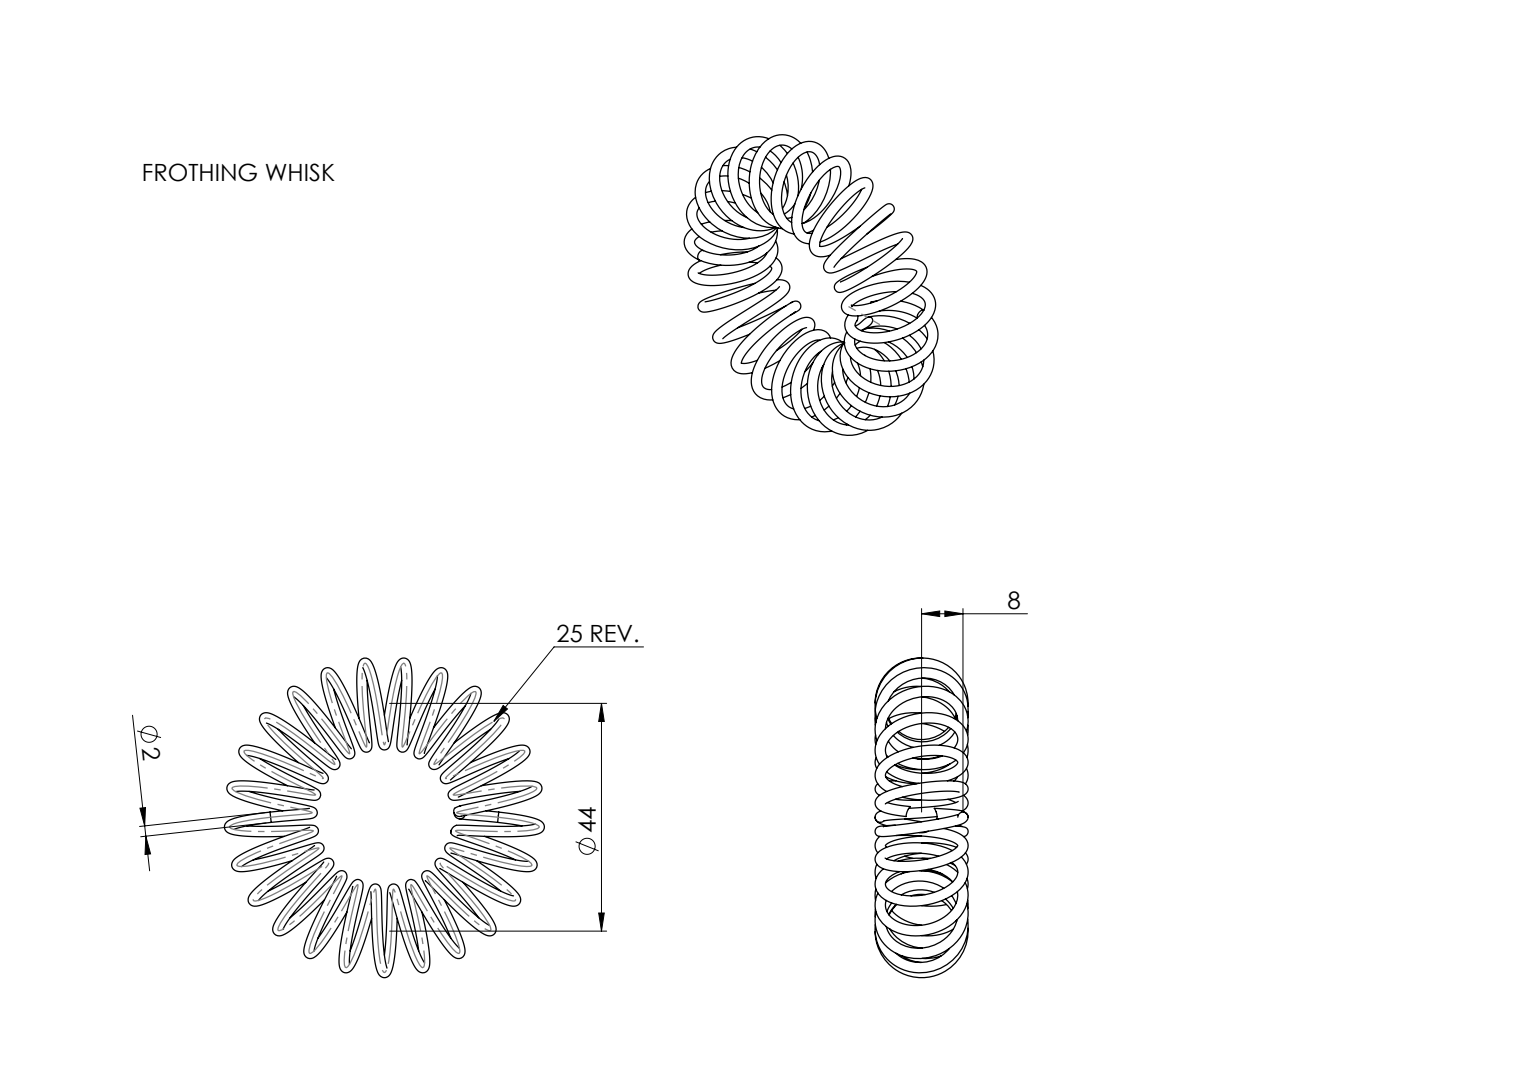
ISO-10303-21;
HEADER;
FILE_DESCRIPTION (('STEP AP214'),
    '1' );
FILE_NAME ('Frothing Whisk.step',
    '2026-10-08T15:02:10',
    ( '' ),
    ( '' ),
    'SwSTEP 2.0',
    'SolidWorks 2026',
    '' );
FILE_SCHEMA (( 'AUTOMOTIVE_DESIGN' ));
ENDSEC;

DATA;
#1=CARTESIAN_POINT ( 'NONE',  ( -16.20471097821853235, -2.781505378741172319, -220.1484675126197317 ) ) ;
#2=CARTESIAN_POINT ( 'NONE',  ( -19.86079186537285324, -0.7838168488858909821, -215.1601656726509475 ) ) ;
#3=CARTESIAN_POINT ( 'NONE',  ( -18.57671526409105667, -15.84599122335686161, -218.9973662248357300 ) ) ;
#5=CARTESIAN_POINT ( 'NONE',  ( 13.07616324839670341, -23.69356132834180784, -230.7206382488779184 ) ) ;
#6=CARTESIAN_POINT ( 'NONE',  ( -16.32047052250102581, 2.570795953410685009, -230.9329235942756213 ) ) ;
#7=CARTESIAN_POINT ( 'NONE',  ( 10.40160332990717151, 27.59713857063802323, -221.5374724512453213 ) ) ;
#8=CARTESIAN_POINT ( 'NONE',  ( -4.824452364631481416, 22.01523768541901305, -216.8350837474290245 ) ) ;
#10=CARTESIAN_POINT ( 'NONE',  ( 20.64894435305043174, -4.471500992710556233, -235.2405168901568686 ) ) ;
#12=CARTESIAN_POINT ( 'NONE',  ( 12.99034161053428349, 11.71468708507361889, -230.9043293568357740 ) ) ;
#13=CARTESIAN_POINT ( 'NONE',  ( -7.812160407601123069, 10.19183344000749081, -223.8148904943605828 ) ) ;
#14=CARTESIAN_POINT ( 'NONE',  ( -12.30606003331388543, 10.59782772616791036, -231.0021630509705801 ) ) ;
#15=CARTESIAN_POINT ( 'NONE',  ( -11.57846532275044460, -10.37575015818511304, -229.3776965522603462 ) ) ;
#17=CARTESIAN_POINT ( 'NONE',  ( 16.21758812354607215, 4.665393561625732488, -232.5634757513959983 ) ) ;
#18=CARTESIAN_POINT ( 'NONE',  ( -25.36936018126600345, 11.57160208538938306, -224.9662154788713622 ) ) ;
#19=CARTESIAN_POINT ( 'NONE',  ( 16.71363093372661979, 20.70203100498337179, -215.6856694095356488 ) ) ;
#20=CARTESIAN_POINT ( 'NONE',  ( 25.85597688020959239, 3.954559836939000039, -230.6766427064781624 ) ) ;
#22=CARTESIAN_POINT ( 'NONE',  ( -4.451292041429703694, -15.86428280493796628, -231.0943874731633798 ) ) ;
#24=CARTESIAN_POINT ( 'NONE',  ( -8.978805095734141872, -14.89723076936793156, -219.0730636071341451 ) ) ;
#25=CARTESIAN_POINT ( 'NONE',  ( -4.813101935419741295, 13.68373293383429434, -229.7840611589179503 ) ) ;
#26=CARTESIAN_POINT ( 'NONE',  ( 1.541778504653760429, -23.48174737203985529, -233.9922866444541967 ) ) ;
#27=CARTESIAN_POINT ( 'NONE',  ( -7.395406416482832590, 12.93623984139929739, -219.2606224730616873 ) ) ;
#28=CARTESIAN_POINT ( 'NONE',  ( 22.70267758588118312, -6.899298642777032420, -215.6456595153534863 ) ) ;
#30=CARTESIAN_POINT ( 'NONE',  ( -13.52935284690462758, -5.503084506376929141, -222.3607690796775671 ) ) ;
#31=CARTESIAN_POINT ( 'NONE',  ( -14.58575946311604277, 2.190332613129932327, -228.6717927865686590 ) ) ;
#33=CARTESIAN_POINT ( 'NONE',  ( -3.139695637132168038, 25.12735071829084177, -230.1469660918596389 ) ) ;
#34=CARTESIAN_POINT ( 'NONE',  ( 18.30177952310522471, 1.918278963380847468, -233.8574151782075887 ) ) ;
#35=CARTESIAN_POINT ( 'NONE',  ( 7.639528166734322667, 11.92751229241157596, -224.6077814063189635 ) ) ;
#36=CARTESIAN_POINT ( 'NONE',  ( 12.15450584778660570, 2.288537795953278220, -225.7049340319972828 ) ) ;
#37=CARTESIAN_POINT ( 'NONE',  ( -3.630465294598614889, -13.73165509241056093, -221.1424077787270619 ) ) ;
#38=CARTESIAN_POINT ( 'NONE',  ( 8.546572992885776543, 19.06776382077057974, -214.7173484156796519 ) ) ;
#40=CARTESIAN_POINT ( 'NONE',  ( 8.654719819004025538, -19.13368099829532909, -232.5229659899653711 ) ) ;
#41=CARTESIAN_POINT ( 'NONE',  ( -9.661739055621840322, 20.41227307912577871, -232.0920144483423257 ) ) ;
#42=CARTESIAN_POINT ( 'NONE',  ( 3.192353461299334061, 22.13718518159985393, -217.1103300728619843 ) ) ;
#43=CARTESIAN_POINT ( 'NONE',  ( -21.08965452150356867, -10.66825825602615296, -217.1903588586143314 ) ) ;
#44=CARTESIAN_POINT ( 'NONE',  ( 28.65393683769942967, 4.398063292302325067, -219.1542358361629965 ) ) ;
#45=CARTESIAN_POINT ( 'NONE',  ( 12.56362091610784049, 9.747446748398973071, -231.6428467497164547 ) ) ;
#47=CARTESIAN_POINT ( 'NONE',  ( 9.333020543840051531, 16.91085096921651143, -217.7308990335875762 ) ) ;
#48=CARTESIAN_POINT ( 'NONE',  ( 25.31834813234691595, -9.473547856983202564, -230.2364162768838298 ) ) ;
#49=CARTESIAN_POINT ( 'NONE',  ( 12.90474009670415967, -3.145873754258878385, -224.5449843457338375 ) ) ;
#51=CARTESIAN_POINT ( 'NONE',  ( 13.61707622192329481, 14.84143455326118932, -217.6958999636067063 ) ) ;
#52=CARTESIAN_POINT ( 'NONE',  ( -13.46535974834342220, -4.471564630954283359, -230.9063312536467834 ) ) ;
#53=CARTESIAN_POINT ( 'NONE',  ( -6.870552667427666904, -18.85419487977974029, -216.2130481585807047 ) ) ;
#54=CARTESIAN_POINT ( 'NONE',  ( 5.609436632608550966, -13.11664087352601094, -229.3324225951633650 ) ) ;
#55=CARTESIAN_POINT ( 'NONE',  ( -1.364406401035816785, 24.33111505239456918, -219.5658712396381418 ) ) ;
#56=CARTESIAN_POINT ( 'NONE',  ( 20.41968681625622040, 10.18377600976054076, -218.1989382652844256 ) ) ;
#57=CARTESIAN_POINT ( 'NONE',  ( -26.58771759052039485, 5.114955214121561511, -218.2823714869195442 ) ) ;
#58=CARTESIAN_POINT ( 'NONE',  ( -9.106229537879125147, 25.89784491087598184, -228.9807674929363372 ) ) ;
#59=CARTESIAN_POINT ( 'NONE',  ( -21.75565187119130428, -2.221346625543990427, -217.0768970814220609 ) ) ;
#62=CARTESIAN_POINT ( 'NONE',  ( -11.85645341316062051, 18.51497629668490674, -217.8828067666886454 ) ) ;
#63=CARTESIAN_POINT ( 'NONE',  ( 15.88043104796248528, 11.88135572392608807, -216.2525917828042168 ) ) ;
#64=CARTESIAN_POINT ( 'NONE',  ( 24.00840102751045890, 17.37402299239434100, -218.3110108534040137 ) ) ;
#66=CARTESIAN_POINT ( 'NONE',  ( 27.81506808824343580, -10.52944849582878106, -221.0913368219556503 ) ) ;
#69=CARTESIAN_POINT ( 'NONE',  ( -8.172572110426221670, 16.86653848210977813, -233.4220330256369493 ) ) ;
#70=EDGE_CURVE ( 'NONE', #4018, #8552, #5732, .T. ) ;
#71=CARTESIAN_POINT ( 'NONE',  ( -12.00435701841128022, -1.798699874815819166, -227.7674894005143074 ) ) ;
#74=CARTESIAN_POINT ( 'NONE',  ( 14.73698509926073186, 4.443590625350892331, -227.4062002049096236 ) ) ;
#75=CARTESIAN_POINT ( 'NONE',  ( -13.69675006931110417, 3.702342960760605539, -228.0723273272095355 ) ) ;
#76=CARTESIAN_POINT ( 'NONE',  ( 9.104026917753444081, -10.66572815660443041, -221.9193219976906448 ) ) ;
#78=CARTESIAN_POINT ( 'NONE',  ( -27.82842955277035202, 11.70195273568964112, -227.9294339757464911 ) ) ;
#80=CARTESIAN_POINT ( 'NONE',  ( -15.15434969228324924, 4.423874646950748613, -230.6144467931089821 ) ) ;
#81=CARTESIAN_POINT ( 'NONE',  ( 1.102456202203287550, -23.13885590315818064, -232.0370787247644557 ) ) ;
#85=CARTESIAN_POINT ( 'NONE',  ( -28.13472254077564116, 12.33996625515159629, -224.9141344439281909 ) ) ;
#86=CARTESIAN_POINT ( 'NONE',  ( 17.16551562789753049, -17.52877442517796780, -218.8649675774640286 ) ) ;
#87=CARTESIAN_POINT ( 'NONE',  ( 12.82607305708569889, -2.701876713238477556, -226.3171933651010761 ) ) ;
#90=CARTESIAN_POINT ( 'NONE',  ( 10.01015180241662605, 20.19019600914695900, -219.1042218506083543 ) ) ;
#92=CARTESIAN_POINT ( 'NONE',  ( 14.78510113471881304, 14.77128235908076803, -230.8056908117964383 ) ) ;
#93=CARTESIAN_POINT ( 'NONE',  ( -2.652888268066178945, -28.18865072326549637, -221.4226523288203623 ) ) ;
#94=CARTESIAN_POINT ( 'NONE',  ( 15.54083024098960486, -10.44392130763852222, -217.6620978190037476 ) ) ;
#96=CARTESIAN_POINT ( 'NONE',  ( -12.43544732248594720, 12.69828336922617318, -219.3367909706387877 ) ) ;
#97=CARTESIAN_POINT ( 'NONE',  ( -24.92290506463145405, 6.124412323591598373, -220.3779252408000104 ) ) ;
#98=CARTESIAN_POINT ( 'NONE',  ( -12.45629340980802269, 5.675423426979704367, -220.8874502847910719 ) ) ;
#100=CARTESIAN_POINT ( 'NONE',  ( -11.04629350503636864, -16.47921676447750983, -219.6257371594006145 ) ) ;
#103=CARTESIAN_POINT ( 'NONE',  ( 22.37138132874926910, 6.723028048925958622, -217.7073806909121743 ) ) ;
#104=CARTESIAN_POINT ( 'NONE',  ( 19.38320831645075870, -15.01455373846949293, -219.3474289024948689 ) ) ;
#105=CARTESIAN_POINT ( 'NONE',  ( 4.603870848087811218, 30.13529352683433515, -225.9623629403671430 ) ) ;
#106=CARTESIAN_POINT ( 'NONE',  ( -16.65698539163286540, 11.03290537638306112, -233.6474915129378758 ) ) ;
#109=CARTESIAN_POINT ( 'NONE',  ( 12.66989206167516357, 2.082990619159506007, -225.6419847029432901 ) ) ;
#111=CARTESIAN_POINT ( 'NONE',  ( 7.168644370073567806, 19.32044210858112265, -233.1278450877711634 ) ) ;
#112=CARTESIAN_POINT ( 'NONE',  ( 22.03647168420945590, 0.3315607655625663064, -232.0572713672586644 ) ) ;
#113=CARTESIAN_POINT ( 'NONE',  ( 6.589392574981438599, -17.08498810221841069, -232.9613445306918322 ) ) ;
#114=CARTESIAN_POINT ( 'NONE',  ( 14.31589812732703670, -5.349901619299376243, -221.2752230612865105 ) ) ;
#117=CARTESIAN_POINT ( 'NONE',  ( 15.01439307471096463, 1.118969480519667048, -226.7488225241675366 ) ) ;
#118=CARTESIAN_POINT ( 'NONE',  ( -15.02551512915570697, -20.93241195546420741, -218.9083119944682778 ) ) ;
#119=VECTOR ( 'NONE', #1597, 1000.000000000000000 ) ;
#121=CARTESIAN_POINT ( 'NONE',  ( -22.13857085231108712, 6.545953331035805789, -217.2801712530867633 ) ) ;
#122=CARTESIAN_POINT ( 'NONE',  ( -0.3197916200495275474, 16.38897215927557482, -229.9606066735827028 ) ) ;
#123=CARTESIAN_POINT ( 'NONE',  ( 2.085064686336211892, 14.99578618537741548, -226.0985834012817861 ) ) ;
#124=CARTESIAN_POINT ( 'NONE',  ( -27.59531865868800082, -2.367229732415436771, -222.8128998708299093 ) ) ;
#125=CARTESIAN_POINT ( 'NONE',  ( 7.995304978256253747, 13.28024228361502779, -220.6535174700288451 ) ) ;
#126=CARTESIAN_POINT ( 'NONE',  ( -10.95054816480499760, 8.339404316518379545, -224.1596700080921778 ) ) ;
#127=CARTESIAN_POINT ( 'NONE',  ( -16.40443871513620522, 4.023423476741658789, -228.9829044427089002 ) ) ;
#128=CARTESIAN_POINT ( 'NONE',  ( -11.18311023676720062, -15.30649302686804347, -231.8766562234714002 ) ) ;
#130=CARTESIAN_POINT ( 'NONE',  ( 20.76808360334631232, 5.412616674732960931, -234.1222385626545304 ) ) ;
#132=CARTESIAN_POINT ( 'NONE',  ( -14.22959263369750182, 18.28478771081826793, -217.8090497856120464 ) ) ;
#134=CARTESIAN_POINT ( 'NONE',  ( 5.964915545484365644, 11.50358694729900577, -229.9646467236423462 ) ) ;
#135=CARTESIAN_POINT ( 'NONE',  ( -21.08008464085897060, -0.9048411197481797119, -217.0000000010748522 ) ) ;
#136=CARTESIAN_POINT ( 'NONE',  ( -20.47121909278842722, -2.147015668718357695, -235.2226201655121258 ) ) ;
#138=CARTESIAN_POINT ( 'NONE',  ( -28.43596199216294806, -10.51226423640377838, -227.0041752157952430 ) ) ;
#139=CARTESIAN_POINT ( 'NONE',  ( -15.64710113362562183, 25.90300453978063189, -220.8637308366217269 ) ) ;
#140=CARTESIAN_POINT ( 'NONE',  ( -5.525229149912007642, -13.32411127922494742, -220.4018445532201440 ) ) ;
#141=CARTESIAN_POINT ( 'NONE',  ( -4.620781219515533778, 16.99182040716223696, -217.1278208835672672 ) ) ;
#142=CARTESIAN_POINT ( 'NONE',  ( 29.03861746756086859, -6.579333063807603743, -229.8282242506458317 ) ) ;
#143=CARTESIAN_POINT ( 'NONE',  ( -29.22168435891936156, -1.352755938724206519, -225.9547066689444250 ) ) ;
#144=CARTESIAN_POINT ( 'NONE',  ( 29.81944548462877975, 8.043843257819576209, -228.1755181449411793 ) ) ;
#146=CARTESIAN_POINT ( 'NONE',  ( -0.7879796667336372851, 21.22375955577181372, -219.1554080315090118 ) ) ;
#147=CARTESIAN_POINT ( 'NONE',  ( -29.16153046926437753, 6.356672163541281506, -226.4393515956758165 ) ) ;
#148=CARTESIAN_POINT ( 'NONE',  ( 18.76922974182421555, 13.12635134380198210, -217.8010375391909008 ) ) ;
#149=CARTESIAN_POINT ( 'NONE',  ( 19.55931020704464274, 3.833820734573247346, -215.4549349108404783 ) ) ;
#150=CARTESIAN_POINT ( 'NONE',  ( 3.585135836405817233, -11.76492230538331896, -228.1718440842192024 ) ) ;
#151=CARTESIAN_POINT ( 'NONE',  ( 1.660345614755502686, 12.19060476922103931, -223.1112690039082906 ) ) ;
#154=CARTESIAN_POINT ( 'NONE',  ( 0.5037192024386412115, -21.28831724695581684, -215.7417742237681466 ) ) ;
#155=CARTESIAN_POINT ( 'NONE',  ( -8.317278876689359279, 23.15034512777772235, -218.2935523245793092 ) ) ;
#156=CARTESIAN_POINT ( 'NONE',  ( 14.20064147608437821, 14.63411858269657806, -233.6150408276221242 ) ) ;
#157=CARTESIAN_POINT ( 'NONE',  ( -26.43144772945995413, -6.745116643720071359, -219.5134289301136050 ) ) ;
#158=CARTESIAN_POINT ( 'NONE',  ( -22.38528940623734798, 16.50235888036280230, -227.1443357386333162 ) ) ;
#159=CARTESIAN_POINT ( 'NONE',  ( -17.89085717681497201, 10.08962028281416856, -232.3705156551908431 ) ) ;
#160=CARTESIAN_POINT ( 'NONE',  ( 27.79670308438203108, 10.67628923451848877, -225.2981230784098727 ) ) ;
#161=VERTEX_POINT ( 'NONE', #16052 ) ;
#162=CARTESIAN_POINT ( 'NONE',  ( 12.23063869552301242, 12.84118223717021934, -218.8273164334868284 ) ) ;
#163=CARTESIAN_POINT ( 'NONE',  ( 10.59565547865383728, -13.75865772189005476, -221.5384683668846435 ) ) ;
#165=CARTESIAN_POINT ( 'NONE',  ( 27.76845665997775114, -9.103683020204879739, -229.9743915588940979 ) ) ;
#166=CARTESIAN_POINT ( 'NONE',  ( -0.6272116608575281083, 20.18031380156121202, -219.3960054794027030 ) ) ;
#170=CARTESIAN_POINT ( 'NONE',  ( 23.04897566969193079, 17.95862962700741861, -223.6438515760422661 ) ) ;
#171=CARTESIAN_POINT ( 'NONE',  ( -11.65988442122670676, -3.998659314375652141, -223.4258670541443621 ) ) ;
#172=CARTESIAN_POINT ( 'NONE',  ( -5.902479482706956659, -14.78727544128710214, -218.5565286504736946 ) ) ;
#173=CARTESIAN_POINT ( 'NONE',  ( 13.04434844185555420, -10.19049307777131297, -230.8679447648462713 ) ) ;
#174=CARTESIAN_POINT ( 'NONE',  ( -7.366083718505351818, 19.86648438590005838, -231.8662444779758971 ) ) ;
#176=CARTESIAN_POINT ( 'NONE',  ( 17.02590609996173754, 6.796709046606974169, -230.8496778635019098 ) ) ;
#177=CARTESIAN_POINT ( 'NONE',  ( -13.55591840520136770, 8.363404288414606924, -231.2690188357804857 ) ) ;
#178=CARTESIAN_POINT ( 'NONE',  ( -5.589224416770360193, 14.13652937339764115, -225.1481999119820330 ) ) ;
#180=CARTESIAN_POINT ( 'NONE',  ( 5.359747511823000465, 20.14556701535824601, -232.9094821222151381 ) ) ;
#181=CARTESIAN_POINT ( 'NONE',  ( -18.90911063232017142, 5.352531560950812839, -219.6301177803536575 ) ) ;
#182=CARTESIAN_POINT ( 'NONE',  ( 13.85207896949186335, 7.847214149978243292, -217.3457543576531066 ) ) ;
#183=CARTESIAN_POINT ( 'NONE',  ( 5.133806223762193532, -16.42362916962670383, -230.4968203642818310 ) ) ;
#187=CARTESIAN_POINT ( 'NONE',  ( -6.101488798441174310, 11.33371047077072369, -225.3616985956418546 ) ) ;
#188=CARTESIAN_POINT ( 'NONE',  ( -25.17982544627478703, 0.9072515815786372784, -215.5253307415545692 ) ) ;
#189=CARTESIAN_POINT ( 'NONE',  ( 26.48152825632016061, -2.044474411990439666, -219.3412966555575565 ) ) ;
#190=CARTESIAN_POINT ( 'NONE',  ( 25.69300549816939494, 5.947472783069708946, -230.6131061331718115 ) ) ;
#191=FACE_OUTER_BOUND ( 'NONE', #11098, .T. ) ;
#193=CARTESIAN_POINT ( 'NONE',  ( 20.25084204406298127, -10.11176871144018818, -232.7817218064674591 ) ) ;
#194=CARTESIAN_POINT ( 'NONE',  ( -8.823862513872974489, 14.92351368520778898, -217.1499513473673346 ) ) ;
#195=CARTESIAN_POINT ( 'NONE',  ( -28.17543631911187063, 3.557555778861649642, -230.1980773687482156 ) ) ;
#196=CARTESIAN_POINT ( 'NONE',  ( -1.432270239486107766, -17.91381153981195951, -219.1344183636291802 ) ) ;
#200=CARTESIAN_POINT ( 'NONE',  ( -20.18153419852512442, 14.25141268122526483, -233.5059133483111964 ) ) ;
#201=CARTESIAN_POINT ( 'NONE',  ( 23.31955656579280145, -13.39010844438576520, -228.3495985225334266 ) ) ;
#202=CARTESIAN_POINT ( 'NONE',  ( -27.85133024402786006, -1.794102530182491773, -229.4204807338591081 ) ) ;
#204=CARTESIAN_POINT ( 'NONE',  ( 24.14003655968566520, 13.76285650325712773, -228.1266575292093819 ) ) ;
#205=CARTESIAN_POINT ( 'NONE',  ( -4.813101935419741295, 13.68373293383429434, -229.7840611589179503 ) ) ;
#206=CARTESIAN_POINT ( 'NONE',  ( 17.42772712443221650, 11.35756022693713341, -231.2166398222404382 ) ) ;
#207=CARTESIAN_POINT ( 'NONE',  ( -7.194605141218047173, -25.04260655977047278, -230.2952862975163271 ) ) ;
#209=CARTESIAN_POINT ( 'NONE',  ( 23.45680152528306550, 2.072154465955917235, -232.7243927205664704 ) ) ;
#212=CARTESIAN_POINT ( 'NONE',  ( 2.579827969572558111, 15.91317371615649101, -219.7652087782269916 ) ) ;
#213=CARTESIAN_POINT ( 'NONE',  ( -22.90687623753526125, 9.466200233939549236, -230.1557007022273638 ) ) ;
#214=CARTESIAN_POINT ( 'NONE',  ( -30.35034897870229287, 7.696526532841741819, -221.5749790623549416 ) ) ;
#216=CARTESIAN_POINT ( 'NONE',  ( -12.46707500365009480, -15.03319212650626824, -230.3369784839848933 ) ) ;
#219=CARTESIAN_POINT ( 'NONE',  ( 24.78222556642275620, 17.97262539535998371, -226.6641400693514470 ) ) ;
#220=CARTESIAN_POINT ( 'NONE',  ( 18.79065350309113214, -20.33706828427738600, -226.6662063318914591 ) ) ;
#221=CARTESIAN_POINT ( 'NONE',  ( 23.49048926389013658, 9.645778135078892035, -218.7307869890797463 ) ) ;
#222=CARTESIAN_POINT ( 'NONE',  ( -16.39453490553961856, 20.24836633112041184, -233.1722131570092245 ) ) ;
#224=CARTESIAN_POINT ( 'NONE',  ( 14.54999166170408209, 3.068772298969228096, -219.4784171371563275 ) ) ;
#226=CARTESIAN_POINT ( 'NONE',  ( 13.43170911749896490, 19.07691563292472026, -232.7497845103644636 ) ) ;
#228=CARTESIAN_POINT ( 'NONE',  ( 6.427665535191954937, -16.40046818492683656, -232.5919299485929912 ) ) ;
#229=CARTESIAN_POINT ( 'NONE',  ( 11.43609017326686050, -13.06727081285745307, -217.8903327850316316 ) ) ;
#232=CARTESIAN_POINT ( 'NONE',  ( -23.95129667199961077, 20.99391807043993552, -227.1541646794576081 ) ) ;
#233=CARTESIAN_POINT ( 'NONE',  ( -22.78589867900506150, -1.373495078166624861, -218.8339345403132370 ) ) ;
#234=CARTESIAN_POINT ( 'NONE',  ( 30.47710800431509170, 7.409378661937554789, -223.2007768404241688 ) ) ;
#235=CARTESIAN_POINT ( 'NONE',  ( -1.301562195391901877, 16.19210386685474390, -220.0867867038183192 ) ) ;
#236=CARTESIAN_POINT ( 'NONE',  ( 1.847452069095833593, 15.11597492720254543, -223.6261404253179421 ) ) ;
#238=CARTESIAN_POINT ( 'NONE',  ( 14.54962894845190036, -2.357901078066860112, -232.0046840244626765 ) ) ;
#240=CARTESIAN_POINT ( 'NONE',  ( 22.66390650824515873, 11.48342577402021725, -231.3155567808436217 ) ) ;
#241=CARTESIAN_POINT ( 'NONE',  ( -11.10182655035041144, 8.778638955377752850, -227.1050196202568827 ) ) ;
#242=CARTESIAN_POINT ( 'NONE',  ( -12.26337789213896201, 9.274758280606999250, -219.9806108963443876 ) ) ;
#243=CARTESIAN_POINT ( 'NONE',  ( -24.60063047153272819, -17.11178239752603858, -226.7032704813509554 ) ) ;
#244=CARTESIAN_POINT ( 'NONE',  ( -16.63766460830045091, 5.158675778507696208, -232.1659425527909093 ) ) ;
#248=CARTESIAN_POINT ( 'NONE',  ( -12.04619960554013502, 10.22290173510000777, -223.1766370265664534 ) ) ;
#249=CARTESIAN_POINT ( 'NONE',  ( 25.41781277602550304, 19.49958712797920057, -223.1230538376805441 ) ) ;
#251=CARTESIAN_POINT ( 'NONE',  ( 27.84414217501293010, 2.965433895642837214, -221.8999927093654492 ) ) ;
#252=CARTESIAN_POINT ( 'NONE',  ( -13.00317340065129557, -2.278067296278880161, -219.8118061108488916 ) ) ;
#254=CARTESIAN_POINT ( 'NONE',  ( -23.08212926897555306, -14.71479305961103101, -218.7697472404056214 ) ) ;
#255=CARTESIAN_POINT ( 'NONE',  ( -7.312583518931054627, 16.22063427959223958, -217.3454962955413521 ) ) ;
#256=CARTESIAN_POINT ( 'NONE',  ( -14.34280792637948743, -22.10828917559366147, -217.4172704053049756 ) ) ;
#257=CARTESIAN_POINT ( 'NONE',  ( 7.743212835174657194, 11.90778931056080481, -226.0491028376908105 ) ) ;
#258=CARTESIAN_POINT ( 'NONE',  ( 6.415926650623908323, -16.27382107952271895, -215.7995092914603674 ) ) ;
#259=CARTESIAN_POINT ( 'NONE',  ( 14.03461600111380037, -0.1787097712218918000, -227.9951367205099473 ) ) ;
#260=CARTESIAN_POINT ( 'NONE',  ( -28.61025869263052712, 6.891613135096296361, -222.2489362813765013 ) ) ;
#261=CARTESIAN_POINT ( 'NONE',  ( -5.764806379010653181, 14.19340719117484007, -223.8851086052821415 ) ) ;
#262=CARTESIAN_POINT ( 'NONE',  ( 26.06405806384012536, 5.488112530166501024, -216.5020692413490622 ) ) ;
#263=CARTESIAN_POINT ( 'NONE',  ( -13.56011990957801139, -0.3895158544032599202, -219.3211261236655218 ) ) ;
#264=CARTESIAN_POINT ( 'NONE',  ( 12.79953165872901266, 10.20044330008568778, -230.3912386799665626 ) ) ;
#265=CARTESIAN_POINT ( 'NONE',  ( -0.4062606655315902371, -23.43967590431752512, -234.4451928229410100 ) ) ;
#266=CARTESIAN_POINT ( 'NONE',  ( 5.264801124131998300, 10.54092478143144795, -226.4890466082630098 ) ) ;
#267=CARTESIAN_POINT ( 'NONE',  ( 21.31262902390056624, 0.4111834581965390645, -232.0572713672585792 ) ) ;
#268=CARTESIAN_POINT ( 'NONE',  ( 0.2152704783746036410, -12.84635275796930642, -226.1081088095504015 ) ) ;
#269=CARTESIAN_POINT ( 'NONE',  ( -11.85645341316062051, 18.51497629668490674, -217.8828067666886454 ) ) ;
#270=CARTESIAN_POINT ( 'NONE',  ( 12.74913679152205148, 9.185760885856177893, -218.6542381594888980 ) ) ;
#271=CARTESIAN_POINT ( 'NONE',  ( -27.88251101234890328, -7.575382714962081820, -221.6715981084135478 ) ) ;
#272=CARTESIAN_POINT ( 'NONE',  ( -18.90911063232017142, 5.352531560950812839, -219.6301177803536575 ) ) ;
#274=CARTESIAN_POINT ( 'NONE',  ( -4.678665819194652187, 12.50541869316310262, -220.1509054161798247 ) ) ;
#275=CARTESIAN_POINT ( 'NONE',  ( 13.89183999136464820, 6.553741795688899252, -220.8646181278399752 ) ) ;
#277=CARTESIAN_POINT ( 'NONE',  ( 10.85678324124089755, -13.97331853324622131, -221.1336851750754420 ) ) ;
#279=CARTESIAN_POINT ( 'NONE',  ( 5.511302051500400090, -18.01881380728196902, -231.5522404100356084 ) ) ;
#280=CARTESIAN_POINT ( 'NONE',  ( -7.928079932584687128, 26.12067226064367986, -221.2051195461628197 ) ) ;
#283=CARTESIAN_POINT ( 'NONE',  ( 21.25094435758043332, 17.68230636442804027, -229.7964888993842010 ) ) ;
#284=CARTESIAN_POINT ( 'NONE',  ( 26.54225689383817866, -6.924125931238839016, -230.1506921200174247 ) ) ;
#285=CARTESIAN_POINT ( 'NONE',  ( -1.632242579688942596, -13.62074943359385415, -221.1585305289511041 ) ) ;
#286=CARTESIAN_POINT ( 'NONE',  ( -3.300598509645395584, -18.18730530649546395, -233.4303386612170925 ) ) ;
#287=CARTESIAN_POINT ( 'NONE',  ( -2.015708574708954259, 26.78900769828807782, -221.5371848586876808 ) ) ;
#289=CARTESIAN_POINT ( 'NONE',  ( 17.24423567610276109, 8.542587572837451404, -218.6562240232607621 ) ) ;
#290=CARTESIAN_POINT ( 'NONE',  ( -11.26857159993117996, 28.96895336474501192, -225.6039696848669678 ) ) ;
#291=CARTESIAN_POINT ( 'NONE',  ( -8.463283775975803280, 12.69606588598396613, -228.6351674091961286 ) ) ;
#293=CARTESIAN_POINT ( 'NONE',  ( -1.433739110790628102, 17.19322394474796667, -219.1420620387681879 ) ) ;
#294=CARTESIAN_POINT ( 'NONE',  ( -16.37512411505367282, 2.406627362596846620, -227.7341547288202719 ) ) ;
#295=CARTESIAN_POINT ( 'NONE',  ( 7.651502705057454889, 16.60422307457919544, -215.4679461133464144 ) ) ;
#296=CARTESIAN_POINT ( 'NONE',  ( 5.452943511046377090, -14.64908918772281865, -221.6090591728701611 ) ) ;
#299=CARTESIAN_POINT ( 'NONE',  ( -11.69688825528096388, 18.63404371591177622, -215.8612738028812714 ) ) ;
#300=CARTESIAN_POINT ( 'NONE',  ( 21.83031488338151149, -1.542591969257156803, -231.3901500139511427 ) ) ;
#301=CARTESIAN_POINT ( 'NONE',  ( 27.02029988085337919, -0.4174685747284823112, -230.1188858631967378 ) ) ;
#302=CARTESIAN_POINT ( 'NONE',  ( 13.03557269046774714, 7.519834803053426775, -226.9490612297269081 ) ) ;
#303=CARTESIAN_POINT ( 'NONE',  ( -13.65925618638770800, 3.289586759644148817, -222.1579143493116533 ) ) ;
#304=CARTESIAN_POINT ( 'NONE',  ( 5.451525948382545117, -12.45300865616632713, -227.8545162512558306 ) ) ;
#306=CARTESIAN_POINT ( 'NONE',  ( -10.30050448363967419, 10.07750059423401190, -220.1837019037183723 ) ) ;
#307=CARTESIAN_POINT ( 'NONE',  ( -12.80532875684362715, 24.61139456694233374, -232.5885756414849084 ) ) ;
#308=CARTESIAN_POINT ( 'NONE',  ( -16.71711190488355570, 0.6105529133557690002, -230.9511258789794681 ) ) ;
#309=CARTESIAN_POINT ( 'NONE',  ( -13.02663300398358892, -17.15584419188240162, -232.5492131852532793 ) ) ;
#312=CARTESIAN_POINT ( 'NONE',  ( -13.65925618638770800, 3.289586759644148817, -222.1579143493116533 ) ) ;
#313=CARTESIAN_POINT ( 'NONE',  ( 8.958604797576050771, -20.52636309154128114, -232.6441826665315205 ) ) ;
#315=EDGE_CURVE ( 'NONE', #15629, #11616, #21983, .T. ) ;
#317=CARTESIAN_POINT ( 'NONE',  ( 20.64430047260004031, 12.67811357335941480, -231.0449411089858813 ) ) ;
#318=CARTESIAN_POINT ( 'NONE',  ( -12.38801939673351704, 9.361418580567464787, -232.8075769614211765 ) ) ;
#321=CARTESIAN_POINT ( 'NONE',  ( 11.40028598017942230, 13.60807601628675023, -220.9105305289655519 ) ) ;
#322=CARTESIAN_POINT ( 'NONE',  ( 2.859576749041432553, -13.55982619688326984, -227.5954719880151345 ) ) ;
#323=CARTESIAN_POINT ( 'NONE',  ( 22.47485217157460724, -0.5904823501021798648, -216.4383471256914220 ) ) ;
#325=CARTESIAN_POINT ( 'NONE',  ( -4.784012432433236484, 23.31984772163034947, -232.0554186943449508 ) ) ;
#326=CARTESIAN_POINT ( 'NONE',  ( -27.32939371162572684, 5.861081283609568260, -224.9659309793921409 ) ) ;
#327=CARTESIAN_POINT ( 'NONE',  ( -20.76981451797363576, 10.27702766794165257, -234.3988437453480742 ) ) ;
#329=CARTESIAN_POINT ( 'NONE',  ( -13.78780214743967214, -7.867619234746639378, -226.3818292120506044 ) ) ;
#332=CARTESIAN_POINT ( 'NONE',  ( 15.21408433160105034, 3.021350230896802103, -222.3056493717910769 ) ) ;
#333=CARTESIAN_POINT ( 'NONE',  ( -2.392195434554431177, -23.29395655963766387, -232.4094703796048691 ) ) ;
#334=CARTESIAN_POINT ( 'NONE',  ( 13.49011766416699842, 7.659170998773840111, -228.1905628957712793 ) ) ;
#335=CARTESIAN_POINT ( 'NONE',  ( -19.00318367631585659, 13.14621133775862916, -233.8403879275295765 ) ) ;
#337=CARTESIAN_POINT ( 'NONE',  ( 22.49659352743751128, 7.060662713609715979, -215.7089950799439180 ) ) ;
#338=CARTESIAN_POINT ( 'NONE',  ( 11.33210854356620523, 22.81476816607802149, -217.8536224460118262 ) ) ;
#340=CARTESIAN_POINT ( 'NONE',  ( 2.378655016347637652, -14.31292064579845302, -219.9942319014987220 ) ) ;
#341=CARTESIAN_POINT ( 'NONE',  ( 14.02668320743028119, -5.282748560960272677, -221.9001732195871739 ) ) ;
#344=CARTESIAN_POINT ( 'NONE',  ( -22.56222084847001597, 18.89892770556097901, -231.8972396388394088 ) ) ;
#345=CARTESIAN_POINT ( 'NONE',  ( -21.86011749369748713, -1.271659148212478385, -218.8339345395071689 ) ) ;
#346=CARTESIAN_POINT ( 'NONE',  ( 18.30177952310522471, 1.918278963380847468, -233.8574151782075887 ) ) ;
#347=CARTESIAN_POINT ( 'NONE',  ( -1.433739110790628102, 17.19322394474796667, -219.1420620387681879 ) ) ;
#348=CARTESIAN_POINT ( 'NONE',  ( 5.563568780623874943, 21.86458082533069103, -218.6474243140849012 ) ) ;
#350=CARTESIAN_POINT ( 'NONE',  ( 16.60513614482655598, -17.51558294309126396, -234.8138649271977556 ) ) ;
#352=B_SPLINE_CURVE_WITH_KNOTS ( 'NONE', 3,
 ( #8357, #15550, #7861, #19875, #11124, #19133, #17576, #21456, #15667, #18213, #874, #4462, #19250, #14508, #21343, #11230, #7115, #13028, #2035, #4244, #2667, #20932 ),
 .UNSPECIFIED., .F., .F.,
 ( 4, 2, 2, 2, 2, 2, 2, 2, 2, 2, 4 ),
 ( 4.821909171845164511E-17, 0.0003011134387877908666, 0.0006022268775755335946, 0.001204453755151019051, 0.001806680632726504615, 0.002408907510301990396, 0.003011134387877475744, 0.003613361265452961091, 0.004215588143028446873, 0.004516701581816189547, 0.004817815020603932220 ),
 .UNSPECIFIED. ) ;
#353=CARTESIAN_POINT ( 'NONE',  ( 15.42212722119060864, 5.401662248084913465, -220.8333402320903645 ) ) ;
#354=CARTESIAN_POINT ( 'NONE',  ( -14.30096418567650041, 6.974026439069829664, -228.7941652905285537 ) ) ;
#355=CARTESIAN_POINT ( 'NONE',  ( -11.19223248830523332, 8.463078350427430507, -222.6400917074981578 ) ) ;
#356=CARTESIAN_POINT ( 'NONE',  ( -29.74115761720981510, -1.844952462305729401, -220.6656484738778943 ) ) ;
#358=CARTESIAN_POINT ( 'NONE',  ( -12.90983082593748676, 14.84936372681532823, -233.8009687022269532 ) ) ;
#360=CARTESIAN_POINT ( 'NONE',  ( 29.55842656951424985, 4.785221541509360854, -220.5134865854112718 ) ) ;
#361=CARTESIAN_POINT ( 'NONE',  ( -13.06839468023815165, 25.32320678245788059, -229.0099538679170053 ) ) ;
#362=CARTESIAN_POINT ( 'NONE',  ( 17.65694480011521250, 15.62497337860048674, -235.2008064134603273 ) ) ;
#363=CARTESIAN_POINT ( 'NONE',  ( -13.93333636822611155, 3.327141996558931947, -221.4468162587888287 ) ) ;
#364=CARTESIAN_POINT ( 'NONE',  ( -21.94322237485859972, -13.31528874885349900, -215.4027562252440759 ) ) ;
#365=B_SPLINE_CURVE_WITH_KNOTS ( 'NONE', 3,
 ( #19193, #15943, #12227, #16055, #301, #15724, #3991, #3770, #10538, #17522, #13928, #189, #519, #20763, #5345, #3654, #17407, #7171, #15832, #5457, #14265, #12340 ),
 .UNSPECIFIED., .F., .F.,
 ( 4, 2, 2, 2, 2, 2, 2, 2, 2, 2, 4 ),
 ( 0.4999446919652688059, 0.5028747035357847839, 0.5058047151063008728, 0.5087347266768169618, 0.5116647382473329397, 0.5145947498178489177, 0.5175247613883648956, 0.5204547729588808735, 0.5233847845293969625, 0.5268031313616656774, 0.5278645943380111394 ),
 .UNSPECIFIED. ) ;
#366=CARTESIAN_POINT ( 'NONE',  ( -29.90835019730369737, -3.078401082523886334, -228.7630230812432046 ) ) ;
#367=CARTESIAN_POINT ( 'NONE',  ( -19.40752943788874774, 15.61499612050012864, -234.7624367253776541 ) ) ;
#368=CARTESIAN_POINT ( 'NONE',  ( -5.519971913460887336, -12.21762732219001713, -227.2962593638428359 ) ) ;
#369=CARTESIAN_POINT ( 'NONE',  ( 8.496844655769807630, 14.66037471857024599, -219.1631158796573118 ) ) ;
#370=CARTESIAN_POINT ( 'NONE',  ( 12.77158894069672357, -20.43488010613652150, -235.1868042311012914 ) ) ;
#372=CARTESIAN_POINT ( 'NONE',  ( -16.32047052250102581, 2.570795953410685009, -230.9329235942756213 ) ) ;
#373=CARTESIAN_POINT ( 'NONE',  ( 1.296323513242173542, 20.09034598902932345, -230.5712631353794961 ) ) ;
#374=CARTESIAN_POINT ( 'NONE',  ( -16.27882490622757672, 1.520697279646460398, -219.2607721384596289 ) ) ;
#375=CARTESIAN_POINT ( 'NONE',  ( 24.57222455393806015, 12.08236629421828212, -229.7319216558644541 ) ) ;
#376=CARTESIAN_POINT ( 'NONE',  ( -22.10934047915427314, 0.9940043559354312386, -216.9999999999999716 ) ) ;
#377=CARTESIAN_POINT ( 'NONE',  ( -16.08690871037762449, -24.16943144049835368, -222.8355329163958345 ) ) ;
#378=CARTESIAN_POINT ( 'NONE',  ( 2.276720224425493821, 13.44951395023989171, -229.9230017221896105 ) ) ;
#380=CARTESIAN_POINT ( 'NONE',  ( -1.821616882984092411, -20.20372127477041246, -234.2708619787750308 ) ) ;
#381=CARTESIAN_POINT ( 'NONE',  ( -8.407534899841293097, 16.91942258446019665, -231.3029992963236339 ) ) ;
#382=CARTESIAN_POINT ( 'NONE',  ( 6.566035546683759883, 15.06745272174450712, -218.8330720708048034 ) ) ;
#383=CARTESIAN_POINT ( 'NONE',  ( -23.77327857871830830, 11.53128597905896768, -221.0855018166512025 ) ) ;
#384=CARTESIAN_POINT ( 'NONE',  ( -13.41298582792616934, 27.85383138489214616, -228.6457525465575884 ) ) ;
#385=CARTESIAN_POINT ( 'NONE',  ( 28.62253243811995418, 3.652502539191337494, -225.4068779441649326 ) ) ;
#387=CARTESIAN_POINT ( 'NONE',  ( 6.831421020708281944, -16.86748893536391591, -229.5305077739217552 ) ) ;
#388=CARTESIAN_POINT ( 'NONE',  ( 11.75796858304313375, -24.75965012883946414, -219.8219186532837455 ) ) ;
#389=CARTESIAN_POINT ( 'NONE',  ( -9.175187729848801155, 26.50888816229029743, -227.9285554593684253 ) ) ;
#391=CARTESIAN_POINT ( 'NONE',  ( 10.85888002857596923, 15.81835858589122878, -232.3913150909872627 ) ) ;
#392=CARTESIAN_POINT ( 'NONE',  ( 19.63495056682994289, -4.096126682090319271, -232.1271738766904207 ) ) ;
#393=CARTESIAN_POINT ( 'NONE',  ( -12.44777057840899559, -8.577008958641105352, -229.4809580173677830 ) ) ;
#394=CARTESIAN_POINT ( 'NONE',  ( 1.729916699924999746, -18.64927252049523432, -233.5000329212076906 ) ) ;
#395=CARTESIAN_POINT ( 'NONE',  ( -3.139695637132168038, 25.12735071829084177, -230.1469660918596389 ) ) ;
#396=CARTESIAN_POINT ( 'NONE',  ( 19.31922195716811430, 9.600631919686000160, -218.1359845693048101 ) ) ;
#397=CARTESIAN_POINT ( 'NONE',  ( -2.772442535524381579, 13.75675912271027457, -228.9770533867650215 ) ) ;
#398=CARTESIAN_POINT ( 'NONE',  ( -4.285397168228398890, 18.56782363833054106, -219.4990091916804715 ) ) ;
#400=CARTESIAN_POINT ( 'NONE',  ( 8.860681144154234801, 27.11956268701432293, -229.8503778060109823 ) ) ;
#401=CARTESIAN_POINT ( 'NONE',  ( 21.96352831578506937, -0.3315607655626218175, -233.9427286327412787 ) ) ;
#402=CARTESIAN_POINT ( 'NONE',  ( 26.50744623559791435, 1.694095366541529923, -217.6968951254705473 ) ) ;
#403=CARTESIAN_POINT ( 'NONE',  ( 5.920964624126254350, -19.79845160325395526, -232.2234910544682123 ) ) ;
#404=CARTESIAN_POINT ( 'NONE',  ( 15.51129552754472307, 0.2180314803830030457, -231.3815478022924879 ) ) ;
#406=CARTESIAN_POINT ( 'NONE',  ( 4.301648988406530094, 13.23079486486395240, -223.2766268961034655 ) ) ;
#407=CARTESIAN_POINT ( 'NONE',  ( 19.48258831087540344, -3.612136468958778934, -219.4255404790470436 ) ) ;
#409=CARTESIAN_POINT ( 'NONE',  ( 15.52719855059926424, 1.633696074270991172, -221.7349885876216433 ) ) ;
#410=CARTESIAN_POINT ( 'NONE',  ( 5.569356713096689226, -12.06902110579006226, -223.1407905962607003 ) ) ;
#412=CARTESIAN_POINT ( 'NONE',  ( -13.58874046263339608, 12.73011668665171392, -216.5659449791897941 ) ) ;
#413=CARTESIAN_POINT ( 'NONE',  ( -8.329232059016652201, 11.81357365351366617, -230.1839637212758021 ) ) ;
#415=CARTESIAN_POINT ( 'NONE',  ( -17.88126539071149779, 5.766250685202066961, -232.9050303536861293 ) ) ;
#416=CARTESIAN_POINT ( 'NONE',  ( -10.46545893407769157, -9.768586176915025732, -226.8636372813723199 ) ) ;
#419=CARTESIAN_POINT ( 'NONE',  ( -29.95012366401462955, 4.746560250930182967, -224.6954343660969471 ) ) ;
#420=CARTESIAN_POINT ( 'NONE',  ( 5.240643865192946116, -17.54789557311951143, -217.3772572127879812 ) ) ;
#423=CARTESIAN_POINT ( 'NONE',  ( 12.56556766396551872, 9.776144415819011613, -223.4791766911294815 ) ) ;
#424=CARTESIAN_POINT ( 'NONE',  ( -14.00980274651940682, 20.05588230486321066, -234.2453272803952586 ) ) ;
#426=CARTESIAN_POINT ( 'NONE',  ( 14.72046356508972309, 21.23077830076469041, -229.4562045376679578 ) ) ;
#427=CARTESIAN_POINT ( 'NONE',  ( 4.354371064427007276, -19.91633591276652382, -233.4790676556106348 ) ) ;
#429=CARTESIAN_POINT ( 'NONE',  ( -4.170472558179216804, 16.67407401355319152, -230.2690496885289804 ) ) ;
#430=CARTESIAN_POINT ( 'NONE',  ( -12.04619960554013502, 10.22290173510000777, -223.1766370265664534 ) ) ;
#431=CARTESIAN_POINT ( 'NONE',  ( -25.00745438246740804, 14.90779342625281778, -219.2410538611701156 ) ) ;
#433=CARTESIAN_POINT ( 'NONE',  ( -20.58582428111024853, -15.24952116403520463, -229.8418230779359135 ) ) ;
#436=CARTESIAN_POINT ( 'NONE',  ( 14.70646826691583975, 6.155951851203820269, -230.2899142379868920 ) ) ;
#437=CARTESIAN_POINT ( 'NONE',  ( 6.831421020708281944, -16.86748893536391591, -229.5305077739217552 ) ) ;
#438=CARTESIAN_POINT ( 'NONE',  ( 26.29894631880581812, 12.29609390142961090, -226.3100047295820332 ) ) ;
#439=CARTESIAN_POINT ( 'NONE',  ( -24.24202834850560606, 19.05981756344202438, -226.6980666352953335 ) ) ;
#441=CARTESIAN_POINT ( 'NONE',  ( 16.77642802340811556, -0.6192566135115280535, -218.8326447441449432 ) ) ;
#443=CARTESIAN_POINT ( 'NONE',  ( 4.603870848087811218, 30.13529352683433515, -225.9623629403671430 ) ) ;
#445=CARTESIAN_POINT ( 'NONE',  ( -11.07688804854283049, -12.81333559660784971, -232.1241261852632363 ) ) ;
#446=CARTESIAN_POINT ( 'NONE',  ( 20.25084204406298127, -10.11176871144018818, -232.7817218064674591 ) ) ;
#449=CARTESIAN_POINT ( 'NONE',  ( -18.67456582549428390, 11.07053394491094345, -214.7114755712704550 ) ) ;
#450=CARTESIAN_POINT ( 'NONE',  ( -16.09675311661892039, -3.241155435977624677, -226.6155721728984531 ) ) ;
#451=CARTESIAN_POINT ( 'NONE',  ( -17.39737143130126285, 7.531548707695031375, -232.0788227848755696 ) ) ;
#452=CARTESIAN_POINT ( 'NONE',  ( 3.219568897812384645, 28.82511222849302257, -221.5626884747494216 ) ) ;
#453=CARTESIAN_POINT ( 'NONE',  ( -2.125813515909480866, 15.68152656492264363, -220.3943115937447317 ) ) ;
#455=CARTESIAN_POINT ( 'NONE',  ( 20.57969228301723419, -8.207465571703625784, -214.6085555290863454 ) ) ;
#457=CARTESIAN_POINT ( 'NONE',  ( 28.02123297569005089, 5.903198806000402143, -227.5759114383273811 ) ) ;
#459=CARTESIAN_POINT ( 'NONE',  ( -12.39195900010699702, 23.13258866008456138, -233.4668451572263166 ) ) ;
#460=CARTESIAN_POINT ( 'NONE',  ( -15.10760069511485604, 3.026516874529453283, -224.5685390982118861 ) ) ;
#461=CARTESIAN_POINT ( 'NONE',  ( -15.34124043857492303, -4.213426711746545372, -218.8308339851419078 ) ) ;
#462=CARTESIAN_POINT ( 'NONE',  ( -19.25929423112888017, 9.818144317380269825, -216.1837936240308409 ) ) ;
#465=CARTESIAN_POINT ( 'NONE',  ( 23.21336156720804667, 12.57464006230432574, -232.9346648124233070 ) ) ;
#466=CARTESIAN_POINT ( 'NONE',  ( -13.01542355754912172, 26.77630951171455820, -225.1545229496516356 ) ) ;
#467=CARTESIAN_POINT ( 'NONE',  ( 11.17228388010293649, 5.622653638471959425, -222.3672781564363845 ) ) ;
#468=CARTESIAN_POINT ( 'NONE',  ( -21.89065952084848021, -0.9940043559354364566, -216.9999999999999716 ) ) ;
#470=CARTESIAN_POINT ( 'NONE',  ( -19.24125987773642166, -8.201885216777814236, -235.2928755229699789 ) ) ;
#472=CARTESIAN_POINT ( 'NONE',  ( -19.29805292978571885, -8.785194383212417080, -233.3520286081516133 ) ) ;
#474=CARTESIAN_POINT ( 'NONE',  ( -1.973648319964989462, 15.33498294326524203, -220.9958390492969329 ) ) ;
#475=CARTESIAN_POINT ( 'NONE',  ( -7.460068573003235670, -29.58770008691625364, -228.1902472473001637 ) ) ;
#476=CARTESIAN_POINT ( 'NONE',  ( 4.484811161826725900, 15.38298568785217313, -219.4617573400562662 ) ) ;
#477=CARTESIAN_POINT ( 'NONE',  ( 3.668385877085885927, -11.51845067838601366, -222.7629028536941291 ) ) ;
#479=CARTESIAN_POINT ( 'NONE',  ( 29.47107563651793427, 6.731311671946880182, -220.0565342412898815 ) ) ;
#480=CARTESIAN_POINT ( 'NONE',  ( 30.39189047201120175, -1.943849802383817993, -228.0804048816970919 ) ) ;
#481=CARTESIAN_POINT ( 'NONE',  ( -4.285397168228398890, 18.56782363833054106, -219.4990091916804715 ) ) ;
#482=CARTESIAN_POINT ( 'NONE',  ( 17.34461553379066601, 6.893916422670210764, -233.3442385185644525 ) ) ;
#483=CARTESIAN_POINT ( 'NONE',  ( 24.42567939027770407, 10.22651298688739097, -219.4562066833365748 ) ) ;
#484=CARTESIAN_POINT ( 'NONE',  ( -13.44952714103469305, -17.53057434768947331, -217.9956016333683237 ) ) ;
#486=CARTESIAN_POINT ( 'NONE',  ( 1.220475224794998370, 29.83033731899746144, -230.4224274340063801 ) ) ;
#490=CARTESIAN_POINT ( 'NONE',  ( -3.608027314846280031, -12.96557536209330763, -219.9492366723279702 ) ) ;
#491=CARTESIAN_POINT ( 'NONE',  ( -7.240690404266621805, 13.01623002570985044, -225.3000933658701967 ) ) ;
#492=CARTESIAN_POINT ( 'NONE',  ( 23.22505041959077232, 19.39625294115234055, -221.5972645870541555 ) ) ;
#493=CARTESIAN_POINT ( 'NONE',  ( -11.82020046940938407, 10.16362659047642758, -224.3364193436540575 ) ) ;
#494=CARTESIAN_POINT ( 'NONE',  ( -3.309130212696198559, 28.80211350556483296, -217.4284252357080334 ) ) ;
#495=CARTESIAN_POINT ( 'NONE',  ( 14.70646826691583975, 6.155951851203820269, -230.2899142379868920 ) ) ;
#496=CARTESIAN_POINT ( 'NONE',  ( 11.33829581046623858, -17.80819325066959635, -230.7883484307220385 ) ) ;
#498=CARTESIAN_POINT ( 'NONE',  ( 11.72194121175188997, -15.95900783718691507, -217.6519982781775013 ) ) ;
#499=CARTESIAN_POINT ( 'NONE',  ( -6.901278853520646628, 15.41233971300566807, -220.5972764307651346 ) ) ;
#501=CARTESIAN_POINT ( 'NONE',  ( 17.60676319847677007, 21.31475060840986302, -219.8266339603936785 ) ) ;
#502=CARTESIAN_POINT ( 'NONE',  ( 24.56541673123750158, -5.996287403333383281, -231.6940117905984664 ) ) ;
#503=CARTESIAN_POINT ( 'NONE',  ( -15.22366728182010043, -5.552021002219007961, -230.2511309519622671 ) ) ;
#504=CARTESIAN_POINT ( 'NONE',  ( -7.800954605602409053, -29.95157606033723496, -226.5906573908930000 ) ) ;
#505=CARTESIAN_POINT ( 'NONE',  ( -5.125319492185865577, 20.53749879880200524, -218.7557759432853288 ) ) ;
#507=CARTESIAN_POINT ( 'NONE',  ( 20.22510869507564024, 17.05975164568011238, -220.7829296213589316 ) ) ;
#508=CARTESIAN_POINT ( 'NONE',  ( -17.75316132689678383, 25.03468689048078843, -222.1645193425721061 ) ) ;
#509=CARTESIAN_POINT ( 'NONE',  ( -9.115411286166651195, 13.66191091052436235, -230.3338332872444312 ) ) ;
#511=CARTESIAN_POINT ( 'NONE',  ( 6.040050017043670394, 13.67534390435379699, -220.4759402345340504 ) ) ;
#512=CARTESIAN_POINT ( 'NONE',  ( -23.67953786836281083, 9.946055673977088674, -229.5560005648173671 ) ) ;
#513=CARTESIAN_POINT ( 'NONE',  ( 20.64287812348744566, 0.2024751443801864337, -216.7518974727033481 ) ) ;
#514=CARTESIAN_POINT ( 'NONE',  ( 15.69671663880151868, -19.77919342852767315, -217.9503656454650411 ) ) ;
#517=CARTESIAN_POINT ( 'NONE',  ( 5.331555957413248059, 27.50712867803999728, -219.0801070358024276 ) ) ;
#518=CARTESIAN_POINT ( 'NONE',  ( 24.34559900986324621, -8.951716371391148286, -220.6604487471163623 ) ) ;
#519=CARTESIAN_POINT ( 'NONE',  ( 25.54997870115619207, -2.097555195297153841, -218.7002440566220400 ) ) ;
#520=CARTESIAN_POINT ( 'NONE',  ( 4.201723131641114328, -20.76291977712905279, -215.9522215885928347 ) ) ;
#521=CARTESIAN_POINT ( 'NONE',  ( -22.17339560624464312, 16.26550580028390769, -232.0582861498566274 ) ) ;
#523=CARTESIAN_POINT ( 'NONE',  ( -11.40916210110096962, 20.01996232974788725, -234.3205435716851923 ) ) ;
#524=CARTESIAN_POINT ( 'NONE',  ( -9.443239614166923701, 9.388015667058336788, -222.3195230688234290 ) ) ;
#525=CARTESIAN_POINT ( 'NONE',  ( -24.95227886253013239, -16.82584358170602101, -223.8363818545792299 ) ) ;
#528=CARTESIAN_POINT ( 'NONE',  ( -15.48255455842386219, 10.01793346089237069, -233.1197357361336913 ) ) ;
#529=CARTESIAN_POINT ( 'NONE',  ( -0.3008257096753846893, -14.77709807386645480, -230.6673697011181048 ) ) ;
#531=CARTESIAN_POINT ( 'NONE',  ( 17.24423567610276109, 8.542587572837451404, -218.6562240232607621 ) ) ;
#532=CARTESIAN_POINT ( 'NONE',  ( -8.894613172508529786, 25.42460746921206294, -232.3150764041658363 ) ) ;
#533=CARTESIAN_POINT ( 'NONE',  ( 13.70753084697862612, 0.1061737631881888994, -227.9987150399367408 ) ) ;
#534=CARTESIAN_POINT ( 'NONE',  ( 10.64724148863252395, 12.28344647332184181, -223.6549461381946173 ) ) ;
#535=CARTESIAN_POINT ( 'NONE',  ( 2.980115756258533644, -14.12936798750240008, -229.0659090661425807 ) ) ;
#537=CARTESIAN_POINT ( 'NONE',  ( -8.857704405076667342, 24.20848540845601704, -218.8859504303524091 ) ) ;
#538=CARTESIAN_POINT ( 'NONE',  ( -13.06839468023815165, 25.32320678245788059, -229.0099538679170053 ) ) ;
#539=CARTESIAN_POINT ( 'NONE',  ( -27.12694304224540076, 7.756125161462346540, -217.3817363082233101 ) ) ;
#541=CARTESIAN_POINT ( 'NONE',  ( -14.65844530258765310, -17.20867344037294444, -230.8340913472024170 ) ) ;
#545=CARTESIAN_POINT ( 'NONE',  ( -25.29098058636142810, 5.014641116111857144, -217.4658967307323110 ) ) ;
#546=CARTESIAN_POINT ( 'NONE',  ( 8.290903921942224031, -23.90349455650518351, -230.1727405421096364 ) ) ;
#547=CARTESIAN_POINT ( 'NONE',  ( 10.78187269046063435, 10.73871010366167944, -221.9206544238666368 ) ) ;
#548=CARTESIAN_POINT ( 'NONE',  ( -8.501641725227710111, 25.47064987787527102, -217.3358698761548737 ) ) ;
#549=CARTESIAN_POINT ( 'NONE',  ( -15.60078324628501356, 3.527872497691606934, -227.4630248446626695 ) ) ;
#551=CARTESIAN_POINT ( 'NONE',  ( 4.484811161826725900, 15.38298568785217313, -219.4617573400562662 ) ) ;
#554=CARTESIAN_POINT ( 'NONE',  ( -15.62091161899253855, -26.00636881980398840, -222.1463585103649905 ) ) ;
#556=CARTESIAN_POINT ( 'NONE',  ( 17.28140336138120858, -11.48510652344925020, -216.9852223368602893 ) ) ;
#559=CARTESIAN_POINT ( 'NONE',  ( -14.08083899843152231, 10.81596681319144970, -234.3239311387574446 ) ) ;
#560=CARTESIAN_POINT ( 'NONE',  ( -27.33303184979533285, -3.055344081261842870, -227.4850045670461043 ) ) ;
#561=CARTESIAN_POINT ( 'NONE',  ( -13.31590776630363315, 5.340120742929252096, -225.6956515496373186 ) ) ;
#562=CARTESIAN_POINT ( 'NONE',  ( 8.379126514044342500, 15.76264856365358646, -232.1787896114811360 ) ) ;
#563=CARTESIAN_POINT ( 'NONE',  ( -1.238249567024760189, 29.30580384236933966, -223.2399636023643836 ) ) ;
#565=CARTESIAN_POINT ( 'NONE',  ( 19.43707201973751708, -21.22621598813149646, -232.3303264720597667 ) ) ;
#567=CARTESIAN_POINT ( 'NONE',  ( 18.46552355142154411, 5.019711608606525211, -231.5099115070375433 ) ) ;
#568=CARTESIAN_POINT ( 'NONE',  ( -4.531689447889125866, 14.11317536318881416, -231.6806015375303502 ) ) ;
#569=CARTESIAN_POINT ( 'NONE',  ( -6.111257124579617894, 15.89946952501658295, -216.3497764690875727 ) ) ;
#570=CARTESIAN_POINT ( 'NONE',  ( -14.31049420963804586, -8.435107166214018903, -218.7432863707801403 ) ) ;
#571=CARTESIAN_POINT ( 'NONE',  ( -9.171998067665157350, 9.395241133357435714, -226.3428046914542051 ) ) ;
#575=CARTESIAN_POINT ( 'NONE',  ( -12.96364545172611571, 10.77137376900670063, -221.1208843751685720 ) ) ;
#576=CARTESIAN_POINT ( 'NONE',  ( -19.50431861204945605, -0.7624880359591150736, -219.4666829195064395 ) ) ;
#577=CARTESIAN_POINT ( 'NONE',  ( -14.87984907657228639, 0.2138881189739126887, -228.7773920408832282 ) ) ;
#578=CARTESIAN_POINT ( 'NONE',  ( 7.995304978256253747, 13.28024228361502779, -220.6535174700288451 ) ) ;
#579=CARTESIAN_POINT ( 'NONE',  ( -24.09642229725868745, -17.04339013636034750, -228.1169379854252384 ) ) ;
#581=CARTESIAN_POINT ( 'NONE',  ( -6.072587425033909803, 24.65158735603439055, -217.4249768037189767 ) ) ;
#582=CARTESIAN_POINT ( 'NONE',  ( -5.636842872076440081, -13.76003991320737541, -219.7405193562604495 ) ) ;
#583=CARTESIAN_POINT ( 'NONE',  ( 16.54345861550681107, 19.37554510112122230, -218.2240151908141002 ) ) ;
#584=CARTESIAN_POINT ( 'NONE',  ( 6.919598145955467849, -31.16410449029495311, -226.5345828574877487 ) ) ;
#587=CARTESIAN_POINT ( 'NONE',  ( -9.954421844142357756, 11.21484508112568079, -226.0177122452137439 ) ) ;
#589=CARTESIAN_POINT ( 'NONE',  ( 21.96352831578812115, -0.3315607655626495731, -233.9427286327413356 ) ) ;
#590=CARTESIAN_POINT ( 'NONE',  ( 13.50603691942335693, 22.79443449215731832, -229.7689193854997995 ) ) ;
#591=CARTESIAN_POINT ( 'NONE',  ( -12.33203608746942237, 8.428128317385924717, -222.9277009507565026 ) ) ;
#592=CARTESIAN_POINT ( 'NONE',  ( 21.31262902390056624, 0.4111834581965390645, -232.0572713672585792 ) ) ;
#593=CARTESIAN_POINT ( 'NONE',  ( -9.981957700435337699, -28.23530775694580441, -222.3321348641582347 ) ) ;
#594=CARTESIAN_POINT ( 'NONE',  ( 13.70863938672594529, 6.616599615120571265, -232.1343637516268643 ) ) ;
#596=CARTESIAN_POINT ( 'NONE',  ( 0.4504461526642338232, -19.62726417856956473, -215.9916429883993487 ) ) ;
#597=CARTESIAN_POINT ( 'NONE',  ( 2.893760225568064115, 14.39521026618305477, -227.6654023557511550 ) ) ;
#599=CARTESIAN_POINT ( 'NONE',  ( 14.69853173970351179, 23.44775873627089524, -231.2711109634281001 ) ) ;
#600=CARTESIAN_POINT ( 'NONE',  ( -8.892156391762910062, 11.89593067802204551, -225.4519868197583889 ) ) ;
#601=CARTESIAN_POINT ( 'NONE',  ( -4.154119475380428916, 11.54776298361823095, -227.0876712548254943 ) ) ;
#602=CARTESIAN_POINT ( 'NONE',  ( 15.28706223449149348, 2.473424253736659306, -227.9634568993954531 ) ) ;
#603=CARTESIAN_POINT ( 'NONE',  ( 9.097575839043912538, -18.13002900832716335, -219.2719510042808224 ) ) ;
#605=CARTESIAN_POINT ( 'NONE',  ( 13.17817051516727922, -26.22376201054615308, -223.3126545406654486 ) ) ;
#606=CARTESIAN_POINT ( 'NONE',  ( -6.769588938507062004, 18.22485903270490937, -231.3660928915624879 ) ) ;
#608=CARTESIAN_POINT ( 'NONE',  ( 27.04607490430786854, 4.607450003618843049, -220.3758934308003461 ) ) ;
#609=CARTESIAN_POINT ( 'NONE',  ( 28.52058947142581502, -1.755848367977142610, -221.9695116608532715 ) ) ;
#610=CARTESIAN_POINT ( 'NONE',  ( -20.11874861854083463, -21.11755179634840474, -229.7504124090357323 ) ) ;
#611=CARTESIAN_POINT ( 'NONE',  ( 1.623338700557370951, -21.82196275546919040, -234.1129525514646730 ) ) ;
#612=CARTESIAN_POINT ( 'NONE',  ( 8.829458998963966465, 22.90677303676718779, -219.2026791561175685 ) ) ;
#614=CARTESIAN_POINT ( 'NONE',  ( -28.99982533490676317, 5.894721259135065949, -231.5937499788843468 ) ) ;
#615=CARTESIAN_POINT ( 'NONE',  ( -3.643097910890548796, 22.16888955197135047, -233.9701981029593298 ) ) ;
#616=CARTESIAN_POINT ( 'NONE',  ( 4.044213993247089967, 16.45246633354041421, -227.9255899743332918 ) ) ;
#617=CARTESIAN_POINT ( 'NONE',  ( -2.692720963948733282, 24.67937284847025481, -218.0912907784291406 ) ) ;
#618=CARTESIAN_POINT ( 'NONE',  ( -12.04619960554013502, 10.22290173510000777, -223.1766370265664534 ) ) ;
#619=CARTESIAN_POINT ( 'NONE',  ( 14.17826651990317188, -1.167225063855702683, -222.4240311848849387 ) ) ;
#620=CARTESIAN_POINT ( 'NONE',  ( 7.045253012492558753, -17.38872841331140862, -218.3726031779064556 ) ) ;
#624=CARTESIAN_POINT ( 'NONE',  ( 4.543450689403089271, 15.91052110650461771, -218.9437823786444426 ) ) ;
#625=CARTESIAN_POINT ( 'NONE',  ( -25.88730550323791491, -2.172607277783750845, -234.4881349215252726 ) ) ;
#628=CARTESIAN_POINT ( 'NONE',  ( 8.021672912688133650, -23.92397517040199872, -233.3380040120402441 ) ) ;
#630=CARTESIAN_POINT ( 'NONE',  ( -21.02719846458807851, 18.12262440796364871, -218.0220709499931502 ) ) ;
#631=CARTESIAN_POINT ( 'NONE',  ( -11.59874896804548250, 27.28969409813203484, -218.8626241359735332 ) ) ;
#633=CARTESIAN_POINT ( 'NONE',  ( -14.00380962569832199, 8.747390586476997854, -231.7950903513155936 ) ) ;
#634=CARTESIAN_POINT ( 'NONE',  ( -15.95714424191699266, -19.90201571590360885, -231.7641511196865451 ) ) ;
#637=CARTESIAN_POINT ( 'NONE',  ( -18.09776816382430908, 23.50806826204562583, -229.9568677523880638 ) ) ;
#638=CARTESIAN_POINT ( 'NONE',  ( 9.923594862512629788, -27.47695806889172943, -228.4416101659923015 ) ) ;
#639=CARTESIAN_POINT ( 'NONE',  ( -11.49049084071896409, 11.06834963248926940, -218.3354249205727058 ) ) ;
#640=CARTESIAN_POINT ( 'NONE',  ( 18.30590144060498403, 15.06309558287673767, -219.0459394567220102 ) ) ;
#641=CARTESIAN_POINT ( 'NONE',  ( 5.711092584709906106, 26.13380667269736790, -220.5232813324456629 ) ) ;
#643=CARTESIAN_POINT ( 'NONE',  ( 24.38255093784924199, 7.851200578213498815, -231.2687759850219607 ) ) ;
#644=CARTESIAN_POINT ( 'NONE',  ( -11.82770121052164924, -14.33821066513346487, -229.8071374592849452 ) ) ;
#646=CARTESIAN_POINT ( 'NONE',  ( -3.996294969088721505, 28.80481464818193515, -222.8623509149411746 ) ) ;
#647=CARTESIAN_POINT ( 'NONE',  ( -20.29166677327761903, 16.18344358422343632, -220.0060062064338524 ) ) ;
#648=CARTESIAN_POINT ( 'NONE',  ( -8.548213857283494477, 12.07277636836182211, -222.5354997492170241 ) ) ;
#649=CARTESIAN_POINT ( 'NONE',  ( -17.67448836398429890, -11.08962652971676199, -218.7915233441472367 ) ) ;
#652=CARTESIAN_POINT ( 'NONE',  ( -28.17543631911187063, 3.557555778861649642, -230.1980773687482156 ) ) ;
#653=CARTESIAN_POINT ( 'NONE',  ( 0.1655890855189643129, -14.86936674525315993, -225.9040401458518943 ) ) ;
#654=CARTESIAN_POINT ( 'NONE',  ( 18.76922974182421555, 13.12635134380198210, -217.8010375391909008 ) ) ;
#655=CARTESIAN_POINT ( 'NONE',  ( -2.817219543927646175, 14.13981714106644993, -229.6779615865167443 ) ) ;
#657=CARTESIAN_POINT ( 'NONE',  ( -26.91858181626453472, 10.72837452931393187, -223.4556356000267670 ) ) ;
#658=CARTESIAN_POINT ( 'NONE',  ( 12.65306858828212810, 29.42930486385247590, -226.3758484992818012 ) ) ;
#659=CARTESIAN_POINT ( 'NONE',  ( 16.84848658399567611, 11.39632653812981644, -217.9589513831453473 ) ) ;
#661=CARTESIAN_POINT ( 'NONE',  ( 14.83698775855651952, 1.948536915275967507, -222.7182371053496865 ) ) ;
#662=CARTESIAN_POINT ( 'NONE',  ( -18.64257584594551531, -16.66392856591270899, -217.1407738418131999 ) ) ;
#663=CARTESIAN_POINT ( 'NONE',  ( 2.967317674205219191, -16.40215926535219282, -217.6245344443522924 ) ) ;
#666=CARTESIAN_POINT ( 'NONE',  ( -7.352050649209116884, 10.05454564170545417, -223.7370967983176229 ) ) ;
#667=CARTESIAN_POINT ( 'NONE',  ( -26.02538399328502905, -8.003917019953526335, -222.3553134616452098 ) ) ;
#668=CARTESIAN_POINT ( 'NONE',  ( -14.35594238341465889, 9.236863657925704629, -219.6542735655305307 ) ) ;
#669=CARTESIAN_POINT ( 'NONE',  ( 23.18902850759750933, 20.27908137164207147, -226.2847847834817117 ) ) ;
#670=CARTESIAN_POINT ( 'NONE',  ( 10.73846460100926592, 12.62787417135106161, -222.6344468496098159 ) ) ;
#672=CARTESIAN_POINT ( 'NONE',  ( 18.85502272441424765, -23.46047257272994102, -219.5236553823413317 ) ) ;
#673=CARTESIAN_POINT ( 'NONE',  ( 16.38151749656409351, 8.902090001712490874, -231.2955017965201989 ) ) ;
#674=CARTESIAN_POINT ( 'NONE',  ( -13.41298582792616934, 27.85383138489214616, -228.6457525465575884 ) ) ;
#676=CARTESIAN_POINT ( 'NONE',  ( -4.155456637169709921, 11.30291311430030987, -225.2606024264729001 ) ) ;
#677=CARTESIAN_POINT ( 'NONE',  ( -22.73457989858237127, -6.881456255901889030, -216.4806380023168799 ) ) ;
#678=CARTESIAN_POINT ( 'NONE',  ( -10.30050448363967419, 10.07750059423401190, -220.1837019037183723 ) ) ;
#681=CARTESIAN_POINT ( 'NONE',  ( 24.21331552874348958, 0.07051084380047288602, -231.7986140076958463 ) ) ;
#682=CARTESIAN_POINT ( 'NONE',  ( -6.804439720554941395, 15.25609613835249156, -218.7834354895107651 ) ) ;
#683=CARTESIAN_POINT ( 'NONE',  ( 17.96045420455031305, -0.3746358454349600908, -217.9627609769914613 ) ) ;
#684=CARTESIAN_POINT ( 'NONE',  ( -23.98802705797876200, 19.46654170242919690, -223.5293093576406989 ) ) ;
#685=CARTESIAN_POINT ( 'NONE',  ( 6.093530912645064745, 16.79941505724243811, -232.1766444656230419 ) ) ;
#687=CARTESIAN_POINT ( 'NONE',  ( 0.3355639943343493026, 23.87279439325363128, -218.0067922387550823 ) ) ;
#688=CARTESIAN_POINT ( 'NONE',  ( -25.61235545225478560, -15.41032726095661509, -226.9890212492312855 ) ) ;
#689=CARTESIAN_POINT ( 'NONE',  ( 11.67669251569587985, 24.04736029062789981, -218.5856804285192254 ) ) ;
#690=CARTESIAN_POINT ( 'NONE',  ( 8.343550503364536297, -10.95302570107183726, -218.8523668966870446 ) ) ;
#692=CARTESIAN_POINT ( 'NONE',  ( -20.97727766418175932, 9.381545086430262970, -232.5968905491617420 ) ) ;
#694=CARTESIAN_POINT ( 'NONE',  ( -17.19162585816985001, -4.675655174483583032, -230.6997921109560821 ) ) ;
#695=CARTESIAN_POINT ( 'NONE',  ( 14.02816775221371337, 20.58276248714641810, -218.7180790146936999 ) ) ;
#696=CARTESIAN_POINT ( 'NONE',  ( -22.38347148959098121, 12.58966534755613687, -218.4978713241202399 ) ) ;
#697=CARTESIAN_POINT ( 'NONE',  ( 15.01439307471096463, 1.118969480519667048, -226.7488225241675366 ) ) ;
#698=CARTESIAN_POINT ( 'NONE',  ( -7.534279315020126155, -14.09704863723370494, -220.2840498463326355 ) ) ;
#699=CARTESIAN_POINT ( 'NONE',  ( 25.17176037151762813, 18.95054595444721102, -221.3490360113488862 ) ) ;
#701=CARTESIAN_POINT ( 'NONE',  ( -27.72233273893307981, -16.15685914833838410, -223.8945077613443289 ) ) ;
#702=CARTESIAN_POINT ( 'NONE',  ( 3.160467108836292116, 14.95099014189016629, -228.9242958482614370 ) ) ;
#703=CARTESIAN_POINT ( 'NONE',  ( 29.89309326230132058, 6.052383583152112223, -228.3539431708548477 ) ) ;
#705=CARTESIAN_POINT ( 'NONE',  ( -12.01777041390050726, 10.97692933293401474, -227.6853890888168053 ) ) ;
#706=CARTESIAN_POINT ( 'NONE',  ( -9.747505956077446854, 15.39125695327449783, -233.2799778227147840 ) ) ;
#707=CARTESIAN_POINT ( 'NONE',  ( 21.19180206786061405, -1.472355559550188264, -231.3901500139509722 ) ) ;
#708=CARTESIAN_POINT ( 'NONE',  ( -5.472810246302690196, -26.30400724048815420, -218.4657170016378416 ) ) ;
#710=CARTESIAN_POINT ( 'NONE',  ( 5.625090746907006611, -14.93184515622287201, -221.0486942310484721 ) ) ;
#712=CARTESIAN_POINT ( 'NONE',  ( 22.18132842682159733, 5.591149267797686839, -232.0584733989884114 ) ) ;
#713=CARTESIAN_POINT ( 'NONE',  ( 26.16486877413895584, -0.2437668799822691745, -230.8325409000573814 ) ) ;
#714=CARTESIAN_POINT ( 'NONE',  ( -19.88402822078561627, -6.951120502836210413, -232.7962440186676361 ) ) ;
#715=CARTESIAN_POINT ( 'NONE',  ( 5.668262076144046979, -25.28042871382391965, -216.8182873783340483 ) ) ;
#716=CARTESIAN_POINT ( 'NONE',  ( 6.173705828530630768, 14.85108299334794957, -222.6284669816953112 ) ) ;
#718=CARTESIAN_POINT ( 'NONE',  ( -12.45629340980802269, 5.675423426979704367, -220.8874502847910719 ) ) ;
#719=CARTESIAN_POINT ( 'NONE',  ( -10.84997096467605182, 25.01800101807719301, -232.4518260228253155 ) ) ;
#720=CARTESIAN_POINT ( 'NONE',  ( -2.532949683519015949, 17.18298404079579100, -229.0924323441805086 ) ) ;
#721=CARTESIAN_POINT ( 'NONE',  ( 11.97659261343968851, -3.740017786417877854, -223.6042415182018033 ) ) ;
#723=CARTESIAN_POINT ( 'NONE',  ( 14.63115627273841923, 9.024791562541032874, -232.5054678133655841 ) ) ;
#724=CARTESIAN_POINT ( 'NONE',  ( -17.07311071032027172, 18.59516984069744794, -230.9440421721702137 ) ) ;
#725=CARTESIAN_POINT ( 'NONE',  ( 18.50073117969547098, -1.889592114545683987, -232.6396648696776026 ) ) ;
#726=CARTESIAN_POINT ( 'NONE',  ( -5.056986327342952947, -15.36481113542577503, -220.7955371552936583 ) ) ;
#729=CARTESIAN_POINT ( 'NONE',  ( 17.68508104102419409, 23.41266195669770767, -227.5327139115408954 ) ) ;
#730=CARTESIAN_POINT ( 'NONE',  ( 14.87638776485545122, -7.040696290218329878, -226.6726542491997805 ) ) ;
#732=CARTESIAN_POINT ( 'NONE',  ( -1.643553855084622928, -13.05119293000219294, -222.7191902239112551 ) ) ;
#734=CARTESIAN_POINT ( 'NONE',  ( 5.169766346882679997, 29.28517558595074988, -221.5178724947562614 ) ) ;
#735=CARTESIAN_POINT ( 'NONE',  ( -10.95054816480499760, 8.339404316518379545, -224.1596700080921778 ) ) ;
#737=CARTESIAN_POINT ( 'NONE',  ( -12.31207293045244988, 6.732038552366256923, -221.0952066824360713 ) ) ;
#738=CARTESIAN_POINT ( 'NONE',  ( -17.01799258133205228, -17.74971190556693657, -217.5843211863294755 ) ) ;
#741=CARTESIAN_POINT ( 'NONE',  ( -3.060450601941519189, 13.29454208326677289, -222.0135664617158682 ) ) ;
#742=CARTESIAN_POINT ( 'NONE',  ( 0.8130732720878883768, -26.02312037787507393, -216.7203152272084878 ) ) ;
#743=CARTESIAN_POINT ( 'NONE',  ( 14.67391514392257612, -1.621881806925726588, -222.4758702327235653 ) ) ;
#744=CARTESIAN_POINT ( 'NONE',  ( -9.443239614166923701, 9.388015667058336788, -222.3195230688234290 ) ) ;
#745=CARTESIAN_POINT ( 'NONE',  ( -13.33011381921379090, 5.829915729572584304, -219.4453182727427816 ) ) ;
#747=CARTESIAN_POINT ( 'NONE',  ( -2.125813515909480866, 15.68152656492264363, -220.3943115937447317 ) ) ;
#749=CARTESIAN_POINT ( 'NONE',  ( 13.80707869872719762, 6.429545566348308760, -225.7152177910682553 ) ) ;
#750=CARTESIAN_POINT ( 'NONE',  ( -9.995627826723184839, -14.18420632236771439, -221.4333122433492633 ) ) ;
#752=CARTESIAN_POINT ( 'NONE',  ( 11.01659168199870287, 19.17922986229587323, -233.3715978632214387 ) ) ;
#753=CARTESIAN_POINT ( 'NONE',  ( -11.82020046940938407, 10.16362659047642758, -224.3364193436540575 ) ) ;
#754=CARTESIAN_POINT ( 'NONE',  ( -11.11821474075380678, 16.53100589793018926, -232.3736596382188395 ) ) ;
#755=CARTESIAN_POINT ( 'NONE',  ( -27.94976817795961210, -4.610981384744690104, -229.1808304932418139 ) ) ;
#759=CARTESIAN_POINT ( 'NONE',  ( -20.54164754914381064, 7.122791156791981493, -233.5720402887671980 ) ) ;
#760=CARTESIAN_POINT ( 'NONE',  ( 4.144298419883110540, -16.00443160190133085, -221.4341300285535965 ) ) ;
#762=CARTESIAN_POINT ( 'NONE',  ( 1.382955251742491898, 16.46353944795171032, -231.7743150979565030 ) ) ;
#764=CARTESIAN_POINT ( 'NONE',  ( 20.92846067405557520, -2.114533307883533109, -233.2756072794335580 ) ) ;
#765=CARTESIAN_POINT ( 'NONE',  ( 15.33651282626308010, 7.807290788239344970, -218.6940806506825652 ) ) ;
#766=CARTESIAN_POINT ( 'NONE',  ( 22.84140515590350518, 18.29101041979067332, -226.2334522600520472 ) ) ;
#768=CARTESIAN_POINT ( 'NONE',  ( -9.606889355748592152, -11.26588727105406385, -229.9123324032181586 ) ) ;
#769=CARTESIAN_POINT ( 'NONE',  ( 1.780803752597676537, -13.83832444325970101, -229.2250779460899537 ) ) ;
#771=CARTESIAN_POINT ( 'NONE',  ( -3.130305314451475418, 18.08417128930788209, -217.9058652980469333 ) ) ;
#772=CARTESIAN_POINT ( 'NONE',  ( 30.30544834784952002, -1.486206387887903047, -219.3838232483325896 ) ) ;
#773=CARTESIAN_POINT ( 'NONE',  ( 22.14341918773124362, -7.622004812940091689, -217.4502831791021720 ) ) ;
#774=CARTESIAN_POINT ( 'NONE',  ( -14.94640692938030746, 5.382918922058764544, -220.5478552936960455 ) ) ;
#775=CARTESIAN_POINT ( 'NONE',  ( 11.63337745479824292, 8.229076005436313679, -220.5472098800687206 ) ) ;
#776=CARTESIAN_POINT ( 'NONE',  ( 18.90025403853754327, 17.70150481658638952, -229.5234643039372315 ) ) ;
#778=CARTESIAN_POINT ( 'NONE',  ( 15.43677305580571435, -6.701975615562529853, -215.9934368197604897 ) ) ;
#781=CARTESIAN_POINT ( 'NONE',  ( 4.952019330116582907, 28.88045068338265509, -217.6369327391592208 ) ) ;
#782=CARTESIAN_POINT ( 'NONE',  ( -5.467362224022371819, 23.92882567691090046, -234.7811165710531611 ) ) ;
#783=CARTESIAN_POINT ( 'NONE',  ( -17.83852468596024110, -8.357198216422425219, -233.0481596892792879 ) ) ;
#784=CARTESIAN_POINT ( 'NONE',  ( -9.749377714296398878, 10.28442384816749922, -229.3722863967025205 ) ) ;
#789=CARTESIAN_POINT ( 'NONE',  ( -8.900302563431933933, 20.17395648083808268, -216.9116515890487733 ) ) ;
#790=CARTESIAN_POINT ( 'NONE',  ( 25.09997929702755926, 1.294103573351435221, -217.0485712200477906 ) ) ;
#791=CARTESIAN_POINT ( 'NONE',  ( -26.74045434827795020, 12.41518252455047744, -220.4617428697642652 ) ) ;
#792=CARTESIAN_POINT ( 'NONE',  ( 15.87442104186276381, 8.674488492264579520, -230.9702037640878416 ) ) ;
#793=CARTESIAN_POINT ( 'NONE',  ( 15.37450427861381286, -5.898921106289613847E-14, -228.0000000000000853 ) ) ;
#795=CARTESIAN_POINT ( 'NONE',  ( 3.522445101072706475, 23.08420003150784439, -231.7850044194335055 ) ) ;
#796=CARTESIAN_POINT ( 'NONE',  ( -21.52428768452188734, -21.65989873160339840, -225.4304055049964006 ) ) ;
#797=CARTESIAN_POINT ( 'NONE',  ( 13.49011766416699842, 7.659170998773840111, -228.1905628957712793 ) ) ;
#798=CARTESIAN_POINT ( 'NONE',  ( -7.215839073791710412, -12.32959168003491968, -224.1142876912989834 ) ) ;
#801=CARTESIAN_POINT ( 'NONE',  ( -12.62195384480319582, 9.244619650382723819, -228.6283004876635516 ) ) ;
#803=CARTESIAN_POINT ( 'NONE',  ( -29.01652113304903935, -3.607535226192160049, -222.1063433863846228 ) ) ;
#804=CARTESIAN_POINT ( 'NONE',  ( 3.241594727517011609, 27.64703009302456138, -225.5540025036233374 ) ) ;
#805=CARTESIAN_POINT ( 'NONE',  ( -10.29720673141181209, 11.14783905173092649, -222.8560683878917530 ) ) ;
#806=CARTESIAN_POINT ( 'NONE',  ( -26.98548179121306845, 3.096138561569834913, -233.8324893795610251 ) ) ;
#807=CARTESIAN_POINT ( 'NONE',  ( -9.206457440458645891, -21.52042488620018545, -217.0715276568171248 ) ) ;
#808=CARTESIAN_POINT ( 'NONE',  ( 16.67941620816951698, 4.093285459228785506, -217.1675623234529269 ) ) ;
#810=CARTESIAN_POINT ( 'NONE',  ( -10.76360437932642533, -14.08317586560949408, -234.4387784497120890 ) ) ;
#811=CARTESIAN_POINT ( 'NONE',  ( -0.7041916573665241152, 14.60214745152014437, -226.3818583194645555 ) ) ;
#813=CARTESIAN_POINT ( 'NONE',  ( 17.91327661571172314, 1.545939370248587075, -216.9938266089438912 ) ) ;
#815=CARTESIAN_POINT ( 'NONE',  ( -6.094651895680649467, 13.59752566126439177, -221.0608041154719103 ) ) ;
#816=CARTESIAN_POINT ( 'NONE',  ( 9.253342549662157523, 15.33540844142859605, -216.2601104504267937 ) ) ;
#817=ORIENTED_EDGE ( 'NONE', *, *, #5810, .F. ) ;
#818=CARTESIAN_POINT ( 'NONE',  ( 2.435323595375026073, -28.08909517487921192, -228.1503986837488469 ) ) ;
#819=CARTESIAN_POINT ( 'NONE',  ( -4.253447013113726527, -22.64852647464574531, -232.0531923962242615 ) ) ;
#820=CARTESIAN_POINT ( 'NONE',  ( 28.51464931495100785, 5.422321182929326966, -223.8116416110474347 ) ) ;
#821=CARTESIAN_POINT ( 'NONE',  ( 17.02763684969102798, -14.67205317233652195, -233.2001291093645818 ) ) ;
#822=CARTESIAN_POINT ( 'NONE',  ( 29.52516483900593158, -0.1522717672070824924, -221.3034020690409704 ) ) ;
#823=CARTESIAN_POINT ( 'NONE',  ( -14.13781561609191328, -15.90667165809925621, -233.6615929499251649 ) ) ;
#824=CARTESIAN_POINT ( 'NONE',  ( 9.253909228257674258, 17.69332415812615977, -230.9900471521432621 ) ) ;
#826=CARTESIAN_POINT ( 'NONE',  ( -20.76981451797363576, 10.27702766794165257, -234.3988437453480742 ) ) ;
#827=CARTESIAN_POINT ( 'NONE',  ( 0.2389779871941385414, 16.64595486589868045, -218.1658233406367629 ) ) ;
#828=CARTESIAN_POINT ( 'NONE',  ( -3.071946796551161984, 23.17078151772539485, -231.0066194318698933 ) ) ;
#829=CARTESIAN_POINT ( 'NONE',  ( 26.86542643433637423, 1.561297562127881511, -231.3515426572852505 ) ) ;
#832=CARTESIAN_POINT ( 'NONE',  ( 6.491278574642851851, 13.23281603069746382, -229.0355254242266767 ) ) ;
#833=CARTESIAN_POINT ( 'NONE',  ( -16.48883219358909713, 20.84100960965193394, -219.4392138569792507 ) ) ;
#834=CARTESIAN_POINT ( 'NONE',  ( 15.06072304412464291, 3.291435955319735651, -218.8606307204261725 ) ) ;
#835=CARTESIAN_POINT ( 'NONE',  ( -6.507186921339367380, -21.94905981650347826, -217.8194053188079238 ) ) ;
#838=CARTESIAN_POINT ( 'NONE',  ( 5.343558017910363667, 26.29639771561252459, -218.1010331760174665 ) ) ;
#839=CARTESIAN_POINT ( 'NONE',  ( 16.20395612672116314, -10.90071921976151081, -219.5016540749954856 ) ) ;
#841=CARTESIAN_POINT ( 'NONE',  ( -3.300598509645395584, -18.18730530649546395, -233.4303386612170925 ) ) ;
#843=CARTESIAN_POINT ( 'NONE',  ( -2.698926868850080041, 12.89339462271858316, -226.7595176699009585 ) ) ;
#845=CARTESIAN_POINT ( 'NONE',  ( -4.154119475380428916, 11.54776298361823095, -227.0876712548254943 ) ) ;
#847=CARTESIAN_POINT ( 'NONE',  ( -12.90983082593748676, 14.84936372681532823, -233.8009687022269532 ) ) ;
#848=CARTESIAN_POINT ( 'NONE',  ( -23.63383474287343589, -9.908731599815467916, -232.6396219513094081 ) ) ;
#851=CARTESIAN_POINT ( 'NONE',  ( 14.96415947227435339, -1.927366939720012606, -222.7010313878448358 ) ) ;
#852=CARTESIAN_POINT ( 'NONE',  ( -18.70100282803782576, 16.58357028540773115, -216.4425743468854080 ) ) ;
#853=CARTESIAN_POINT ( 'NONE',  ( -3.877698871368953082, -12.59008950621349676, -229.3284496285515388 ) ) ;
#854=CARTESIAN_POINT ( 'NONE',  ( 28.22932473237819551, -8.039268142081398949, -226.6539694142420558 ) ) ;
#855=CARTESIAN_POINT ( 'NONE',  ( -18.39892766464214446, 25.11039525536027739, -225.3444503920457294 ) ) ;
#856=CARTESIAN_POINT ( 'NONE',  ( -28.99982533490676317, 5.894721259135065949, -231.5937499788843468 ) ) ;
#857=CARTESIAN_POINT ( 'NONE',  ( -0.7292515499105728383, 28.18841485102515776, -220.8637599502617093 ) ) ;
#859=CARTESIAN_POINT ( 'NONE',  ( 26.92457506054779515, 6.538608665672222209, -219.8654465082432807 ) ) ;
#860=CARTESIAN_POINT ( 'NONE',  ( -8.182256202386261279, -21.48229377488409497, -218.8195705044138606 ) ) ;
#863=CARTESIAN_POINT ( 'NONE',  ( 3.312424284731937618, 15.29837714273186045, -229.5209971419123747 ) ) ;
#864=CARTESIAN_POINT ( 'NONE',  ( -15.95412330064426065, 13.09400588185824077, -218.6613039563597169 ) ) ;
#865=CARTESIAN_POINT ( 'NONE',  ( -15.63515374589483109, 24.59141623553136569, -226.9057426066772507 ) ) ;
#866=CARTESIAN_POINT ( 'NONE',  ( 21.96352831578812115, -0.3315607655626495731, -233.9427286327413356 ) ) ;
#869=CARTESIAN_POINT ( 'NONE',  ( 19.29259174080182504, 0.5828707127177102931, -219.2781652733668807 ) ) ;
#870=CARTESIAN_POINT ( 'NONE',  ( -5.974374721719333259, -11.49502099717533454, -225.7652523315031488 ) ) ;
#871=CARTESIAN_POINT ( 'NONE',  ( 15.44226594370987726, 1.149341673865845959, -227.7740803137426724 ) ) ;
#873=CARTESIAN_POINT ( 'NONE',  ( -0.9414827276148034496, 23.96885519606619752, -216.4491898092606164 ) ) ;
#874=CARTESIAN_POINT ( 'NONE',  ( 14.69910494674137702, -2.970304755374192585, -224.5345499258161794 ) ) ;
#875=UNCERTAINTY_MEASURE_WITH_UNIT (LENGTH_MEASURE( 1.000000000000000082E-05 ), #1097, 'distance_accuracy_value', 'NONE');
#877=CARTESIAN_POINT ( 'NONE',  ( 13.85822045549773129, -1.469587484828172919, -226.8778453516271156 ) ) ;
#878=CARTESIAN_POINT ( 'NONE',  ( 9.818699534354031755, 13.69084898312510390, -233.4870046949650089 ) ) ;
#879=CARTESIAN_POINT ( 'NONE',  ( 17.60676319847677007, 21.31475060840986302, -219.8266339603936785 ) ) ;
#881=CARTESIAN_POINT ( 'NONE',  ( -13.44328839870790837, -7.440897691988615392, -217.2299511873609106 ) ) ;
#882=CARTESIAN_POINT ( 'NONE',  ( -15.22366728182010043, -5.552021002219007961, -230.2511309519622671 ) ) ;
#886=CARTESIAN_POINT ( 'NONE',  ( -9.350291727197115321, 27.53754332352430367, -230.1504993026967441 ) ) ;
#887=CARTESIAN_POINT ( 'NONE',  ( 26.46513128492211564, -16.79977778982552650, -229.3906297761492681 ) ) ;
#888=CARTESIAN_POINT ( 'NONE',  ( 20.15756451863428111, -2.090604891399794774, -217.8900786001194945 ) ) ;
#890=CARTESIAN_POINT ( 'NONE',  ( -16.32047052250102581, 2.570795953410685009, -230.9329235942756213 ) ) ;
#891=CARTESIAN_POINT ( 'NONE',  ( 18.81274554574540403, 10.85963742466947224, -234.0446454529665345 ) ) ;
#892=CARTESIAN_POINT ( 'NONE',  ( 8.250760074138732136, 14.96691001493985951, -221.7548416114337613 ) ) ;
#894=CARTESIAN_POINT ( 'NONE',  ( 1.792482182455914064, -21.59191373485632681, -217.1959973011389593 ) ) ;
#896=CARTESIAN_POINT ( 'NONE',  ( -5.191169535941942748, 31.49570301054888688, -227.4714364261087098 ) ) ;
#897=CARTESIAN_POINT ( 'NONE',  ( -4.877547524699579640, 12.94924496403020697, -219.3991240521417581 ) ) ;
#898=CARTESIAN_POINT ( 'NONE',  ( 25.79934686323926840, -4.908228874239597417, -218.4849570602390543 ) ) ;
#899=CARTESIAN_POINT ( 'NONE',  ( -11.26857159993117996, 28.96895336474501192, -225.6039696848669678 ) ) ;
#902=CARTESIAN_POINT ( 'NONE',  ( 2.770531592831002143, 22.28948935999365943, -215.1307751200139649 ) ) ;
#903=CARTESIAN_POINT ( 'NONE',  ( 14.29548763234129538, 2.320071712424730315, -230.2610858871018422 ) ) ;
#904=CARTESIAN_POINT ( 'NONE',  ( -27.29953305526601426, 11.21644211419729054, -229.3676346105362995 ) ) ;
#905=CARTESIAN_POINT ( 'NONE',  ( 14.22574309452842733, 4.476723532073429546, -225.5862451792618231 ) ) ;
#906=CARTESIAN_POINT ( 'NONE',  ( 15.61471550013173548, 0.4039561045782734117, -227.9741642728169211 ) ) ;
#908=CARTESIAN_POINT ( 'NONE',  ( -1.386728072030569692, 16.52832439466973824, -230.7516952943509807 ) ) ;
#909=CARTESIAN_POINT ( 'NONE',  ( -22.23616899077527975, -11.51447210886970751, -217.5950109096934568 ) ) ;
#910=CARTESIAN_POINT ( 'NONE',  ( 15.76910524310159900, 5.601482066865847820, -220.3440822020379528 ) ) ;
#911=CARTESIAN_POINT ( 'NONE',  ( -3.600307272616782406, -16.89541809348436630, -217.5924753110707570 ) ) ;
#913=CARTESIAN_POINT ( 'NONE',  ( -25.19248792833826300, 13.40115236862232528, -221.2817950683888455 ) ) ;
#915=CARTESIAN_POINT ( 'NONE',  ( 8.211296573249146746, -12.45047565346596130, -222.1279395315445413 ) ) ;
#916=CARTESIAN_POINT ( 'NONE',  ( 13.41709597927210496, 19.57823531746157997, -218.2666972400567147 ) ) ;
#917=CARTESIAN_POINT ( 'NONE',  ( -22.04240660558204823, 19.10355008918698871, -223.9524535985323723 ) ) ;
#918=CARTESIAN_POINT ( 'NONE',  ( -10.98447002683091256, 8.146786682930290624, -230.8316952156193338 ) ) ;
#919=CARTESIAN_POINT ( 'NONE',  ( -15.58915292315067802, -7.289217648355976742, -221.6802381019405175 ) ) ;
#921=CARTESIAN_POINT ( 'NONE',  ( 29.33969601628096768, 11.98971187598327504, -225.2039690377576733 ) ) ;
#923=CARTESIAN_POINT ( 'NONE',  ( -13.46535974834342220, -4.471564630954283359, -230.9063312536467834 ) ) ;
#924=CARTESIAN_POINT ( 'NONE',  ( -3.996294969088721505, 28.80481464818193515, -222.8623509149411746 ) ) ;
#926=CARTESIAN_POINT ( 'NONE',  ( 12.23284375931666013, 4.108221165122169616, -224.0993108960438462 ) ) ;
#927=CARTESIAN_POINT ( 'NONE',  ( -6.496078068315311427, 23.46891392553531119, -233.1042179568201220 ) ) ;
#928=CARTESIAN_POINT ( 'NONE',  ( 10.35958063030883025, 8.003303894222913328, -225.9303204057916048 ) ) ;
#931=CARTESIAN_POINT ( 'NONE',  ( -0.6467335922136470128, -17.26771294536504442, -230.4732896975262122 ) ) ;
#932=MECHANICAL_DESIGN_GEOMETRIC_PRESENTATION_REPRESENTATION('',(#4162),#19607);
#933=CARTESIAN_POINT ( 'NONE',  ( 7.092430827040528740, -27.48041265710635628, -228.4891580147104548 ) ) ;
#934=CARTESIAN_POINT ( 'NONE',  ( 20.58703255433590940, 0.4816031003617209372, -231.9427175861361263 ) ) ;
#935=CARTESIAN_POINT ( 'NONE',  ( 17.15627899979664051, -18.64955541608202694, -217.1729447097152388 ) ) ;
#936=CARTESIAN_POINT ( 'NONE',  ( -26.98579662683621194, -8.531126968542736222, -229.5232528995939845 ) ) ;
#937=CARTESIAN_POINT ( 'NONE',  ( -5.420780812268581883, -12.08122409751860360, -226.5143039284326392 ) ) ;
#938=CARTESIAN_POINT ( 'NONE',  ( 3.060417506408009469, 27.46204888741655026, -226.6022202862033623 ) ) ;
#941=CARTESIAN_POINT ( 'NONE',  ( -22.10934047915441170, 0.9940043559354162506, -215.0000000000000000 ) ) ;
#942=CARTESIAN_POINT ( 'NONE',  ( 4.343013938751969505, 13.02036404005131587, -224.7825435359082178 ) ) ;
#943=CARTESIAN_POINT ( 'NONE',  ( 0.6289891638115701067, 16.47510600144228832, -227.0521699048171342 ) ) ;
#944=CARTESIAN_POINT ( 'NONE',  ( 13.17462184258262070, -16.01403271225657932, -214.6792330615317610 ) ) ;
#946=CARTESIAN_POINT ( 'NONE',  ( 11.96568375430165254, 8.504117401580989721, -219.8633768076029753 ) ) ;
#947=CARTESIAN_POINT ( 'NONE',  ( -11.86888352782322897, 15.29489941890347282, -218.1379771575364259 ) ) ;
#948=CARTESIAN_POINT ( 'NONE',  ( -16.23590288079963173, 0.2625226423351309513, -226.8300841971807813 ) ) ;
#949=CARTESIAN_POINT ( 'NONE',  ( -1.544051355262263225, -15.46116467022245011, -222.0171457641791903 ) ) ;
#953=CARTESIAN_POINT ( 'NONE',  ( 11.87982377808925527, 10.85265283465803421, -229.5027252913499183 ) ) ;
#954=CARTESIAN_POINT ( 'NONE',  ( 11.49416291172809856, -12.02598964588280595, -221.0946228713814889 ) ) ;
#956=CARTESIAN_POINT ( 'NONE',  ( -18.14952719657095415, 1.368063294522122275, -218.0005379682515922 ) ) ;
#957=CARTESIAN_POINT ( 'NONE',  ( -1.608171596096409806, -16.77465153034988887, -217.4618546331240054 ) ) ;
#958=CARTESIAN_POINT ( 'NONE',  ( 4.730976410881341465, 17.65764351829336931, -217.6025626048331674 ) ) ;
#960=CARTESIAN_POINT ( 'NONE',  ( 3.714886539878811789, 12.88803176524806560, -219.5889136906770034 ) ) ;
#962=CARTESIAN_POINT ( 'NONE',  ( -17.39699619235753048, 15.64332637722790054, -216.0406373264262641 ) ) ;
#963=CARTESIAN_POINT ( 'NONE',  ( -14.28784611495131784, -7.281039336628973402, -230.6208668958216208 ) ) ;
#966=CARTESIAN_POINT ( 'NONE',  ( -7.395406416482832590, 12.93623984139929739, -219.2606224730616873 ) ) ;
#967=CARTESIAN_POINT ( 'NONE',  ( -3.564252528062037406, -12.01378896085460291, -227.6748268428467270 ) ) ;
#968=CARTESIAN_POINT ( 'NONE',  ( 14.83290459615719215, -2.296615622475745688, -226.9301701175285757 ) ) ;
#969=CARTESIAN_POINT ( 'NONE',  ( -15.66530208164916260, 23.23467148471576849, -218.1250122661128046 ) ) ;
#970=CARTESIAN_POINT ( 'NONE',  ( -12.13127060986278316, 5.971392262169284315, -229.0615017441034524 ) ) ;
#972=CARTESIAN_POINT ( 'NONE',  ( 5.248013545904832711, 18.51731616863089158, -219.3673127389703552 ) ) ;
#974=CARTESIAN_POINT ( 'NONE',  ( -12.12559971566433958, 1.856299769312002912, -227.8748781050665286 ) ) ;
#975=CARTESIAN_POINT ( 'NONE',  ( -14.93084585968405875, -14.53813297593447373, -219.1962364975631772 ) ) ;
#977=CARTESIAN_POINT ( 'NONE',  ( 15.37089934297015503, 20.64239674606488961, -217.2018742121147170 ) ) ;
#978=CARTESIAN_POINT ( 'NONE',  ( 2.276720224425493821, 13.44951395023989171, -229.9230017221896105 ) ) ;
#979=CARTESIAN_POINT ( 'NONE',  ( 30.81364357021286793, -2.580535071768633060, -224.0234450364292513 ) ) ;
#982=CARTESIAN_POINT ( 'NONE',  ( 18.69835413980967687, -1.262199651413310031, -230.6153330080101966 ) ) ;
#984=CARTESIAN_POINT ( 'NONE',  ( -3.496415903701482808, -16.44974864882642152, -218.6042005240371111 ) ) ;
#985=CARTESIAN_POINT ( 'NONE',  ( 24.03642272140365677, 3.646960756862087205, -218.2320643939070806 ) ) ;
#986=CARTESIAN_POINT ( 'NONE',  ( -10.24288955603410933, 28.30762631303078791, -220.8855665231519083 ) ) ;
#988=CARTESIAN_POINT ( 'NONE',  ( 13.70635042947887428, -1.390919209824193592, -225.3477037409554953 ) ) ;
#990=CARTESIAN_POINT ( 'NONE',  ( 11.20580770355584299, 27.81589616365139150, -231.3138133330081132 ) ) ;
#993=CARTESIAN_POINT ( 'NONE',  ( 25.80927844399814930, 11.21489550116160316, -221.3538377621514996 ) ) ;
#995=CARTESIAN_POINT ( 'NONE',  ( 14.68060984531904012, -6.704174034294832829, -225.1581031080203559 ) ) ;
#996=CARTESIAN_POINT ( 'NONE',  ( -25.61235545225478560, -15.41032726095661509, -226.9890212492312855 ) ) ;
#999=CARTESIAN_POINT ( 'NONE',  ( -6.072587425033909803, 24.65158735603439055, -217.4249768037189767 ) ) ;
#1000=CARTESIAN_POINT ( 'NONE',  ( 25.69865375807269459, -17.81673768310515626, -220.5381737609034474 ) ) ;
#1001=CARTESIAN_POINT ( 'NONE',  ( 22.44368505003003378, -11.72633196808685163, -232.1179326287041533 ) ) ;
#1002=CARTESIAN_POINT ( 'NONE',  ( -26.19327040236159831, 13.44417515682194875, -223.7810975255189874 ) ) ;
#1003=CARTESIAN_POINT ( 'NONE',  ( 24.81079154715000357, 3.171651085595392772, -216.4177249688571578 ) ) ;
#1004=CARTESIAN_POINT ( 'NONE',  ( 20.22510869507564024, 17.05975164568011238, -220.7829296213589316 ) ) ;
#1006=CARTESIAN_POINT ( 'NONE',  ( 8.821624174887295666, -16.56651460208862758, -234.0193988870521196 ) ) ;
#1008=CARTESIAN_POINT ( 'NONE',  ( -1.302381543002304687, 18.65968181418110206, -215.1730913991678449 ) ) ;
#1009=CARTESIAN_POINT ( 'NONE',  ( 4.719925043692215993, 22.16918918211828782, -214.6883144083888908 ) ) ;
#1010=CARTESIAN_POINT ( 'NONE',  ( 21.29805123434030634, -10.14609140759417905, -218.4136040999194108 ) ) ;
#1011=CARTESIAN_POINT ( 'NONE',  ( -8.823862513872974489, 14.92351368520778898, -217.1499513473673346 ) ) ;
#1013=CARTESIAN_POINT ( 'NONE',  ( -5.727886109716582297, 15.25217619989539486, -230.5419623196804650 ) ) ;
#1014=CARTESIAN_POINT ( 'NONE',  ( 29.96674103997387206, 4.060923908484647349, -228.5323681967686298 ) ) ;
#1015=CARTESIAN_POINT ( 'NONE',  ( -22.11084984981285118, 10.96048252433489623, -216.6117774006995376 ) ) ;
#1016=CARTESIAN_POINT ( 'NONE',  ( 16.00819137755116373, 4.595691552992191120, -229.5669508871464757 ) ) ;
#1017=CARTESIAN_POINT ( 'NONE',  ( 9.489894741926459432, 25.96007012349547338, -222.3210984495278524 ) ) ;
#1018=CARTESIAN_POINT ( 'NONE',  ( 15.50065424546137827, 0.1434261877680026442, -227.9977536057407690 ) ) ;
#1020=CARTESIAN_POINT ( 'NONE',  ( 6.685304925496912354, 17.61973327427626046, -230.4152170797364931 ) ) ;
#1021=CARTESIAN_POINT ( 'NONE',  ( -11.39823187951283501, -7.998194509987097689, -226.8062974464413912 ) ) ;
#1022=CARTESIAN_POINT ( 'NONE',  ( 15.89706143421296147, 10.57416387607782227, -218.3862415393350318 ) ) ;
#1023=CARTESIAN_POINT ( 'NONE',  ( -7.879270980303660465, -15.58863178937888350, -218.8267223810934752 ) ) ;
#1025=CARTESIAN_POINT ( 'NONE',  ( -26.11114532382342901, 12.73400870066318902, -227.7653936945517046 ) ) ;
#1026=CARTESIAN_POINT ( 'NONE',  ( 19.33791609681259160, -22.44220124466257360, -223.0821732511882090 ) ) ;
#1028=CARTESIAN_POINT ( 'NONE',  ( 10.97349919442152810, 9.416813005082010690, -227.3764328406868742 ) ) ;
#1029=CARTESIAN_POINT ( 'NONE',  ( -12.43544732248594720, 12.69828336922617318, -219.3367909706387877 ) ) ;
#1030=CARTESIAN_POINT ( 'NONE',  ( -12.61443312487471324, 8.399394471292156439, -217.5740162615319093 ) ) ;
#1032=CARTESIAN_POINT ( 'NONE',  ( -24.13290183362846264, -6.995619630784887022, -220.0347092962472288 ) ) ;
#1034=CARTESIAN_POINT ( 'NONE',  ( 11.17228388010293649, 5.622653638471959425, -222.3672781564363845 ) ) ;
#1036=CARTESIAN_POINT ( 'NONE',  ( -15.94006964721192432, -5.209069452486915885, -233.2212940081757040 ) ) ;
#1037=CARTESIAN_POINT ( 'NONE',  ( 8.175342817246784577, 19.41817470142738244, -216.6818271833384699 ) ) ;
#1038=CARTESIAN_POINT ( 'NONE',  ( -21.48978835671764287, 1.062155088816892468, -219.0000000007146355 ) ) ;
#1039=CARTESIAN_POINT ( 'NONE',  ( -10.45265333418718612, 16.71118685480038479, -231.7490466715443631 ) ) ;
#1040=CARTESIAN_POINT ( 'NONE',  ( 4.024086222410633518, 12.48004227094270746, -230.0177668608922374 ) ) ;
#1042=CARTESIAN_POINT ( 'NONE',  ( 0.6118723529980315545, -20.11903950562274446, -217.9558718073025716 ) ) ;
#1044=CARTESIAN_POINT ( 'NONE',  ( -6.723652888800149441, -28.28510889945508211, -226.1741921951756638 ) ) ;
#1045=CARTESIAN_POINT ( 'NONE',  ( 16.38151749656409351, 8.902090001712490874, -231.2955017965201989 ) ) ;
#1046=CARTESIAN_POINT ( 'NONE',  ( 13.82188917133564132, -5.740199443570373816, -227.9076376976435654 ) ) ;
#1047=CARTESIAN_POINT ( 'NONE',  ( 30.21546680466445167, 0.1681144524405517038, -223.7059097242262737 ) ) ;
#1048=CARTESIAN_POINT ( 'NONE',  ( -8.878187501988019648, -11.23476449186280846, -221.0271673637577123 ) ) ;
#1049=CARTESIAN_POINT ( 'NONE',  ( 3.755404788550845474, 24.96758616565139022, -220.0839658302907935 ) ) ;
#1051=CARTESIAN_POINT ( 'NONE',  ( -16.40095417437164471, 2.582410108382750646, -233.5151473761628154 ) ) ;
#1052=CARTESIAN_POINT ( 'NONE',  ( -0.9414827276148034496, 23.96885519606619752, -216.4491898092606164 ) ) ;
#1053=CARTESIAN_POINT ( 'NONE',  ( 2.445562843591592372, 25.89340784564244657, -229.2671352353737859 ) ) ;
#1054=CARTESIAN_POINT ( 'NONE',  ( 15.44393261315032184, -28.37553556939610999, -226.2064134899511600 ) ) ;
#1055=CARTESIAN_POINT ( 'NONE',  ( 28.03290210476798094, 13.48017620089690638, -224.9212082181537937 ) ) ;
#1056=CARTESIAN_POINT ( 'NONE',  ( -11.83954511762131112, 10.58068896997146346, -226.6171226499791089 ) ) ;
#1057=CARTESIAN_POINT ( 'NONE',  ( -20.67624351032310059, -0.8683020119106035217, -219.0957770725675005 ) ) ;
#1058=CARTESIAN_POINT ( 'NONE',  ( -6.749503758482277682, -23.22604375411988187, -218.1095993038993299 ) ) ;
#1061=CARTESIAN_POINT ( 'NONE',  ( 15.85665641241444668, 18.24713744004561988, -217.7195292979064902 ) ) ;
#1062=CARTESIAN_POINT ( 'NONE',  ( 13.74877878529187747, -9.499568690286848138, -221.9332727739125346 ) ) ;
#1063=CARTESIAN_POINT ( 'NONE',  ( -24.15814485343234352, 4.373587128574028426, -232.6698675874553430 ) ) ;
#1064=CARTESIAN_POINT ( 'NONE',  ( -9.078153229956912540, -10.71731945587431056, -228.5228069477245469 ) ) ;
#1066=CARTESIAN_POINT ( 'NONE',  ( 4.907833106823921376, 13.98151846258800290, -229.0190609869640923 ) ) ;
#1067=CARTESIAN_POINT ( 'NONE',  ( 3.490829917597003895, 11.40812925993816229, -222.8973702487053004 ) ) ;
#1069=CARTESIAN_POINT ( 'NONE',  ( -3.205260335674071648, 17.52234722004434531, -232.9754319808710363 ) ) ;
#1070=CARTESIAN_POINT ( 'NONE',  ( -30.29980174031923923, -2.072322947205907706, -221.9291348703773679 ) ) ;
#1073=CARTESIAN_POINT ( 'NONE',  ( -14.83974801774860630, 13.71714848582103485, -216.0935642439352762 ) ) ;
#1074=CARTESIAN_POINT ( 'NONE',  ( -2.809719670556939608, -23.45209095268191390, -234.3886352793013543 ) ) ;
#1076=CARTESIAN_POINT ( 'NONE',  ( -15.58461825850822180, 18.91734573546571951, -233.7691177939990723 ) ) ;
#1077=CARTESIAN_POINT ( 'NONE',  ( -12.79639481117843935, 1.974037863663017589, -229.6094308443170746 ) ) ;
#1078=CARTESIAN_POINT ( 'NONE',  ( -0.4548635697939061306, 27.30478022265488036, -219.8474162243132071 ) ) ;
#1080=CARTESIAN_POINT ( 'NONE',  ( 22.37742875470728876, 11.29804624588327577, -218.9256858961603882 ) ) ;
#1081=CARTESIAN_POINT ( 'NONE',  ( -6.877419757825867563, -14.31154863906730412, -224.3431884172090918 ) ) ;
#1083=CARTESIAN_POINT ( 'NONE',  ( -15.11329978779464689, 11.41628732213579411, -231.7124318929555500 ) ) ;
#1084=CARTESIAN_POINT ( 'NONE',  ( 10.95881707662767290, 12.06788758096456782, -231.4359029166177208 ) ) ;
#1085=CARTESIAN_POINT ( 'NONE',  ( -4.021035526861677312, 25.02763064454595110, -216.6167103172201678 ) ) ;
#1086=CARTESIAN_POINT ( 'NONE',  ( 14.79879825009101069, -3.130997509566451953, -219.4569190381675696 ) ) ;
#1089=CARTESIAN_POINT ( 'NONE',  ( -13.58874046263339608, 12.73011668665171392, -216.5659449791897941 ) ) ;
#1090=CARTESIAN_POINT ( 'NONE',  ( -15.77287877451090203, -21.23371664991514152, -233.2776952697515185 ) ) ;
#1092=CARTESIAN_POINT ( 'NONE',  ( 10.02513374692848913, 18.81568788741115128, -217.1505009242214612 ) ) ;
#1095=CARTESIAN_POINT ( 'NONE',  ( -15.10945752141584464, 6.470132813599071220, -220.1568141593501764 ) ) ;
#1096=CARTESIAN_POINT ( 'NONE',  ( 13.09827881591457022, 28.40264942367575784, -221.1045935444571455 ) ) ;
#1097=( LENGTH_UNIT ( ) NAMED_UNIT ( * ) SI_UNIT ( .MILLI., .METRE. ) );
#1099=CARTESIAN_POINT ( 'NONE',  ( 16.54345861550681107, 19.37554510112122230, -218.2240151908141002 ) ) ;
#1101=CARTESIAN_POINT ( 'NONE',  ( 17.78543650172321833, -3.538499054913423869, -220.4382406111031401 ) ) ;
#1103=CARTESIAN_POINT ( 'NONE',  ( -12.13177435108894642, -8.392035797555511323, -228.8392847287196332 ) ) ;
#1106=CARTESIAN_POINT ( 'NONE',  ( -1.238249567024760189, 29.30580384236933966, -223.2399636023643836 ) ) ;
#1107=CARTESIAN_POINT ( 'NONE',  ( 15.19497947618244460, -8.176986896541109218, -234.2449823452919304 ) ) ;
#1108=CARTESIAN_POINT ( 'NONE',  ( 22.14671607713456325, -14.13547298543019437, -218.1897693226341914 ) ) ;
#1109=CARTESIAN_POINT ( 'NONE',  ( -13.97943781666340790, 5.798109546139844639, -228.2992319913466019 ) ) ;
#1110=CARTESIAN_POINT ( 'NONE',  ( 14.33191776452776622, 5.147404080619256916, -219.0172570056664938 ) ) ;
#1111=CARTESIAN_POINT ( 'NONE',  ( 12.94599882983645145, 15.82237817288049442, -219.3332542656393116 ) ) ;
#1113=CARTESIAN_POINT ( 'NONE',  ( -0.09985864093865706725, -15.05342968659714309, -222.4585048042796132 ) ) ;
#1115=CARTESIAN_POINT ( 'NONE',  ( -15.35982698007958724, 5.508237851081846159, -233.6994028941782631 ) ) ;
#1116=CARTESIAN_POINT ( 'NONE',  ( 7.393167209263542539, 10.77319710117329699, -221.1179833906701049 ) ) ;
#1117=CARTESIAN_POINT ( 'NONE',  ( -2.577721557973523314, 25.83760098923793791, -215.4660676095525389 ) ) ;
#1118=CARTESIAN_POINT ( 'NONE',  ( 29.05460218321669785, -4.534277981440765437, -222.0637325791020373 ) ) ;
#1119=CARTESIAN_POINT ( 'NONE',  ( -8.172572110426221670, 16.86653848210977813, -233.4220330256369493 ) ) ;
#1120=CARTESIAN_POINT ( 'NONE',  ( -20.94800339253696109, 4.477632454355491731, -216.5423208360950298 ) ) ;
#1121=CARTESIAN_POINT ( 'NONE',  ( 2.165130313308041288, 31.55305250914585002, -225.6791154433767304 ) ) ;
#1122=CARTESIAN_POINT ( 'NONE',  ( -18.04102731735134313, 0.8647102676311391178, -229.4625228093430849 ) ) ;
#1123=CARTESIAN_POINT ( 'NONE',  ( -15.15434969228324924, 4.423874646950748613, -230.6144467931089821 ) ) ;
#1124=CARTESIAN_POINT ( 'NONE',  ( 18.76922974182421555, 13.12635134380198210, -217.8010375391909008 ) ) ;
#1125=CARTESIAN_POINT ( 'NONE',  ( 2.445562843591592372, 25.89340784564244657, -229.2671352353737859 ) ) ;
#1128=CARTESIAN_POINT ( 'NONE',  ( 8.539351012053531420, 16.03230746435535181, -220.6282946404833751 ) ) ;
#1129=CARTESIAN_POINT ( 'NONE',  ( -14.76273180397945772, -6.370707202906876532, -220.0066229284273334 ) ) ;
#1130=CARTESIAN_POINT ( 'NONE',  ( 17.00168025137501004, 6.212099629982537508, -219.0548246536471595 ) ) ;
#1131=CARTESIAN_POINT ( 'NONE',  ( -5.234434610370643171, -17.78654814248861626, -233.1081320952062867 ) ) ;
#1134=CARTESIAN_POINT ( 'NONE',  ( -16.12870690754239078, 23.19263481078822053, -221.6099859194323471 ) ) ;
#1136=CARTESIAN_POINT ( 'NONE',  ( 13.93061470302797389, -11.80544459979379646, -217.9389246709861538 ) ) ;
#1137=CARTESIAN_POINT ( 'NONE',  ( 26.72610819325501907, 14.97064052581051108, -224.6384473985499426 ) ) ;
#1138=CARTESIAN_POINT ( 'NONE',  ( -11.03778527004271659, 26.96286968643956428, -225.4057095641571209 ) ) ;
#1139=CARTESIAN_POINT ( 'NONE',  ( -12.14471622011552832, 3.716031503296523653, -220.6237729066402835 ) ) ;
#1140=CARTESIAN_POINT ( 'NONE',  ( -23.54933555373352050, -14.29320362656835997, -227.5895276738501423 ) ) ;
#1142=CARTESIAN_POINT ( 'NONE',  ( 15.87399429023076003, -1.683916961781461552, -230.8621029165058758 ) ) ;
#1145=CARTESIAN_POINT ( 'NONE',  ( -18.48589171870721870, -21.38265182533571362, -233.2911668074952729 ) ) ;
#1146=CARTESIAN_POINT ( 'NONE',  ( 20.26651059498356844, 18.95255124124090074, -231.7206897233655525 ) ) ;
#1147=CARTESIAN_POINT ( 'NONE',  ( 25.50289296650958448, 5.998088869914441901, -233.1161630295026157 ) ) ;
#1149=CARTESIAN_POINT ( 'NONE',  ( -4.021035526861677312, 25.02763064454595110, -216.6167103172201678 ) ) ;
#1151=CARTESIAN_POINT ( 'NONE',  ( 12.46318849118074112, 25.01309605388695445, -216.9820503660967859 ) ) ;
#1153=CARTESIAN_POINT ( 'NONE',  ( 0.5598654370342924791, -17.79304497667748564, -219.0037976856824571 ) ) ;
#1154=CARTESIAN_POINT ( 'NONE',  ( -6.507186921339367380, -21.94905981650347826, -217.8194053188079238 ) ) ;
#1156=CARTESIAN_POINT ( 'NONE',  ( -13.91932826323387395, 8.983986115891950064, -216.4624824187541776 ) ) ;
#1157=CARTESIAN_POINT ( 'NONE',  ( 17.28140336138120858, -11.48510652344925020, -216.9852223368602893 ) ) ;
#1158=CARTESIAN_POINT ( 'NONE',  ( -18.34948365288241590, -1.907751280579004893, -231.5848060246952116 ) ) ;
#1159=CARTESIAN_POINT ( 'NONE',  ( -21.28605893225895684, -20.43870967537180050, -221.0356759888913700 ) ) ;
#1160=CARTESIAN_POINT ( 'NONE',  ( 16.73391517716289911, 11.95167056011791828, -233.0268722588312755 ) ) ;
#1162=CARTESIAN_POINT ( 'NONE',  ( -9.982417347796181062, 8.907629238417765549, -225.5124013436514474 ) ) ;
#1163=CARTESIAN_POINT ( 'NONE',  ( 13.25330606581809789, 10.40242132629824034, -230.9170765704288044 ) ) ;
#1164=CARTESIAN_POINT ( 'NONE',  ( 11.67669251569587985, 24.04736029062789981, -218.5856804285192254 ) ) ;
#1165=CARTESIAN_POINT ( 'NONE',  ( 20.85755584069816493, 20.53615333921957742, -227.2010381488614996 ) ) ;
#1166=CARTESIAN_POINT ( 'NONE',  ( 12.01003603113874441, -9.270215614621081457, -232.3219482526175170 ) ) ;
#1167=CARTESIAN_POINT ( 'NONE',  ( 20.26651059498356844, 18.95255124124090074, -231.7206897233655525 ) ) ;
#1168=CARTESIAN_POINT ( 'NONE',  ( -12.14452111807825041, 26.21581784948545035, -221.1455569020914140 ) ) ;
#1169=CARTESIAN_POINT ( 'NONE',  ( -2.609511328024065602, -16.97143768612226822, -230.2205646068415490 ) ) ;
#1170=CARTESIAN_POINT ( 'NONE',  ( -14.87984907657228639, 0.2138881189739126887, -228.7773920408832282 ) ) ;
#1174=CARTESIAN_POINT ( 'NONE',  ( 25.80927844399814930, 11.21489550116160316, -221.3538377621514996 ) ) ;
#1175=CARTESIAN_POINT ( 'NONE',  ( 10.87273020620571629, -12.78363999705779186, -228.8712466752294858 ) ) ;
#1177=CARTESIAN_POINT ( 'NONE',  ( -10.11868820210310282, -13.51996935893276053, -218.1704188629865371 ) ) ;
#1178=CARTESIAN_POINT ( 'NONE',  ( -0.9414827276148034496, 23.96885519606619752, -216.4491898092606164 ) ) ;
#1179=CARTESIAN_POINT ( 'NONE',  ( 7.587775680576782200, 20.81864918083767435, -235.2547171215352364 ) ) ;
#1181=CARTESIAN_POINT ( 'NONE',  ( -2.698926868850080041, 12.89339462271858316, -226.7595176699009585 ) ) ;
#1182=CARTESIAN_POINT ( 'NONE',  ( 28.84595539031434797, -3.450543886267656735, -229.1532420603894877 ) ) ;
#1183=CARTESIAN_POINT ( 'NONE',  ( 29.37495210618232022, -3.074218464324032229, -220.1817713028459025 ) ) ;
#1185=CARTESIAN_POINT ( 'NONE',  ( -3.082945806077231676, 30.69897765966285874, -224.2387254578930822 ) ) ;
#1186=CARTESIAN_POINT ( 'NONE',  ( -13.54879968420069503, -27.67624318860520916, -230.2549257473255579 ) ) ;
#1187=CARTESIAN_POINT ( 'NONE',  ( 13.47054497134856277, -24.75371201277411615, -218.7687119198782000 ) ) ;
#1189=CARTESIAN_POINT ( 'NONE',  ( 20.98776729843937972, -13.55153944770713359, -217.5092423276211946 ) ) ;
#1191=CARTESIAN_POINT ( 'NONE',  ( 16.55609572527610851, 2.729108819536508967, -230.5704679660131831 ) ) ;
#1192=CARTESIAN_POINT ( 'NONE',  ( 6.332229114051408203, 16.75791367489523154, -229.7702805136205200 ) ) ;
#1194=CARTESIAN_POINT ( 'NONE',  ( -25.59521542166570640, 7.637420400166985424, -216.4190921938142935 ) ) ;
#1195=CARTESIAN_POINT ( 'NONE',  ( -23.09090074015852778, -15.52172445179926896, -222.9863534629544972 ) ) ;
#1197=CARTESIAN_POINT ( 'NONE',  ( -12.82737030338386219, 8.595865151885988098, -221.6735325378515142 ) ) ;
#1198=CARTESIAN_POINT ( 'NONE',  ( 2.535512286608554433, 13.86868953312499109, -224.9313928733152181 ) ) ;
#1199=CARTESIAN_POINT ( 'NONE',  ( 2.291262277241625345, 17.20278591336981222, -216.2185160402476924 ) ) ;
#1200=CARTESIAN_POINT ( 'NONE',  ( -22.73111095712577168, -10.24355154293710690, -230.8570942615963872 ) ) ;
#1203=CARTESIAN_POINT ( 'NONE',  ( -22.04257564474043818, 18.72061943465525857, -219.1781831295219263 ) ) ;
#1204=CARTESIAN_POINT ( 'NONE',  ( -17.08385316318651448, -18.56764924811779949, -215.7277288032969977 ) ) ;
#1206=CARTESIAN_POINT ( 'NONE',  ( 17.60676319847677007, 21.31475060840986302, -219.8266339603936785 ) ) ;
#1212=CARTESIAN_POINT ( 'NONE',  ( -19.27153818831731158, 23.75761453444584248, -221.9111479746408975 ) ) ;
#1213=CARTESIAN_POINT ( 'NONE',  ( 22.05207439088920651, 1.190718621721708947, -218.4927357815377604 ) ) ;
#1217=CARTESIAN_POINT ( 'NONE',  ( 23.48259192634075632, -8.786327662478353062, -220.0176983167915807 ) ) ;
#1218=CARTESIAN_POINT ( 'NONE',  ( -16.76449091996730090, -6.021196472930381738, -231.5810252088758432 ) ) ;
#1221=CARTESIAN_POINT ( 'NONE',  ( -8.894613172508529786, 25.42460746921206294, -232.3150764041658363 ) ) ;
#1222=CARTESIAN_POINT ( 'NONE',  ( 12.79824285610881063, -25.13061632922516253, -232.1172912921500426 ) ) ;
#1224=CARTESIAN_POINT ( 'NONE',  ( 26.54225689383817866, -6.924125931238839016, -230.1506921200174247 ) ) ;
#1225=CARTESIAN_POINT ( 'NONE',  ( -13.96147744945181124, 5.260363697127891314, -222.3342733685200301 ) ) ;
#1226=CARTESIAN_POINT ( 'NONE',  ( -17.72669652144150376, 1.460525322529694581, -220.6883622781615202 ) ) ;
#1227=CARTESIAN_POINT ( 'NONE',  ( 14.73597170006453361, 7.272367905564328439, -221.0092474305599239 ) ) ;
#1229=CARTESIAN_POINT ( 'NONE',  ( -0.8455829679720252567, -23.09678443543459991, -232.4899849032512122 ) ) ;
#1230=CARTESIAN_POINT ( 'NONE',  ( 15.01439307471096463, 1.118969480519667048, -226.7488225241675366 ) ) ;
#1231=CARTESIAN_POINT ( 'NONE',  ( -20.87212828950092813, -0.8819659211619411687, -215.0000000018925448 ) ) ;
#1232=CARTESIAN_POINT ( 'NONE',  ( 15.23494377589453919, 15.24947835004434538, -215.7641128510430519 ) ) ;
#1233=CARTESIAN_POINT ( 'NONE',  ( 1.557078628722260438, 24.20011951319323273, -235.1441088220640268 ) ) ;
#1234=CARTESIAN_POINT ( 'NONE',  ( 16.50219604690516206, -6.005650786285340104, -230.9082164827931933 ) ) ;
#1235=CARTESIAN_POINT ( 'NONE',  ( -14.73016414256368911, 22.23431809695627237, -217.1425123644553707 ) ) ;
#1236=CARTESIAN_POINT ( 'NONE',  ( -28.13472254077564116, 12.33996625515159629, -224.9141344439281909 ) ) ;
#1238=CARTESIAN_POINT ( 'NONE',  ( 8.865150807857233417, 8.939496441981303221, -220.7647208555746090 ) ) ;
#1239=CARTESIAN_POINT ( 'NONE',  ( -27.56397725925346975, 4.259055856374357241, -222.4951663284069241 ) ) ;
#1240=CARTESIAN_POINT ( 'NONE',  ( -3.673551555920188783, 29.81207051619892923, -228.8770490300152005 ) ) ;
#1242=CARTESIAN_POINT ( 'NONE',  ( 25.33562512631297281, 12.25422971834577268, -228.6777356031426791 ) ) ;
#1243=CARTESIAN_POINT ( 'NONE',  ( 7.067550969709256670, 17.75197616922148569, -219.3387126207321955 ) ) ;
#1244=CARTESIAN_POINT ( 'NONE',  ( 15.05575868828727515, -2.428864548505686560, -227.9368649688638584 ) ) ;
#1246=CARTESIAN_POINT ( 'NONE',  ( -26.43144772945995413, -6.745116643720071359, -219.5134289301136050 ) ) ;
#1247=CARTESIAN_POINT ( 'NONE',  ( 14.68783945462866924, 9.535285537539673228, -219.4694094309942045 ) ) ;
#1248=CARTESIAN_POINT ( 'NONE',  ( -2.827720241434194648, -28.87017495157254743, -218.9856045314649577 ) ) ;
#1250=CARTESIAN_POINT ( 'NONE',  ( -10.32994309255856535, 16.55762392127841665, -218.3313395458419279 ) ) ;
#1251=CARTESIAN_POINT ( 'NONE',  ( 11.63416633096549369, -11.60453582225250990, -230.7583135875248104 ) ) ;
#1252=CARTESIAN_POINT ( 'NONE',  ( 12.79953165872901266, 10.20044330008568778, -230.3912386799665626 ) ) ;
#1253=CARTESIAN_POINT ( 'NONE',  ( -4.080659539198054020, 15.43130099126780408, -228.8058965243247656 ) ) ;
#1254=CARTESIAN_POINT ( 'NONE',  ( -17.58289524052909414, 0.7988212499981205417, -233.9567931471624149 ) ) ;
#1255=CARTESIAN_POINT ( 'NONE',  ( -23.46219451118877330, -13.03948552059806509, -221.3852197888554372 ) ) ;
#1256=CARTESIAN_POINT ( 'NONE',  ( 28.77543668145700195, 2.466904630248945907, -219.6646827587300947 ) ) ;
#1259=CARTESIAN_POINT ( 'NONE',  ( -23.85689329484546661, -4.322701801676343436, -216.0188046937498996 ) ) ;
#1260=CARTESIAN_POINT ( 'NONE',  ( 23.18902850759750933, 20.27908137164207147, -226.2847847834817117 ) ) ;
#1261=CARTESIAN_POINT ( 'NONE',  ( -26.04932551096112192, 5.001193774903864409, -228.9498367494266802 ) ) ;
#1262=CARTESIAN_POINT ( 'NONE',  ( 2.291262277241625345, 17.20278591336981222, -216.2185160402476924 ) ) ;
#1263=CARTESIAN_POINT ( 'NONE',  ( 7.803634760976553508, 10.78293796201124266, -229.6314106675118865 ) ) ;
#1264=EDGE_CURVE ( 'NONE', #8552, #15629, #3655, .T. ) ;
#1265=CARTESIAN_POINT ( 'NONE',  ( -3.786803964513834941, -14.74062382431161566, -229.2965385003435586 ) ) ;
#1267=CARTESIAN_POINT ( 'NONE',  ( 2.283233934795953601, -16.37150177406293849, -220.5471140349473842 ) ) ;
#1268=CARTESIAN_POINT ( 'NONE',  ( -11.89542918462869103, -0.2773029175206048191, -224.4556830488584467 ) ) ;
#1269=CARTESIAN_POINT ( 'NONE',  ( 14.31589812732703670, -5.349901619299376243, -221.2752230612865105 ) ) ;
#1270=CARTESIAN_POINT ( 'NONE',  ( -20.85586116824185510, -1.996934699305910499, -232.3804859832740135 ) ) ;
#1272=CARTESIAN_POINT ( 'NONE',  ( -13.33530847390368024, -5.065163879519744228, -226.5386329521395226 ) ) ;
#1274=CARTESIAN_POINT ( 'NONE',  ( 10.59524789654300925, 9.532374763983630928, -223.0758647391057821 ) ) ;
#1276=CARTESIAN_POINT ( 'NONE',  ( -21.12280458060320498, 13.61074013710079988, -216.5529903464332335 ) ) ;
#1277=CARTESIAN_POINT ( 'NONE',  ( 12.14863411169100971, 10.95505907656739097, -219.3725293661985063 ) ) ;
#1278=CARTESIAN_POINT ( 'NONE',  ( 12.04687593227112430, 27.54339840196571743, -224.6466266724203820 ) ) ;
#1279=CARTESIAN_POINT ( 'NONE',  ( 13.50603691942335693, 22.79443449215731832, -229.7689193854997995 ) ) ;
#1280=CARTESIAN_POINT ( 'NONE',  ( 15.81704710165450756, -18.55181613945514840, -214.8869746720286287 ) ) ;
#1281=CARTESIAN_POINT ( 'NONE',  ( -9.982417347796181062, 8.907629238417765549, -225.5124013436514474 ) ) ;
#1282=CARTESIAN_POINT ( 'NONE',  ( -5.566280468132954518, 29.91920859341914962, -222.2705790733167817 ) ) ;
#1283=CARTESIAN_POINT ( 'NONE',  ( -19.75205891382245227, -22.10994567413457546, -223.7241504221178729 ) ) ;
#1284=CARTESIAN_POINT ( 'NONE',  ( -17.96792326766206926, -0.6237852504629022299, -217.9759415197746932 ) ) ;
#1286=CARTESIAN_POINT ( 'NONE',  ( 22.66390650824515873, 11.48342577402021725, -231.3155567808436217 ) ) ;
#1287=CARTESIAN_POINT ( 'NONE',  ( 15.27128302093890255, -22.10320814337061535, -229.9052109820655119 ) ) ;
#1288=CARTESIAN_POINT ( 'NONE',  ( -21.23733589435050817, 17.25275849955597351, -229.9547908233139708 ) ) ;
#1290=CARTESIAN_POINT ( 'NONE',  ( -21.28605893225895684, -20.43870967537180050, -221.0356759888913700 ) ) ;
#1291=CARTESIAN_POINT ( 'NONE',  ( -19.11923763334766946, 1.257783214997954202, -219.7591028439344711 ) ) ;
#1292=CARTESIAN_POINT ( 'NONE',  ( 12.58577552758108986, 11.40439409249366420, -217.4478085440898951 ) ) ;
#1294=CARTESIAN_POINT ( 'NONE',  ( 3.763426558366607111, 28.60172112197566818, -230.1816715025297526 ) ) ;
#1295=CARTESIAN_POINT ( 'NONE',  ( -26.47652094774193188, -8.527600130219385122, -218.5932275281782324 ) ) ;
#1298=CARTESIAN_POINT ( 'NONE',  ( -3.003186468682855104, 15.63968344752823469, -231.5301608670590667 ) ) ;
#1299=CARTESIAN_POINT ( 'NONE',  ( -17.24073315697368969, -20.31883122441189826, -234.2947248507418863 ) ) ;
#1300=CARTESIAN_POINT ( 'NONE',  ( 2.378655016347637652, -14.31292064579845302, -219.9942319014987220 ) ) ;
#1301=CARTESIAN_POINT ( 'NONE',  ( 22.14341918773124362, -7.622004812940091689, -217.4502831791021720 ) ) ;
#1302=CARTESIAN_POINT ( 'NONE',  ( -10.30040261405712698, 19.75576125044891285, -218.0811964201226658 ) ) ;
#1303=CARTESIAN_POINT ( 'NONE',  ( 10.90137817157632227, 16.64712710991609868, -230.5401786220292593 ) ) ;
#1305=CARTESIAN_POINT ( 'NONE',  ( -21.75607741976026333, 20.26169853110213381, -228.4128163609909450 ) ) ;
#1306=CARTESIAN_POINT ( 'NONE',  ( -15.14636561941736481, -8.091785236158230532, -228.8632199501622608 ) ) ;
#1308=CARTESIAN_POINT ( 'NONE',  ( -14.87932799058895128, 18.71706570923887369, -231.8731726670167745 ) ) ;
#1309=CARTESIAN_POINT ( 'NONE',  ( 26.28575214971901630, 3.591103948354015696, -217.0994821834097763 ) ) ;
#1310=CARTESIAN_POINT ( 'NONE',  ( -5.529079411693809121, 13.00503897727793401, -226.8014833675713646 ) ) ;
#1312=CARTESIAN_POINT ( 'NONE',  ( 17.93010821528303822, -10.80507700282924688, -233.3968735006674251 ) ) ;
#1315=CARTESIAN_POINT ( 'NONE',  ( -17.39699619235753048, 15.64332637722790054, -216.0406373264262641 ) ) ;
#1316=CARTESIAN_POINT ( 'NONE',  ( -7.243062456665192883, -20.67674855546218637, -233.5126394780404553 ) ) ;
#1318=CARTESIAN_POINT ( 'NONE',  ( 4.907833106823921376, 13.98151846258800290, -229.0190609869640923 ) ) ;
#1320=PRODUCT_DEFINITION_CONTEXT ( 'detailed design', #3384, 'design' ) ;
#1321=CARTESIAN_POINT ( 'NONE',  ( 19.06763123184207487, -2.048228142369658666, -218.2337357994572073 ) ) ;
#1323=CARTESIAN_POINT ( 'NONE',  ( -28.17543631911187063, 3.557555778861649642, -230.1980773687482156 ) ) ;
#1324=CARTESIAN_POINT ( 'NONE',  ( -17.94782256308196366, 19.07396065564992682, -232.7143578890335220 ) ) ;
#1325=CARTESIAN_POINT ( 'NONE',  ( 14.21126657910812874, 6.833562750302326627, -220.2783117037562874 ) ) ;
#1326=CARTESIAN_POINT ( 'NONE',  ( 14.45550103314422508, 0.1264054796715357587, -222.0026434553262504 ) ) ;
#1329=CARTESIAN_POINT ( 'NONE',  ( 26.42227051273691885, -8.869064526452445918, -225.3570890864022260 ) ) ;
#1330=CARTESIAN_POINT ( 'NONE',  ( -22.23616899077527975, -11.51447210886970751, -217.5950109096934568 ) ) ;
#1333=CARTESIAN_POINT ( 'NONE',  ( 8.250760074138732136, 14.96691001493985951, -221.7548416114337613 ) ) ;
#1334=CARTESIAN_POINT ( 'NONE',  ( 8.477993572791891808, -8.340333012420144243, -224.9486226631276793 ) ) ;
#1335=CARTESIAN_POINT ( 'NONE',  ( 6.741123954526870854, -14.00899218320067341, -219.0418835583997179 ) ) ;
#1337=CARTESIAN_POINT ( 'NONE',  ( -9.954421844142357756, 11.21484508112568079, -226.0177122452137439 ) ) ;
#1338=CARTESIAN_POINT ( 'NONE',  ( 17.22423229049764970, 1.395540479540137380, -217.3898520248025363 ) ) ;
#1339=CARTESIAN_POINT ( 'NONE',  ( 22.37742875470728876, 11.29804624588327577, -218.9256858961603882 ) ) ;
#1340=CARTESIAN_POINT ( 'NONE',  ( -7.719684133369767665, -19.28933804209621528, -218.9187502689394478 ) ) ;
#1342=CARTESIAN_POINT ( 'NONE',  ( -11.10150084103673684, 3.549415896002023896, -226.0408865487038952 ) ) ;
#1344=CARTESIAN_POINT ( 'NONE',  ( 4.228809304811371739, 12.93497549386982470, -230.7917784105561907 ) ) ;
#1345=CARTESIAN_POINT ( 'NONE',  ( -0.4465333940385243228, 12.27026616490476485, -221.3722328744566425 ) ) ;
#1346=CARTESIAN_POINT ( 'NONE',  ( 15.06969459085678942, -9.685035337269850331, -230.1890524597188801 ) ) ;
#1347=CARTESIAN_POINT ( 'NONE',  ( -11.69688825528096388, 18.63404371591177622, -215.8612738028812714 ) ) ;
#1348=CARTESIAN_POINT ( 'NONE',  ( -13.56774755469388616, 7.311522441667196226, -219.1912666243428021 ) ) ;
#1349=CARTESIAN_POINT ( 'NONE',  ( 3.137667653003819446, 15.44806861187908176, -232.6841782316817842 ) ) ;
#1350=CARTESIAN_POINT ( 'NONE',  ( -16.66929017373293931, 3.065794289431343689, -220.7800282905443794 ) ) ;
#1351=CARTESIAN_POINT ( 'NONE',  ( -3.082945806077231676, 30.69897765966285874, -224.2387254578930822 ) ) ;
#1352=CARTESIAN_POINT ( 'NONE',  ( 19.20300624114736721, 0.6066039755357417462, -231.5046416827383950 ) ) ;
#1353=CARTESIAN_POINT ( 'NONE',  ( 12.83388873239664996, 22.07510045760132655, -230.4740059944613222 ) ) ;
#1354=CARTESIAN_POINT ( 'NONE',  ( 24.56541673123750158, -5.996287403333383281, -231.6940117905984664 ) ) ;
#1356=CARTESIAN_POINT ( 'NONE',  ( -28.87859926594958537, -0.8320174534291842061, -222.6356913548140142 ) ) ;
#1357=CARTESIAN_POINT ( 'NONE',  ( 14.80394259695730064, 1.224172658189580432, -225.4564070658925061 ) ) ;
#1358=CARTESIAN_POINT ( 'NONE',  ( -20.91998163778511355, -19.58520498255836628, -224.2692832511962990 ) ) ;
#1360=CARTESIAN_POINT ( 'NONE',  ( -12.78923236353123727, 15.53885160143439315, -231.8946633672937878 ) ) ;
#1361=CARTESIAN_POINT ( 'NONE',  ( 21.28562020585086501, -15.94148943779260819, -218.1725164024425396 ) ) ;
#1362=CARTESIAN_POINT ( 'NONE',  ( 11.83256327006771969, 5.988634687709346593, -225.8999299265561831 ) ) ;
#1363=CARTESIAN_POINT ( 'NONE',  ( -17.14223598032838325, 23.31797360549976261, -226.5771676936548431 ) ) ;
#1364=CARTESIAN_POINT ( 'NONE',  ( -7.834600152078401436, 27.83486203824852012, -220.1209588485844222 ) ) ;
#1366=CARTESIAN_POINT ( 'NONE',  ( -13.13215111221786024, -8.938624195428067409, -226.3235457059856515 ) ) ;
#1367=CARTESIAN_POINT ( 'NONE',  ( 20.09685469220202236, -2.033783885649083079, -233.1448060988079760 ) ) ;
#1369=CARTESIAN_POINT ( 'NONE',  ( -28.08095947817005822, 1.343466879924336999, -219.1986237337335695 ) ) ;
#1370=CARTESIAN_POINT ( 'NONE',  ( 5.702651035983461902, 12.42242820409033222, -224.7304266323218656 ) ) ;
#1371=CARTESIAN_POINT ( 'NONE',  ( -17.29038495093124084, 2.707785585324113065, -229.0475017805649998 ) ) ;
#1372=CARTESIAN_POINT ( 'NONE',  ( 2.000982021813747291, 12.72833461843010205, -228.3416607300594308 ) ) ;
#1373=CARTESIAN_POINT ( 'NONE',  ( 17.76485367938521875, 4.373152267827974171, -218.8623009891758215 ) ) ;
#1374=CARTESIAN_POINT ( 'NONE',  ( -8.731539701382653007, -8.828156491469059119, -227.3463890218280596 ) ) ;
#1376=CARTESIAN_POINT ( 'NONE',  ( -17.81508947870519322, -18.77243306401324219, -218.1930932538018340 ) ) ;
#1378=CARTESIAN_POINT ( 'NONE',  ( -27.53108621362071773, 14.15137273650544536, -219.7961709676081625 ) ) ;
#1379=CARTESIAN_POINT ( 'NONE',  ( 8.257114973007913861, -25.39836461225790742, -232.6217252414676295 ) ) ;
#1380=CARTESIAN_POINT ( 'NONE',  ( 26.60633779560760459, -14.33430814915920593, -230.5388497754989885 ) ) ;
#1381=CARTESIAN_POINT ( 'NONE',  ( -16.76449091996730090, -6.021196472930381738, -231.5810252088758432 ) ) ;
#1383=CARTESIAN_POINT ( 'NONE',  ( 20.40268796714816801, 18.65534563792085621, -219.5587498978784993 ) ) ;
#1385=CARTESIAN_POINT ( 'NONE',  ( -21.29946384424354733, 21.01772963953914442, -222.5871995662667757 ) ) ;
#1386=CARTESIAN_POINT ( 'NONE',  ( 9.575488824002899690, 13.89846378187365694, -220.1158735840035945 ) ) ;
#1387=CARTESIAN_POINT ( 'NONE',  ( 17.43816562714825125, 15.15720016074785903, -232.3748236813696906 ) ) ;
#1388=CARTESIAN_POINT ( 'NONE',  ( 21.46274988498219471, 20.25395488059580984, -223.1777011585387243 ) ) ;
#1389=CARTESIAN_POINT ( 'NONE',  ( 10.56186985702850833, -7.684747726859879613, -229.4341029534429026 ) ) ;
#1390=CARTESIAN_POINT ( 'NONE',  ( -10.24168223636446662, 16.14271751156598356, -231.4847994864913971 ) ) ;
#1391=CARTESIAN_POINT ( 'NONE',  ( -28.99926036811508467, 3.909990568804979194, -228.9613767892386988 ) ) ;
#1394=CARTESIAN_POINT ( 'NONE',  ( 11.62313423782632782, 11.98467543564608029, -219.7293303032897995 ) ) ;
#1395=CARTESIAN_POINT ( 'NONE',  ( 5.240643865192946116, -17.54789557311951143, -217.3772572127879812 ) ) ;
#1396=CARTESIAN_POINT ( 'NONE',  ( -14.94640692938030746, 5.382918922058764544, -220.5478552936960455 ) ) ;
#1398=CARTESIAN_POINT ( 'NONE',  ( 10.25948093768852054, 28.38842464930171872, -224.3436940787075855 ) ) ;
#1399=CARTESIAN_POINT ( 'NONE',  ( -16.76449091996730090, -6.021196472930381738, -231.5810252088758432 ) ) ;
#1400=CARTESIAN_POINT ( 'NONE',  ( 12.23284375931666013, 4.108221165122169616, -224.0993108960438462 ) ) ;
#1401=CARTESIAN_POINT ( 'NONE',  ( 7.116434306140963173, 9.967665124511082553, -224.4990387090310833 ) ) ;
#1403=CARTESIAN_POINT ( 'NONE',  ( -10.84997096467605182, 25.01800101807719301, -232.4518260228253155 ) ) ;
#1404=CARTESIAN_POINT ( 'NONE',  ( 15.15335612453267089, -12.60200553607942098, -219.4566848265094166 ) ) ;
#1405=CARTESIAN_POINT ( 'NONE',  ( 28.46281617689634302, -10.50803404096709137, -222.5507679334694728 ) ) ;
#1407=CARTESIAN_POINT ( 'NONE',  ( 4.656903975822286768, 13.45000048768594780, -227.6722060245555497 ) ) ;
#1408=CARTESIAN_POINT ( 'NONE',  ( -15.80613518906033121, -10.93105391054944597, -234.9065563738643903 ) ) ;
#1409=CARTESIAN_POINT ( 'NONE',  ( 7.437838793555467731, -20.85539581353325289, -233.9154700400843865 ) ) ;
#1410=CARTESIAN_POINT ( 'NONE',  ( 11.90144651507291051, -8.898305237537579515, -228.5592478859710184 ) ) ;
#1411=CARTESIAN_POINT ( 'NONE',  ( -8.112279890008961658, 11.99566605360304727, -225.9834628568286519 ) ) ;
#1412=CARTESIAN_POINT ( 'NONE',  ( 12.91443243054181700, 13.28840485332751875, -229.6651346406987955 ) ) ;
#1413=CARTESIAN_POINT ( 'NONE',  ( -16.15126510923403202, -0.4755054218165427615, -219.3066569788202571 ) ) ;
#1414=CARTESIAN_POINT ( 'NONE',  ( -23.49520248890869212, 11.82830312093803649, -233.3871405502527807 ) ) ;
#1415=CARTESIAN_POINT ( 'NONE',  ( -18.22136682449241363, -9.036057809225649606, -231.1742889867359736 ) ) ;
#1416=ORIENTED_EDGE ( 'NONE', *, *, #4968, .F. ) ;
#1417=CARTESIAN_POINT ( 'NONE',  ( -8.435479365662203577, 14.12888021429238528, -220.5365774424437859 ) ) ;
#1418=CARTESIAN_POINT ( 'NONE',  ( 13.86383614057800884, 4.939477956453596441, -219.6543243356308324 ) ) ;
#1419=CARTESIAN_POINT ( 'NONE',  ( -3.712761995161701911, 23.50704853188985766, -216.1220552374512067 ) ) ;
#1420=CARTESIAN_POINT ( 'NONE',  ( 12.99512476935412231, -3.120572961704727977, -223.7636045402963987 ) ) ;
#1424=CARTESIAN_POINT ( 'NONE',  ( -18.70100282803782576, 16.58357028540773115, -216.4425743468854080 ) ) ;
#1425=CARTESIAN_POINT ( 'NONE',  ( -11.51027863121307782, -1.790843358437596677, -225.0773512427349203 ) ) ;
#1427=CARTESIAN_POINT ( 'NONE',  ( 12.10245006109274080, 26.02147364279441888, -220.6079829738538649 ) ) ;
#1429=CARTESIAN_POINT ( 'NONE',  ( 16.07085865561684201, -17.65509622858733252, -216.6880805489183501 ) ) ;
#1431=CARTESIAN_POINT ( 'NONE',  ( -13.10651848559790444, 3.262242204071156948, -224.3513854875720597 ) ) ;
#1432=CARTESIAN_POINT ( 'NONE',  ( -8.929606928624414408, 11.65278034267609186, -219.1999234847403386 ) ) ;
#1433=CARTESIAN_POINT ( 'NONE',  ( 13.59483335902903178, 5.678732573479117640, -228.5032236586631313 ) ) ;
#1434=CARTESIAN_POINT ( 'NONE',  ( -4.879290506874147226, -14.18937706998098136, -223.0759034783553147 ) ) ;
#1437=CARTESIAN_POINT ( 'NONE',  ( 25.18785298611088308, 3.974282393449815931, -218.7636041058819956 ) ) ;
#1438=CARTESIAN_POINT ( 'NONE',  ( 28.08231343014353243, -2.974470402155979354, -225.4253119135968291 ) ) ;
#1439=CARTESIAN_POINT ( 'NONE',  ( 14.35226977795134040, -1.892513177579410844, -227.3278729267533151 ) ) ;
#1443=CARTESIAN_POINT ( 'NONE',  ( 11.00580183749007190, 25.74996642444834904, -225.8602305833924788 ) ) ;
#1445=CARTESIAN_POINT ( 'NONE',  ( 13.14132348467506439, -13.49276336982165780, -234.5843434792288633 ) ) ;
#1446=CARTESIAN_POINT ( 'NONE',  ( 11.32394539683753720, -15.63383003174572572, -233.0723040138117881 ) ) ;
#1447=CARTESIAN_POINT ( 'NONE',  ( -17.08384421609436643, 23.56421365837046622, -225.2902702884460666 ) ) ;
#1448=CARTESIAN_POINT ( 'NONE',  ( 27.69955354773053458, 12.81264626165819287, -221.7750850138309602 ) ) ;
#1449=CARTESIAN_POINT ( 'NONE',  ( 27.66944030902029539, 6.857614156517904291, -220.9860880211026313 ) ) ;
#1450=CARTESIAN_POINT ( 'NONE',  ( -8.696851061449722309, -24.60219662023354914, -220.1357990587600852 ) ) ;
#1452=CARTESIAN_POINT ( 'NONE',  ( -27.53108621362071773, 14.15137273650544536, -219.7961709676081625 ) ) ;
#1453=CARTESIAN_POINT ( 'NONE',  ( 3.714886539878811789, 12.88803176524806560, -219.5889136906770034 ) ) ;
#1454=CARTESIAN_POINT ( 'NONE',  ( 13.51502823286059929, -13.46037062290453790, -230.3041566501836144 ) ) ;
#1455=CARTESIAN_POINT ( 'NONE',  ( 9.586902571418640662, 24.43292817174309661, -231.9968623198229807 ) ) ;
#1456=CARTESIAN_POINT ( 'NONE',  ( -13.98136146596813845, 3.850743984385103680, -228.7620665878280590 ) ) ;
#1457=CARTESIAN_POINT ( 'NONE',  ( 13.79814099039094089, 16.09927043668092850, -214.6489469124405502 ) ) ;
#1458=CARTESIAN_POINT ( 'NONE',  ( -16.48591407464216729, 7.092323989942422635, -218.8909951703408012 ) ) ;
#1459=CARTESIAN_POINT ( 'NONE',  ( -6.474151797443945533, 21.29193859232740138, -215.9573456447696458 ) ) ;
#1460=CARTESIAN_POINT ( 'NONE',  ( 24.03642272140365677, 3.646960756862087205, -218.2320643939070806 ) ) ;
#1461=CARTESIAN_POINT ( 'NONE',  ( 8.686008240521225332, 26.11221116136006515, -227.6539570933143466 ) ) ;
#1462=CARTESIAN_POINT ( 'NONE',  ( 27.96460686140487084, -1.872811165202790340, -220.9791906660856000 ) ) ;
#1465=CARTESIAN_POINT ( 'NONE',  ( -31.04415783139704388, 5.868882651865275690, -221.1472518903637194 ) ) ;
#1466=CARTESIAN_POINT ( 'NONE',  ( -13.98007945013786291, -9.257046693524761949, -228.3752161438062842 ) ) ;
#1468=CARTESIAN_POINT ( 'NONE',  ( -14.94618804342693075, 22.09718979644185666, -219.6454806548149463 ) ) ;
#1470=CARTESIAN_POINT ( 'NONE',  ( 2.283233934795953601, -16.37150177406293849, -220.5471140349473842 ) ) ;
#1471=CARTESIAN_POINT ( 'NONE',  ( 12.54860906168727652, 6.077542143275485031, -228.1605930327268368 ) ) ;
#1472=CARTESIAN_POINT ( 'NONE',  ( -8.857704405076667342, 24.20848540845601704, -218.8859504303524091 ) ) ;
#1473=CARTESIAN_POINT ( 'NONE',  ( -23.66836017558062011, 21.44695383684080525, -223.6245772351065568 ) ) ;
#1475=CARTESIAN_POINT ( 'NONE',  ( 24.13177372007769961, -1.862525787088729956, -215.1116454360890202 ) ) ;
#1477=CARTESIAN_POINT ( 'NONE',  ( 12.58590500897257947, 11.38573988265384607, -230.4867078522624695 ) ) ;
#1478=CARTESIAN_POINT ( 'NONE',  ( -17.00265675087485917, 7.324244386240115645, -218.5600005870616656 ) ) ;
#1479=CARTESIAN_POINT ( 'NONE',  ( -21.93223149637851677, 1.726402211042445067, -231.1052103444381203 ) ) ;
#1481=CARTESIAN_POINT ( 'NONE',  ( -29.73963803141277396, -7.146848409970624871, -220.9878827551818858 ) ) ;
#1482=CARTESIAN_POINT ( 'NONE',  ( 16.64575860537911112, 25.12688477742292648, -227.5050599151411745 ) ) ;
#1483=CARTESIAN_POINT ( 'NONE',  ( -15.99768154740552717, 2.245235659047613908, -226.7015216759272107 ) ) ;
#1484=CARTESIAN_POINT ( 'NONE',  ( -2.917590128672695293, 18.81591489065672818, -216.3635620530855022 ) ) ;
#1485=CARTESIAN_POINT ( 'NONE',  ( 27.08994772491946890, 9.675875910685000747, -221.3471992134593336 ) ) ;
#1486=CARTESIAN_POINT ( 'NONE',  ( -7.253640667752737414, -12.78251829042625687, -230.3353663933772282 ) ) ;
#1488=CARTESIAN_POINT ( 'NONE',  ( -10.22552941266963877, -9.699191453761107695, -225.4315674810442545 ) ) ;
#1489=CARTESIAN_POINT ( 'NONE',  ( -28.88770769694534479, 14.24820799418726480, -223.2044777450442155 ) ) ;
#1490=CARTESIAN_POINT ( 'NONE',  ( 4.201723131641114328, -20.76291977712905279, -215.9522215885928347 ) ) ;
#1491=CARTESIAN_POINT ( 'NONE',  ( -2.208416658185406334, 29.10348627872611615, -219.8480645685746424 ) ) ;
#1492=CARTESIAN_POINT ( 'NONE',  ( 14.87770435525805013, -9.987123395515542512, -215.8225415630120665 ) ) ;
#1493=CARTESIAN_POINT ( 'NONE',  ( -20.18470553695442860, -13.13924840112635195, -232.9662461559857718 ) ) ;
#1494=CARTESIAN_POINT ( 'NONE',  ( 16.82251835652528982, 18.18719385133374544, -231.8032941011735772 ) ) ;
#1495=CARTESIAN_POINT ( 'NONE',  ( -10.46043650402819125, 8.998596506756641134, -222.4402691847174083 ) ) ;
#1496=CARTESIAN_POINT ( 'NONE',  ( 8.778334628954494789, 12.71782457734010841, -222.1923057070808909 ) ) ;
#1498=CARTESIAN_POINT ( 'NONE',  ( 14.39473142419577023, 15.98257177912839389, -217.4557725731239373 ) ) ;
#1499=CARTESIAN_POINT ( 'NONE',  ( 9.094331215210646135, 23.85463374792894342, -219.7669638091879847 ) ) ;
#1500=CARTESIAN_POINT ( 'NONE',  ( 5.982199551433209805, -30.67818700677413091, -221.2919386232889849 ) ) ;
#1501=CARTESIAN_POINT ( 'NONE',  ( -13.06839468023815165, 25.32320678245788059, -229.0099538679170053 ) ) ;
#1506=CARTESIAN_POINT ( 'NONE',  ( 8.990474075060864934, -28.03008174514034678, -221.5310560963409330 ) ) ;
#1507=CARTESIAN_POINT ( 'NONE',  ( -23.20103936322198024, 10.64725167743880085, -231.7714206262400864 ) ) ;
#1508=CARTESIAN_POINT ( 'NONE',  ( -1.038524475621362075, 14.89017051181998141, -222.3948816610352139 ) ) ;
#1510=CARTESIAN_POINT ( 'NONE',  ( -24.15031621174628285, -13.05338392360020627, -219.0842748323915714 ) ) ;
#1511=CARTESIAN_POINT ( 'NONE',  ( -17.29038495093124084, 2.707785585324113065, -229.0475017805649998 ) ) ;
#1513=CARTESIAN_POINT ( 'NONE',  ( 13.06625079052675531, 10.14096931681969238, -232.1435240729728093 ) ) ;
#1515=CARTESIAN_POINT ( 'NONE',  ( -7.825349071214003693, 24.14595706726266755, -216.5959661901539732 ) ) ;
#1516=CARTESIAN_POINT ( 'NONE',  ( 11.99204520814221553, -11.76515119196726467, -228.0494177468141572 ) ) ;
#1517=CARTESIAN_POINT ( 'NONE',  ( 20.33239098169031323, -9.013719117183370599, -216.4483480702011775 ) ) ;
#1519=CARTESIAN_POINT ( 'NONE',  ( 4.354034006296288339, 14.09944204372416188, -221.2519525881239417 ) ) ;
#1520=CARTESIAN_POINT ( 'NONE',  ( -10.37549270978917448, -7.969494006339708392, -220.1790165754723603 ) ) ;
#1521=CARTESIAN_POINT ( 'NONE',  ( -14.34280792637948743, -22.10828917559366147, -217.4172704053049756 ) ) ;
#1522=CARTESIAN_POINT ( 'NONE',  ( 12.73130673999417795, -23.76414828096303467, -217.7386337832039942 ) ) ;
#1523=CARTESIAN_POINT ( 'NONE',  ( -11.11479000491124047, 20.76372272540567110, -218.2001872134434564 ) ) ;
#1524=CARTESIAN_POINT ( 'NONE',  ( 7.951191770265756631, 20.55701948568933091, -231.2149185317973661 ) ) ;
#1525=CARTESIAN_POINT ( 'NONE',  ( -21.02719846458807851, 18.12262440796364871, -218.0220709499931502 ) ) ;
#1526=CARTESIAN_POINT ( 'NONE',  ( -24.69837543585720141, 12.57569301576483589, -232.4521327773205428 ) ) ;
#1527=CARTESIAN_POINT ( 'NONE',  ( -24.95561420934758701, -9.148537957313763513, -219.7769960911953149 ) ) ;
#1530=CARTESIAN_POINT ( 'NONE',  ( -8.317278876689359279, 23.15034512777772235, -218.2935523245793092 ) ) ;
#1531=CARTESIAN_POINT ( 'NONE',  ( 16.21758812354607215, 4.665393561625732488, -232.5634757513959983 ) ) ;
#1532=CARTESIAN_POINT ( 'NONE',  ( 5.964915545484365644, 11.50358694729900577, -229.9646467236423462 ) ) ;
#1533=CARTESIAN_POINT ( 'NONE',  ( 21.28562020585086501, -15.94148943779260819, -218.1725164024425396 ) ) ;
#1536=CARTESIAN_POINT ( 'NONE',  ( -15.20262116893801974, 8.038155052917188570, -217.6767387945475036 ) ) ;
#1537=CARTESIAN_POINT ( 'NONE',  ( -17.92393051735373888, -14.45097846726422830, -234.9711082062119374 ) ) ;
#1539=CARTESIAN_POINT ( 'NONE',  ( 5.069241901512100412, 14.34986542013820632, -229.6420000777802954 ) ) ;
#1541=CARTESIAN_POINT ( 'NONE',  ( 11.90144651507291051, -8.898305237537579515, -228.5592478859710184 ) ) ;
#1542=CARTESIAN_POINT ( 'NONE',  ( -25.29098058636142810, 5.014641116111857144, -217.4658967307323110 ) ) ;
#1545=CARTESIAN_POINT ( 'NONE',  ( 21.14328650935969023, 6.072767611243683916, -217.6422864096696514 ) ) ;
#1546=SHAPE_REPRESENTATION ( 'Frothing Whisk', ( #6677 ), #13476 ) ;
#1547=CARTESIAN_POINT ( 'NONE',  ( -5.534391910549205207, -14.54353160188980709, -228.1022699408985943 ) ) ;
#1550=CARTESIAN_POINT ( 'NONE',  ( 18.54610009393809023, 0.6523581019769808531, -231.1787333216317677 ) ) ;
#1552=CARTESIAN_POINT ( 'NONE',  ( 11.40994021191102092, -13.94644022156852969, -230.1289083636806936 ) ) ;
#1553=CARTESIAN_POINT ( 'NONE',  ( 12.99467735515414191, -2.323045947487815788, -223.0925300893006238 ) ) ;
#1556=CARTESIAN_POINT ( 'NONE',  ( 14.66646255503707152, 18.43809875292740230, -219.3480462970252063 ) ) ;
#1557=CARTESIAN_POINT ( 'NONE',  ( 8.539351012053531420, 16.03230746435535181, -220.6282946404833751 ) ) ;
#1558=CARTESIAN_POINT ( 'NONE',  ( 22.27668549480667792, -16.40903445915953895, -216.4638184065479152 ) ) ;
#1559=CARTESIAN_POINT ( 'NONE',  ( 9.104026917753444081, -10.66572815660443041, -221.9193219976906448 ) ) ;
#1561=CARTESIAN_POINT ( 'NONE',  ( -8.435479365662203577, 14.12888021429238528, -220.5365774424437859 ) ) ;
#1562=CARTESIAN_POINT ( 'NONE',  ( -17.55809605150417951, 6.636094600389130349, -229.8856864643722986 ) ) ;
#1563=CARTESIAN_POINT ( 'NONE',  ( 21.15841376125116824, 4.865517895153391947, -217.1795922978051578 ) ) ;
#1565=CARTESIAN_POINT ( 'NONE',  ( -5.427686778165598191, -19.74436295060356272, -231.6150980610854901 ) ) ;
#1568=CARTESIAN_POINT ( 'NONE',  ( -11.89542918462869103, -0.2773029175206048191, -224.4556830488584467 ) ) ;
#1569=ORIENTED_EDGE ( 'NONE', *, *, #7048, .T. ) ;
#1571=CARTESIAN_POINT ( 'NONE',  ( 19.97628502126439187, 24.50819884991013708, -224.8824979922784735 ) ) ;
#1572=CARTESIAN_POINT ( 'NONE',  ( 12.63976474005154493, -11.16289257830726278, -221.8494566150397134 ) ) ;
#1574=CARTESIAN_POINT ( 'NONE',  ( 9.107417252317809186, 16.30291009569977234, -218.0131178633739921 ) ) ;
#1575=CARTESIAN_POINT ( 'NONE',  ( -16.71711190488355570, 0.6105529133557690002, -230.9511258789794681 ) ) ;
#1576=CARTESIAN_POINT ( 'NONE',  ( 11.50837930502119733, 10.86662242793286381, -233.1728506169798436 ) ) ;
#1577=CARTESIAN_POINT ( 'NONE',  ( -22.14646582578067679, 6.967411055428133437, -231.6932229095398270 ) ) ;
#1578=CARTESIAN_POINT ( 'NONE',  ( -11.26857159993117996, 28.96895336474501192, -225.6039696848669678 ) ) ;
#1579=DIRECTION ( 'NONE',  ( 0.03647168421188083653, 0.3315607655626302552, 0.9427286327412950362 ) ) ;
#1580=CARTESIAN_POINT ( 'NONE',  ( 5.609436632608550966, -13.11664087352601094, -229.3324225951633650 ) ) ;
#1581=CARTESIAN_POINT ( 'NONE',  ( 14.62702828724412285, -1.994068170757606673, -224.0552340365271959 ) ) ;
#1583=CARTESIAN_POINT ( 'NONE',  ( -15.89118508636071958, -1.798691612803976492, -229.3605869667087234 ) ) ;
#1584=CARTESIAN_POINT ( 'NONE',  ( 16.64225601860865211, 1.926018578292457928, -220.2177910260893725 ) ) ;
#1585=CARTESIAN_POINT ( 'NONE',  ( -10.37556110177195023, -11.10057404503678846, -224.0577835142470349 ) ) ;
#1588=CARTESIAN_POINT ( 'NONE',  ( 11.64632602964496044, -20.35392056169815689, -232.5450580586399383 ) ) ;
#1589=CARTESIAN_POINT ( 'NONE',  ( -18.14952719657095415, 1.368063294522122275, -218.0005379682515922 ) ) ;
#1590=CARTESIAN_POINT ( 'NONE',  ( -8.611121136347097860, 17.46802294375265419, -231.5575697815534113 ) ) ;
#1591=CARTESIAN_POINT ( 'NONE',  ( -7.626320092023432196, 21.25423560278784407, -233.8867968595558295 ) ) ;
#1592=CARTESIAN_POINT ( 'NONE',  ( 12.55122320111375700, -1.519965464208375749, -221.0350040576933281 ) ) ;
#1593=CARTESIAN_POINT ( 'NONE',  ( 12.04687593227112430, 27.54339840196571743, -224.6466266724203820 ) ) ;
#1594=CARTESIAN_POINT ( 'NONE',  ( -24.19163806436329978, 8.131440952769249719, -230.9341214615949127 ) ) ;
#1595=CARTESIAN_POINT ( 'NONE',  ( 17.98589043827631428, 2.945998030785370592, -233.4030907785035538 ) ) ;
#1597=DIRECTION ( 'NONE',  ( 1.000000000000000000, 0.000000000000000000, 0.000000000000000000 ) ) ;
#1598=CARTESIAN_POINT ( 'NONE',  ( 9.774133712851615030, 11.09751083462123766, -229.6876724410067823 ) ) ;
#1600=CARTESIAN_POINT ( 'NONE',  ( -18.90911063232017142, 5.352531560950812839, -219.6301177803536575 ) ) ;
#1601=CARTESIAN_POINT ( 'NONE',  ( 2.631948090663005946, 31.21493676147814611, -222.3107766067421380 ) ) ;
#1602=CARTESIAN_POINT ( 'NONE',  ( 11.75630001506626776, 9.075791953625659048, -230.4239556728226717 ) ) ;
#1603=CARTESIAN_POINT ( 'NONE',  ( -13.04380155829002419, -28.08004287256819609, -224.7912146079995352 ) ) ;
#1605=CARTESIAN_POINT ( 'NONE',  ( -5.218961787268129093, -16.18493974670746027, -219.8229902141834771 ) ) ;
#1606=CARTESIAN_POINT ( 'NONE',  ( -12.19796877179171446, 17.24929682309303658, -234.5722138766719809 ) ) ;
#1607=CARTESIAN_POINT ( 'NONE',  ( 2.098184199980985376, -13.29281380427311099, -222.1652846463370281 ) ) ;
#1608=CARTESIAN_POINT ( 'NONE',  ( -2.808235066048971440, 30.42019778760651150, -222.6481917607299295 ) ) ;
#1609=CARTESIAN_POINT ( 'NONE',  ( 13.04627209130898002, -4.074791396861574988, -220.3858784301183675 ) ) ;
#1610=CARTESIAN_POINT ( 'NONE',  ( -24.92024473536680773, -13.74570206812420103, -220.1598944320903115 ) ) ;
#1611=CARTESIAN_POINT ( 'NONE',  ( 12.63974878616558328, 15.03448928898568759, -231.7036488814491406 ) ) ;
#1613=CARTESIAN_POINT ( 'NONE',  ( -27.17783334270200157, 15.20409188923851751, -223.6555185980277258 ) ) ;
#1614=CARTESIAN_POINT ( 'NONE',  ( 16.43556216695724004, 8.397919695511960825, -216.7971521583719152 ) ) ;
#1616=CARTESIAN_POINT ( 'NONE',  ( 22.02796522526679723, 16.41909032291435366, -220.1590600991317217 ) ) ;
#1617=CARTESIAN_POINT ( 'NONE',  ( 15.56183105618911355, 23.93598532278018354, -223.2746693648072664 ) ) ;
#1618=CARTESIAN_POINT ( 'NONE',  ( 4.956111054478943068, -16.91316901532391270, -234.1076498343193748 ) ) ;
#1619=CARTESIAN_POINT ( 'NONE',  ( -11.10144104376680652, 18.49675466419975578, -232.2931259015917647 ) ) ;
#1620=ADVANCED_FACE ( 'NONE', ( #14536 ), #3699, .F. ) ;
#1621=CARTESIAN_POINT ( 'NONE',  ( 19.20300624114736721, 0.6066039755357417462, -231.5046416827383950 ) ) ;
#1622=CARTESIAN_POINT ( 'NONE',  ( 7.717439423011566824, -15.08909893080012132, -230.2794769249191518 ) ) ;
#1623=CARTESIAN_POINT ( 'NONE',  ( -13.70798801564395752, 13.71024986321384809, -218.3360451569033955 ) ) ;
#1624=CARTESIAN_POINT ( 'NONE',  ( -2.435715273212520238, 23.41098772907853132, -217.6796576669356966 ) ) ;
#1625=CARTESIAN_POINT ( 'NONE',  ( -25.82802808205240552, -14.78441951539553401, -222.6940535085979604 ) ) ;
#1626=CARTESIAN_POINT ( 'NONE',  ( 18.40125535140034430, 0.01434342441762339639, -233.2485400239426099 ) ) ;
#1628=CARTESIAN_POINT ( 'NONE',  ( 11.00045714400293306, 20.20239058357963913, -215.1666500215986275 ) ) ;
#1630=CARTESIAN_POINT ( 'NONE',  ( 12.10245006109274080, 26.02147364279441888, -220.6079829738538649 ) ) ;
#1631=CARTESIAN_POINT ( 'NONE',  ( 23.53402537799887284, -10.66620622184993650, -219.3119847637072439 ) ) ;
#1632=AXIS2_PLACEMENT_3D ( 'NONE', #2945, #9501, #9832 ) ;
#1633=CARTESIAN_POINT ( 'NONE',  ( 22.55746627616819566, -14.21542447219996852, -231.9819121152456205 ) ) ;
#1635=CARTESIAN_POINT ( 'NONE',  ( 0.7245137624042983227, 13.44764381486384330, -223.4043886706536455 ) ) ;
#1636=CARTESIAN_POINT ( 'NONE',  ( -10.91546170668013005, -7.896971223757457636, -230.5866998909293102 ) ) ;
#1637=CARTESIAN_POINT ( 'NONE',  ( -10.11868820210310282, -13.51996935893276053, -218.1704188629865371 ) ) ;
#1638=CARTESIAN_POINT ( 'NONE',  ( 6.741123954526870854, -14.00899218320067341, -219.0418835583997179 ) ) ;
#1639=CARTESIAN_POINT ( 'NONE',  ( -8.791002657293931932, 17.82034842365333205, -218.5247019341474584 ) ) ;
#1640=CARTESIAN_POINT ( 'NONE',  ( 8.250760074138732136, 14.96691001493985951, -221.7548416114337613 ) ) ;
#1641=CARTESIAN_POINT ( 'NONE',  ( -17.79285498209129202, 9.187865686019035749, -216.3798185811636756 ) ) ;
#1642=CARTESIAN_POINT ( 'NONE',  ( -31.12406087576577463, 7.316399946619934092, -225.0171288978685027 ) ) ;
#1643=CARTESIAN_POINT ( 'NONE',  ( -15.15256618962804858, -12.22297499669621423, -230.3735341043967821 ) ) ;
#1645=CARTESIAN_POINT ( 'NONE',  ( -4.784012432433236484, 23.31984772163034947, -232.0554186943449508 ) ) ;
#1647=CARTESIAN_POINT ( 'NONE',  ( 14.33191776452776622, 5.147404080619256916, -219.0172570056664938 ) ) ;
#1648=CARTESIAN_POINT ( 'NONE',  ( 24.61409543538958289, 19.88121288930873476, -228.5015986536257344 ) ) ;
#1649=CARTESIAN_POINT ( 'NONE',  ( 12.90474009670415967, -3.145873754258878385, -224.5449843457338375 ) ) ;
#1653=CARTESIAN_POINT ( 'NONE',  ( -7.429838964355703901, 14.87322129099639234, -232.2632863647814077 ) ) ;
#1654=CARTESIAN_POINT ( 'NONE',  ( -23.48355816166749932, -5.921172941748132246, -214.8630305010649408 ) ) ;
#1656=CARTESIAN_POINT ( 'NONE',  ( 25.33562512631297281, 12.25422971834577268, -228.6777356031426791 ) ) ;
#1657=CARTESIAN_POINT ( 'NONE',  ( -20.26851768784797869, -0.8260594303982465858, -217.1279713726092098 ) ) ;
#1658=CARTESIAN_POINT ( 'NONE',  ( 10.24538335401965661, -11.82980241027587276, -219.3753974371782363 ) ) ;
#1659=CARTESIAN_POINT ( 'NONE',  ( -18.08305592660031991, 4.022743421239192152, -217.2335041149100050 ) ) ;
#1660=CARTESIAN_POINT ( 'NONE',  ( 14.68015846516680867, 2.651775288685355836, -224.1317433549420173 ) ) ;
#1661=CARTESIAN_POINT ( 'NONE',  ( -6.454554286546707154, -27.99704349260872149, -227.4356265632874852 ) ) ;
#1663=CARTESIAN_POINT ( 'NONE',  ( 24.03642272140365677, 3.646960756862087205, -218.2320643939070806 ) ) ;
#1665=CARTESIAN_POINT ( 'NONE',  ( 14.47405021949252557, -20.16114635186222159, -231.2055612633458566 ) ) ;
#1669=CARTESIAN_POINT ( 'NONE',  ( 9.280831573919673616, 14.67893982993557422, -228.6940810986570796 ) ) ;
#1670=CARTESIAN_POINT ( 'NONE',  ( 8.312165662451315384, 13.84431584962456974, -225.8109542921768025 ) ) ;
#1671=CARTESIAN_POINT ( 'NONE',  ( 20.62543286083822380, -24.26207512693059343, -224.4080524747341201 ) ) ;
#1672=CARTESIAN_POINT ( 'NONE',  ( 15.34510829589250491, -24.56813251781886009, -230.1307231235174982 ) ) ;
#1675=CARTESIAN_POINT ( 'NONE',  ( -22.07068341299880743, 18.38202870573248049, -227.7785760498121306 ) ) ;
#1676=CARTESIAN_POINT ( 'NONE',  ( -17.99155049254074612, 5.190958499132906745, -220.1449419322306937 ) ) ;
#1677=CARTESIAN_POINT ( 'NONE',  ( 15.70179827786738969, 6.572001003133339125, -229.5476218741844434 ) ) ;
#1679=CARTESIAN_POINT ( 'NONE',  ( -14.02781974392415165, -24.18658813864446344, -225.1634145543362706 ) ) ;
#1682=CARTESIAN_POINT ( 'NONE',  ( 15.18181359483165949, 6.369295616116027681, -230.7949408486033462 ) ) ;
#1683=CARTESIAN_POINT ( 'NONE',  ( 15.70595326690115634, -18.65841243762358559, -219.6423885132037981 ) ) ;
#1684=CARTESIAN_POINT ( 'NONE',  ( 15.12287735332712835, 21.03907941686458116, -231.7894952627153202 ) ) ;
#1685=CARTESIAN_POINT ( 'NONE',  ( -6.282398543089500187, 12.01615879894893801, -228.5121145169883903 ) ) ;
#1687=CARTESIAN_POINT ( 'NONE',  ( 6.550054208186137039, 12.38618022562281595, -231.5087189857719068 ) ) ;
#1688=CARTESIAN_POINT ( 'NONE',  ( -10.83439284573031536, 18.36737820296253432, -234.3014274143859836 ) ) ;
#1689=CARTESIAN_POINT ( 'NONE',  ( -8.823862513872974489, 14.92351368520778898, -217.1499513473673346 ) ) ;
#1691=CARTESIAN_POINT ( 'NONE',  ( -3.300598509645395584, -18.18730530649546395, -233.4303386612170925 ) ) ;
#1695=CARTESIAN_POINT ( 'NONE',  ( -29.27492217116574480, -1.185422171198730501, -224.8132346143397342 ) ) ;
#1696=CARTESIAN_POINT ( 'NONE',  ( 22.18132842682159733, 5.591149267797686839, -232.0584733989884114 ) ) ;
#1697=CARTESIAN_POINT ( 'NONE',  ( -14.57915343259292307, -9.548365625374035659, -229.2620333697842057 ) ) ;
#1698=CARTESIAN_POINT ( 'NONE',  ( 9.759123193367146953, -21.89695672029116480, -217.8292787338521919 ) ) ;
#1699=CARTESIAN_POINT ( 'NONE',  ( -21.43408368508570305, 3.680162304907783621, -233.1134812316964542 ) ) ;
#1700=CARTESIAN_POINT ( 'NONE',  ( -0.9249541874382023465, 14.55235618511626328, -223.7321818898853962 ) ) ;
#1701=CARTESIAN_POINT ( 'NONE',  ( -6.702936938788568888, 25.88675107068059944, -218.1129661040884287 ) ) ;
#1702=CARTESIAN_POINT ( 'NONE',  ( 11.91821674756695693, -1.593691010653677242, -227.2895864140137405 ) ) ;
#1704=CARTESIAN_POINT ( 'NONE',  ( 14.39473142419577023, 15.98257177912839389, -217.4557725731239373 ) ) ;
#1705=CARTESIAN_POINT ( 'NONE',  ( -19.27153818831731158, 23.75761453444584248, -221.9111479746408975 ) ) ;
#1706=CARTESIAN_POINT ( 'NONE',  ( -11.59479561055411345, 9.544396733298208702, -229.1494558965577255 ) ) ;
#1707=CARTESIAN_POINT ( 'NONE',  ( -10.39692419770002552, -10.11462123336039021, -222.6538761800393047 ) ) ;
#1709=CARTESIAN_POINT ( 'NONE',  ( 12.81769551943392393, 4.437328497131001193, -221.7762769673541072 ) ) ;
#1710=CARTESIAN_POINT ( 'NONE',  ( -20.41147829968989313, 3.432784889297933795, -230.9611049257633510 ) ) ;
#1711=CARTESIAN_POINT ( 'NONE',  ( 13.12946830070648652, 6.370976456471619365, -231.5124810213676483 ) ) ;
#1712=CARTESIAN_POINT ( 'NONE',  ( 15.28706223449149348, 2.473424253736659306, -227.9634568993954531 ) ) ;
#1713=CARTESIAN_POINT ( 'NONE',  ( -9.698809215651296611, -24.51491891025427350, -232.5150754403024962 ) ) ;
#1715=CARTESIAN_POINT ( 'NONE',  ( -10.94940667656068634, -10.80050631132953498, -220.7362776234490127 ) ) ;
#1717=CARTESIAN_POINT ( 'NONE',  ( -18.07648963816576781, 14.36622924931724654, -235.1425738388569187 ) ) ;
#1718=CARTESIAN_POINT ( 'NONE',  ( 11.32394539683753720, -15.63383003174572572, -233.0723040138117881 ) ) ;
#1719=CARTESIAN_POINT ( 'NONE',  ( -10.45786516112131892, 23.61456281964591852, -233.2869923610001592 ) ) ;
#1720=CARTESIAN_POINT ( 'NONE',  ( 29.08354724566992644, -8.084875104304042992, -220.4391609833976133 ) ) ;
#1721=CARTESIAN_POINT ( 'NONE',  ( -16.64477864544768337, -2.947896226079009807, -219.6737919733007516 ) ) ;
#1723=CARTESIAN_POINT ( 'NONE',  ( 26.75666476377482539, 8.100664119735744961, -232.1611550320539834 ) ) ;
#1725=CARTESIAN_POINT ( 'NONE',  ( -6.573387563318148885, 17.69612765735440973, -231.1211991061559274 ) ) ;
#1726=CARTESIAN_POINT ( 'NONE',  ( 12.43753614017300713, 2.441361880258234862, -222.2750447601761721 ) ) ;
#1727=CARTESIAN_POINT ( 'NONE',  ( 10.78187269046063435, 10.73871010366167944, -221.9206544238666368 ) ) ;
#1728=CARTESIAN_POINT ( 'NONE',  ( 28.53243699394185384, 6.329221954355706004, -218.6437889135959267 ) ) ;
#1729=CARTESIAN_POINT ( 'NONE',  ( -3.300732473188277005, -24.68991359470437175, -216.3853901891898488 ) ) ;
#1730=CARTESIAN_POINT ( 'NONE',  ( 2.291262277241625345, 17.20278591336981222, -216.2185160402476924 ) ) ;
#1732=CARTESIAN_POINT ( 'NONE',  ( 2.478093603766003294, -30.50979708220057063, -227.6059245187310012 ) ) ;
#1733=CARTESIAN_POINT ( 'NONE',  ( -24.79507334250576278, 6.844873424762779379, -218.1074956078844878 ) ) ;
#1734=CARTESIAN_POINT ( 'NONE',  ( -2.692720963948733282, 24.67937284847025481, -218.0912907784291406 ) ) ;
#1735=CARTESIAN_POINT ( 'NONE',  ( -12.13177435108894642, -8.392035797555511323, -228.8392847287196332 ) ) ;
#1736=CARTESIAN_POINT ( 'NONE',  ( 26.91963614581376874, 6.107751173605064920, -232.2246916053503298 ) ) ;
#1738=CARTESIAN_POINT ( 'NONE',  ( 18.69149182921226782, 24.00661454656289706, -229.8257469855424517 ) ) ;
#1739=CARTESIAN_POINT ( 'NONE',  ( 7.168644370073567806, 19.32044210858112265, -233.1278450877711634 ) ) ;
#1740=CARTESIAN_POINT ( 'NONE',  ( 13.95302107590712737, -11.87212821339389812, -220.3052895324516385 ) ) ;
#1741=CARTESIAN_POINT ( 'NONE',  ( 10.05733608402134216, -9.620616164199983444, -224.9449885650552119 ) ) ;
#1743=CARTESIAN_POINT ( 'NONE',  ( 11.57669841200422134, 10.63052136557218574, -228.9489978335593889 ) ) ;
#1744=CARTESIAN_POINT ( 'NONE',  ( -13.68978490692228256, -5.239663260684684687, -218.7416303080107411 ) ) ;
#1745=CARTESIAN_POINT ( 'NONE',  ( -15.62091161899253855, -26.00636881980398840, -222.1463585103649905 ) ) ;
#1746=CARTESIAN_POINT ( 'NONE',  ( 12.02378739738799140, -16.98783239109716092, -233.4545636224233931 ) ) ;
#1747=CARTESIAN_POINT ( 'NONE',  ( -13.44241955326339166, 15.88952131657459965, -217.2587743382015901 ) ) ;
#1748=CARTESIAN_POINT ( 'NONE',  ( 19.59567110982616001, 18.11097967140601028, -228.7314497914969706 ) ) ;
#1749=CARTESIAN_POINT ( 'NONE',  ( -14.83974801774860630, 13.71714848582103485, -216.0935642439352762 ) ) ;
#1750=CARTESIAN_POINT ( 'NONE',  ( -15.57505478537380306, 24.84242291948262249, -225.5907943047649837 ) ) ;
#1751=CARTESIAN_POINT ( 'NONE',  ( 20.33239098169031323, -9.013719117183370599, -216.4483480702011775 ) ) ;
#1752=CARTESIAN_POINT ( 'NONE',  ( -4.142636420702924482, 14.17169704882741321, -225.1666440184957310 ) ) ;
#1753=CARTESIAN_POINT ( 'NONE',  ( 26.91963614581376874, 6.107751173605064920, -232.2246916053503298 ) ) ;
#1754=CARTESIAN_POINT ( 'NONE',  ( 14.75291830987536557, 13.43762972591284033, -235.1407057970265839 ) ) ;
#1756=CARTESIAN_POINT ( 'NONE',  ( 16.18295504345472580, -4.390854861972272261, -232.0514848646187716 ) ) ;
#1759=CARTESIAN_POINT ( 'NONE',  ( 0.6364901924797052857, 13.89978473517355617, -221.8840706290426397 ) ) ;
#1760=CARTESIAN_POINT ( 'NONE',  ( -11.66037817688884992, -1.871521667041048609, -223.1840616512448037 ) ) ;
#1762=CARTESIAN_POINT ( 'NONE',  ( 13.49011766416699842, 7.659170998773840111, -228.1905628957712793 ) ) ;
#1763=CARTESIAN_POINT ( 'NONE',  ( -13.10651848559790444, 3.262242204071156948, -224.3513854875720597 ) ) ;
#1764=CARTESIAN_POINT ( 'NONE',  ( 11.78320976064766690, -8.193118641535518165, -222.2581747538435479 ) ) ;
#1765=CARTESIAN_POINT ( 'NONE',  ( -18.46722752239034193, 0.9784074152395518809, -232.1633353206286188 ) ) ;
#1766=CARTESIAN_POINT ( 'NONE',  ( -22.11084984981285118, 10.96048252433489623, -216.6117774006995376 ) ) ;
#1767=CARTESIAN_POINT ( 'NONE',  ( 0.4703770282364683197, -28.19050476347214484, -228.5103440588500519 ) ) ;
#1770=CARTESIAN_POINT ( 'NONE',  ( -28.17543631911187063, 3.557555778861649642, -230.1980773687482156 ) ) ;
#1771=CARTESIAN_POINT ( 'NONE',  ( 12.91525526572063853, -9.549346049255611035, -226.1928206613168584 ) ) ;
#1772=CARTESIAN_POINT ( 'NONE',  ( 13.19509313252292060, -2.019678201665313644, -222.7800808301278437 ) ) ;
#1774=CARTESIAN_POINT ( 'NONE',  ( 12.16813927252146144, 18.27141895336136912, -230.9123895730235745 ) ) ;
#1775=CARTESIAN_POINT ( 'NONE',  ( 1.719513778997906694, 15.52930330544231730, -222.3959083836286368 ) ) ;
#1776=CARTESIAN_POINT ( 'NONE',  ( -4.358491045216396742, -15.83376542237952300, -229.0450454480885583 ) ) ;
#1777=CARTESIAN_POINT ( 'NONE',  ( 19.06435866915521515, -20.24829071055443563, -218.8318535520223804 ) ) ;
#1778=CARTESIAN_POINT ( 'NONE',  ( -13.88743542672353826, 10.36310385030668613, -230.6144170796622745 ) ) ;
#1779=CARTESIAN_POINT ( 'NONE',  ( -23.77327857871830830, 11.53128597905896768, -221.0855018166512025 ) ) ;
#1780=CARTESIAN_POINT ( 'NONE',  ( -15.64716994811699813, 6.210654946517923491, -217.0002936794128345 ) ) ;
#1781=CARTESIAN_POINT ( 'NONE',  ( -7.589660848220153078, -14.86992855705293692, -228.0480809167547136 ) ) ;
#1784=CARTESIAN_POINT ( 'NONE',  ( 15.33651282626308010, 7.807290788239344970, -218.6940806506825652 ) ) ;
#1785=CARTESIAN_POINT ( 'NONE',  ( 13.59384321027942910, -22.95766697980085169, -228.5239052398278830 ) ) ;
#1786=CARTESIAN_POINT ( 'NONE',  ( 17.19674704922021391, 23.07334190050143974, -228.8256488842130238 ) ) ;
#1787=CARTESIAN_POINT ( 'NONE',  ( -7.913358619554302642, 16.16796202616373890, -233.0981776325470491 ) ) ;
#1788=CARTESIAN_POINT ( 'NONE',  ( 14.17826651990317188, -1.167225063855702683, -222.4240311848849387 ) ) ;
#1789=CARTESIAN_POINT ( 'NONE',  ( 0.7245137624042983227, 13.44764381486384330, -223.4043886706536455 ) ) ;
#1791=CARTESIAN_POINT ( 'NONE',  ( 1.729916699924999746, -18.64927252049523432, -233.5000329212076906 ) ) ;
#1792=CARTESIAN_POINT ( 'NONE',  ( 13.96958060839473958, -9.488587112651741151, -218.7731372952745232 ) ) ;
#1795=CARTESIAN_POINT ( 'NONE',  ( -30.66857674073067130, 4.440060741118782239, -229.9901150862898476 ) ) ;
#1796=CARTESIAN_POINT ( 'NONE',  ( -15.44264673875841432, -21.96030778071044054, -219.6531968376115174 ) ) ;
#1797=CARTESIAN_POINT ( 'NONE',  ( 5.511302051500400090, -18.01881380728196902, -231.5522404100356084 ) ) ;
#1798=CARTESIAN_POINT ( 'NONE',  ( 15.14859676485869500, 2.119979922547468032, -231.9009926880791284 ) ) ;
#1799=CARTESIAN_POINT ( 'NONE',  ( 2.464084843620814702, 29.35663482419208492, -227.0015060686748143 ) ) ;
#1800=CARTESIAN_POINT ( 'NONE',  ( -19.40752943788874774, 15.61499612050012864, -234.7624367253776541 ) ) ;
#1802=CARTESIAN_POINT ( 'NONE',  ( 30.72375212156453372, -9.269427080566114086, -227.3728682798597731 ) ) ;
#1803=CARTESIAN_POINT ( 'NONE',  ( 21.35706335192880445, 15.67286272432725092, -219.2578158352350783 ) ) ;
#1804=CARTESIAN_POINT ( 'NONE',  ( -24.53276002501160136, 17.12571705644413811, -226.2419685911331442 ) ) ;
#1805=CARTESIAN_POINT ( 'NONE',  ( -24.33894786102607455, 16.69464852328507831, -227.6320542475859554 ) ) ;
#1806=CARTESIAN_POINT ( 'NONE',  ( -14.26331330459994540, -11.99770975811722451, -232.1846756268951708 ) ) ;
#1808=CARTESIAN_POINT ( 'NONE',  ( 14.33191776452776622, 5.147404080619256916, -219.0172570056664938 ) ) ;
#1809=CARTESIAN_POINT ( 'NONE',  ( -17.65560862077320081, 21.92186454631220371, -221.3776075196718693 ) ) ;
#1810=CARTESIAN_POINT ( 'NONE',  ( 19.07698357483942786, 25.86742807064150895, -222.6991278896559834 ) ) ;
#1811=CARTESIAN_POINT ( 'NONE',  ( 13.89183999136464820, 6.553741795688899252, -220.8646181278399752 ) ) ;
#1812=CARTESIAN_POINT ( 'NONE',  ( -18.30187879049682209, -3.992092017665997972, -215.1717549395094693 ) ) ;
#1814=CARTESIAN_POINT ( 'NONE',  ( -13.01444359484612079, -23.32256785062423887, -219.1545357706015693 ) ) ;
#1815=CARTESIAN_POINT ( 'NONE',  ( -9.439286754415764591, 28.32957437491962338, -228.7842975624562598 ) ) ;
#1816=CARTESIAN_POINT ( 'NONE',  ( 6.427665535191954937, -16.40046818492683656, -232.5919299485929912 ) ) ;
#1817=CARTESIAN_POINT ( 'NONE',  ( 2.008896548638861024, 20.64812324442097591, -233.5818019448501843 ) ) ;
#1818=CARTESIAN_POINT ( 'NONE',  ( 25.69249634387097814, -4.932549985819596472, -232.9896235759753438 ) ) ;
#1819=DIRECTION ( 'NONE',  ( -0.9940043559354229119, 0.1093404791529896669, -4.060016141862974029E-14 ) ) ;
#1821=CARTESIAN_POINT ( 'NONE',  ( 19.55931020704464274, 3.833820734573247346, -215.4549349108404783 ) ) ;
#1823=CARTESIAN_POINT ( 'NONE',  ( -6.564517230509238743, 23.65597541655194647, -219.1225629381441991 ) ) ;
#1824=CARTESIAN_POINT ( 'NONE',  ( 13.06430160593375689, 2.561628050526134182, -220.6026188403641299 ) ) ;
#1825=CARTESIAN_POINT ( 'NONE',  ( 8.812073984913094904, 13.12649198322903210, -229.9172071780580495 ) ) ;
#1826=CARTESIAN_POINT ( 'NONE',  ( 30.47710800431509170, 7.409378661937554789, -223.2007768404241688 ) ) ;
#1827=CARTESIAN_POINT ( 'NONE',  ( 5.002389762228888870, -13.81148461055073362, -218.0662212534467983 ) ) ;
#1828=CARTESIAN_POINT ( 'NONE',  ( 1.867752180833619713, 31.25122076096762669, -227.4007918511463231 ) ) ;
#1830=CARTESIAN_POINT ( 'NONE',  ( -4.226568860449858356, -15.17239585821433678, -217.2407179915541349 ) ) ;
#1831=CARTESIAN_POINT ( 'NONE',  ( -7.464187997994982560, 14.20693289415472016, -228.8865298551900764 ) ) ;
#1833=CARTESIAN_POINT ( 'NONE',  ( 1.939863782649466017, 28.20584428268631783, -229.4487744520996273 ) ) ;
#1834=CARTESIAN_POINT ( 'NONE',  ( -16.64477864544768337, -2.947896226079009807, -219.6737919733007516 ) ) ;
#1835=CARTESIAN_POINT ( 'NONE',  ( -16.03353370602922467, 4.897644413504528060, -222.5335369890782999 ) ) ;
#1836=CARTESIAN_POINT ( 'NONE',  ( -17.00265675087485917, 7.324244386240115645, -218.5600005870616656 ) ) ;
#1837=CARTESIAN_POINT ( 'NONE',  ( 28.09488075336259527, 3.911739131332936381, -227.7543364642411632 ) ) ;
#1839=CARTESIAN_POINT ( 'NONE',  ( 8.689059922489732912, 15.18271246186214363, -218.7354841152034908 ) ) ;
#1840=CARTESIAN_POINT ( 'NONE',  ( 26.90273745076186884, -10.52087603942467808, -226.9519702360728957 ) ) ;
#1842=CARTESIAN_POINT ( 'NONE',  ( 26.86480837698434243, -8.606671353193281249, -231.2046318962545683 ) ) ;
#1843=CARTESIAN_POINT ( 'NONE',  ( -0.7879796667336372851, 21.22375955577181372, -219.1554080315090118 ) ) ;
#1846=CARTESIAN_POINT ( 'NONE',  ( 12.85408565574548412, 7.821283853063205171, -223.1248833997948111 ) ) ;
#1847=CARTESIAN_POINT ( 'NONE',  ( -9.864471611369220128, -7.448779108659549841, -221.8449511945744064 ) ) ;
#1848=CARTESIAN_POINT ( 'NONE',  ( -4.670971249126254499, -22.80666086768999890, -234.0323572959307512 ) ) ;
#1849=CARTESIAN_POINT ( 'NONE',  ( 8.818493748348606331, -10.89961555176610375, -227.9481955143288303 ) ) ;
#1850=CARTESIAN_POINT ( 'NONE',  ( -6.208492967940078877, 16.71913201805454463, -230.4912298573936766 ) ) ;
#1852=CARTESIAN_POINT ( 'NONE',  ( 13.38540196930496862, 9.639609424068478205, -227.8779021328794840 ) ) ;
#1853=CARTESIAN_POINT ( 'NONE',  ( -20.94800339253696109, 4.477632454355491731, -216.5423208360950298 ) ) ;
#1854=CARTESIAN_POINT ( 'NONE',  ( -12.67136363292824086, 22.56975222910433843, -219.0840033572168011 ) ) ;
#1855=CARTESIAN_POINT ( 'NONE',  ( 29.37495210618232022, -3.074218464324032229, -220.1817713028459025 ) ) ;
#1857=CARTESIAN_POINT ( 'NONE',  ( -0.7041916573665241152, 14.60214745152014437, -226.3818583194645555 ) ) ;
#1858=CARTESIAN_POINT ( 'NONE',  ( -16.98287383830707142, 1.584866439881522648, -221.5391863673846444 ) ) ;
#1859=CARTESIAN_POINT ( 'NONE',  ( 23.07558131619435571, 16.33594519118144817, -217.0553921114837124 ) ) ;
#1860=CARTESIAN_POINT ( 'NONE',  ( 4.804712767000853368, -14.77773536573586455, -228.5128529893618747 ) ) ;
#1861=CARTESIAN_POINT ( 'NONE',  ( -22.05223281125454804, 0.4748437386657365367, -217.8785187290425256 ) ) ;
#1863=CARTESIAN_POINT ( 'NONE',  ( -7.825349071214003693, 24.14595706726266755, -216.5959661901539732 ) ) ;
#1864=CARTESIAN_POINT ( 'NONE',  ( -10.99009178837907186, -10.32629327015668785, -231.8361825614163365 ) ) ;
#1867=CARTESIAN_POINT ( 'NONE',  ( 14.98418162551161714, 4.450317369940187895, -227.9894155827521161 ) ) ;
#1868=CARTESIAN_POINT ( 'NONE',  ( -22.47200958260654957, 4.697452857301940732, -216.5879371680706242 ) ) ;
#1869=CARTESIAN_POINT ( 'NONE',  ( 8.649266908999912573, -10.50942778440553482, -226.4415026780416440 ) ) ;
#1870=CARTESIAN_POINT ( 'NONE',  ( -7.825349071214003693, 24.14595706726266755, -216.5959661901539732 ) ) ;
#1871=CARTESIAN_POINT ( 'NONE',  ( -17.96792326766206926, -0.6237852504629022299, -217.9759415197746932 ) ) ;
#1872=CARTESIAN_POINT ( 'NONE',  ( -6.723652888800149441, -28.28510889945508211, -226.1741921951756638 ) ) ;
#1875=CARTESIAN_POINT ( 'NONE',  ( -11.79584727357715934, 6.509288465425584036, -222.6080315736180921 ) ) ;
#1876=CARTESIAN_POINT ( 'NONE',  ( 10.38773686668317531, -11.52324865342443516, -226.2052026729718932 ) ) ;
#1877=CARTESIAN_POINT ( 'NONE',  ( -28.87859926594958537, -0.8320174534291842061, -222.6356913548140142 ) ) ;
#1880=CARTESIAN_POINT ( 'NONE',  ( 27.30736127486511577, 7.960716467858479639, -228.6121938484450595 ) ) ;
#1881=CARTESIAN_POINT ( 'NONE',  ( -20.38637754046084183, 19.95723714148678241, -217.5201383746364172 ) ) ;
#1882=CARTESIAN_POINT ( 'NONE',  ( 13.38540196930496862, 9.639609424068478205, -227.8779021328794840 ) ) ;
#1883=CARTESIAN_POINT ( 'NONE',  ( -0.4481215836501183380, -14.49514564254841353, -225.8120917640279970 ) ) ;
#1884=CARTESIAN_POINT ( 'NONE',  ( 19.25263663724807728, -8.631913731826720948, -234.6583132812941983 ) ) ;
#1886=CARTESIAN_POINT ( 'NONE',  ( 2.630208337444488453, 16.40323635460054774, -219.2570070657488088 ) ) ;
#1887=CARTESIAN_POINT ( 'NONE',  ( -25.20870746202117729, 11.68425842440532136, -223.9066764530103342 ) ) ;
#1888=CARTESIAN_POINT ( 'NONE',  ( -21.39667546302236900, 3.687493526428279100, -235.1435990565495047 ) ) ;
#1890=CARTESIAN_POINT ( 'NONE',  ( -16.02814206296035593, -12.75525137407698040, -230.7643788161867633 ) ) ;
#1893=CARTESIAN_POINT ( 'NONE',  ( 16.31458447723494132, 2.619382102851042671, -229.5862799001085364 ) ) ;
#1894=CARTESIAN_POINT ( 'NONE',  ( 15.15335612453267089, -12.60200553607942098, -219.4566848265094166 ) ) ;
#1895=CARTESIAN_POINT ( 'NONE',  ( 5.331555957413248059, 27.50712867803999728, -219.0801070358024276 ) ) ;
#1897=CARTESIAN_POINT ( 'NONE',  ( -17.39699619235753048, 15.64332637722790054, -216.0406373264262641 ) ) ;
#1900=CARTESIAN_POINT ( 'NONE',  ( 15.51445714770079931, 9.275596138242290678, -215.8565574371285436 ) ) ;
#1901=CARTESIAN_POINT ( 'NONE',  ( 4.907833106823921376, 13.98151846258800290, -229.0190609869640923 ) ) ;
#1902=CARTESIAN_POINT ( 'NONE',  ( 15.16859210357277554, 1.744254869442751099, -222.5574993570340609 ) ) ;
#1903=CARTESIAN_POINT ( 'NONE',  ( -7.800954605602409053, -29.95157606033723496, -226.5906573908930000 ) ) ;
#1904=CARTESIAN_POINT ( 'NONE',  ( 17.15627899979664051, -18.64955541608202694, -217.1729447097152388 ) ) ;
#1907=CARTESIAN_POINT ( 'NONE',  ( -26.42613204384124259, 13.88327151024443395, -218.2510073314678323 ) ) ;
#1908=CARTESIAN_POINT ( 'NONE',  ( -27.21693968233852701, -2.213369147249347524, -221.9579181326467392 ) ) ;
#1911=CARTESIAN_POINT ( 'NONE',  ( 12.43753614017300713, 2.441361880258234862, -222.2750447601761721 ) ) ;
#1912=CARTESIAN_POINT ( 'NONE',  ( -3.223980134944351317, 26.83284996841001302, -219.5167893230652965 ) ) ;
#1913=CARTESIAN_POINT ( 'NONE',  ( 4.936777854427027989, 27.97379167488809060, -227.0886654730259124 ) ) ;
#1915=CARTESIAN_POINT ( 'NONE',  ( 30.30544834784952002, -1.486206387887903047, -219.3838232483325896 ) ) ;
#1917=CARTESIAN_POINT ( 'NONE',  ( 15.61962121506769385, 4.525360868525488911, -229.0684696061408090 ) ) ;
#1918=CARTESIAN_POINT ( 'NONE',  ( -13.01696012539752445, 9.878799299062107409, -218.8446158128127195 ) ) ;
#1919=CARTESIAN_POINT ( 'NONE',  ( -15.23792247720107440, 7.806131751461257373, -230.3336101049160902 ) ) ;
#1920=CARTESIAN_POINT ( 'NONE',  ( -19.02606456345395358, -20.49905271945607055, -219.9673098173381902 ) ) ;
#1921=CARTESIAN_POINT ( 'NONE',  ( -26.02440924314744919, 2.824604386891162111, -232.0644005296583430 ) ) ;
#1924=CARTESIAN_POINT ( 'NONE',  ( 27.13894094332088969, 12.30518789341946295, -220.2765066586875093 ) ) ;
#1925=AXIS2_PLACEMENT_3D ( 'NONE', #13735, #11707, #10354 ) ;
#1926=CARTESIAN_POINT ( 'NONE',  ( -19.72392517715239535, 13.50888179936880107, -230.7714862421596251 ) ) ;
#1927=CARTESIAN_POINT ( 'NONE',  ( 8.126072675580726212, 14.68573014611672534, -233.8823376361746966 ) ) ;
#1928=CARTESIAN_POINT ( 'NONE',  ( 19.30248206944178335, -1.297331563427565726, -230.8957665284791290 ) ) ;
#1929=CARTESIAN_POINT ( 'NONE',  ( -12.51550321509044927, -6.200974036110347143, -231.2371560537167170 ) ) ;
#1931=CARTESIAN_POINT ( 'NONE',  ( -11.96453848309674228, -6.796862595549911568, -223.8262896469332759 ) ) ;
#1932=CARTESIAN_POINT ( 'NONE',  ( -5.861205904341304951, 14.21969934012253312, -219.3213214613830644 ) ) ;
#1933=CARTESIAN_POINT ( 'NONE',  ( -2.270280637033633475, -14.48864307936496765, -230.4581659391201072 ) ) ;
#1934=CARTESIAN_POINT ( 'NONE',  ( -7.189383125363055349, 14.28512618638020548, -231.7475838278701303 ) ) ;
#1935=CARTESIAN_POINT ( 'NONE',  ( 5.326148043627311424, -14.37544986528147639, -217.4292808685971750 ) ) ;
#1936=CARTESIAN_POINT ( 'NONE',  ( -23.14980455159086503, 0.3541108476526578785, -217.8785187302087536 ) ) ;
#1937=CARTESIAN_POINT ( 'NONE',  ( -28.31595744342370580, 5.786754998807587924, -229.0820962600229223 ) ) ;
#1938=CARTESIAN_POINT ( 'NONE',  ( -9.060146982536336324, 27.14942986116457746, -225.6568961786626062 ) ) ;
#1939=CARTESIAN_POINT ( 'NONE',  ( -13.81390866287826746, 1.832988708064121175, -224.4361041349432639 ) ) ;
#1940=CARTESIAN_POINT ( 'NONE',  ( -21.89065952084861522, -0.9940043559354512226, -215.0000000000000000 ) ) ;
#1941=CARTESIAN_POINT ( 'NONE',  ( 15.15306935214909778, 7.771180183537883757, -217.5526096523957165 ) ) ;
#1942=CARTESIAN_POINT ( 'NONE',  ( -0.1762641309874839746, -13.43768854674724977, -229.3744256026976416 ) ) ;
#1943=CARTESIAN_POINT ( 'NONE',  ( 1.898427734299754421, 12.47096978853034521, -227.5043976727869506 ) ) ;
#1945=CARTESIAN_POINT ( 'NONE',  ( 20.89184612657454920, 5.404957034965973683, -232.0952743654565609 ) ) ;
#1946=CARTESIAN_POINT ( 'NONE',  ( -7.274850400134849515, -18.40080456867533698, -234.8703629377345692 ) ) ;
#1947=CARTESIAN_POINT ( 'NONE',  ( -8.857704405076667342, 24.20848540845601704, -218.8859504303524091 ) ) ;
#1948=CARTESIAN_POINT ( 'NONE',  ( 5.702651035983461902, 12.42242820409033222, -224.7304266323218656 ) ) ;
#1950=CARTESIAN_POINT ( 'NONE',  ( -17.21167111787709914, -1.850592482912338799, -230.8442569545952665 ) ) ;
#1951=CARTESIAN_POINT ( 'NONE',  ( -14.67397018911906770, 9.031553917454052893, -228.4349422195089119 ) ) ;
#1952=CARTESIAN_POINT ( 'NONE',  ( -4.334570222994868161, 11.62786715207288601, -222.6396919303362267 ) ) ;
#1953=CARTESIAN_POINT ( 'NONE',  ( 27.54521312182184545, 10.10774643363308023, -222.6232199463151744 ) ) ;
#1955=CARTESIAN_POINT ( 'NONE',  ( 7.240923751923983964, -14.90955521745277501, -222.5312387745455283 ) ) ;
#1957=CARTESIAN_POINT ( 'NONE',  ( 11.29822263435752205, -11.23247557268489771, -230.2410575525588570 ) ) ;
#1958=CARTESIAN_POINT ( 'NONE',  ( -3.130917144532865848, 26.01013079854885390, -229.4331404728494874 ) ) ;
#1962=CARTESIAN_POINT ( 'NONE',  ( 14.31308345469695453, 12.76656023072872159, -231.9445021321040770 ) ) ;
#1963=CARTESIAN_POINT ( 'NONE',  ( -30.62445638522240188, 0.2907099072661952222, -224.9999970559163387 ) ) ;
#1964=CARTESIAN_POINT ( 'NONE',  ( -7.800954605602409053, -29.95157606033723496, -226.5906573908930000 ) ) ;
#1965=CARTESIAN_POINT ( 'NONE',  ( 8.021672912688133650, -23.92397517040199872, -233.3380040120402441 ) ) ;
#1966=CARTESIAN_POINT ( 'NONE',  ( -7.058999618647554541, 24.62458660126260312, -219.6630466582859356 ) ) ;
#1968=CARTESIAN_POINT ( 'NONE',  ( 12.91676121433235913, 9.519065828383201477, -226.8102878246443765 ) ) ;
#1969=CARTESIAN_POINT ( 'NONE',  ( -3.326157069579807946, 13.92020081821418565, -220.5733722327383930 ) ) ;
#1970=CARTESIAN_POINT ( 'NONE',  ( -13.96653539523557619, 20.94398119165846239, -231.8597527081015528 ) ) ;
#1971=CARTESIAN_POINT ( 'NONE',  ( -3.494873682963683059, 27.70407912598904687, -220.5214894769905243 ) ) ;
#1972=CARTESIAN_POINT ( 'NONE',  ( -19.67797246974518544, 1.229961341702398681, -219.4743747885323160 ) ) ;
#1973=CARTESIAN_POINT ( 'NONE',  ( 11.20713200305815427, 28.28922876448651635, -219.1239564724620834 ) ) ;
#1974=CARTESIAN_POINT ( 'NONE',  ( 13.17817051516727922, -26.22376201054615308, -223.3126545406654486 ) ) ;
#1977=CARTESIAN_POINT ( 'NONE',  ( 1.773982976645536835, 19.12448993322812285, -233.2315972735944172 ) ) ;
#1978=CARTESIAN_POINT ( 'NONE',  ( 16.24842259479558848, -3.494976385286828080, -222.6392560871376816 ) ) ;
#1980=CARTESIAN_POINT ( 'NONE',  ( 21.60524407607017849, 3.028118258437591415, -217.8361640396714449 ) ) ;
#1981=CARTESIAN_POINT ( 'NONE',  ( -26.58771759052039485, 5.114955214121561511, -218.2823714869195442 ) ) ;
#1983=CARTESIAN_POINT ( 'NONE',  ( 2.513843158659109456, -14.78137297724497401, -219.3443999184743518 ) ) ;
#1984=CARTESIAN_POINT ( 'NONE',  ( -6.855867220396999251, 12.17758473459128332, -220.6375607554995213 ) ) ;
#1986=CARTESIAN_POINT ( 'NONE',  ( -29.30406754532526037, 5.063969254119831120, -221.8212091093853076 ) ) ;
#1987=CARTESIAN_POINT ( 'NONE',  ( -9.225692202065292946, -15.38374647092247116, -218.6784895636799320 ) ) ;
#1989=CARTESIAN_POINT ( 'NONE',  ( -25.61997837663875188, 10.01664178086244483, -231.6711741719404074 ) ) ;
#1990=CARTESIAN_POINT ( 'NONE',  ( 20.36520141328406552, -18.94542628267938156, -227.6082859645964902 ) ) ;
#1993=CARTESIAN_POINT ( 'NONE',  ( 24.96615890023450035, 5.871290975262302148, -218.1661911638112201 ) ) ;
#1995=CARTESIAN_POINT ( 'NONE',  ( -7.312583518931054627, 16.22063427959223958, -217.3454962955413521 ) ) ;
#1997=CARTESIAN_POINT ( 'NONE',  ( 20.58393751692968721, 18.55948753678544705, -226.8933397075267635 ) ) ;
#1998=CARTESIAN_POINT ( 'NONE',  ( 0.3267584840439746174, -16.39795729406718650, -220.1296710765888065 ) ) ;
#1999=CARTESIAN_POINT ( 'NONE',  ( 26.13397685888192257, -0.5417465609251845837, -217.5756777990261526 ) ) ;
#2001=CARTESIAN_POINT ( 'NONE',  ( 0.8374361358884788720, 23.73768315274483953, -232.4065959030912154 ) ) ;
#2002=CARTESIAN_POINT ( 'NONE',  ( -16.58624905143161143, 8.715293938925766426, -220.0618460037763384 ) ) ;
#2003=CARTESIAN_POINT ( 'NONE',  ( -25.59521542166570640, 7.637420400166985424, -216.4190921938142935 ) ) ;
#2004=CARTESIAN_POINT ( 'NONE',  ( -14.51900513504577717, -8.991447007532661573, -221.0515111571761793 ) ) ;
#2007=CARTESIAN_POINT ( 'NONE',  ( 27.84414217501293010, 2.965433895642837214, -221.8999927093654492 ) ) ;
#2008=CARTESIAN_POINT ( 'NONE',  ( 0.4541713596374759021, -15.35025901140449989, -222.0332685144132370 ) ) ;
#2009=CARTESIAN_POINT ( 'NONE',  ( 26.24002132888527328, 11.62331517472360964, -222.5300873157218859 ) ) ;
#2010=CARTESIAN_POINT ( 'NONE',  ( -13.58874046263339608, 12.73011668665171392, -216.5659449791897941 ) ) ;
#2012=CARTESIAN_POINT ( 'NONE',  ( 20.64287812348744566, 0.2024751443801864337, -216.7518974727033481 ) ) ;
#2014=CARTESIAN_POINT ( 'NONE',  ( 5.141746912158045468, 22.01688500372448232, -216.6678693612369386 ) ) ;
#2015=CARTESIAN_POINT ( 'NONE',  ( 14.15986309589296788, 2.061458568213107245, -222.8204610720217147 ) ) ;
#2016=CARTESIAN_POINT ( 'NONE',  ( -1.608171596096409806, -16.77465153034988887, -217.4618546331240054 ) ) ;
#2017=CARTESIAN_POINT ( 'NONE',  ( 25.69672030403964769, -15.30292110028031338, -224.0206579222720791 ) ) ;
#2020=CARTESIAN_POINT ( 'NONE',  ( -7.399925907206128528, 10.29859031525428037, -227.1614041762800298 ) ) ;
#2021=CARTESIAN_POINT ( 'NONE',  ( -25.38303270991942284, -1.762464254583185452, -219.8781034644853776 ) ) ;
#2022=CARTESIAN_POINT ( 'NONE',  ( 29.47107563651793427, 6.731311671946880182, -220.0565342412898815 ) ) ;
#2023=CARTESIAN_POINT ( 'NONE',  ( 0.3632086708616291126, 21.06287758167331958, -232.5112839711303820 ) ) ;
#2024=CARTESIAN_POINT ( 'NONE',  ( 5.142103055192286831, 28.18228231877369439, -225.8998064704803994 ) ) ;
#2026=CARTESIAN_POINT ( 'NONE',  ( 9.181101971147782592, -9.127577137574531818, -229.3209091633710273 ) ) ;
#2027=VERTEX_POINT ( 'NONE', #10233 ) ;
#2029=CARTESIAN_POINT ( 'NONE',  ( 19.19288224840068935, 10.13059690604263174, -232.1906135022504998 ) ) ;
#2030=CARTESIAN_POINT ( 'NONE',  ( -14.58670098223046629, 7.239570004716886942, -229.3284954533748135 ) ) ;
#2031=CARTESIAN_POINT ( 'NONE',  ( -21.66801938871533650, 16.28801167444048659, -218.5240035253498547 ) ) ;
#2032=CARTESIAN_POINT ( 'NONE',  ( -30.78084016402396372, -2.501288241119758116, -224.5721874330603214 ) ) ;
#2033=CARTESIAN_POINT ( 'NONE',  ( -10.65455960636934662, 10.37188583052882862, -219.5197110153079620 ) ) ;
#2035=CARTESIAN_POINT ( 'NONE',  ( 14.88115968084168728, -2.531949626111721585, -226.6122033079182074 ) ) ;
#2036=CARTESIAN_POINT ( 'NONE',  ( 22.36788034568564854, -2.140002702436959225, -217.7104380410378610 ) ) ;
#2039=CARTESIAN_POINT ( 'NONE',  ( -11.83954511762131112, 10.58068896997146346, -226.6171226499791089 ) ) ;
#2040=CARTESIAN_POINT ( 'NONE',  ( 12.58033168766476528, 20.35631482982274676, -235.1670639654690547 ) ) ;
#2041=CARTESIAN_POINT ( 'NONE',  ( -16.15126510923403202, -0.4755054218165427615, -219.3066569788202571 ) ) ;
#2042=CARTESIAN_POINT ( 'NONE',  ( -28.75820353979175081, -10.31764292692039753, -230.8958203355234389 ) ) ;
#2043=CARTESIAN_POINT ( 'NONE',  ( -25.32486352395475393, -3.505876693931964549, -233.0869506614649822 ) ) ;
#2044=CARTESIAN_POINT ( 'NONE',  ( -23.16143087541734502, 21.36835206473086046, -221.8715256527013651 ) ) ;
#2045=CARTESIAN_POINT ( 'NONE',  ( -11.06377138986482933, -15.30386857868810857, -217.0411070525910873 ) ) ;
#2046=CARTESIAN_POINT ( 'NONE',  ( 17.68508104102419409, 23.41266195669770767, -227.5327139115408954 ) ) ;
#2047=CARTESIAN_POINT ( 'NONE',  ( 3.531840179394873491, -11.29480931768500618, -224.5922842895475355 ) ) ;
#2049=CARTESIAN_POINT ( 'NONE',  ( 12.43753614017300713, 2.441361880258234862, -222.2750447601761721 ) ) ;
#2050=CARTESIAN_POINT ( 'NONE',  ( -2.612157044224189484, 27.88031182936952135, -224.5292183073761692 ) ) ;
#2051=CARTESIAN_POINT ( 'NONE',  ( -24.15814485343234352, 4.373587128574028426, -232.6698675874553430 ) ) ;
#2052=CARTESIAN_POINT ( 'NONE',  ( 15.42212722119060864, 5.401662248084913465, -220.8333402320903645 ) ) ;
#2053=CARTESIAN_POINT ( 'NONE',  ( 15.89621445970763070, 6.639162626453350313, -232.5295318698041456 ) ) ;
#2054=CARTESIAN_POINT ( 'NONE',  ( -9.132447960227011663, -28.48575439045284696, -228.2342138548108892 ) ) ;
#2055=CARTESIAN_POINT ( 'NONE',  ( 10.22554538262735413, 24.20440706210576209, -215.6176527921760737 ) ) ;
#2057=CARTESIAN_POINT ( 'NONE',  ( -14.97068153222459408, -28.62142063984003215, -225.0224449979507142 ) ) ;
#2058=CARTESIAN_POINT ( 'NONE',  ( -7.375127652145912371, 13.01042140126078195, -223.9959097520547004 ) ) ;
#2059=CARTESIAN_POINT ( 'NONE',  ( 11.96568375430165254, 8.504117401580989721, -219.8633768076029753 ) ) ;
#2060=CARTESIAN_POINT ( 'NONE',  ( -29.27492217116574480, -1.185422171198730501, -224.8132346143397342 ) ) ;
#2061=CARTESIAN_POINT ( 'NONE',  ( -17.75632171729475317, 14.45153669854845901, -218.6240360064753929 ) ) ;
#2062=CARTESIAN_POINT ( 'NONE',  ( -9.251743101293765648, 14.06372330290396278, -232.4239003576353468 ) ) ;
#2063=CARTESIAN_POINT ( 'NONE',  ( 15.92396645628901020, -0.3225394686005420009, -223.0199929375764327 ) ) ;
#2065=CARTESIAN_POINT ( 'NONE',  ( 6.629309777743229937, -15.42610274396934855, -227.9597969125812256 ) ) ;
#2066=CARTESIAN_POINT ( 'NONE',  ( 13.07616324839670341, -23.69356132834180784, -230.7206382488779184 ) ) ;
#2067=CARTESIAN_POINT ( 'NONE',  ( -2.618694198633108261, 15.69630225547860825, -226.1451761977223498 ) ) ;
#2070=CARTESIAN_POINT ( 'NONE',  ( 16.54345861550681107, 19.37554510112122230, -218.2240151908141002 ) ) ;
#2071=CARTESIAN_POINT ( 'NONE',  ( -13.18205254385204661, -0.5588607053421433823, -223.2849229087554761 ) ) ;
#2072=CARTESIAN_POINT ( 'NONE',  ( -25.82802808205240552, -14.78441951539553401, -222.6940535085979604 ) ) ;
#2073=CARTESIAN_POINT ( 'NONE',  ( 7.486336813247038258, -29.35413437595724773, -221.4114973598149447 ) ) ;
#2074=CARTESIAN_POINT ( 'NONE',  ( -5.600903697806950632, 21.62055466701630735, -218.6671277943675307 ) ) ;
#2076=CARTESIAN_POINT ( 'NONE',  ( 18.51425713624010427, 11.82474821235740592, -231.3645840199355632 ) ) ;
#2077=CARTESIAN_POINT ( 'NONE',  ( -11.42613629117093765, 28.09170287990588832, -228.7150250545069241 ) ) ;
#2078=CARTESIAN_POINT ( 'NONE',  ( -6.901278853520646628, 15.41233971300566807, -220.5972764307651346 ) ) ;
#2081=CARTESIAN_POINT ( 'NONE',  ( 2.808299412262623473, 18.06245856371233316, -217.9832661743849656 ) ) ;
#2082=CARTESIAN_POINT ( 'NONE',  ( -15.82760502346409304, 5.624826830110399634, -227.5369622385896946 ) ) ;
#2083=CARTESIAN_POINT ( 'NONE',  ( 27.08260752785270853, 4.114838227474355570, -232.2882281786467331 ) ) ;
#2084=CARTESIAN_POINT ( 'NONE',  ( 5.380811198380419214, -14.52623441703906160, -221.9013399998540024 ) ) ;
#2087=CARTESIAN_POINT ( 'NONE',  ( 4.343013938751969505, 13.02036404005131587, -224.7825435359082178 ) ) ;
#2088=CARTESIAN_POINT ( 'NONE',  ( 24.96598054343045447, -3.653363829669123319, -219.8248103142179559 ) ) ;
#2090=CARTESIAN_POINT ( 'NONE',  ( 22.86997486125673618, 17.56009411325475966, -222.3578648042903296 ) ) ;
#2091=CARTESIAN_POINT ( 'NONE',  ( 12.73130673999417795, -23.76414828096303467, -217.7386337832039942 ) ) ;
#2093=CARTESIAN_POINT ( 'NONE',  ( -16.39453490553961856, 20.24836633112041184, -233.1722131570092245 ) ) ;
#2094=CARTESIAN_POINT ( 'NONE',  ( -19.58639255110637478, 14.91076398872931819, -217.1105532241463720 ) ) ;
#2095=CARTESIAN_POINT ( 'NONE',  ( 20.54442553493903389, -1.409480604460696007, -231.2888200459364327 ) ) ;
#2096=CARTESIAN_POINT ( 'NONE',  ( -16.38803511840525218, -9.809678413005567421, -217.1940421839195494 ) ) ;
#2099=CARTESIAN_POINT ( 'NONE',  ( -22.47200958260654957, 4.697452857301940732, -216.5879371680706242 ) ) ;
#2100=CARTESIAN_POINT ( 'NONE',  ( 0.2152704783746036410, -12.84635275796930642, -226.1081088095504015 ) ) ;
#2103=CARTESIAN_POINT ( 'NONE',  ( 24.93482953594869755, 13.13888391581411241, -222.4369546851285691 ) ) ;
#2104=CARTESIAN_POINT ( 'NONE',  ( -21.64120863631820413, 17.87363223393748868, -233.1390268986752119 ) ) ;
#2107=CARTESIAN_POINT ( 'NONE',  ( 20.92326490933994876, 18.00580109995737033, -222.6060933800056034 ) ) ;
#2108=CARTESIAN_POINT ( 'NONE',  ( -0.5904090961472509003, -15.19049578300894510, -228.4387523405810612 ) ) ;
#2111=CARTESIAN_POINT ( 'NONE',  ( -1.772400894765090662, 19.49811434610897010, -217.8797837662441168 ) ) ;
#2112=CARTESIAN_POINT ( 'NONE',  ( -8.985448925281199095, 11.82743561134668475, -224.1067108988273162 ) ) ;
#2113=CARTESIAN_POINT ( 'NONE',  ( -29.98527381603928887, 6.316825171121390525, -230.1108345570740994 ) ) ;
#2114=CARTESIAN_POINT ( 'NONE',  ( -13.68888474783054399, -8.264665463295720826, -223.0168115903771024 ) ) ;
#2117=CARTESIAN_POINT ( 'NONE',  ( 12.91815243135930480, 5.607966342865584153, -224.2227256053222959 ) ) ;
#2118=CARTESIAN_POINT ( 'NONE',  ( 6.833096512853454207, -24.74801519961247465, -219.7405977492105364 ) ) ;
#2119=CARTESIAN_POINT ( 'NONE',  ( 15.87442104186276381, 8.674488492264579520, -230.9702037640878416 ) ) ;
#2120=CARTESIAN_POINT ( 'NONE',  ( -12.90983082593748676, 14.84936372681532823, -233.8009687022269532 ) ) ;
#2122=CARTESIAN_POINT ( 'NONE',  ( 22.17049319811867036, 0.5483778423327810847, -216.5715983009590673 ) ) ;
#2123=CARTESIAN_POINT ( 'NONE',  ( 4.354034006296288339, 14.09944204372416188, -221.2519525881239417 ) ) ;
#2126=CARTESIAN_POINT ( 'NONE',  ( -6.722478243781921492, -14.20656108661463612, -231.4169491518476889 ) ) ;
#2127=CARTESIAN_POINT ( 'NONE',  ( 16.07085865561684201, -17.65509622858733252, -216.6880805489183501 ) ) ;
#2130=CARTESIAN_POINT ( 'NONE',  ( -9.964021556040458805, 12.25789996591640119, -217.8262340283327774 ) ) ;
#2131=CARTESIAN_POINT ( 'NONE',  ( -16.09622215267033596, -6.362375831002168525, -228.5323951500822943 ) ) ;
#2132=CARTESIAN_POINT ( 'NONE',  ( -14.69827142695382527, 14.49176359921644597, -217.9600391472806109 ) ) ;
#2133=CARTESIAN_POINT ( 'NONE',  ( 3.312424284731937618, 15.29837714273186045, -229.5209971419123747 ) ) ;
#2134=CARTESIAN_POINT ( 'NONE',  ( 5.112468059216026539, 15.05346046978967856, -223.6558835435016590 ) ) ;
#2136=CARTESIAN_POINT ( 'NONE',  ( 9.167096742983094515, -14.53852251116023986, -217.0563232478103828 ) ) ;
#2138=CARTESIAN_POINT ( 'NONE',  ( 24.58316096239279602, 5.861425670879941485, -231.3104446318280623 ) ) ;
#2139=CARTESIAN_POINT ( 'NONE',  ( -7.752954785937490989, 10.21341112307795385, -225.5135920495299615 ) ) ;
#2140=CARTESIAN_POINT ( 'NONE',  ( -15.61959985466312872, 8.133362592386543355, -230.7826037412100106 ) ) ;
#2141=CARTESIAN_POINT ( 'NONE',  ( -24.78729321827560739, -16.46449136890227294, -222.3867555963062443 ) ) ;
#2142=CARTESIAN_POINT ( 'NONE',  ( -27.82842955277035202, 11.70195273568964112, -227.9294339757464911 ) ) ;
#2144=CARTESIAN_POINT ( 'NONE',  ( 21.52074627118099315, 8.791036694007010155, -215.9547738671300294 ) ) ;
#2145=CARTESIAN_POINT ( 'NONE',  ( -18.64931821476190876, 22.04453097546810270, -226.2485927806324923 ) ) ;
#2146=CARTESIAN_POINT ( 'NONE',  ( 18.26039090677515375, 26.14311541888654844, -228.1864986152887127 ) ) ;
#2147=CARTESIAN_POINT ( 'NONE',  ( -13.11494368899652052, 3.355507568391938200, -225.9121440085824304 ) ) ;
#2148=CARTESIAN_POINT ( 'NONE',  ( -23.48355816166749932, -5.921172941748132246, -214.8630305010649408 ) ) ;
#2149=CARTESIAN_POINT ( 'NONE',  ( -25.34460520202507539, -7.988444519707189606, -217.6292756219348234 ) ) ;
#2150=CARTESIAN_POINT ( 'NONE',  ( -1.946052076048385482, 22.23149728939677061, -232.8927760318659068 ) ) ;
#2151=CARTESIAN_POINT ( 'NONE',  ( -6.012234575298915473, -13.00555924700598709, -229.4955436083688483 ) ) ;
#2152=CARTESIAN_POINT ( 'NONE',  ( 6.093530912645064745, 16.79941505724243811, -232.1766444656230419 ) ) ;
#2153=CARTESIAN_POINT ( 'NONE',  ( 8.798770371347417907, -12.71349942585338333, -232.9159113209695704 ) ) ;
#2155=CARTESIAN_POINT ( 'NONE',  ( 13.98152565379061052, 2.156981915107639036, -230.5667344709999611 ) ) ;
#2157=CARTESIAN_POINT ( 'NONE',  ( -0.6272116608575281083, 20.18031380156121202, -219.3960054794027030 ) ) ;
#2158=CARTESIAN_POINT ( 'NONE',  ( -22.13857085231108712, 6.545953331035805789, -217.2801712530867633 ) ) ;
#2159=CARTESIAN_POINT ( 'NONE',  ( 20.23125423326388628, 7.836699765464857137, -217.8891354894872450 ) ) ;
#2160=CARTESIAN_POINT ( 'NONE',  ( 16.73391517716289911, 11.95167056011791828, -233.0268722588312755 ) ) ;
#2161=CARTESIAN_POINT ( 'NONE',  ( -14.39178795515995724, -23.41959061255243313, -230.2514514786898019 ) ) ;
#2162=CARTESIAN_POINT ( 'NONE',  ( 2.987882271643250931, 28.57355997650491020, -217.8917278841813925 ) ) ;
#2164=CARTESIAN_POINT ( 'NONE',  ( -11.40836237951390508, -18.42461209671423816, -214.6264694599774430 ) ) ;
#2165=CARTESIAN_POINT ( 'NONE',  ( -4.466732464217805898, 19.42663028452474450, -231.9485309169485561 ) ) ;
#2166=CARTESIAN_POINT ( 'NONE',  ( 14.63115627273841923, 9.024791562541032874, -232.5054678133655841 ) ) ;
#2167=CARTESIAN_POINT ( 'NONE',  ( -21.10507617219916199, 14.90539259013048756, -229.7677326419877488 ) ) ;
#2169=CARTESIAN_POINT ( 'NONE',  ( -4.695076324262313250, 31.85502299853856201, -223.8918597786031341 ) ) ;
#2171=CARTESIAN_POINT ( 'NONE',  ( 19.87150736056128864, 8.436445599727830924, -233.0166429845654932 ) ) ;
#2172=CARTESIAN_POINT ( 'NONE',  ( 17.47473467751515486, -18.15791173363047051, -230.0427332633545632 ) ) ;
#2173=CARTESIAN_POINT ( 'NONE',  ( 15.50624253654579654, -15.96056326703506478, -233.0338314371582840 ) ) ;
#2174=CARTESIAN_POINT ( 'NONE',  ( -2.532302712337851425, 16.54370602006230939, -228.1940632970506613 ) ) ;
#2176=CARTESIAN_POINT ( 'NONE',  ( 17.19674704922021391, 23.07334190050143974, -228.8256488842130238 ) ) ;
#2177=CARTESIAN_POINT ( 'NONE',  ( -16.32911940539174367, -0.4850290419235887551, -232.0399150213553412 ) ) ;
#2178=CARTESIAN_POINT ( 'NONE',  ( -15.58529874627549461, -6.917566422457355202, -219.0138643999995054 ) ) ;
#2179=CARTESIAN_POINT ( 'NONE',  ( 4.201723131641114328, -20.76291977712905279, -215.9522215885928347 ) ) ;
#2180=CARTESIAN_POINT ( 'NONE',  ( -6.769588938507062004, 18.22485903270490937, -231.3660928915624879 ) ) ;
#2182=CARTESIAN_POINT ( 'NONE',  ( 17.42772712443221650, 11.35756022693713341, -231.2166398222404382 ) ) ;
#2183=CARTESIAN_POINT ( 'NONE',  ( -11.24282496690421596, 12.44430180464951086, -232.4405891940542404 ) ) ;
#2184=CARTESIAN_POINT ( 'NONE',  ( -10.52776196018457711, 13.57482816453351937, -219.2327734183297423 ) ) ;
#2186=CARTESIAN_POINT ( 'NONE',  ( 10.25948093768852054, 28.38842464930171872, -224.3436940787075855 ) ) ;
#2187=CARTESIAN_POINT ( 'NONE',  ( -20.21481434941064848, 7.972326285609216967, -230.8475376972877484 ) ) ;
#2188=CARTESIAN_POINT ( 'NONE',  ( 29.21307215008108216, 4.139194015751272104, -229.9658791484231699 ) ) ;
#2189=CARTESIAN_POINT ( 'NONE',  ( 4.725966861008204845, -14.24791254766627624, -227.2781441550517343 ) ) ;
#2193=CARTESIAN_POINT ( 'NONE',  ( 7.995304978256253747, 13.28024228361502779, -220.6535174700288451 ) ) ;
#2194=CARTESIAN_POINT ( 'NONE',  ( 28.03541074264261113, -3.118360251426135488, -224.4433144283077581 ) ) ;
#2196=CARTESIAN_POINT ( 'NONE',  ( 20.58703255433590940, 0.4816031003617209372, -231.9427175861361263 ) ) ;
#2197=CARTESIAN_POINT ( 'NONE',  ( 1.127544764349826867, -27.89617517048659323, -231.9509945439240823 ) ) ;
#2198=CARTESIAN_POINT ( 'NONE',  ( -18.09776816382430908, 23.50806826204562583, -229.9568677523880638 ) ) ;
#2199=CARTESIAN_POINT ( 'NONE',  ( -13.31245686955614005, 26.96290519511623174, -230.1796856776773836 ) ) ;
#2201=CARTESIAN_POINT ( 'NONE',  ( -24.68906941503829700, 2.445024713909649705, -232.6803430500543755 ) ) ;
#2202=CARTESIAN_POINT ( 'NONE',  ( -8.978805095734141872, -14.89723076936793156, -219.0730636071341451 ) ) ;
#2205=CARTESIAN_POINT ( 'NONE',  ( -24.48580119005125866, 9.312492396273500006, -232.5498413856076070 ) ) ;
#2206=CARTESIAN_POINT ( 'NONE',  ( -0.6133843921297743584, -15.86829592205942419, -231.9438830533787268 ) ) ;
#2209=CARTESIAN_POINT ( 'NONE',  ( 14.37653162493774239, 9.985418694807894013, -229.1686718965858063 ) ) ;
#2210=CARTESIAN_POINT ( 'NONE',  ( -5.607934827417612844, 15.68271927908880770, -232.1026723719274969 ) ) ;
#2212=CARTESIAN_POINT ( 'NONE',  ( 21.07144422417032104, 18.33581350331571969, -223.6711752364813890 ) ) ;
#2213=CARTESIAN_POINT ( 'NONE',  ( -1.686103422391260764, -28.85289795882446029, -227.6662241409997876 ) ) ;
#2215=CARTESIAN_POINT ( 'NONE',  ( -1.038524475621362075, 14.89017051181998141, -222.3948816610352139 ) ) ;
#2216=CARTESIAN_POINT ( 'NONE',  ( -12.33583941212908108, 22.27382123621224608, -231.6290720151527296 ) ) ;
#2217=CARTESIAN_POINT ( 'NONE',  ( -21.07387565400155438, 1.107905485989369554, -215.0000000023499069 ) ) ;
#2220=CARTESIAN_POINT ( 'NONE',  ( -13.03991958801536555, -12.43893258430110471, -220.5791972147702040 ) ) ;
#2223=CARTESIAN_POINT ( 'NONE',  ( -29.88125065636863198, 4.504452993877526623, -226.2048141718237275 ) ) ;
#2224=CARTESIAN_POINT ( 'NONE',  ( 8.343784211782431015, -26.96289276196324636, -225.6651636531778422 ) ) ;
#2225=CARTESIAN_POINT ( 'NONE',  ( 11.62313423782632782, 11.98467543564608029, -219.7293303032897995 ) ) ;
#2226=CARTESIAN_POINT ( 'NONE',  ( 1.773982976645536835, 19.12448993322812285, -233.2315972735944172 ) ) ;
#2229=CARTESIAN_POINT ( 'NONE',  ( 29.00474534066713872, 11.29707752057770698, -221.8682176444242771 ) ) ;
#2232=CARTESIAN_POINT ( 'NONE',  ( 7.639528166734322667, 11.92751229241157596, -224.6077814063189635 ) ) ;
#2234=CARTESIAN_POINT ( 'NONE',  ( -8.379125946468517938, -29.31735857037017468, -221.8060643354269814 ) ) ;
#2235=CARTESIAN_POINT ( 'NONE',  ( 24.05826999138443156, -14.97270453765939102, -220.1026142722873260 ) ) ;
#2237=CARTESIAN_POINT ( 'NONE',  ( -9.503027668167838726, 6.959046566381404730, -225.7241663910276941 ) ) ;
#2238=CARTESIAN_POINT ( 'NONE',  ( -21.34127571194312623, -5.850660018714998856, -219.1209233896074977 ) ) ;
#2240=CARTESIAN_POINT ( 'NONE',  ( -14.57944476639264764, 6.129437248167259433, -229.4766146696829310 ) ) ;
#2241=CARTESIAN_POINT ( 'NONE',  ( 12.95792863868717149, 16.83236386576623644, -216.3406066345214356 ) ) ;
#2242=CARTESIAN_POINT ( 'NONE',  ( 6.332229114051408203, 16.75791367489523154, -229.7702805136205200 ) ) ;
#2244=CARTESIAN_POINT ( 'NONE',  ( 11.13603681652449318, -5.602932040673746172, -228.8141337797931101 ) ) ;
#2246=CARTESIAN_POINT ( 'NONE',  ( 20.89184612657454920, 5.404957034965973683, -232.0952743654565609 ) ) ;
#2249=CARTESIAN_POINT ( 'NONE',  ( -10.30034651166687887, 25.05454868506992838, -216.5587736482213188 ) ) ;
#2250=CARTESIAN_POINT ( 'NONE',  ( -12.98662328632235585, 28.83726371277012035, -223.5970274767108776 ) ) ;
#2251=CARTESIAN_POINT ( 'NONE',  ( -18.41550138691291139, -5.273244084890690075, -216.7348800533310964 ) ) ;
#2252=CARTESIAN_POINT ( 'NONE',  ( -12.44873260470819787, 7.411970124596155785, -229.4214091473984070 ) ) ;
#2254=CARTESIAN_POINT ( 'NONE',  ( 27.02029988085337919, -0.4174685747284823112, -230.1188858631967378 ) ) ;
#2255=CARTESIAN_POINT ( 'NONE',  ( -18.67270963783218463, 15.11229250701181925, -218.9067109956068578 ) ) ;
#2256=CARTESIAN_POINT ( 'NONE',  ( 14.54999166170408209, 3.068772298969228096, -219.4784171371563275 ) ) ;
#2257=CARTESIAN_POINT ( 'NONE',  ( 24.32561047128371001, 1.769413244618101011, -218.8629106451077462 ) ) ;
#2258=CARTESIAN_POINT ( 'NONE',  ( 10.83706092800007781, 10.12544885278926543, -227.1716144446442343 ) ) ;
#2260=CARTESIAN_POINT ( 'NONE',  ( -13.36955836198420577, -3.222265253903016990, -227.4060678739157026 ) ) ;
#2261=CARTESIAN_POINT ( 'NONE',  ( -1.243734262319729389, 14.23902626181890518, -226.4313640849764795 ) ) ;
#2262=CARTESIAN_POINT ( 'NONE',  ( 0.7326557587344989519, -29.96088689026728602, -229.4725774697800205 ) ) ;
#2263=CARTESIAN_POINT ( 'NONE',  ( 10.02513374692848913, 18.81568788741115128, -217.1505009242214612 ) ) ;
#2264=CARTESIAN_POINT ( 'NONE',  ( 6.835279263914467052, -26.27742004305391177, -233.7345821414606348 ) ) ;
#2265=CARTESIAN_POINT ( 'NONE',  ( -19.74163224554151697, 8.726897413558679872, -232.6665747339030190 ) ) ;
#2266=CARTESIAN_POINT ( 'NONE',  ( 18.79106389458910442, -5.302521403133691358, -233.5021979784848440 ) ) ;
#2268=CARTESIAN_POINT ( 'NONE',  ( 4.555016420009541989, 17.65848956729471197, -229.5875910199184204 ) ) ;
#2269=CARTESIAN_POINT ( 'NONE',  ( -12.87285471141929172, 9.485162256560764504, -229.1865421006261840 ) ) ;
#2270=CARTESIAN_POINT ( 'NONE',  ( 14.85123888640019452, 5.067529763532427012, -221.9058491819374979 ) ) ;
#2271=CARTESIAN_POINT ( 'NONE',  ( -12.33332453308451804, -15.34461866416700282, -218.5928953102074388 ) ) ;
#2272=CARTESIAN_POINT ( 'NONE',  ( 11.21112214669106777, 5.418350954422431975, -227.6539796508718325 ) ) ;
#2276=CARTESIAN_POINT ( 'NONE',  ( 1.145088139557171036, -28.55736460288477119, -218.6379321102267284 ) ) ;
#2277=CARTESIAN_POINT ( 'NONE',  ( -7.965409144353247761, 13.56739834143082213, -221.6246244520798712 ) ) ;
#2278=CARTESIAN_POINT ( 'NONE',  ( 11.64932556965463561, 7.668732705389711413, -229.0406978839571366 ) ) ;
#2279=CARTESIAN_POINT ( 'NONE',  ( -19.33106196848021341, 9.919700385716687663, -219.0532654734256255 ) ) ;
#2280=CARTESIAN_POINT ( 'NONE',  ( -12.39195900010699702, 23.13258866008456138, -233.4668451572263166 ) ) ;
#2281=CARTESIAN_POINT ( 'NONE',  ( 25.70381634773192658, 10.55338509461953400, -230.3576492130207782 ) ) ;
#2282=CARTESIAN_POINT ( 'NONE',  ( 10.85023464552735462, -16.86364573545779777, -230.5238403791007045 ) ) ;
#2283=CARTESIAN_POINT ( 'NONE',  ( 19.66153801111809685, -22.47763448259700780, -224.4992982350615023 ) ) ;
#2284=CARTESIAN_POINT ( 'NONE',  ( 0.9458336400950161371, 17.49535648476021876, -228.8359568483051589 ) ) ;
#2287=CARTESIAN_POINT ( 'NONE',  ( 22.03647168420945590, 0.3315607655625663064, -232.0572713672586644 ) ) ;
#2288=CARTESIAN_POINT ( 'NONE',  ( -30.16187987321119834, 0.7031948255570967810, -222.4584828387981474 ) ) ;
#2289=CARTESIAN_POINT ( 'NONE',  ( -8.878187501988019648, -11.23476449186280846, -221.0271673637577123 ) ) ;
#2291=CARTESIAN_POINT ( 'NONE',  ( 0.7326557587344989519, -29.96088689026728602, -229.4725774697800205 ) ) ;
#2292=CARTESIAN_POINT ( 'NONE',  ( 7.508136856874425114, 24.19512352541684663, -230.0608033085341617 ) ) ;
#2294=CARTESIAN_POINT ( 'NONE',  ( -14.99655511003079233, 2.316638599135941945, -232.4215266639120046 ) ) ;
#2296=CARTESIAN_POINT ( 'NONE',  ( -3.003186468682855104, 15.63968344752823469, -231.5301608670590667 ) ) ;
#2297=CARTESIAN_POINT ( 'NONE',  ( 1.820119372073704112, 23.17972341190215246, -230.7270437017659503 ) ) ;
#2299=CARTESIAN_POINT ( 'NONE',  ( 2.508382434586714282, 15.09451298870656011, -220.9010239894319625 ) ) ;
#2300=CARTESIAN_POINT ( 'NONE',  ( -26.87016840655871874, 6.086699737350822481, -222.9228935003981746 ) ) ;
#2301=CARTESIAN_POINT ( 'NONE',  ( 13.72784977962315267, 2.687686193488206143, -220.8507880271885995 ) ) ;
#2302=CARTESIAN_POINT ( 'NONE',  ( 9.009845654114897684, -15.13764346805314354, -231.2790349225496129 ) ) ;
#2305=CARTESIAN_POINT ( 'NONE',  ( 8.329997790135040603, 12.51216704542961899, -228.7022893680961602 ) ) ;
#2306=CARTESIAN_POINT ( 'NONE',  ( 17.64863983146639015, -7.217312291206318342, -219.9249463058993399 ) ) ;
#2308=CARTESIAN_POINT ( 'NONE',  ( 0.04660897052267574947, -31.13860575300111577, -224.7746869833732717 ) ) ;
#2310=CARTESIAN_POINT ( 'NONE',  ( -11.42613629117093765, 28.09170287990588832, -228.7150250545069241 ) ) ;
#2311=CARTESIAN_POINT ( 'NONE',  ( -8.413706464639300719, 10.92140547936800843, -220.6417935981040728 ) ) ;
#2312=B_SPLINE_CURVE_WITH_KNOTS ( 'NONE', 3,
 ( #6129, #20177, #6355, #11319, #12896, #11207, #2751, #13227, #9632, #16494, #1183, #18073, #8061, #2645, #8510, #18736, #4887, #22220, #3302, #7036, #20630, #15146, #49, #5217, #12205, #15587, #9968, #3528, #10186, #17055, #17269, #15373, #13677, #1842, #165, #3193, #16827, #1405, #12098, #8615, #21988, #15476, #1517, #10076, #15263, #5324, #16941, #18845, #6811, #13791, #20514, #13907, #6922, #4996, #8720, #3085, #6699, #18953, #20407, #11872, #1633, #6581, #5104, #8277, #10408, #20743, #13451, #20292, #11767, #18631, #11984, #8395, #22113, #13571, #3421, #10300, #17164, #1741, #3860, #10741, #10959, #1957, #17606, #12317, #3970, #2173, #7372, #7585, #19495, #14129, #8836, #2283, #17499, #19170, #8946, #21286, #3747, #12540, #498, #7479, #14241, #17382, #10843, #20851, #9052, #17831, #5553, #16031, #16138, #17718, #9168, #19387, #9278, #15920, #21074, #2066, #5662, #10632, #15812, #605, #20965, #388, #5882, #7257, #14349, #21181, #12433, #5766, #19283, #19059, #710, #12648, #14452, #4082, #2394, #3635, #7148, #10516, #14014, #15702, #279, #5433, #16687, #15008, #11178, #11507, #933, #18375, #19714, #4193, #11288, #18269, #16467, #21847, #11070, #12758, #2938, #1267, #6328, #6214, #13089, #19935, #17939, #12867, #9826, #4633, #18044, #8143, #9381, #4523, #20045, #4406, #19608, #2503, #16355, #2614, #7916, #9495, #19820, #4296, #7811, #14676, #11401, #21510, #16242, #6101, #18159, #2831, #12973, #9713, #2724, #819, #7698, #16573, #14567, #9605, #1044, #21621, #21403, #21736, #5994, #14780, #1154, #8031, #14897, #13201, #1605, #12071, #13764, #22081, #15558, #6670, #20602, #8483, #5189, #10161, #10380, #4741, #18928, #6552, #17140, #22195, #6782, #8692, #13306, #6437, #20487, #1814, #16913, #11847, #18712, #8591, #6894, #5078, #24, #20148, #3503, #20264, #17243, #3392, #8366, #11958, #21959, #11619, #10051, #18606, #18492, #13543, #3052, #3275, #9942, #16802, #10274, #1376, #8252, #15120, #13424, #20378, #4861, #1715, #15452, #11738, #3167, #1488, #15236, #4971, #18820, #17030, #15346, #13652, #15674, #7347, #14101, #10717, #10933, #579, #17472, #5297, #5638, #20825, #254, #12405, #17804, #12622, #2371, #19364, #9253, #3945, #20716, #14213, #1931, #20939, #14322, #8921, #10821, #19468, #21048, #12514, #472, #4058, #5526, #21155, #3836, #138, #12178, #5743, #7122, #17691, #2149, #7006, #19256, #15893, #19032, #13988, #13878, #3610, #5405, #10488, #17354, #2260, #7454, #16004, #8811, #12289, #19141, #3721, #9142, #2043, #10603, #15787, #366, #7233, #17583, #9029, #18020, #11047, #9582, #8003, #21484, #9471 ),
 .UNSPECIFIED., .F., .F.,
 ( 4, 2, 2, 2, 2, 2, 2, 2, 2, 2, 2, 2, 2, 2, 2, 2, 2, 2, 2, 2, 2, 2, 2, 2, 2, 2, 2, 2, 2, 2, 2, 2, 2, 2, 2, 2, 2, 2, 2, 2, 2, 2, 2, 2, 2, 2, 2, 2, 2, 2, 2, 2, 2, 2, 2, 2, 2, 2, 2, 2, 2, 2, 2, 2, 2, 2, 2, 2, 2, 2, 2, 2, 2, 2, 2, 2, 2, 2, 2, 2, 2, 2, 2, 2, 2, 2, 2, 2, 2, 2, 2, 2, 2, 2, 2, 2, 2, 2, 2, 2, 2, 2, 2, 2, 2, 2, 2, 2, 2, 2, 2, 2, 2, 2, 2, 2, 2, 2, 2, 2, 2, 2, 2, 2, 2, 2, 2, 2, 2, 2, 2, 2, 2, 2, 2, 2, 2, 2, 2, 2, 2, 2, 2, 2, 2, 2, 2, 2, 2, 2, 2, 2, 2, 2, 2, 2, 2, 2, 2, 2, 2, 2, 2, 2, 2, 2, 2, 2, 2, 4 ),
 ( 0.4999446919652688059, 0.5028747035357847839, 0.5058047151063008728, 0.5087347266768169618, 0.5116647382473329397, 0.5145947498178489177, 0.5175247613883648956, 0.5204547729588808735, 0.5233847845293969625, 0.5268031313616656774, 0.5285123047777999794, 0.5302214781939342814, 0.5336398250262029963, 0.5353489984423374093, 0.5370581718584717112, 0.5404765186907403152, 0.5438948655230090301, 0.5473132123552777450, 0.5507315591875463490, 0.5541499060198149529, 0.5575682528520836678, 0.5609865996843523828, 0.5644049465166209867, 0.5661141199327552886, 0.5678232933488895906, 0.5712416401811581945, 0.5729508135972924965, 0.5746599870134267984, 0.5780783338456955134, 0.5814966806779642283, 0.5849150275102328322, 0.5883333743425015472, 0.5917517211747702621, 0.5951700680070388660, 0.5985884148393075810, 0.6020067616715762959, 0.6037159350877105979, 0.6054251085038448998, 0.6088434553361135038, 0.6122618021683822187, 0.6139709755845166317, 0.6156801490006509336, 0.6190984958329195376, 0.6225168426651882525, 0.6259351894974569674, 0.6293535363297255714, 0.6327718831619942863, 0.6361902299942630012, 0.6396085768265316052, 0.6430269236588003201, 0.6447360970749347331, 0.6464452704910690350, 0.6498636173233376390, 0.6532819641556063539, 0.6549911375717407669, 0.6567003109878750688, 0.6601186578201436728, 0.6635370046524122767, 0.6669553514846809916, 0.6703736983169497066, 0.6737920451492183105, 0.6772103919814870254, 0.6806287388137557404, 0.6840470856460243443, 0.6857562590621586462, 0.6866108457702257972, 0.6874654324782930592, 0.6908837793105617742, 0.6943021261428303781, 0.6960112995589646800, 0.6977204729750989820, 0.7011388198073676969, 0.7045571666396364119, 0.7079755134719050158, 0.7113938603041736197, 0.7148122071364423347, 0.7182305539687110496, 0.7216489008009796535, 0.7250672476332483685, 0.7267764210493827814, 0.7284855944655170834, 0.7319039412977856873, 0.7353222881300544023, 0.7387406349623231172, 0.7421589817945917211, 0.7455773286268603250, 0.7489956754591290400, 0.7524140222913977549, 0.7558323691236663588, 0.7592507159559350738, 0.7626690627882037887, 0.7660874096204723926, 0.7695057564527411076, 0.7729241032850098225, 0.7763424501172784264, 0.7797607969495471414, 0.7831791437818158563, 0.7865974906140844602, 0.7900158374463531752, 0.7934341842786218901, 0.7968525311108904940, 0.8002708779431590980, 0.8036892247754278129, 0.8053983981915622259, 0.8071075716076965278, 0.8105259184399651318, 0.8122350918560994337, 0.8139442652722337357, 0.8173626121045024506, 0.8207809589367711656, 0.8241993057690397695, 0.8276176526013083734, 0.8310359994335770883, 0.8344543462658458033, 0.8378726930981144072, 0.8412910399303831221, 0.8430002133465175351, 0.8447093867626518371, 0.8481277335949204410, 0.8515460804271891559, 0.8549644272594578709, 0.8583827740917264748, 0.8618011209239951897, 0.8652194677562639047, 0.8686378145885325086, 0.8720561614208012235, 0.8754745082530699385, 0.8788928550853385424, 0.8823112019176071463, 0.8857295487498758613, 0.8874387221660102743, 0.8891478955821445762, 0.8925662424144131801, 0.8942754158305474821, 0.8959845892466818951, 0.8994029360789506100, 0.9028212829112192139, 0.9062396297434879289, 0.9096579765757566438, 0.9130763234080252477, 0.9164946702402939627, 0.9199130170725626776, 0.9233313639048312815, 0.9250405373209655835, 0.9267497107370999965, 0.9301680575693687114, 0.9335864044016373153, 0.9352955778177716173, 0.9370047512339059192, 0.9404230980661746342, 0.9438414448984433491, 0.9472597917307119531, 0.9506781385629806680, 0.9540964853952493829, 0.9575148322275179869, 0.9609331790597867018, 0.9643515258920554167, 0.9660606993081897187, 0.9677698727243240207, 0.9711882195565927356, 0.9728973929727271486, 0.9746065663888614505, 0.9780249132211300545, 0.9814432600533987694, 0.9848616068856674843, 0.9882799537179360883, 0.9912099652884520662, 0.9941399768589680441, 0.9970699884294840221, 1.000000000000000000 ),
 .UNSPECIFIED. ) ;
#2313=CARTESIAN_POINT ( 'NONE',  ( -8.172572110426221670, 16.86653848210977813, -233.4220330256369493 ) ) ;
#2314=CARTESIAN_POINT ( 'NONE',  ( -14.03072379416114757, -18.13329758221107824, -232.5220584501505812 ) ) ;
#2317=CARTESIAN_POINT ( 'NONE',  ( -7.429838964355703901, 14.87322129099639234, -232.2632863647814077 ) ) ;
#2318=CARTESIAN_POINT ( 'NONE',  ( 3.810076078852552950, -13.18001539772800612, -226.2402971015400510 ) ) ;
#2320=CARTESIAN_POINT ( 'NONE',  ( -21.02719846458807851, 18.12262440796364871, -218.0220709499931502 ) ) ;
#2322=CARTESIAN_POINT ( 'NONE',  ( 13.80707869872719762, 6.429545566348308760, -225.7152177910682553 ) ) ;
#2323=CARTESIAN_POINT ( 'NONE',  ( -23.95129667199961077, 20.99391807043993552, -227.1541646794576081 ) ) ;
#2325=CARTESIAN_POINT ( 'NONE',  ( 16.01130065545721592, 20.79417322911648114, -220.9619135886794652 ) ) ;
#2326=CARTESIAN_POINT ( 'NONE',  ( -7.589660848220153078, -14.86992855705293692, -228.0480809167547136 ) ) ;
#2328=CARTESIAN_POINT ( 'NONE',  ( -3.223980134944351317, 26.83284996841001302, -219.5167893230652965 ) ) ;
#2329=CARTESIAN_POINT ( 'NONE',  ( -12.80756961294691010, 26.82110654133967387, -223.7464923486294026 ) ) ;
#2330=CARTESIAN_POINT ( 'NONE',  ( -18.17591565587962776, 16.23604867791855355, -233.2845329962925121 ) ) ;
#2332=CARTESIAN_POINT ( 'NONE',  ( -16.14140970932308505, -18.57031478189210816, -230.2506069696216287 ) ) ;
#2336=CARTESIAN_POINT ( 'NONE',  ( -14.10849459794400751, -0.2436790717799666162, -223.1085195285415921 ) ) ;
#2337=CARTESIAN_POINT ( 'NONE',  ( 7.240923751923983964, -14.90955521745277501, -222.5312387745455283 ) ) ;
#2338=CARTESIAN_POINT ( 'NONE',  ( 14.85123888640019452, 5.067529763532427012, -221.9058491819374979 ) ) ;
#2339=CARTESIAN_POINT ( 'NONE',  ( -0.3969026096611234511, 20.89748314411456676, -216.3289738411752978 ) ) ;
#2340=CARTESIAN_POINT ( 'NONE',  ( 18.50073117969547098, -1.889592114545683987, -232.6396648696776026 ) ) ;
#2341=CARTESIAN_POINT ( 'NONE',  ( 11.78717493688862206, 28.63884142527983556, -229.7724827508652652 ) ) ;
#2342=CARTESIAN_POINT ( 'NONE',  ( 10.83706092800007781, 10.12544885278926543, -227.1716144446442343 ) ) ;
#2345=CARTESIAN_POINT ( 'NONE',  ( -12.42894476027428929, -17.97759322220185396, -216.3110355466728834 ) ) ;
#2347=CARTESIAN_POINT ( 'NONE',  ( 8.021672912688133650, -23.92397517040199872, -233.3380040120402441 ) ) ;
#2350=CARTESIAN_POINT ( 'NONE',  ( -11.80036766549451599, 3.629178540272184783, -221.4826559383200220 ) ) ;
#2351=CARTESIAN_POINT ( 'NONE',  ( -19.94082127283490280, -7.534429669270808816, -230.8553971038493557 ) ) ;
#2352=CARTESIAN_POINT ( 'NONE',  ( -17.49393085256189906, 10.63366922396483361, -217.7502683347138657 ) ) ;
#2353=CARTESIAN_POINT ( 'NONE',  ( 23.22505041959077232, 19.39625294115234055, -221.5972645870541555 ) ) ;
#2354=CARTESIAN_POINT ( 'NONE',  ( 17.35243190875273811, 16.67741344734974263, -230.5744436858935558 ) ) ;
#2356=CARTESIAN_POINT ( 'NONE',  ( 7.445043070300236820, -12.68569377707410339, -219.2962123921901991 ) ) ;
#2357=CARTESIAN_POINT ( 'NONE',  ( 12.71450444683213021, 7.595266944807587350, -224.4213778964231665 ) ) ;
#2359=CARTESIAN_POINT ( 'NONE',  ( -4.695076324262313250, 31.85502299853856201, -223.8918597786031341 ) ) ;
#2360=CARTESIAN_POINT ( 'NONE',  ( -4.365576370787875859, 13.02741211227440665, -230.2897948137907917 ) ) ;
#2361=CARTESIAN_POINT ( 'NONE',  ( -28.12632608809566293, -1.403418003803144742, -218.5233027210585988 ) ) ;
#2362=CARTESIAN_POINT ( 'NONE',  ( -25.80904414196669450, 12.19501778665756220, -219.1732313092283846 ) ) ;
#2366=CARTESIAN_POINT ( 'NONE',  ( 27.32546652195855685, -7.354568365469916991, -229.0866163655393279 ) ) ;
#2367=CARTESIAN_POINT ( 'NONE',  ( 1.984991703947643904, 14.51738422979996912, -218.4500278854917781 ) ) ;
#2368=CARTESIAN_POINT ( 'NONE',  ( 14.81251837262747983, -1.020578734748967209, -221.0290343291311785 ) ) ;
#2369=CARTESIAN_POINT ( 'NONE',  ( 15.70515172005171323, -0.7403987186381333352, -226.4590404369862995 ) ) ;
#2370=CARTESIAN_POINT ( 'NONE',  ( 4.543450689403089271, 15.91052110650461771, -218.9437823786444426 ) ) ;
#2371=CARTESIAN_POINT ( 'NONE',  ( -16.38803511840525218, -9.809678413005567421, -217.1940421839195494 ) ) ;
#2372=CARTESIAN_POINT ( 'NONE',  ( -2.043230952238195286, 23.63069326910348877, -232.6835180461029040 ) ) ;
#2373=CARTESIAN_POINT ( 'NONE',  ( -1.608171596096409806, -16.77465153034988887, -217.4618546331240054 ) ) ;
#2374=CARTESIAN_POINT ( 'NONE',  ( 13.61707622192329481, 14.84143455326118932, -217.6958999636067063 ) ) ;
#2375=CARTESIAN_POINT ( 'NONE',  ( 20.24215890739238688, -18.92204689856563249, -233.5548650425709241 ) ) ;
#2377=CARTESIAN_POINT ( 'NONE',  ( -12.43544732248594720, 12.69828336922617318, -219.3367909706387877 ) ) ;
#2379=CARTESIAN_POINT ( 'NONE',  ( -26.22128172021140813, -2.843310382428120064, -218.3980250098940132 ) ) ;
#2380=CARTESIAN_POINT ( 'NONE',  ( 6.608541902967795423, 16.43938546752961116, -220.2982508316308952 ) ) ;
#2381=CARTESIAN_POINT ( 'NONE',  ( -16.28025842329327944, 6.985656672962045732, -231.4191468057695715 ) ) ;
#2382=CARTESIAN_POINT ( 'NONE',  ( 25.80927844399814930, 11.21489550116160316, -221.3538377621514996 ) ) ;
#2383=CARTESIAN_POINT ( 'NONE',  ( -7.215839073791710412, -12.32959168003491968, -224.1142876912989834 ) ) ;
#2384=CARTESIAN_POINT ( 'NONE',  ( 17.85905871012913693, 8.463974683125162102, -234.6532732619751300 ) ) ;
#2385=CARTESIAN_POINT ( 'NONE',  ( -10.53630953054794794, -7.637555647514923329, -229.7964863767589918 ) ) ;
#2386=CARTESIAN_POINT ( 'NONE',  ( 5.955271202636533090, 21.50135983300913267, -233.0184468368920534 ) ) ;
#2387=CARTESIAN_POINT ( 'NONE',  ( 27.79746884017060538, 13.63637251724950339, -226.5788410723774575 ) ) ;
#2388=CARTESIAN_POINT ( 'NONE',  ( -9.852301241816233457, 15.10013604187968461, -230.8124578431014697 ) ) ;
#2390=CARTESIAN_POINT ( 'NONE',  ( -3.687581766460184429, 30.01855770642711718, -218.8323691868875187 ) ) ;
#2391=CARTESIAN_POINT ( 'NONE',  ( -20.26851768784797869, -0.8260594303982465858, -217.1279713726092098 ) ) ;
#2393=CARTESIAN_POINT ( 'NONE',  ( 0.3833872033527188639, -14.95856321834011915, -223.3240416624371107 ) ) ;
#2394=CARTESIAN_POINT ( 'NONE',  ( 4.823266655078461085, -13.86048651889774241, -224.7145696108100026 ) ) ;
#2397=CARTESIAN_POINT ( 'NONE',  ( 14.54149994592679107, 8.070685273005897997, -229.7292930672863349 ) ) ;
#2398=CARTESIAN_POINT ( 'NONE',  ( -13.36635042947306573, -0.3940246778032021058, -227.3384152261055249 ) ) ;
#2400=CARTESIAN_POINT ( 'NONE',  ( -17.58118739749173898, -8.238107657346720458, -217.5252134542318458 ) ) ;
#2401=CARTESIAN_POINT ( 'NONE',  ( 8.257114973007913861, -25.39836461225790742, -232.6217252414676295 ) ) ;
#2402=CARTESIAN_POINT ( 'NONE',  ( 12.83388873239664996, 22.07510045760132655, -230.4740059944613222 ) ) ;
#2404=CARTESIAN_POINT ( 'NONE',  ( -12.88152464663890306, 6.317716727793897924, -230.5294309895745073 ) ) ;
#2405=CARTESIAN_POINT ( 'NONE',  ( -7.429838964355703901, 14.87322129099639234, -232.2632863647814077 ) ) ;
#2406=CARTESIAN_POINT ( 'NONE',  ( 3.325336547283623378, 18.92213121405483633, -219.7480163085221818 ) ) ;
#2407=CARTESIAN_POINT ( 'NONE',  ( 24.67321061357916889, 1.914345543126667826, -232.4367140101115581 ) ) ;
#2408=ORIENTED_EDGE ( 'NONE', *, *, #21324, .T. ) ;
#2409=CARTESIAN_POINT ( 'NONE',  ( 11.09231067055629616, 7.417581979752235100, -227.5152062457793534 ) ) ;
#2410=CARTESIAN_POINT ( 'NONE',  ( -15.95412330064426065, 13.09400588185824077, -218.6613039563597169 ) ) ;
#2411=CARTESIAN_POINT ( 'NONE',  ( 14.96462366732929716, 7.179279272144128754, -233.2042342402542374 ) ) ;
#2412=CARTESIAN_POINT ( 'NONE',  ( -7.180402128846711918, -26.42159752827261698, -220.2116303544826224 ) ) ;
#2414=EDGE_LOOP ( 'NONE', ( #22124, #8855 ) ) ;
#2415=CARTESIAN_POINT ( 'NONE',  ( 3.763426558366607111, 28.60172112197566818, -230.1816715025297526 ) ) ;
#2416=CARTESIAN_POINT ( 'NONE',  ( 15.78601976571614962, -10.64697985159532401, -219.7411765650222151 ) ) ;
#2417=CARTESIAN_POINT ( 'NONE',  ( -22.10934047915427314, 0.9940043559354312386, -216.9999999999999716 ) ) ;
#2418=CARTESIAN_POINT ( 'NONE',  ( 7.958080982411646076, -16.12895853103474408, -217.0903302464454612 ) ) ;
#2420=CARTESIAN_POINT ( 'NONE',  ( -1.249406995060579062, 25.48934319316224162, -216.9406480707515072 ) ) ;
#2421=CARTESIAN_POINT ( 'NONE',  ( -11.10182655035041144, 8.778638955377752850, -227.1050196202568827 ) ) ;
#2423=CARTESIAN_POINT ( 'NONE',  ( -17.65835845419170624, 22.55329142274348442, -231.2673511165784532 ) ) ;
#2424=CARTESIAN_POINT ( 'NONE',  ( -14.26331330459994540, -11.99770975811722451, -232.1846756268951708 ) ) ;
#2427=CARTESIAN_POINT ( 'NONE',  ( -3.501680520304516264, 14.31538576447642264, -219.8967178229432307 ) ) ;
#2428=CARTESIAN_POINT ( 'NONE',  ( 1.145088139557171036, -28.55736460288477119, -218.6379321102267284 ) ) ;
#2429=CARTESIAN_POINT ( 'NONE',  ( 14.21523762536935820, -1.512798260419094598, -222.4093369397272397 ) ) ;
#2430=CARTESIAN_POINT ( 'NONE',  ( -14.00380962569832199, 8.747390586476997854, -231.7950903513155936 ) ) ;
#2431=CARTESIAN_POINT ( 'NONE',  ( -19.26845014167239611, 9.481468541508135672, -234.4856117705182328 ) ) ;
#2432=CARTESIAN_POINT ( 'NONE',  ( -9.060295054034883222, 29.20313342278041802, -224.2979742714222482 ) ) ;
#2434=CARTESIAN_POINT ( 'NONE',  ( 21.15841376125116824, 4.865517895153391947, -217.1795922978051578 ) ) ;
#2435=CARTESIAN_POINT ( 'NONE',  ( -6.842387616420496421, -14.58019248909694632, -223.2484495378617453 ) ) ;
#2437=CARTESIAN_POINT ( 'NONE',  ( 5.955271202636533090, 21.50135983300913267, -233.0184468368920534 ) ) ;
#2438=CARTESIAN_POINT ( 'NONE',  ( -14.22959263369750182, 18.28478771081826793, -217.8090497856120464 ) ) ;
#2439=CARTESIAN_POINT ( 'NONE',  ( -9.403561938624596550, 12.70246821120386471, -220.7484614495429582 ) ) ;
#2441=CARTESIAN_POINT ( 'NONE',  ( 28.19769730429874599, -1.268543021275377658, -231.5188709829604363 ) ) ;
#2444=CARTESIAN_POINT ( 'NONE',  ( -13.69675006931110417, 3.702342960760605539, -228.0723273272095355 ) ) ;
#2445=CARTESIAN_POINT ( 'NONE',  ( 7.487558183825500535, -19.68056729374139380, -230.9679144533258466 ) ) ;
#2446=CARTESIAN_POINT ( 'NONE',  ( 14.32085100525799248, 9.220655089380342062, -219.9006227404039464 ) ) ;
#2447=CARTESIAN_POINT ( 'NONE',  ( -3.755296588130283553, 23.77975947300719284, -233.7323173085780752 ) ) ;
#2449=CARTESIAN_POINT ( 'NONE',  ( -16.90857133559978465, -0.4126725064255206687, -221.6276144895144569 ) ) ;
#2450=CARTESIAN_POINT ( 'NONE',  ( 7.803634760976553508, 10.78293796201124266, -229.6314106675118865 ) ) ;
#2451=CARTESIAN_POINT ( 'NONE',  ( 12.99034161053428349, 11.71468708507361889, -230.9043293568357740 ) ) ;
#2454=CARTESIAN_POINT ( 'NONE',  ( -6.870552667427666904, -18.85419487977974029, -216.2130481585807047 ) ) ;
#2455=CARTESIAN_POINT ( 'NONE',  ( 15.10937218716165020, -26.44221868192832758, -222.7999243300199907 ) ) ;
#2458=CARTESIAN_POINT ( 'NONE',  ( -8.328662059352005542, 28.53523473722178139, -221.4280032538016201 ) ) ;
#2459=CARTESIAN_POINT ( 'NONE',  ( 14.54962894845190036, -2.357901078066860112, -232.0046840244626765 ) ) ;
#2460=CARTESIAN_POINT ( 'NONE',  ( 27.96460686140487084, -1.872811165202790340, -220.9791906660856000 ) ) ;
#2461=CARTESIAN_POINT ( 'NONE',  ( 19.40629804599390340, 15.10110417999774057, -216.3942729496570223 ) ) ;
#2462=CARTESIAN_POINT ( 'NONE',  ( 11.40028598017942230, 13.60807601628675023, -220.9105305289655519 ) ) ;
#2464=CARTESIAN_POINT ( 'NONE',  ( 22.27668549480667792, -16.40903445915953895, -216.4638184065479152 ) ) ;
#2467=CARTESIAN_POINT ( 'NONE',  ( -2.218529449563984901, 24.06491599887877442, -214.8915873797660652 ) ) ;
#2468=CARTESIAN_POINT ( 'NONE',  ( -5.543543819386913540, 14.51457927969963713, -217.3847528063896846 ) ) ;
#2469=CARTESIAN_POINT ( 'NONE',  ( -12.65123680455331190, -6.798726433138870817, -228.2089845657881710 ) ) ;
#2470=CARTESIAN_POINT ( 'NONE',  ( -18.70100282803782576, 16.58357028540773115, -216.4425743468854080 ) ) ;
#2473=CARTESIAN_POINT ( 'NONE',  ( 18.22947608839760747, -6.525328669204546905, -217.7409786913911205 ) ) ;
#2474=CARTESIAN_POINT ( 'NONE',  ( -1.406618399933933006, 16.47239985789244443, -232.2564017133012726 ) ) ;
#2475=CARTESIAN_POINT ( 'NONE',  ( 20.92846067405557520, -2.114533307883533109, -233.2756072794335580 ) ) ;
#2476=CARTESIAN_POINT ( 'NONE',  ( -11.49049084071896409, 11.06834963248926940, -218.3354249205727058 ) ) ;
#2477=CARTESIAN_POINT ( 'NONE',  ( 15.33737796850231305, 13.57479350230705428, -232.3313557812109025 ) ) ;
#2479=CARTESIAN_POINT ( 'NONE',  ( 5.142103055192286831, 28.18228231877369439, -225.8998064704803994 ) ) ;
#2480=CARTESIAN_POINT ( 'NONE',  ( -16.21268175593173311, -5.852138355245464219, -231.1837890105803410 ) ) ;
#2481=CARTESIAN_POINT ( 'NONE',  ( 26.29894631880581812, 12.29609390142961090, -226.3100047295820332 ) ) ;
#2482=B_SPLINE_CURVE_WITH_KNOTS ( 'NONE', 3,
 ( #2417, #2636, #11093, #2744, #956, #14695, #12671, #13109, #7719, #9299, #16486, #19519, #17960, #4105, #10983, #14590, #12992, #1063, #7936, #21425, #21308, #14800, #21642, #6236, #2849, #4762, #1733, #3411, #20397, #4988, #6689, #22211, #1396, #18396, #13220, #9960, #15255, #13563, #6457, #3184, #9847, #8500, #18837, #10068, #10291, #1507, #21978, #8162, #16932, #6572, #11863, #16708, #3072, #3293, #8607, #11639, #13326, #18510, #17157, #11976, #20504, #5095, #18623, #8387, #15467, #6348, #20168, #20065, #4653, #15365, #18728, #2961, #10178, #8270, #1288, #13443, #15137, #22101, #11526, #15028, #17047, #16819, #21867, #20283, #1623, #4878, #11757, #6801, #13669, #17490, #20956, #21067, #3961, #17709, #12088, #14232, #3626, #5205, #19161, #5544, #7364, #3737, #3519, #12195, #10399, #10621, #18944, #20622, #12532, #19051, #269, #17259, #10836, #5313, #2277, #2058, #491, #10505, #1831, #8709, #9160, #381, #12306, #15576, #41, #6912, #20733, #5655, #17372, #19380, #7024, #13783, #8936, #1947, #155, #12423, #13896, #8826, #15691, #7139, #15803, #14005, #19274, #20841, #5424, #7249, #14120, #3853, #10733, #17598, #2165, #9045, #15911, #21503, #11394, #9375, #19600, #5872, #924, #7692, #16235, #2826, #4187, #6093, #11063, #17933, #2495, #17824, #12862, #811, #7804, #19486, #12752, #12968, #18262, #21279, #16129, #14560, #13083, #21614, #7911, #16022, #21172, #21396, #9271, #14669, #5988, #4291, #4514, #16462, #19706, #5759, #19813, #19928, #14444, #7470, #597, #702, #9488, #11170, #4397, #18038, #2386, #2606, #12639, #7578, #4076, #16350, #14339, #10951, #11282, #18152, #2717, #9599, #1037, #14774, #6205, #13300, #18598, #16906, #9817, #1370, #20481, #11841, #10154, #20256, #20141, #9933, #14888, #8359, #8022, #4964, #1482, #5072, #16795, #4734, #15340, #11950, #6776, #6431, #17022, #4853, #16680, #8246, #6664, #11730, #22188, #1598, #3046, #18813, #15114, #8477, #4626, #16566, #21951, #1146, #21729, #13645, #1260, #20372, #13535, #11611, #18483, #6320, #9706, #15229, #13194, #6544, #13415, #3161, #18706, #20039, #11500, #2930, #10045, #3269, #8135, #18369, #15001, #22074, #21839, #18922, #465, #6999, #15551, #10712, #10481, #17237, #1924, #20595, #15447, #2144, #10374, #17134, #5398, #1808, #3497, #8915, #1709, #5634, #9024, #14094, #7228, #8685, #15782, #17, #8584, #130, #15886, #17577, #13872, #7341, #6887, #19134, #13757, #360, #21044, #19027, #20711, #5292, #10596, #12172, #14208, #12510, #3604, #20933, #17346, #8805 ),
 .UNSPECIFIED., .F., .F.,
 ( 4, 2, 2, 2, 2, 2, 2, 2, 2, 2, 2, 2, 2, 2, 2, 2, 2, 2, 2, 2, 2, 2, 2, 2, 2, 2, 2, 2, 2, 2, 2, 2, 2, 2, 2, 2, 2, 2, 2, 2, 2, 2, 2, 2, 2, 2, 2, 2, 2, 2, 2, 2, 2, 2, 2, 2, 2, 2, 2, 2, 2, 2, 2, 2, 2, 2, 2, 2, 2, 2, 2, 2, 2, 2, 2, 2, 2, 2, 2, 2, 2, 2, 2, 2, 2, 2, 2, 2, 2, 2, 2, 2, 2, 2, 2, 2, 2, 2, 2, 2, 2, 2, 2, 2, 2, 2, 2, 2, 2, 2, 2, 2, 2, 2, 2, 2, 2, 2, 2, 2, 2, 2, 2, 2, 2, 2, 2, 2, 2, 2, 2, 2, 2, 2, 2, 2, 2, 2, 2, 2, 2, 2, 2, 2, 2, 2, 2, 2, 2, 2, 2, 2, 2, 2, 2, 2, 2, 2, 2, 2, 2, 2, 2, 4 ),
 ( 0.000000000000000000, 0.001952908952989333875, 0.003905817905978667751, 0.007323408573709997045, 0.01074099924144132634, 0.01415858990917265650, 0.01586738524303832332, 0.01757618057690398666, 0.02099377124463531682, 0.02441136191236664699, 0.02782895258009797368, 0.03124654324782930384, 0.03466413391556063400, 0.03808172458329196070, 0.04149931525102329433, 0.04491690591875462102, 0.04662570125262028436, 0.04833449658648594771, 0.05175208725421727440, 0.05346088258808293775, 0.05516967792194860110, 0.05858726858967993473, 0.06200485925741126836, 0.06542244992514259505, 0.06884004059287393562, 0.07225763126060526231, 0.07567522192833658901, 0.07909281259606792958, 0.08251040326379925627, 0.08421919859766491268, 0.08592799393153058296, 0.08934558459926195129, 0.09276317526699331961, 0.09447197060085900377, 0.09618076593472468794, 0.09959835660245604239, 0.1030159472701873968, 0.1064335379379187652, 0.1098511286056501335, 0.1132687192733815018, 0.1166863099411127869, 0.1201039006088440858, 0.1235214912765753847, 0.1252302866104410273, 0.1269390819443066698, 0.1303566726120379826, 0.1320654679459036251, 0.1337742632797692677, 0.1371918539475005527, 0.1406094446152318378, 0.1440270352829631784, 0.1474446259506944912, 0.1508622166184258040, 0.1542798072861571446, 0.1576973979538884851, 0.1611149886216198257, 0.1645325792893511663, 0.1679501699570824791, 0.1713677606248137919, 0.1747853512925451325, 0.1764941466264108028, 0.1782029419602764730, 0.1816205326280078136, 0.1850381232957391542, 0.1884557139634704670, 0.1918733046312017798, 0.1952908952989331204, 0.1987084859666644610, 0.2021260766343957738, 0.2055436673021270866, 0.2072524626359927569, 0.2089612579698584272, 0.2123788486375897677, 0.2140876439714554380, 0.2157964393053211083, 0.2192140299730524489, 0.2226316206407837617, 0.2260492113085151300, 0.2294668019762464706, 0.2328843926439778111, 0.2363019833117091517, 0.2397195739794404923, 0.2431371646471718329, 0.2465547553149031734, 0.2499723459826345140, 0.2533899366503657991, 0.2568075273180971396, 0.2602251179858284802, 0.2636427086535597653, 0.2670602993212909948, 0.2704778899890223909, 0.2738954806567537315, 0.2773130713244850165, 0.2807306619922163571, 0.2841482526599476977, 0.2858570479938133957, 0.2875658433276790382, 0.2909834339954103788, 0.2926922293292760768, 0.2944010246631417194, 0.2978186153308730599, 0.3012362059986043450, 0.3046537966663356856, 0.3080713873340670261, 0.3114889780017983112, 0.3149065686695296518, 0.3183241593372609923, 0.3217417500049923329, 0.3234505453388579754, 0.3251593406727236735, 0.3285769313404549585, 0.3319945220081862991, 0.3354121126759176397, 0.3388297033436489247, 0.3422472940113802653, 0.3456648846791116059, 0.3490824753468429464, 0.3525000660145742870, 0.3559176566823056276, 0.3593352473500369682, 0.3627528380177683087, 0.3661704286854996493, 0.3695880193532309343, 0.3730056100209622749, 0.3747144053548279174, 0.3764232006886936155, 0.3798407913564249005, 0.3832583820241562411, 0.3866759726918875817, 0.3900935633596189223, 0.3935111540273502628, 0.3969287446950816034, 0.4003463353628129440, 0.4037639260305442845, 0.4054727213644099271, 0.4071815166982756251, 0.4105991073660069102, 0.4140166980337382507, 0.4157254933676038933, 0.4174342887014695913, 0.4208518793692008764, 0.4242694700369322169, 0.4276870607046635575, 0.4311046513723948981, 0.4345222420401262386, 0.4379398327078575237, 0.4413574233755888643, 0.4447750140433202048, 0.4464838093771859029, 0.4481926047110515454, 0.4516101953787828860, 0.4533189907126485840, 0.4550277860465142266, 0.4584453767142455671, 0.4618629673819769077, 0.4652805580497082483, 0.4686981487174395888, 0.4721157393851709294, 0.4755333300529022145, 0.4789509207206334995, 0.4823685113883648956, 0.4840773067222305381, 0.4857861020560961807, 0.4878404479772363023 ),
 .UNSPECIFIED. ) ;
#2483=CARTESIAN_POINT ( 'NONE',  ( -0.1874296312810625753, -16.87674362306512776, -233.1597105263269611 ) ) ;
#2485=CARTESIAN_POINT ( 'NONE',  ( -13.70798801564395752, 13.71024986321384809, -218.3360451569033955 ) ) ;
#2487=CARTESIAN_POINT ( 'NONE',  ( -25.99367553232993799, -4.794975032520305547, -231.0351783075731191 ) ) ;
#2488=CARTESIAN_POINT ( 'NONE',  ( 3.191455400233187412, 17.67480163422566619, -220.7055581859663107 ) ) ;
#2489=CARTESIAN_POINT ( 'NONE',  ( -15.36327147092456791, 5.453733681707060299, -220.0043800961136355 ) ) ;
#2490=CARTESIAN_POINT ( 'NONE',  ( -22.04004491965229207, 12.41871177236473578, -215.2165492276571115 ) ) ;
#2491=CARTESIAN_POINT ( 'NONE',  ( -20.29356827505781879, -18.19569389227462253, -221.0297756488607490 ) ) ;
#2492=CARTESIAN_POINT ( 'NONE',  ( 29.08100487150598212, 12.14819438347179670, -226.9621620069135020 ) ) ;
#2494=CARTESIAN_POINT ( 'NONE',  ( -26.37829495954481374, -14.45191861565034053, -218.9345690753252711 ) ) ;
#2495=CARTESIAN_POINT ( 'NONE',  ( -1.301562195391901877, 16.19210386685474390, -220.0867867038183192 ) ) ;
#2496=CARTESIAN_POINT ( 'NONE',  ( 30.52813181070726856, 5.438803974502569361, -223.5441926215666513 ) ) ;
#2497=CARTESIAN_POINT ( 'NONE',  ( -18.64931821476190876, 22.04453097546810270, -226.2485927806324923 ) ) ;
#2498=CARTESIAN_POINT ( 'NONE',  ( 7.174260007897984792, 9.971262771497068300, -226.2872513832048469 ) ) ;
#2501=CARTESIAN_POINT ( 'NONE',  ( 5.786710755275625395, -21.74573425722988063, -218.5323380358915131 ) ) ;
#2503=CARTESIAN_POINT ( 'NONE',  ( -0.1049609700611137120, -29.11428177772140558, -224.8408750893923411 ) ) ;
#2505=CARTESIAN_POINT ( 'NONE',  ( 19.19288224840068935, 10.13059690604263174, -232.1906135022504998 ) ) ;
#2506=CARTESIAN_POINT ( 'NONE',  ( 12.31511859722645852, -8.491226738247512174, -220.9006323875693738 ) ) ;
#2507=CARTESIAN_POINT ( 'NONE',  ( -19.50907964299920039, -17.77536300509877876, -217.8007844881196320 ) ) ;
#2508=CARTESIAN_POINT ( 'NONE',  ( -5.636842872076440081, -13.76003991320737541, -219.7405193562604495 ) ) ;
#2509=CARTESIAN_POINT ( 'NONE',  ( 9.382249691333727881, 26.55946126407900820, -224.4468135941759215 ) ) ;
#2511=CARTESIAN_POINT ( 'NONE',  ( -12.79639481117843935, 1.974037863663017589, -229.6094308443170746 ) ) ;
#2512=CARTESIAN_POINT ( 'NONE',  ( 3.449504654906655254, 27.59247159270940841, -231.3461799890608859 ) ) ;
#2513=CARTESIAN_POINT ( 'NONE',  ( 3.174664235197445006, 17.30896320251298448, -221.0803896709622620 ) ) ;
#2514=CARTESIAN_POINT ( 'NONE',  ( 13.34086609499694553, -4.728578536804411314, -230.1381470621469134 ) ) ;
#2516=CARTESIAN_POINT ( 'NONE',  ( 12.74913679152205148, 9.185760885856177893, -218.6542381594888980 ) ) ;
#2517=CARTESIAN_POINT ( 'NONE',  ( -14.67397018911906770, 9.031553917454052893, -228.4349422195089119 ) ) ;
#2518=CARTESIAN_POINT ( 'NONE',  ( 29.00474534066713872, 11.29707752057770698, -221.8682176444242771 ) ) ;
#2520=CARTESIAN_POINT ( 'NONE',  ( -7.182761810198031505, -27.78193072152378207, -222.3754761716870973 ) ) ;
#2523=CARTESIAN_POINT ( 'NONE',  ( 17.60676319847677007, 21.31475060840986302, -219.8266339603936785 ) ) ;
#2524=CARTESIAN_POINT ( 'NONE',  ( 14.80019294276752007, -6.608272808847591051, -224.1005182637183566 ) ) ;
#2526=CARTESIAN_POINT ( 'NONE',  ( -5.420780812268581883, -12.08122409751860360, -226.5143039284326392 ) ) ;
#2528=CARTESIAN_POINT ( 'NONE',  ( 1.217121169770782663, 15.31158828575123110, -230.6845728599757308 ) ) ;
#2529=CARTESIAN_POINT ( 'NONE',  ( -1.302381543002304687, 18.65968181418110206, -215.1730913991678449 ) ) ;
#2531=CARTESIAN_POINT ( 'NONE',  ( -6.101488798441174310, 11.33371047077072369, -225.3616985956418546 ) ) ;
#2532=CARTESIAN_POINT ( 'NONE',  ( 23.56599333006272445, -4.960096179470117050, -217.5996013647105372 ) ) ;
#2535=CARTESIAN_POINT ( 'NONE',  ( -6.282398543089500187, 12.01615879894893801, -228.5121145169883903 ) ) ;
#2536=CARTESIAN_POINT ( 'NONE',  ( 4.470318609411144450, -14.75491745724135306, -219.7618428768379886 ) ) ;
#2537=CARTESIAN_POINT ( 'NONE',  ( 25.69761320619099720, -8.403105518750903613, -219.2599777650661110 ) ) ;
#2538=CARTESIAN_POINT ( 'NONE',  ( -9.151299407007059017, 9.196974979111923076, -223.9483834032048719 ) ) ;
#2539=CARTESIAN_POINT ( 'NONE',  ( -31.12406087576577463, 7.316399946619934092, -225.0171288978685027 ) ) ;
#2540=CARTESIAN_POINT ( 'NONE',  ( -2.129100187576105530, 26.11057959790866789, -231.5939360033278547 ) ) ;
#2542=CARTESIAN_POINT ( 'NONE',  ( 27.94758519801750296, 7.894658480667867018, -227.3974864124137127 ) ) ;
#2543=CARTESIAN_POINT ( 'NONE',  ( -18.43493186415240714, -20.29552032882516244, -227.2236339120829030 ) ) ;
#2544=CARTESIAN_POINT ( 'NONE',  ( 12.08198696763335178, 15.54678077493410981, -216.6084679670902631 ) ) ;
#2545=CARTESIAN_POINT ( 'NONE',  ( -21.01242583983345469, 16.60754347445175227, -220.8286358486543293 ) ) ;
#2546=CARTESIAN_POINT ( 'NONE',  ( -15.33438615632468149, 23.56248205204123991, -229.2747191038674544 ) ) ;
#2547=CARTESIAN_POINT ( 'NONE',  ( -26.22128172021140813, -2.843310382428120064, -218.3980250098940132 ) ) ;
#2549=ORIENTED_EDGE ( 'NONE', *, *, #7214, .F. ) ;
#2550=CARTESIAN_POINT ( 'NONE',  ( -17.96792326766206926, -0.6237852504629022299, -217.9759415197746932 ) ) ;
#2551=CARTESIAN_POINT ( 'NONE',  ( -3.607128793317693649, -14.45447024314366402, -228.6383918289709811 ) ) ;
#2552=CARTESIAN_POINT ( 'NONE',  ( 13.96368202411823844, 1.657567506656081546, -227.5008844161029629 ) ) ;
#2553=CARTESIAN_POINT ( 'NONE',  ( -4.104500432947460808, 15.73223271406093460, -218.0734292856946297 ) ) ;
#2556=CARTESIAN_POINT ( 'NONE',  ( -15.82952867276381603, 3.677461268355039170, -227.9997968350711801 ) ) ;
#2557=CARTESIAN_POINT ( 'NONE',  ( 10.35958063030883025, 8.003303894222913328, -225.9303204057916048 ) ) ;
#2558=CARTESIAN_POINT ( 'NONE',  ( 11.62313423782632782, 11.98467543564608029, -219.7293303032897995 ) ) ;
#2560=CARTESIAN_POINT ( 'NONE',  ( -30.36433721104044992, -10.30696067327809651, -227.5875578433412159 ) ) ;
#2561=CARTESIAN_POINT ( 'NONE',  ( -20.83683780809167629, -19.66850649927503625, -219.7460615899071570 ) ) ;
#2562=CARTESIAN_POINT ( 'NONE',  ( 8.709470447750865318, -17.43408031369701661, -216.5121658579468829 ) ) ;
#2566=CARTESIAN_POINT ( 'NONE',  ( -12.19796877179171446, 17.24929682309303658, -234.5722138766719809 ) ) ;
#2567=CARTESIAN_POINT ( 'NONE',  ( 11.82206472115893447, -5.594380913675770728, -219.9420363600394239 ) ) ;
#2568=CARTESIAN_POINT ( 'NONE',  ( 14.34945462593695531, -6.128426910066905542, -229.1128190117150041 ) ) ;
#2569=CARTESIAN_POINT ( 'NONE',  ( -12.06153928353927540, 8.661506524875534296, -226.8425068572842349 ) ) ;
#2570=CARTESIAN_POINT ( 'NONE',  ( 8.821742718405863215, 10.82866050966069160, -221.4785132813277642 ) ) ;
#2571=CARTESIAN_POINT ( 'NONE',  ( 11.21155440434494643, 24.57152134148167733, -221.7155903571010356 ) ) ;
#2574=CARTESIAN_POINT ( 'NONE',  ( 3.550474435626596037, -26.82390172985419952, -218.7255222707324549 ) ) ;
#2577=CARTESIAN_POINT ( 'NONE',  ( -3.309130212696198559, 28.80211350556483296, -217.4284252357080334 ) ) ;
#2578=CARTESIAN_POINT ( 'NONE',  ( -4.531689447889125866, 14.11317536318881416, -231.6806015375303502 ) ) ;
#2579=CARTESIAN_POINT ( 'NONE',  ( 14.29170853205465264, -5.149528714972483989, -227.7869631675187350 ) ) ;
#2580=CARTESIAN_POINT ( 'NONE',  ( -3.326157069579807946, 13.92020081821418565, -220.5733722327383930 ) ) ;
#2583=CARTESIAN_POINT ( 'NONE',  ( -5.529079411693809121, 13.00503897727793401, -226.8014833675713646 ) ) ;
#2584=CARTESIAN_POINT ( 'NONE',  ( 17.72360441613731652, -1.822637811265336749, -232.2813868768326984 ) ) ;
#2585=CARTESIAN_POINT ( 'NONE',  ( -13.58874046263339608, 12.73011668665171392, -216.5659449791897941 ) ) ;
#2586=CARTESIAN_POINT ( 'NONE',  ( 21.53262694368047647, 11.06794636811408594, -231.8394491640143826 ) ) ;
#2589=CARTESIAN_POINT ( 'NONE',  ( -1.565160934061885500, 18.19073094521525391, -232.0278805765578909 ) ) ;
#2590=CARTESIAN_POINT ( 'NONE',  ( -16.76449091996730090, -6.021196472930381738, -231.5810252088758432 ) ) ;
#2591=CARTESIAN_POINT ( 'NONE',  ( 12.71450444683213021, 7.595266944807587350, -224.4213778964231665 ) ) ;
#2592=CARTESIAN_POINT ( 'NONE',  ( 1.444415905432371749, -18.02453083990606331, -216.1804672466811894 ) ) ;
#2595=CARTESIAN_POINT ( 'NONE',  ( -13.88743542672353826, 10.36310385030668613, -230.6144170796622745 ) ) ;
#2598=CARTESIAN_POINT ( 'NONE',  ( 11.29822263435752205, -11.23247557268489771, -230.2410575525588570 ) ) ;
#2599=CARTESIAN_POINT ( 'NONE',  ( 9.094331215210646135, 23.85463374792894342, -219.7669638091879847 ) ) ;
#2600=CARTESIAN_POINT ( 'NONE',  ( -15.30295614572244922, 9.661125001905515930, -218.8475896279880146 ) ) ;
#2601=CARTESIAN_POINT ( 'NONE',  ( -9.722597143579921664, 7.159547510896417499, -227.5730737101346222 ) ) ;
#2602=CARTESIAN_POINT ( 'NONE',  ( -14.57915343259292307, -9.548365625374035659, -229.2620333697842057 ) ) ;
#2603=CARTESIAN_POINT ( 'NONE',  ( 10.02118533929671074, 10.65166262057242008, -217.7534731326719566 ) ) ;
#2605=CARTESIAN_POINT ( 'NONE',  ( -26.65136949509196640, -16.37772123076025466, -229.1931346627563073 ) ) ;
#2606=CARTESIAN_POINT ( 'NONE',  ( 7.163080459435270164, 24.05253566895842354, -232.4475987112033408 ) ) ;
#2608=CARTESIAN_POINT ( 'NONE',  ( 14.50618777373884960, 4.375057440872940795, -230.8807389798650433 ) ) ;
#2610=CARTESIAN_POINT ( 'NONE',  ( -5.974114889119001681, 17.52937113675171332, -232.3862906442651592 ) ) ;
#2611=CARTESIAN_POINT ( 'NONE',  ( 9.818699534354031755, 13.69084898312510390, -233.4870046949650089 ) ) ;
#2612=CARTESIAN_POINT ( 'NONE',  ( 8.483411394722875087, -26.22410139474833457, -227.7697325675642617 ) ) ;
#2614=CARTESIAN_POINT ( 'NONE',  ( -0.6703493356118243041, -28.01673786290986712, -221.2203946787553548 ) ) ;
#2615=CARTESIAN_POINT ( 'NONE',  ( 18.60971343765040942, 2.368090295052050820, -218.6871071987073094 ) ) ;
#2616=CARTESIAN_POINT ( 'NONE',  ( 11.90144651507291051, -8.898305237537579515, -228.5592478859710184 ) ) ;
#2617=CARTESIAN_POINT ( 'NONE',  ( 13.49429091642815770, -0.3433647160923702368, -223.9641315955981895 ) ) ;
#2618=CARTESIAN_POINT ( 'NONE',  ( -14.34280792637948743, -22.10828917559366147, -217.4172704053049756 ) ) ;
#2619=CARTESIAN_POINT ( 'NONE',  ( 7.249842700832647147, 18.24319783868832801, -219.1110502051974720 ) ) ;
#2620=CARTESIAN_POINT ( 'NONE',  ( 21.15841376125116824, 4.865517895153391947, -217.1795922978051578 ) ) ;
#2621=CARTESIAN_POINT ( 'NONE',  ( 4.559463107227270662, 13.27337529356814017, -226.9596205199204633 ) ) ;
#2622=CARTESIAN_POINT ( 'NONE',  ( 3.198229568054530070, 16.42319727383711481, -222.3960047798183552 ) ) ;
#2623=CARTESIAN_POINT ( 'NONE',  ( 16.22685372911609036, -0.3790667790403521309, -218.4894315352551644 ) ) ;
#2627=CARTESIAN_POINT ( 'NONE',  ( 17.24952650401854370, 25.19767938110938843, -224.5319471861414797 ) ) ;
#2628=CARTESIAN_POINT ( 'NONE',  ( -13.41250421226414069, 17.27419134292087577, -217.6844171132545966 ) ) ;
#2629=CARTESIAN_POINT ( 'NONE',  ( -27.56397725925346975, 4.259055856374357241, -222.4951663284069241 ) ) ;
#2630=CARTESIAN_POINT ( 'NONE',  ( 4.788325992165110456, -24.70830725884669121, -218.5516572218182603 ) ) ;
#2634=CARTESIAN_POINT ( 'NONE',  ( 15.89706143421296147, 10.57416387607782227, -218.3862415393350318 ) ) ;
#2635=CARTESIAN_POINT ( 'NONE',  ( 18.63320037895408277, -18.75851321891666146, -220.1409915463867151 ) ) ;
#2636=CARTESIAN_POINT ( 'NONE',  ( -21.28183200535960040, 1.085030287403131233, -217.0000000015322712 ) ) ;
#2637=CARTESIAN_POINT ( 'NONE',  ( -8.379125946468517938, -29.31735857037017468, -221.8060643354269814 ) ) ;
#2639=CARTESIAN_POINT ( 'NONE',  ( 4.883314309504700468, 19.06839645569368358, -217.0171359871271193 ) ) ;
#2641=CARTESIAN_POINT ( 'NONE',  ( -5.028549462823471039, 18.55099042571767143, -234.6264744246184648 ) ) ;
#2643=CARTESIAN_POINT ( 'NONE',  ( -6.571166997218196748, 12.74865329367398736, -229.9840124400968762 ) ) ;
#2644=CARTESIAN_POINT ( 'NONE',  ( 23.00003818093501806, -2.342406833639917085, -233.2756072794339843 ) ) ;
#2645=CARTESIAN_POINT ( 'NONE',  ( 23.84888352507021736, -3.411310983279423947, -216.3556234003997645 ) ) ;
#2647=CARTESIAN_POINT ( 'NONE',  ( -11.24282496690421596, 12.44430180464951086, -232.4405891940542404 ) ) ;
#2648=CARTESIAN_POINT ( 'NONE',  ( -12.81114484120449504, -26.81657559919244349, -231.7433950434849805 ) ) ;
#2649=CARTESIAN_POINT ( 'NONE',  ( 19.63495056682994289, -4.096126682090319271, -232.1271738766904207 ) ) ;
#2650=CARTESIAN_POINT ( 'NONE',  ( -13.58874046263339608, 12.73011668665171392, -216.5659449791897941 ) ) ;
#2651=CARTESIAN_POINT ( 'NONE',  ( 17.32394486779715592, 4.028159306070694612, -218.4253989884176690 ) ) ;
#2652=CARTESIAN_POINT ( 'NONE',  ( 4.482815116226093188, 26.97722808566452812, -229.2080185206130238 ) ) ;
#2654=CARTESIAN_POINT ( 'NONE',  ( 21.91535456744164279, 7.573568724377624406, -232.0371228855588868 ) ) ;
#2655=CARTESIAN_POINT ( 'NONE',  ( -8.785593564164850378, -26.69987990810942691, -222.9015467003982849 ) ) ;
#2657=CARTESIAN_POINT ( 'NONE',  ( 9.798337081649805214, 12.27506320122302697, -218.9346733583377613 ) ) ;
#2658=CARTESIAN_POINT ( 'NONE',  ( -6.260151855817680300, 29.88549235135308635, -226.8929519981915064 ) ) ;
#2659=CARTESIAN_POINT ( 'NONE',  ( -14.78201816772319077, -5.155518158621814173, -222.1275223803717154 ) ) ;
#2662=CARTESIAN_POINT ( 'NONE',  ( 15.92396645628901020, -0.3225394686005420009, -223.0199929375764327 ) ) ;
#2663=CARTESIAN_POINT ( 'NONE',  ( -5.077014288276974874, -29.41487918302398796, -226.0100937268998962 ) ) ;
#2664=CARTESIAN_POINT ( 'NONE',  ( 14.19800769603076240, 4.587407146151301518, -224.2928935459285071 ) ) ;
#2666=CARTESIAN_POINT ( 'NONE',  ( 5.248230734842167955, 23.54336384919183445, -216.8914391693808739 ) ) ;
#2667=CARTESIAN_POINT ( 'NONE',  ( 14.85895087972432549, -2.358194654258901846, -226.8569002201626290 ) ) ;
#2669=CARTESIAN_POINT ( 'NONE',  ( -24.19163806436329978, 8.131440952769249719, -230.9341214615949127 ) ) ;
#2670=CARTESIAN_POINT ( 'NONE',  ( 22.90621760533471019, 17.25363305745006670, -230.8615280072714597 ) ) ;
#2673=CARTESIAN_POINT ( 'NONE',  ( 20.41153371889344825, 17.18812948447019551, -230.7531656956970778 ) ) ;
#2675=CARTESIAN_POINT ( 'NONE',  ( 17.75464445068659458, -4.950329359371821170, -229.7529072665692240 ) ) ;
#2676=CARTESIAN_POINT ( 'NONE',  ( -15.51091956967506391, -1.782849713491490018, -228.8089183834494520 ) ) ;
#2680=CARTESIAN_POINT ( 'NONE',  ( -9.290933312444883185, 29.15551353946876745, -225.8551562993724247 ) ) ;
#2681=CARTESIAN_POINT ( 'NONE',  ( 23.82514222742702614, -14.35463969081363267, -233.5616060903067535 ) ) ;
#2682=CARTESIAN_POINT ( 'NONE',  ( 20.25084204406298127, -10.11176871144018818, -232.7817218064674591 ) ) ;
#2683=CARTESIAN_POINT ( 'NONE',  ( -19.74163224554151697, 8.726897413558679872, -232.6665747339030190 ) ) ;
#2684=CARTESIAN_POINT ( 'NONE',  ( 22.73582563804385970, 20.20868311426415431, -227.8513184012435886 ) ) ;
#2685=CARTESIAN_POINT ( 'NONE',  ( 20.92326490933994876, 18.00580109995737033, -222.6060933800056034 ) ) ;
#2687=CARTESIAN_POINT ( 'NONE',  ( 3.098311947274309919, -13.44192016451707872, -223.0038505953381502 ) ) ;
#2688=CARTESIAN_POINT ( 'NONE',  ( 19.20300624114736721, 0.6066039755357417462, -231.5046416827383950 ) ) ;
#2689=CARTESIAN_POINT ( 'NONE',  ( -4.365576370787875859, 13.02741211227440665, -230.2897948137907917 ) ) ;
#2690=CARTESIAN_POINT ( 'NONE',  ( -14.58084844870496966, 13.85720943031455832, -233.3219724312919254 ) ) ;
#2691=CARTESIAN_POINT ( 'NONE',  ( 19.92157794555808437, -7.202678279460218214, -232.3584036642729416 ) ) ;
#2692=CARTESIAN_POINT ( 'NONE',  ( -6.101488798441174310, 11.33371047077072369, -225.3616985956418546 ) ) ;
#2695=CARTESIAN_POINT ( 'NONE',  ( -5.786930954831501772, 15.78543306641166311, -231.0475152612371517 ) ) ;
#2696=CARTESIAN_POINT ( 'NONE',  ( -16.66921372850992000, 0.4301828684420727078, -227.8397539831347842 ) ) ;
#2697=CARTESIAN_POINT ( 'NONE',  ( -15.20262116893801974, 8.038155052917188570, -217.6767387945475036 ) ) ;
#2698=CARTESIAN_POINT ( 'NONE',  ( 26.24002132888527328, 11.62331517472360964, -222.5300873157218859 ) ) ;
#2699=CARTESIAN_POINT ( 'NONE',  ( 3.528957931946373971, 27.43889307663531696, -223.4805233499528185 ) ) ;
#2700=CARTESIAN_POINT ( 'NONE',  ( 15.44208300017355739, 0.06603094323067049132, -228.0000000000006253 ) ) ;
#2701=CARTESIAN_POINT ( 'NONE',  ( 7.951191770265756631, 20.55701948568933091, -231.2149185317973661 ) ) ;
#2702=CARTESIAN_POINT ( 'NONE',  ( -15.74157322273402748, -13.22745315869835636, -216.7831660370879661 ) ) ;
#2703=CARTESIAN_POINT ( 'NONE',  ( 14.98418162551161714, 4.450317369940187895, -227.9894155827521161 ) ) ;
#2704=CARTESIAN_POINT ( 'NONE',  ( -3.535116539333309049, -19.81104435003528152, -216.2789031305144931 ) ) ;
#2706=CARTESIAN_POINT ( 'NONE',  ( -12.05423124486310904, 12.38527783110887803, -219.7419643105747014 ) ) ;
#2707=DIRECTION ( 'NONE',  ( 1.000000000000000000, 0.000000000000000000, 0.000000000000000000 ) ) ;
#2708=CARTESIAN_POINT ( 'NONE',  ( 14.49023023880111083, -12.14520762395643061, -217.6171285705176501 ) ) ;
#2709=CARTESIAN_POINT ( 'NONE',  ( 3.673290835002071653, 15.92545533070904895, -226.4848186297188022 ) ) ;
#2710=CARTESIAN_POINT ( 'NONE',  ( -14.35594238341465889, 9.236863657925704629, -219.6542735655305307 ) ) ;
#2711=CARTESIAN_POINT ( 'NONE',  ( -20.02994071726468661, 1.326980477106467271, -234.9527056834518532 ) ) ;
#2712=CARTESIAN_POINT ( 'NONE',  ( -15.83567870103663466, -7.501751145129069265, -221.2716155488439824 ) ) ;
#2714=CARTESIAN_POINT ( 'NONE',  ( 8.865150807857233417, 8.939496441981303221, -220.7647208555746090 ) ) ;
#2716=CARTESIAN_POINT ( 'NONE',  ( -22.21568756412429835, -23.56320124644456016, -225.3776980696049463 ) ) ;
#2717=CARTESIAN_POINT ( 'NONE',  ( 9.527502190795640757, 23.55559004943647139, -217.4101659741468211 ) ) ;
#2718=CARTESIAN_POINT ( 'NONE',  ( 12.93042813863272755, 0.4488092930645843914, -225.5263188864764174 ) ) ;
#2719=CARTESIAN_POINT ( 'NONE',  ( -13.23768812067001477, 12.78288831771969569, -230.4179793829127902 ) ) ;
#2720=CARTESIAN_POINT ( 'NONE',  ( 7.116434306140963173, 9.967665124511082553, -224.4990387090310833 ) ) ;
#2723=CARTESIAN_POINT ( 'NONE',  ( 0.005738405568439595983, -15.19016956849912070, -227.2100150994057230 ) ) ;
#2724=CARTESIAN_POINT ( 'NONE',  ( -3.515149843921121509, -20.22121776728782550, -231.9652171757311123 ) ) ;
#2725=CARTESIAN_POINT ( 'NONE',  ( 21.60524407607017849, 3.028118258437591415, -217.8361640396714449 ) ) ;
#2726=CARTESIAN_POINT ( 'NONE',  ( 15.11994912051959972, -12.48385213956034079, -232.8079920308188377 ) ) ;
#2727=CARTESIAN_POINT ( 'NONE',  ( -27.85133024402786006, -1.794102530182491773, -229.4204807338591081 ) ) ;
#2728=CARTESIAN_POINT ( 'NONE',  ( -15.62091161899253855, -26.00636881980398840, -222.1463585103649905 ) ) ;
#2729=CARTESIAN_POINT ( 'NONE',  ( 11.41090957555148222, 16.52772439454343711, -218.2458222691329013 ) ) ;
#2730=CARTESIAN_POINT ( 'NONE',  ( 2.967317674205219191, -16.40215926535219282, -217.6245344443522924 ) ) ;
#2732=CARTESIAN_POINT ( 'NONE',  ( -13.63442241228529994, 1.608023091903783008, -219.2326980015357094 ) ) ;
#2733=CARTESIAN_POINT ( 'NONE',  ( 7.769483725421269860, 20.68783433326350263, -233.2348178266662728 ) ) ;
#2734=CARTESIAN_POINT ( 'NONE',  ( 0.1979841192334154676, 16.22068729745496540, -223.9539336445596973 ) ) ;
#2735=CARTESIAN_POINT ( 'NONE',  ( 8.798770371347417907, -12.71349942585338333, -232.9159113209695704 ) ) ;
#2736=CARTESIAN_POINT ( 'NONE',  ( 11.63337745479824292, 8.229076005436313679, -220.5472098800687206 ) ) ;
#2737=CARTESIAN_POINT ( 'NONE',  ( -18.64931821476190876, 22.04453097546810270, -226.2485927806324923 ) ) ;
#2738=CARTESIAN_POINT ( 'NONE',  ( -27.01279207917464475, 4.316569700791554887, -221.4451031230926219 ) ) ;
#2739=CARTESIAN_POINT ( 'NONE',  ( -0.6703493356118243041, -28.01673786290986712, -221.2203946787553548 ) ) ;
#2742=CARTESIAN_POINT ( 'NONE',  ( 22.84140515590350518, 18.29101041979067332, -226.2334522600520472 ) ) ;
#2743=CARTESIAN_POINT ( 'NONE',  ( 13.30832375548903990, -9.333840824262514602, -222.9696809959601183 ) ) ;
#2744=CARTESIAN_POINT ( 'NONE',  ( -18.88895772509644644, 1.306698388790553444, -217.6272550812279292 ) ) ;
#2745=CARTESIAN_POINT ( 'NONE',  ( -5.279374154171231126, -12.28263746854076466, -222.5283095625445640 ) ) ;
#2746=CARTESIAN_POINT ( 'NONE',  ( -2.934221234790329369, 15.07857928364152222, -230.9558365497803720 ) ) ;
#2747=CARTESIAN_POINT ( 'NONE',  ( 4.065638640983322283, 32.08830473489500434, -226.0249194102539150 ) ) ;
#2749=CARTESIAN_POINT ( 'NONE',  ( -12.78558550453068854, 7.693178343823584342, -230.0800953344970878 ) ) ;
#2750=CARTESIAN_POINT ( 'NONE',  ( -13.68337831708448782, -3.656824064325736590, -221.3737413816871538 ) ) ;
#2751=CARTESIAN_POINT ( 'NONE',  ( 30.39189047201120175, -1.943849802383817993, -228.0804048816970919 ) ) ;
#2753=CARTESIAN_POINT ( 'NONE',  ( -9.250876228778270871, 9.538614635316015722, -227.1332118982684563 ) ) ;
#2754=CARTESIAN_POINT ( 'NONE',  ( -22.21568756412429835, -23.56320124644456016, -225.3776980696049463 ) ) ;
#2755=CARTESIAN_POINT ( 'NONE',  ( 22.44368505003003378, -11.72633196808685163, -232.1179326287041533 ) ) ;
#2756=CARTESIAN_POINT ( 'NONE',  ( -12.31207293045244988, 6.732038552366256923, -221.0952066824360713 ) ) ;
#2757=CARTESIAN_POINT ( 'NONE',  ( -11.84805200323110164, 5.835720598137266180, -228.2740675967047537 ) ) ;
#2758=CARTESIAN_POINT ( 'NONE',  ( 2.482746429915354547, 16.41797261123590346, -229.5599230346982154 ) ) ;
#2760=CARTESIAN_POINT ( 'NONE',  ( -19.59898341672158040, 3.279988180491820504, -234.9371679595475086 ) ) ;
#2761=CARTESIAN_POINT ( 'NONE',  ( -13.20043892455957746, -23.63849784199488369, -228.2145582502841989 ) ) ;
#2763=CARTESIAN_POINT ( 'NONE',  ( -25.19248792833826300, 13.40115236862232528, -221.2817950683888455 ) ) ;
#2764=CARTESIAN_POINT ( 'NONE',  ( 9.880827190695510964, 24.82036951119805579, -218.1633337467656020 ) ) ;
#2765=CARTESIAN_POINT ( 'NONE',  ( -2.508488193221233953, 16.03207605874066033, -217.8880952293912969 ) ) ;
#2767=CARTESIAN_POINT ( 'NONE',  ( 18.43413881788024611, -3.292634616013774274, -216.7808090690139409 ) ) ;
#2770=CARTESIAN_POINT ( 'NONE',  ( -24.02434186778878455, 18.57431834865475651, -228.2662945587547370 ) ) ;
#2771=CARTESIAN_POINT ( 'NONE',  ( -4.832117640292445060, -22.41582585812286865, -216.8192401332019870 ) ) ;
#2773=CARTESIAN_POINT ( 'NONE',  ( 10.66614775643814994, 26.29080367171353672, -230.0818785118670178 ) ) ;
#2775=CARTESIAN_POINT ( 'NONE',  ( -12.30606003331388543, 10.59782772616791036, -231.0021630509705801 ) ) ;
#2776=CARTESIAN_POINT ( 'NONE',  ( 17.88619020626327938, 19.43517936004721847, -216.7078103882350604 ) ) ;
#2777=CARTESIAN_POINT ( 'NONE',  ( 15.48387324202036908, 0.7120489543666520538, -222.0826739725034997 ) ) ;
#2778=CARTESIAN_POINT ( 'NONE',  ( 14.39473142419577023, 15.98257177912839389, -217.4557725731239373 ) ) ;
#2780=CARTESIAN_POINT ( 'NONE',  ( 18.87161431088011199, -9.942086275362749248, -230.8324498438813350 ) ) ;
#2781=CARTESIAN_POINT ( 'NONE',  ( -16.64477864544768337, -2.947896226079009807, -219.6737919733007516 ) ) ;
#2785=CARTESIAN_POINT ( 'NONE',  ( -2.665457046508036942, 16.94988614842223029, -218.7621057649994896 ) ) ;
#2786=CARTESIAN_POINT ( 'NONE',  ( 16.57791564354289093, -3.035441731457511949, -233.7002882787241163 ) ) ;
#2787=CARTESIAN_POINT ( 'NONE',  ( 15.84759643368428428, -7.142586963752317608, -231.1761396821659673 ) ) ;
#2788=CARTESIAN_POINT ( 'NONE',  ( -29.22672729369577738, 6.588740615114764054, -224.9915299386302934 ) ) ;
#2789=CARTESIAN_POINT ( 'NONE',  ( 29.89309326230132058, 6.052383583152112223, -228.3539431708548477 ) ) ;
#2790=CARTESIAN_POINT ( 'NONE',  ( 16.53859560591101641, 22.24348416270211359, -223.7250258089275974 ) ) ;
#2792=CARTESIAN_POINT ( 'NONE',  ( 13.17262855481386374, -26.22572064374609013, -230.8671443076513583 ) ) ;
#2793=CARTESIAN_POINT ( 'NONE',  ( 14.80394259695730064, 1.224172658189580432, -225.4564070658925061 ) ) ;
#2794=CARTESIAN_POINT ( 'NONE',  ( -20.73319232323294514, 5.144688277016327582, -214.6391322078443977 ) ) ;
#2795=CARTESIAN_POINT ( 'NONE',  ( 7.116434306140963173, 9.967665124511082553, -224.4990387090310833 ) ) ;
#2796=CARTESIAN_POINT ( 'NONE',  ( 4.952019330116582907, 28.88045068338265509, -217.6369327391592208 ) ) ;
#2797=CARTESIAN_POINT ( 'NONE',  ( 13.38912848839664704, -8.011079660592983487, -223.8512906815321628 ) ) ;
#2799=CARTESIAN_POINT ( 'NONE',  ( -2.817219543927646175, 14.13981714106644993, -229.6779615865167443 ) ) ;
#2803=CARTESIAN_POINT ( 'NONE',  ( -6.581016643627174645, 27.50493254600863935, -230.8763182197739070 ) ) ;
#2804=CARTESIAN_POINT ( 'NONE',  ( -15.12838653695630420, 3.161599240781852949, -225.7834014684609656 ) ) ;
#2805=CARTESIAN_POINT ( 'NONE',  ( -13.56774755469388616, 7.311522441667196226, -219.1912666243428021 ) ) ;
#2806=CARTESIAN_POINT ( 'NONE',  ( 13.49011766416699842, 7.659170998773840111, -228.1905628957712793 ) ) ;
#2807=CARTESIAN_POINT ( 'NONE',  ( 13.50603691942335693, 22.79443449215731832, -229.7689193854997995 ) ) ;
#2808=CARTESIAN_POINT ( 'NONE',  ( 15.55281408287027922, 0.9489306161008197460, -227.8472323654694947 ) ) ;
#2810=CARTESIAN_POINT ( 'NONE',  ( 11.27486163995310164, 25.12851252939060487, -222.6718455410222930 ) ) ;
#2811=CARTESIAN_POINT ( 'NONE',  ( -17.58118739749173898, -8.238107657346720458, -217.5252134542318458 ) ) ;
#2812=CARTESIAN_POINT ( 'NONE',  ( 20.23125423326388628, 7.836699765464857137, -217.8891354894872450 ) ) ;
#2813=CARTESIAN_POINT ( 'NONE',  ( -0.4062606655315902371, -23.43967590431752512, -234.4451928229410100 ) ) ;
#2815=CARTESIAN_POINT ( 'NONE',  ( -7.873497077133136735, 15.44270125396616677, -230.2562282217168672 ) ) ;
#2817=CARTESIAN_POINT ( 'NONE',  ( 11.72194121175188997, -15.95900783718691507, -217.6519982781775013 ) ) ;
#2818=CARTESIAN_POINT ( 'NONE',  ( 8.645835506124264214, 12.38899589144949687, -223.4673650485651990 ) ) ;
#2819=CARTESIAN_POINT ( 'NONE',  ( -7.965409144353247761, 13.56739834143082213, -221.6246244520798712 ) ) ;
#2820=CARTESIAN_POINT ( 'NONE',  ( -14.08083899843152231, 10.81596681319144970, -234.3239311387574446 ) ) ;
#2822=CARTESIAN_POINT ( 'NONE',  ( -19.42704602366333688, -5.151203963165301936, -219.4215732619585708 ) ) ;
#2823=CARTESIAN_POINT ( 'NONE',  ( -16.23590288079963173, 0.2625226423351309513, -226.8300841971807813 ) ) ;
#2825=CARTESIAN_POINT ( 'NONE',  ( -10.70714119831929168, -8.316548062297686172, -219.3892619542279192 ) ) ;
#2826=CARTESIAN_POINT ( 'NONE',  ( -2.692720963948733282, 24.67937284847025481, -218.0912907784291406 ) ) ;
#2827=CARTESIAN_POINT ( 'NONE',  ( 21.52074627118099315, 8.791036694007010155, -215.9547738671300294 ) ) ;
#2828=CARTESIAN_POINT ( 'NONE',  ( -17.65560862077320081, 21.92186454631220371, -221.3776075196718693 ) ) ;
#2829=CARTESIAN_POINT ( 'NONE',  ( 11.78717493688862206, 28.63884142527983556, -229.7724827508652652 ) ) ;
#2830=CARTESIAN_POINT ( 'NONE',  ( 3.112457940538468470, -21.91845672593830940, -231.6743386618371403 ) ) ;
#2831=CARTESIAN_POINT ( 'NONE',  ( -2.389036117848273300, -16.12222041688038132, -229.2542492100865559 ) ) ;
#2832=CARTESIAN_POINT ( 'NONE',  ( -18.67456582549428390, 11.07053394491094345, -214.7114755712704550 ) ) ;
#2833=CARTESIAN_POINT ( 'NONE',  ( 21.39922646226391478, -21.53954253117021977, -224.1701659532164967 ) ) ;
#2834=CARTESIAN_POINT ( 'NONE',  ( -14.48876282330270016, -2.056064607042531911, -223.6537127325441361 ) ) ;
#2835=CARTESIAN_POINT ( 'NONE',  ( -5.519971913460887336, -12.21762732219001713, -227.2962593638428359 ) ) ;
#2836=CARTESIAN_POINT ( 'NONE',  ( 26.51393280883522863, 15.12455065102723495, -226.1955201378414415 ) ) ;
#2838=CARTESIAN_POINT ( 'NONE',  ( -10.10782416658048710, 9.083762506436128703, -227.1045422723873344 ) ) ;
#2839=CARTESIAN_POINT ( 'NONE',  ( -3.673551555920188783, 29.81207051619892923, -228.8770490300152005 ) ) ;
#2840=CARTESIAN_POINT ( 'NONE',  ( 9.931717191100288389, 12.93133689537362940, -228.8926047089119038 ) ) ;
#2841=CARTESIAN_POINT ( 'NONE',  ( 10.88145840916109819, -7.482884786208209960, -219.8679920012262414 ) ) ;
#2842=CARTESIAN_POINT ( 'NONE',  ( 23.22505041959077232, 19.39625294115234055, -221.5972645870541555 ) ) ;
#2843=CARTESIAN_POINT ( 'NONE',  ( -14.20363567091065349, 7.857660128015216294, -223.4151327167956822 ) ) ;
#2844=CARTESIAN_POINT ( 'NONE',  ( -2.389036117848273300, -16.12222041688038132, -229.2542492100865559 ) ) ;
#2847=CARTESIAN_POINT ( 'NONE',  ( 19.72515656911863147, 14.02277373989196541, -218.0718040828188009 ) ) ;
#2848=CARTESIAN_POINT ( 'NONE',  ( 12.37559490515920579, -12.83230305503110991, -219.7713711637379106 ) ) ;
#2849=CARTESIAN_POINT ( 'NONE',  ( -27.92885697401080591, 6.962042978589167319, -220.9552227796709190 ) ) ;
#2850=CARTESIAN_POINT ( 'NONE',  ( -1.632242579688942596, -13.62074943359385415, -221.1585305289511041 ) ) ;
#2851=CARTESIAN_POINT ( 'NONE',  ( -3.843007962268670585, 27.94983497691806917, -231.4302614368887703 ) ) ;
#2852=CARTESIAN_POINT ( 'NONE',  ( 4.024086222410633518, 12.48004227094270746, -230.0177668608922374 ) ) ;
#2854=CARTESIAN_POINT ( 'NONE',  ( 0.6364901924797052857, 13.89978473517355617, -221.8840706290426397 ) ) ;
#2855=CARTESIAN_POINT ( 'NONE',  ( -12.88620494227545343, -3.269292211592822461, -225.1464181993036391 ) ) ;
#2858=CARTESIAN_POINT ( 'NONE',  ( 0.6364901924797052857, 13.89978473517355617, -221.8840706290426397 ) ) ;
#2859=CARTESIAN_POINT ( 'NONE',  ( -6.776294192501696401, -30.39940938379458046, -221.2799938066956997 ) ) ;
#2860=CARTESIAN_POINT ( 'NONE',  ( 22.14671607713456325, -14.13547298543019437, -218.1897693226341914 ) ) ;
#2861=CARTESIAN_POINT ( 'NONE',  ( -3.514547081416551588, 30.38636916157537016, -227.3529586180979436 ) ) ;
#2862=CARTESIAN_POINT ( 'NONE',  ( -14.99655511003079233, 2.316638599135941945, -232.4215266639120046 ) ) ;
#2863=CARTESIAN_POINT ( 'NONE',  ( 5.142103055192286831, 28.18228231877369439, -225.8998064704803994 ) ) ;
#2864=CARTESIAN_POINT ( 'NONE',  ( -20.26851768784797869, -0.8260594303982465858, -217.1279713726092098 ) ) ;
#2865=CARTESIAN_POINT ( 'NONE',  ( -14.01966324001334385, 10.60695606488527964, -217.6333332521996340 ) ) ;
#2866=CARTESIAN_POINT ( 'NONE',  ( -12.19937816677273013, -10.70901586236097636, -226.3808855409166370 ) ) ;
#2869=CARTESIAN_POINT ( 'NONE',  ( -13.75208518020500748, 5.661250135068270239, -227.6647651141479685 ) ) ;
#2870=CARTESIAN_POINT ( 'NONE',  ( 6.040050017043670394, 13.67534390435379699, -220.4759402345340504 ) ) ;
#2871=CARTESIAN_POINT ( 'NONE',  ( -1.884624261322229266, 13.00421381464247084, -226.7648460381863345 ) ) ;
#2872=CARTESIAN_POINT ( 'NONE',  ( -18.30524310960561252, -4.731645231655051909, -231.4308113063693781 ) ) ;
#2875=CARTESIAN_POINT ( 'NONE',  ( -10.51143808951550085, 11.41308718311005066, -231.3573069600382439 ) ) ;
#2876=CARTESIAN_POINT ( 'NONE',  ( -20.07469464351956390, -22.83895492621963896, -220.1373730632280967 ) ) ;
#2877=CARTESIAN_POINT ( 'NONE',  ( 13.64549276890110008, 1.404530603506124020, -227.6530344292614245 ) ) ;
#2878=CARTESIAN_POINT ( 'NONE',  ( 15.12287735332712835, 21.03907941686458116, -231.7894952627153202 ) ) ;
#2881=CARTESIAN_POINT ( 'NONE',  ( 28.33476664927451338, -0.7768526459456059907, -228.3750448408243869 ) ) ;
#2882=CARTESIAN_POINT ( 'NONE',  ( -13.66744685701839046, 5.938820276054873837, -223.0954633396572149 ) ) ;
#2883=CARTESIAN_POINT ( 'NONE',  ( 15.46952826979347151, 3.173892190046953665, -221.7237849701489552 ) ) ;
#2884=CARTESIAN_POINT ( 'NONE',  ( 13.92641534307036189, 0.2825193253608765387, -222.0121013341077969 ) ) ;
#2887=CARTESIAN_POINT ( 'NONE',  ( 20.53331905177824979, -5.913034700419025569, -230.9395893631423462 ) ) ;
#2889=CARTESIAN_POINT ( 'NONE',  ( -26.07210576407111446, -8.413030596423759278, -230.6002792590230115 ) ) ;
#2892=CARTESIAN_POINT ( 'NONE',  ( -11.23881320317003407, 15.84151802331611236, -234.2799649731619809 ) ) ;
#2893=CARTESIAN_POINT ( 'NONE',  ( 30.30402220111207612, -9.997565949388443229, -221.8870099070453250 ) ) ;
#2894=CARTESIAN_POINT ( 'NONE',  ( 28.78651053433536333, -0.9604905981993369091, -227.3547688931310233 ) ) ;
#2895=CARTESIAN_POINT ( 'NONE',  ( -14.35594238341465889, 9.236863657925704629, -219.6542735655305307 ) ) ;
#2896=CARTESIAN_POINT ( 'NONE',  ( 15.39025625686376841, 1.044190007782545226, -218.9203249718910911 ) ) ;
#2897=CARTESIAN_POINT ( 'NONE',  ( 12.91676121433235913, 9.519065828383201477, -226.8102878246443765 ) ) ;
#2898=CARTESIAN_POINT ( 'NONE',  ( -0.7782973328492528431, -21.73504563028646075, -232.5926793935175283 ) ) ;
#2900=CARTESIAN_POINT ( 'NONE',  ( -20.06846544527470400, 7.877362284741439069, -235.3910773253824402 ) ) ;
#2901=CARTESIAN_POINT ( 'NONE',  ( 19.66122710937851537, 22.83208755991274330, -220.0578523118790883 ) ) ;
#2902=CARTESIAN_POINT ( 'NONE',  ( 3.982203626615636427, 14.63895582687697150, -217.4952312584269123 ) ) ;
#2903=CARTESIAN_POINT ( 'NONE',  ( 24.22993967103762714, -2.502297861120115208, -232.9814837474525007 ) ) ;
#2904=CARTESIAN_POINT ( 'NONE',  ( -7.913358619554302642, 16.16796202616373890, -233.0981776325470491 ) ) ;
#2905=CARTESIAN_POINT ( 'NONE',  ( -24.48580119005125866, 9.312492396273500006, -232.5498413856076070 ) ) ;
#2907=CARTESIAN_POINT ( 'NONE',  ( 16.71363093372661979, 20.70203100498337179, -215.6856694095356488 ) ) ;
#2908=CARTESIAN_POINT ( 'NONE',  ( -15.60078324628501356, 3.527872497691606934, -227.4630248446626695 ) ) ;
#2909=CARTESIAN_POINT ( 'NONE',  ( -24.48580119005125866, 9.312492396273500006, -232.5498413856076070 ) ) ;
#2910=CARTESIAN_POINT ( 'NONE',  ( 14.54149994592679107, 8.070685273005897997, -229.7292930672863349 ) ) ;
#2911=CARTESIAN_POINT ( 'NONE',  ( 8.632180352507942800, 16.83956698119041917, -230.4752415867875186 ) ) ;
#2915=CARTESIAN_POINT ( 'NONE',  ( -10.42804209284631156, -14.08702332024887305, -217.7386024361820489 ) ) ;
#2916=CARTESIAN_POINT ( 'NONE',  ( 18.76922974182421555, 13.12635134380198210, -217.8010375391909008 ) ) ;
#2917=CARTESIAN_POINT ( 'NONE',  ( -1.925327751674894339, -31.30071588347811584, -225.0681195224254623 ) ) ;
#2920=CARTESIAN_POINT ( 'NONE',  ( -6.720912670637915198, 19.69156892798266512, -217.8848069150180891 ) ) ;
#2921=CARTESIAN_POINT ( 'NONE',  ( 12.70013114424463296, -16.94540864491495924, -217.3462533088837745 ) ) ;
#2922=CARTESIAN_POINT ( 'NONE',  ( 8.812670488384366507, 12.21486833790445914, -225.9961634525829197 ) ) ;
#2923=CARTESIAN_POINT ( 'NONE',  ( -4.742143146070755932, 15.01230778631049567, -221.4832709320255049 ) ) ;
#2924=CARTESIAN_POINT ( 'NONE',  ( -28.12586305337175219, 12.75764838638491305, -230.3810511299127768 ) ) ;
#2925=CARTESIAN_POINT ( 'NONE',  ( -14.94274040728286046, -6.247332224397157852, -226.1562440284360491 ) ) ;
#2926=CARTESIAN_POINT ( 'NONE',  ( 17.72360441613731652, -1.822637811265336749, -232.2813868768326984 ) ) ;
#2929=CARTESIAN_POINT ( 'NONE',  ( 22.03647168421188240, 0.3315607655626218175, -232.0572713672587213 ) ) ;
#2930=CARTESIAN_POINT ( 'NONE',  ( 11.09231067055629616, 7.417581979752235100, -227.5152062457793534 ) ) ;
#2931=CARTESIAN_POINT ( 'NONE',  ( -16.27736488614644372, 5.941157768540612949, -228.4237983497913547 ) ) ;
#2933=CARTESIAN_POINT ( 'NONE',  ( 5.030854775705693172, 19.94152319263364603, -234.9034581965229336 ) ) ;
#2934=CARTESIAN_POINT ( 'NONE',  ( 3.641537757978871248, 12.43698445400491437, -220.3805014257186485 ) ) ;
#2935=CARTESIAN_POINT ( 'NONE',  ( -7.509561119170069077, -14.53281319394193538, -217.7574163112487042 ) ) ;
#2938=CARTESIAN_POINT ( 'NONE',  ( 2.641673488600395636, -17.65289918763021149, -219.1873688300129288 ) ) ;
#2940=CARTESIAN_POINT ( 'NONE',  ( -26.09112266552012471, 5.807188091516064077, -215.7774933166620883 ) ) ;
#2941=CARTESIAN_POINT ( 'NONE',  ( 25.69672030403964769, -15.30292110028031338, -224.0206579222720791 ) ) ;
#2942=CARTESIAN_POINT ( 'NONE',  ( 28.89510310306777541, -0.2847990887752292477, -220.1812426115722303 ) ) ;
#2943=CARTESIAN_POINT ( 'NONE',  ( -11.07688804854283049, -12.81333559660784971, -232.1241261852632363 ) ) ;
#2944=CARTESIAN_POINT ( 'NONE',  ( 20.88350594575732799, 13.65521425050155813, -232.8060468608549911 ) ) ;
#2945=CARTESIAN_POINT ( 'NONE',  ( -22.00000000000137490, -2.602085213965210642E-15, -216.9999999999999716 ) ) ;
#2946=CARTESIAN_POINT ( 'NONE',  ( -11.88513743913613752, 17.65694776598872195, -232.6054623148957035 ) ) ;
#2947=CARTESIAN_POINT ( 'NONE',  ( 15.15306935214909778, 7.771180183537883757, -217.5526096523957165 ) ) ;
#2948=CARTESIAN_POINT ( 'NONE',  ( 12.18657022793382794, 26.76558097653315471, -221.8882195427397335 ) ) ;
#2949=CARTESIAN_POINT ( 'NONE',  ( 20.40268796714816801, 18.65534563792085621, -219.5587498978784993 ) ) ;
#2950=CARTESIAN_POINT ( 'NONE',  ( 27.71804559688024128, -15.88771542466010978, -225.5747850090131692 ) ) ;
#2951=CARTESIAN_POINT ( 'NONE',  ( 27.69955354773053458, 12.81264626165819287, -221.7750850138309602 ) ) ;
#2952=CARTESIAN_POINT ( 'NONE',  ( -14.60180519431160917, 24.46340507526420893, -221.8423643191928534 ) ) ;
#2953=CARTESIAN_POINT ( 'NONE',  ( -6.593106361191484410, 26.27107262772703322, -231.8730401762632596 ) ) ;
#2954=CARTESIAN_POINT ( 'NONE',  ( -7.786003226018990198, -12.23758553950863082, -224.1954257758910671 ) ) ;
#2955=CARTESIAN_POINT ( 'NONE',  ( -18.46722752239034193, 0.9784074152395518809, -232.1633353206286188 ) ) ;
#2959=CARTESIAN_POINT ( 'NONE',  ( 22.02796522526679723, 16.41909032291435366, -220.1590600991317217 ) ) ;
#2960=CARTESIAN_POINT ( 'NONE',  ( 11.44298997664856721, -19.26084286805135193, -217.6324489131326914 ) ) ;
#2961=CARTESIAN_POINT ( 'NONE',  ( -17.99720854823001659, 13.97888873227035056, -232.2992184661552244 ) ) ;
#2962=CARTESIAN_POINT ( 'NONE',  ( -9.625604265899946554, -19.21123364792547505, -233.9327940972253259 ) ) ;
#2963=CARTESIAN_POINT ( 'NONE',  ( -16.04492519386327487, 1.819644280589142626, -223.4665098021627614 ) ) ;
#2964=CARTESIAN_POINT ( 'NONE',  ( 3.490345297502855715, 11.17751288514984331, -224.7799703251421022 ) ) ;
#2966=CARTESIAN_POINT ( 'NONE',  ( 0.4042326456706432647, 15.50845657815858303, -219.2680337625893401 ) ) ;
#2967=CARTESIAN_POINT ( 'NONE',  ( -28.43596199216294806, -10.51226423640377838, -227.0041752157952430 ) ) ;
#2970=CARTESIAN_POINT ( 'NONE',  ( 0.9046320824004248085, 13.39785254849979701, -226.4815711199935890 ) ) ;
#2971=CARTESIAN_POINT ( 'NONE',  ( -4.907461209876205821, -14.28794023480369368, -232.2749568027591636 ) ) ;
#2972=CARTESIAN_POINT ( 'NONE',  ( 7.080148886126969465, -28.65852557119563926, -219.9679292432588227 ) ) ;
#2976=CARTESIAN_POINT ( 'NONE',  ( -13.96653539523557619, 20.94398119165846239, -231.8597527081015528 ) ) ;
#2977=CARTESIAN_POINT ( 'NONE',  ( 13.55451907249704213, 16.71566520821242818, -219.1474322952048226 ) ) ;
#2979=CARTESIAN_POINT ( 'NONE',  ( -29.50764134580612463, 7.783340782857166573, -219.9768238800827191 ) ) ;
#2980=CARTESIAN_POINT ( 'NONE',  ( -21.98560163549725033, -7.841739570055646702, -218.0982455035688474 ) ) ;
#2982=CARTESIAN_POINT ( 'NONE',  ( -4.466732464217805898, 19.42663028452474450, -231.9485309169485561 ) ) ;
#2983=CARTESIAN_POINT ( 'NONE',  ( 13.19406830060760605, 4.163358546877222288, -228.8532745215267425 ) ) ;
#2984=CARTESIAN_POINT ( 'NONE',  ( 3.137667653003819446, 15.44806861187908176, -232.6841782316817842 ) ) ;
#2985=CARTESIAN_POINT ( 'NONE',  ( 19.19076252585518105, -11.68002947460017715, -233.4322573972352188 ) ) ;
#2988=CARTESIAN_POINT ( 'NONE',  ( -24.24202834850560606, 19.05981756344202438, -226.6980666352953335 ) ) ;
#2989=CARTESIAN_POINT ( 'NONE',  ( -10.66474234094022755, -20.68992156881482813, -215.8674331684499634 ) ) ;
#2991=CARTESIAN_POINT ( 'NONE',  ( 14.39473142419577023, 15.98257177912839389, -217.4557725731239373 ) ) ;
#2995=FACE_OUTER_BOUND ( 'NONE', #18266, .T. ) ;
#2996=CARTESIAN_POINT ( 'NONE',  ( -14.95675039876920032, 11.42095949000369259, -217.2220932760075129 ) ) ;
#2997=CARTESIAN_POINT ( 'NONE',  ( 25.85597688020959239, 3.954559836939000039, -230.6766427064781624 ) ) ;
#2999=CARTESIAN_POINT ( 'NONE',  ( 14.72991611006397861, 0.1487069797637389501, -222.0036671020463359 ) ) ;
#3002=CARTESIAN_POINT ( 'NONE',  ( 15.95205345792057550, -4.116367354408478896, -227.2937718740910498 ) ) ;
#3003=CARTESIAN_POINT ( 'NONE',  ( -15.89118508636071958, -1.798691612803976492, -229.3605869667087234 ) ) ;
#3006=CARTESIAN_POINT ( 'NONE',  ( 10.48640380280471618, 25.27581435651469022, -227.8976696013017715 ) ) ;
#3007=CARTESIAN_POINT ( 'NONE',  ( 4.565444334214069144, -15.90021673156186388, -218.4840512714275462 ) ) ;
#3008=CARTESIAN_POINT ( 'NONE',  ( 9.358654279681809740, -11.94480763145079472, -229.8864256833185777 ) ) ;
#3009=CARTESIAN_POINT ( 'NONE',  ( -20.71192633727912380, 6.339941255257877550, -217.2401662359725094 ) ) ;
#3010=CARTESIAN_POINT ( 'NONE',  ( -16.98287383830707142, 1.584866439881522648, -221.5391863673846444 ) ) ;
#3011=CARTESIAN_POINT ( 'NONE',  ( 13.80707869872719762, 6.429545566348308760, -225.7152177910682553 ) ) ;
#3014=CARTESIAN_POINT ( 'NONE',  ( 4.683166109028750412, -21.42534054955530110, -233.6038185840237986 ) ) ;
#3016=CARTESIAN_POINT ( 'NONE',  ( -26.09112266552012471, 5.807188091516064077, -215.7774933166620883 ) ) ;
#3017=CARTESIAN_POINT ( 'NONE',  ( 19.20222574149634909, 21.83532798770326266, -218.6913543321078919 ) ) ;
#3018=CARTESIAN_POINT ( 'NONE',  ( -0.2758005215353623862, 11.79991891162212525, -226.8645588387054488 ) ) ;
#3019=CARTESIAN_POINT ( 'NONE',  ( 15.93530172229541364, -10.24337635388110890, -230.8272463582829630 ) ) ;
#3020=CARTESIAN_POINT ( 'NONE',  ( -6.201839134465864767, 11.37481922992157379, -223.7040893475979146 ) ) ;
#3021=CARTESIAN_POINT ( 'NONE',  ( -15.82069055112642353, 8.315535108674763976, -217.2800172218543935 ) ) ;
#3022=CARTESIAN_POINT ( 'NONE',  ( 7.283976506941576723, 24.82246917020504284, -234.3244871078919402 ) ) ;
#3023=CARTESIAN_POINT ( 'NONE',  ( -22.70558257617108922, 14.65737936663030538, -230.9775454010380997 ) ) ;
#3024=CARTESIAN_POINT ( 'NONE',  ( -8.501641725227710111, 25.47064987787527102, -217.3358698761548737 ) ) ;
#3027=CARTESIAN_POINT ( 'NONE',  ( 7.249842700832647147, 18.24319783868832801, -219.1110502051974720 ) ) ;
#3028=CARTESIAN_POINT ( 'NONE',  ( 25.69761320619099720, -8.403105518750903613, -219.2599777650661110 ) ) ;
#3031=CARTESIAN_POINT ( 'NONE',  ( 21.60524407607017849, 3.028118258437591415, -217.8361640396714449 ) ) ;
#3032=CARTESIAN_POINT ( 'NONE',  ( -15.97267037792306255, -23.58045393237649279, -221.6247985403941527 ) ) ;
#3035=CARTESIAN_POINT ( 'NONE',  ( -16.84845737324940984, 22.31296517946017488, -228.8910390263689010 ) ) ;
#3036=CARTESIAN_POINT ( 'NONE',  ( 18.70674991763376482, -20.04093309878971496, -230.8534322170362714 ) ) ;
#3037=CARTESIAN_POINT ( 'NONE',  ( 11.54460987479198053, 9.649171130674412566, -228.7280371210653698 ) ) ;
#3038=CARTESIAN_POINT ( 'NONE',  ( -7.464187997994982560, 14.20693289415472016, -228.8865298551900764 ) ) ;
#3039=CARTESIAN_POINT ( 'NONE',  ( -9.060295054034883222, 29.20313342278041802, -224.2979742714222482 ) ) ;
#3041=CARTESIAN_POINT ( 'NONE',  ( -12.96306772261163154, -8.963621967909368493, -225.1938837381851215 ) ) ;
#3042=CARTESIAN_POINT ( 'NONE',  ( 16.22460398937575121, -0.7285105026664867589, -219.3274985887512116 ) ) ;
#3045=CARTESIAN_POINT ( 'NONE',  ( -30.56371166594826150, 0.09613004385584933420, -226.3268674980304525 ) ) ;
#3046=CARTESIAN_POINT ( 'NONE',  ( 10.12956299421491302, 11.38773431477224385, -230.3175791991728829 ) ) ;
#3047=CARTESIAN_POINT ( 'NONE',  ( -16.88145396433676027, 5.002512658926777434, -221.2364783498041731 ) ) ;
#3048=CARTESIAN_POINT ( 'NONE',  ( 10.66732316618037402, 25.78610527446713263, -216.5597036843431624 ) ) ;
#3049=CARTESIAN_POINT ( 'NONE',  ( 13.15438416660314225, 5.520603777723624539, -227.0878346348094681 ) ) ;
#3050=CARTESIAN_POINT ( 'NONE',  ( -11.17605908769978740, -26.51801958233905765, -230.6004191093659301 ) ) ;
#3052=CARTESIAN_POINT ( 'NONE',  ( -18.96646980336054611, -22.16549408654085696, -227.7928771762007329 ) ) ;
#3053=CARTESIAN_POINT ( 'NONE',  ( -28.12586305337175219, 12.75764838638491305, -230.3810511299127768 ) ) ;
#3054=CARTESIAN_POINT ( 'NONE',  ( 14.65870393774896030, -26.09170264574407838, -221.2973805112574723 ) ) ;
#3055=CARTESIAN_POINT ( 'NONE',  ( -28.46519324992292965, -8.397260794665152517, -225.6705986409035347 ) ) ;
#3057=CARTESIAN_POINT ( 'NONE',  ( -14.37894460687751597, -1.926260335694933268, -225.0161641904981593 ) ) ;
#3059=CARTESIAN_POINT ( 'NONE',  ( 14.91731358302415877, 13.33846450914490056, -217.2468882285060658 ) ) ;
#3061=CARTESIAN_POINT ( 'NONE',  ( -21.75607741976026333, 20.26169853110213381, -228.4128163609909450 ) ) ;
#3062=CARTESIAN_POINT ( 'NONE',  ( 23.08329078023534109, 11.96623404944238978, -217.1428499060670845 ) ) ;
#3063=CARTESIAN_POINT ( 'NONE',  ( 18.29617186523616468, 23.20920553663278341, -223.4372550713720216 ) ) ;
#3064=CARTESIAN_POINT ( 'NONE',  ( 9.489894741926459432, 25.96007012349547338, -222.3210984495278524 ) ) ;
#3066=CARTESIAN_POINT ( 'NONE',  ( 13.52447848812844100, -22.07588418332509050, -234.6412735253872484 ) ) ;
#3067=CARTESIAN_POINT ( 'NONE',  ( -5.529079411693809121, 13.00503897727793401, -226.8014833675713646 ) ) ;
#3070=CARTESIAN_POINT ( 'NONE',  ( 11.57669841200422134, 10.63052136557218574, -228.9489978335593889 ) ) ;
#3071=CARTESIAN_POINT ( 'NONE',  ( 6.466495776945791363, -21.72297233841655029, -216.6235280138562302 ) ) ;
#3072=CARTESIAN_POINT ( 'NONE',  ( -24.39036648059286350, 13.21953970265592027, -220.1632778389106591 ) ) ;
#3075=CARTESIAN_POINT ( 'NONE',  ( 8.860681144154234801, 27.11956268701432293, -229.8503778060109823 ) ) ;
#3077=CARTESIAN_POINT ( 'NONE',  ( -16.21268175593173311, -5.852138355245464219, -231.1837890105803410 ) ) ;
#3079=CARTESIAN_POINT ( 'NONE',  ( -22.10934047915413814, 0.9940043559354462266, -218.9999999999999716 ) ) ;
#3081=CARTESIAN_POINT ( 'NONE',  ( 15.23494377589453919, 15.24947835004434538, -215.7641128510430519 ) ) ;
#3083=CARTESIAN_POINT ( 'NONE',  ( -1.249406995060579062, 25.48934319316224162, -216.9406480707515072 ) ) ;
#3084=CARTESIAN_POINT ( 'NONE',  ( 23.21483485987735307, -16.21330837850192097, -225.6840547952056397 ) ) ;
#3085=CARTESIAN_POINT ( 'NONE',  ( 14.46917091355089902, -8.493370822347547033, -231.7163745456035997 ) ) ;
#3087=CARTESIAN_POINT ( 'NONE',  ( 4.559463107227270662, 13.27337529356814017, -226.9596205199204633 ) ) ;
#3088=CARTESIAN_POINT ( 'NONE',  ( -18.91688971021567767, -12.73417920357403688, -235.2301191595167040 ) ) ;
#3089=CARTESIAN_POINT ( 'NONE',  ( 5.569356713096689226, -12.06902110579006226, -223.1407905962607003 ) ) ;
#3090=CARTESIAN_POINT ( 'NONE',  ( 17.15627899979664051, -18.64955541608202694, -217.1729447097152388 ) ) ;
#3091=CARTESIAN_POINT ( 'NONE',  ( -16.90193019167508126, 18.45790510038867893, -217.5707532411249758 ) ) ;
#3092=CARTESIAN_POINT ( 'NONE',  ( 12.60818910183731489, 13.02403301690871729, -229.3305689548085695 ) ) ;
#3094=CARTESIAN_POINT ( 'NONE',  ( -12.27164519775873686, 10.97713184439464840, -231.6269036897678291 ) ) ;
#3095=CARTESIAN_POINT ( 'NONE',  ( -16.02814206296035593, -12.75525137407698040, -230.7643788161867633 ) ) ;
#3098=CARTESIAN_POINT ( 'NONE',  ( -5.365396334125453137, 16.47374957271378904, -219.4721119688156534 ) ) ;
#3099=CARTESIAN_POINT ( 'NONE',  ( 28.03290210476798094, 13.48017620089690638, -224.9212082181537937 ) ) ;
#3100=CARTESIAN_POINT ( 'NONE',  ( -6.593106361191484410, 26.27107262772703322, -231.8730401762632596 ) ) ;
#3101=CARTESIAN_POINT ( 'NONE',  ( 11.97732832373273126, -6.576952149368169742, -223.6031523087739572 ) ) ;
#3103=VERTEX_POINT ( 'NONE', #11445 ) ;
#3104=CARTESIAN_POINT ( 'NONE',  ( -9.151299407007059017, 9.196974979111923076, -223.9483834032048719 ) ) ;
#3105=CARTESIAN_POINT ( 'NONE',  ( -14.03169683822311420, -2.573853926495621725, -218.3324423281324016 ) ) ;
#3107=CARTESIAN_POINT ( 'NONE',  ( 11.62313423782632782, 11.98467543564608029, -219.7293303032897995 ) ) ;
#3110=CARTESIAN_POINT ( 'NONE',  ( 19.06435866915521515, -20.24829071055443563, -218.8318535520223804 ) ) ;
#3112=CARTESIAN_POINT ( 'NONE',  ( -20.54164754914381064, 7.122791156791981493, -233.5720402887671980 ) ) ;
#3114=CARTESIAN_POINT ( 'NONE',  ( -13.25293905438448405, 17.39325876214774524, -215.6628841494472510 ) ) ;
#3115=CARTESIAN_POINT ( 'NONE',  ( 28.09488075336259527, 3.911739131332936381, -227.7543364642411632 ) ) ;
#3116=CARTESIAN_POINT ( 'NONE',  ( -5.139154528335864391, -14.05392405596956529, -226.2842807754188641 ) ) ;
#3118=CARTESIAN_POINT ( 'NONE',  ( 16.91879448796214191, 0.8271603773820436212, -230.0510230802265710 ) ) ;
#3120=CARTESIAN_POINT ( 'NONE',  ( 15.68576712525985251, -3.705577278900763716, -224.6781181500375908 ) ) ;
#3121=CARTESIAN_POINT ( 'NONE',  ( -22.51170993270524789, -14.32174306031543054, -231.7292175355062795 ) ) ;
#3124=CARTESIAN_POINT ( 'NONE',  ( 5.195682580001069084, 14.86321519495278665, -224.7851167466743334 ) ) ;
#3125=CARTESIAN_POINT ( 'NONE',  ( 11.19883971596842720, -26.43874323075700161, -218.8478122585937626 ) ) ;
#3126=CARTESIAN_POINT ( 'NONE',  ( 21.05631363308661363, -21.50266115212419393, -222.6654548186096747 ) ) ;
#3127=CARTESIAN_POINT ( 'NONE',  ( -11.85645341316062051, 18.51497629668490674, -217.8828067666886454 ) ) ;
#3128=CARTESIAN_POINT ( 'NONE',  ( 12.81769551943392393, 4.437328497131001193, -221.7762769673541072 ) ) ;
#3129=CARTESIAN_POINT ( 'NONE',  ( 28.52435124311170966, 7.611291969169514005, -224.8315247833735384 ) ) ;
#3130=CARTESIAN_POINT ( 'NONE',  ( -6.114698591673049854, -22.00309638965383030, -231.6969144128436540 ) ) ;
#3132=CARTESIAN_POINT ( 'NONE',  ( -13.91932826323387395, 8.983986115891950064, -216.4624824187541776 ) ) ;
#3133=CARTESIAN_POINT ( 'NONE',  ( 3.490345297502855715, 11.17751288514984331, -224.7799703251421022 ) ) ;
#3134=CARTESIAN_POINT ( 'NONE',  ( 9.638496285600583136, -13.08983061985817464, -223.8709389748426588 ) ) ;
#3135=CARTESIAN_POINT ( 'NONE',  ( 1.217121169770782663, 15.31158828575123110, -230.6845728599757308 ) ) ;
#3136=CARTESIAN_POINT ( 'NONE',  ( -29.30406754532526037, 5.063969254119831120, -221.8212091093853076 ) ) ;
#3137=CARTESIAN_POINT ( 'NONE',  ( 18.99256614858759207, 26.22894869843687715, -224.5811130452664202 ) ) ;
#3138=CARTESIAN_POINT ( 'NONE',  ( -16.75232826114664775, 4.232868982398014346, -229.4158550594996200 ) ) ;
#3139=CARTESIAN_POINT ( 'NONE',  ( -6.855867220396999251, 12.17758473459128332, -220.6375607554995213 ) ) ;
#3141=CARTESIAN_POINT ( 'NONE',  ( 4.152856881432678726, 16.71326706899027670, -228.3712188091315909 ) ) ;
#3145=CARTESIAN_POINT ( 'NONE',  ( -31.76239872120898511, 5.177298019713663990, -226.5714959923072342 ) ) ;
#3146=CARTESIAN_POINT ( 'NONE',  ( -18.87172488519036762, -12.11125346135639802, -231.2159161446224402 ) ) ;
#3148=CARTESIAN_POINT ( 'NONE',  ( -7.375127652145912371, 13.01042140126078195, -223.9959097520547004 ) ) ;
#3149=CARTESIAN_POINT ( 'NONE',  ( 1.967796959512672306, -15.42100964229427085, -222.1538042820122314 ) ) ;
#3150=CARTESIAN_POINT ( 'NONE',  ( 16.82251835652528982, 18.18719385133374544, -231.8032941011735772 ) ) ;
#3151=CARTESIAN_POINT ( 'NONE',  ( -16.84845737324940984, 22.31296517946017488, -228.8910390263689010 ) ) ;
#3152=CARTESIAN_POINT ( 'NONE',  ( -7.312583518931054627, 16.22063427959223958, -217.3454962955413521 ) ) ;
#3154=CARTESIAN_POINT ( 'NONE',  ( -16.09675311661892039, -3.241155435977624677, -226.6155721728984531 ) ) ;
#3155=CARTESIAN_POINT ( 'NONE',  ( 7.762960416026701616, 12.60702317161859121, -221.9096828323375235 ) ) ;
#3157=CARTESIAN_POINT ( 'NONE',  ( -25.11055959288653128, 8.701823109978603199, -230.2231080656787583 ) ) ;
#3158=CARTESIAN_POINT ( 'NONE',  ( 26.50744623559791435, 1.694095366541529923, -217.6968951254705473 ) ) ;
#3160=CARTESIAN_POINT ( 'NONE',  ( 27.02029988085337919, -0.4174685747284823112, -230.1188858631967378 ) ) ;
#3161=CARTESIAN_POINT ( 'NONE',  ( 11.96568375430165254, 8.504117401580989721, -219.8633768076029753 ) ) ;
#3162=CARTESIAN_POINT ( 'NONE',  ( -15.19607346356906952, 9.485739149828241068, -229.2407115334993080 ) ) ;
#3163=CARTESIAN_POINT ( 'NONE',  ( -3.162425552858488143, 20.40327580806445695, -216.0004724541873316 ) ) ;
#3164=CARTESIAN_POINT ( 'NONE',  ( 20.02669998934234741, 11.93441252203826508, -216.7824909737982182 ) ) ;
#3165=CARTESIAN_POINT ( 'NONE',  ( -8.465184826868526358, -8.692222964613778302, -225.5402182279159149 ) ) ;
#3167=CARTESIAN_POINT ( 'NONE',  ( -10.30161254035895091, -9.966167094494833734, -223.3409979381218875 ) ) ;
#3169=CARTESIAN_POINT ( 'NONE',  ( -12.14471622011552832, 3.716031503296523653, -220.6237729066402835 ) ) ;
#3170=CARTESIAN_POINT ( 'NONE',  ( 7.088126259304779353, -19.25156530781288566, -233.7785425911077937 ) ) ;
#3171=CARTESIAN_POINT ( 'NONE',  ( 20.72180063689699026, -9.651256082433341987, -234.7026181832539180 ) ) ;
#3172=CARTESIAN_POINT ( 'NONE',  ( -14.48876282330270016, -2.056064607042531911, -223.6537127325441361 ) ) ;
#3173=CARTESIAN_POINT ( 'NONE',  ( 22.22999428328319382, 14.15012104770485557, -232.1858878619060249 ) ) ;
#3174=CARTESIAN_POINT ( 'NONE',  ( -10.52776196018457711, 13.57482816453351937, -219.2327734183297423 ) ) ;
#3175=CARTESIAN_POINT ( 'NONE',  ( 22.22999428328319382, 14.15012104770485557, -232.1858878619060249 ) ) ;
#3176=CARTESIAN_POINT ( 'NONE',  ( 10.07175337281514871, 14.76776740066196325, -231.7834566702614723 ) ) ;
#3177=CARTESIAN_POINT ( 'NONE',  ( 14.02816775221371337, 20.58276248714641810, -218.7180790146936999 ) ) ;
#3178=CARTESIAN_POINT ( 'NONE',  ( 21.11934605992122727, -20.14300392389669270, -232.3867613253685249 ) ) ;
#3179=CARTESIAN_POINT ( 'NONE',  ( -6.255852670334142829, 13.96671599789818252, -220.4426911866496823 ) ) ;
#3183=CARTESIAN_POINT ( 'NONE',  ( 9.500235314199413139, -15.98409598254677455, -218.3811512014305265 ) ) ;
#3184=CARTESIAN_POINT ( 'NONE',  ( -14.57944476639264764, 6.129437248167259433, -229.4766146696829310 ) ) ;
#3185=CARTESIAN_POINT ( 'NONE',  ( 0.8374361358884788720, 23.73768315274483953, -232.4065959030912154 ) ) ;
#3187=CARTESIAN_POINT ( 'NONE',  ( -13.72709560065558421, -5.132649126379569715, -227.9317987811764965 ) ) ;
#3188=CARTESIAN_POINT ( 'NONE',  ( 17.91327661571172314, 1.545939370248587075, -216.9938266089438912 ) ) ;
#3189=CARTESIAN_POINT ( 'NONE',  ( 9.100443535964535258, 24.01370002727352215, -234.5397711707082635 ) ) ;
#3191=CARTESIAN_POINT ( 'NONE',  ( -1.881996891245037995, 28.05344686410985489, -218.6379207300106202 ) ) ;
#3192=CARTESIAN_POINT ( 'NONE',  ( 12.63976474005154493, -11.16289257830726278, -221.8494566150397134 ) ) ;
#3193=CARTESIAN_POINT ( 'NONE',  ( 28.81324478616323148, -9.895151559995404966, -227.1624192579662918 ) ) ;
#3195=CARTESIAN_POINT ( 'NONE',  ( 9.586902571418640662, 24.43292817174309661, -231.9968623198229807 ) ) ;
#3196=CARTESIAN_POINT ( 'NONE',  ( -30.46088052942827318, -8.161173215405806758, -225.9185547777119893 ) ) ;
#3197=CARTESIAN_POINT ( 'NONE',  ( 0.04660897052267574947, -31.13860575300111577, -224.7746869833732717 ) ) ;
#3198=CARTESIAN_POINT ( 'NONE',  ( 19.68037530048075112, -17.97179847169212508, -231.8517058357153076 ) ) ;
#3199=CARTESIAN_POINT ( 'NONE',  ( -22.57344584932824105, 14.14390280519600473, -217.2212543695777924 ) ) ;
#3201=CARTESIAN_POINT ( 'NONE',  ( 7.497537106193371770, 19.52448593130572618, -231.1338690134634248 ) ) ;
#3202=CARTESIAN_POINT ( 'NONE',  ( -15.48255455842386219, 10.01793346089237069, -233.1197357361336913 ) ) ;
#3203=CARTESIAN_POINT ( 'NONE',  ( -20.76981451797363576, 10.27702766794165257, -234.3988437453480742 ) ) ;
#3204=CARTESIAN_POINT ( 'NONE',  ( -14.26213125333782727, -4.747741064748048245, -225.2154851558723294 ) ) ;
#3206=CARTESIAN_POINT ( 'NONE',  ( -10.40174557315337900, 22.75579539577861965, -231.4492192189165962 ) ) ;
#3207=CARTESIAN_POINT ( 'NONE',  ( 14.50618777373884960, 4.375057440872940795, -230.8807389798650433 ) ) ;
#3208=CARTESIAN_POINT ( 'NONE',  ( 5.179557175392591972, 10.46258103618983881, -224.6216839350439614 ) ) ;
#3209=CARTESIAN_POINT ( 'NONE',  ( 26.86480837698434243, -8.606671353193281249, -231.2046318962545683 ) ) ;
#3211=ORIENTED_EDGE ( 'NONE', *, *, #4968, .T. ) ;
#3212=CARTESIAN_POINT ( 'NONE',  ( -23.98802705797876200, 19.46654170242919690, -223.5293093576406989 ) ) ;
#3213=CARTESIAN_POINT ( 'NONE',  ( -29.95626564321166541, -9.027512590954497540, -220.3228832733970819 ) ) ;
#3215=CARTESIAN_POINT ( 'NONE',  ( 10.78187269046063435, 10.73871010366167944, -221.9206544238666368 ) ) ;
#3217=CARTESIAN_POINT ( 'NONE',  ( 15.54083024098960486, -10.44392130763852222, -217.6620978190037476 ) ) ;
#3218=CARTESIAN_POINT ( 'NONE',  ( -29.95012366401462955, 4.746560250930182967, -224.6954343660969471 ) ) ;
#3219=CARTESIAN_POINT ( 'NONE',  ( -8.329232059016652201, 11.81357365351366617, -230.1839637212758021 ) ) ;
#3220=CARTESIAN_POINT ( 'NONE',  ( 28.56567312134318826, 3.451746495494312672, -224.1550573921799412 ) ) ;
#3221=CARTESIAN_POINT ( 'NONE',  ( -4.902442737337177725, -13.94343087703807704, -224.3742458082145959 ) ) ;
#3223=CARTESIAN_POINT ( 'NONE',  ( 15.05360126642391450, 1.481754003466396963, -222.9454997252120734 ) ) ;
#3225=CARTESIAN_POINT ( 'NONE',  ( 11.76368234164141136, -12.26645877504561888, -220.6132173800162946 ) ) ;
#3226=CARTESIAN_POINT ( 'NONE',  ( 12.88473959921682166, -2.638886110283121589, -223.5604664187585229 ) ) ;
#3228=CARTESIAN_POINT ( 'NONE',  ( 6.332229114051408203, 16.75791367489523154, -229.7702805136205200 ) ) ;
#3229=CARTESIAN_POINT ( 'NONE',  ( 5.646952844456516019, 23.06006924884521325, -218.8221376988549878 ) ) ;
#3230=CARTESIAN_POINT ( 'NONE',  ( 16.60513614482655598, -17.51558294309126396, -234.8138649271977556 ) ) ;
#3231=CARTESIAN_POINT ( 'NONE',  ( 13.47054497134856277, -24.75371201277411615, -218.7687119198782000 ) ) ;
#3233=CARTESIAN_POINT ( 'NONE',  ( -16.84845737324940984, 22.31296517946017488, -228.8910390263689010 ) ) ;
#3234=CARTESIAN_POINT ( 'NONE',  ( 22.42925200799500729, 5.652256920629083581, -234.0734181799116698 ) ) ;
#3235=CARTESIAN_POINT ( 'NONE',  ( 24.38255093784924199, 7.851200578213498815, -231.2687759850219607 ) ) ;
#3237=CARTESIAN_POINT ( 'NONE',  ( -3.190684129821126813, -24.11035010539542611, -218.3286195476113392 ) ) ;
#3239=CARTESIAN_POINT ( 'NONE',  ( -13.00859847561873117, 4.399982435993697649, -231.0885370824921097 ) ) ;
#3241=CARTESIAN_POINT ( 'NONE',  ( 14.65697969206133067, 11.40587726087447606, -233.3943609825344652 ) ) ;
#3242=CARTESIAN_POINT ( 'NONE',  ( 11.33829581046623858, -17.80819325066959635, -230.7883484307220385 ) ) ;
#3243=CARTESIAN_POINT ( 'NONE',  ( 7.995304978256253747, 13.28024228361502779, -220.6535174700288451 ) ) ;
#3244=CARTESIAN_POINT ( 'NONE',  ( -27.82842955277035202, 11.70195273568964112, -227.9294339757464911 ) ) ;
#3245=CARTESIAN_POINT ( 'NONE',  ( 8.373295497769937867, 8.203271496719947820, -226.1884629658694053 ) ) ;
#3246=CARTESIAN_POINT ( 'NONE',  ( -13.43384090552117271, 6.057765724406720231, -225.7182623230366119 ) ) ;
#3247=CARTESIAN_POINT ( 'NONE',  ( -9.740348021262962064, 16.12529029871877384, -216.4361617420699702 ) ) ;
#3248=CARTESIAN_POINT ( 'NONE',  ( 15.05360126642391450, 1.481754003466396963, -222.9454997252120734 ) ) ;
#3249=CARTESIAN_POINT ( 'NONE',  ( 8.115778909262310492, -29.92983049028717346, -224.5060555478150377 ) ) ;
#3253=CARTESIAN_POINT ( 'NONE',  ( -14.48876282330270016, -2.056064607042531911, -223.6537127325441361 ) ) ;
#3254=CARTESIAN_POINT ( 'NONE',  ( -20.02994071726468661, 1.326980477106467271, -234.9527056834518532 ) ) ;
#3255=CARTESIAN_POINT ( 'NONE',  ( -20.29356827505781879, -18.19569389227462253, -221.0297756488607490 ) ) ;
#3258=CARTESIAN_POINT ( 'NONE',  ( 5.625090746907006611, -14.93184515622287201, -221.0486942310484721 ) ) ;
#3259=CARTESIAN_POINT ( 'NONE',  ( 11.41090957555148222, 16.52772439454343711, -218.2458222691329013 ) ) ;
#3260=CARTESIAN_POINT ( 'NONE',  ( -13.51991436508781597, 16.61129329384914755, -232.1184346153593197 ) ) ;
#3261=CARTESIAN_POINT ( 'NONE',  ( -16.89013823391154290, 26.38860451648245231, -225.6449744083545852 ) ) ;
#3263=CARTESIAN_POINT ( 'NONE',  ( 28.26377063890550190, -1.722554810693586180, -217.1290174754948623 ) ) ;
#3265=CARTESIAN_POINT ( 'NONE',  ( 10.57926812561479757, 10.00910231482511215, -225.8341706491384286 ) ) ;
#3266=CARTESIAN_POINT ( 'NONE',  ( -22.32700334442577272, 3.978587747811427988, -218.4803616146862453 ) ) ;
#3267=CARTESIAN_POINT ( 'NONE',  ( 30.57915561709945251, 3.468229287067555067, -223.8876084027091906 ) ) ;
#3269=CARTESIAN_POINT ( 'NONE',  ( 12.96449997971774870, 8.285709878278680662, -230.9518598506670628 ) ) ;
#3270=CARTESIAN_POINT ( 'NONE',  ( -27.32939371162572684, 5.861081283609568260, -224.9659309793921409 ) ) ;
#3271=CARTESIAN_POINT ( 'NONE',  ( 6.523529190399725231, 13.69551997595937465, -217.3678933099786832 ) ) ;
#3272=CARTESIAN_POINT ( 'NONE',  ( 21.14328650935969023, 6.072767611243683916, -217.6422864096696514 ) ) ;
#3273=CARTESIAN_POINT ( 'NONE',  ( -7.835169104947472540, -15.11139199849201908, -217.2594261031170220 ) ) ;
#3275=CARTESIAN_POINT ( 'NONE',  ( -19.65071121466273496, -22.30814805266854606, -225.1308016072272267 ) ) ;
#3277=CARTESIAN_POINT ( 'NONE',  ( -20.87212828950092813, -0.8819659211619411687, -215.0000000018925448 ) ) ;
#3278=CARTESIAN_POINT ( 'NONE',  ( 8.021672912688133650, -23.92397517040199872, -233.3380040120402441 ) ) ;
#3279=CARTESIAN_POINT ( 'NONE',  ( -2.735889804569492600, 12.71735652435744512, -225.1194195722198117 ) ) ;
#3280=CARTESIAN_POINT ( 'NONE',  ( 12.01003603113874441, -9.270215614621081457, -232.3219482526175170 ) ) ;
#3281=CARTESIAN_POINT ( 'NONE',  ( -18.11268275035277853, -3.459088653808292335, -218.4233329573673359 ) ) ;
#3282=CARTESIAN_POINT ( 'NONE',  ( 13.71882454279727526, 6.278400000045776252, -230.2269611870541723 ) ) ;
#3284=CARTESIAN_POINT ( 'NONE',  ( -17.07051451008491938, 15.19890664381897949, -233.6014043774825666 ) ) ;
#3285=CARTESIAN_POINT ( 'NONE',  ( 11.83256327006771969, 5.988634687709346593, -225.8999299265561831 ) ) ;
#3287=CARTESIAN_POINT ( 'NONE',  ( 12.23063869552301242, 12.84118223717021934, -218.8273164334868284 ) ) ;
#3288=CARTESIAN_POINT ( 'NONE',  ( 6.402706778685327116, 14.41397785959879307, -226.0127495172349086 ) ) ;
#3289=CARTESIAN_POINT ( 'NONE',  ( -3.642659482353215239, -13.10753628101701018, -222.6432544668793980 ) ) ;
#3290=CARTESIAN_POINT ( 'NONE',  ( -6.804439720554941395, 15.25609613835249156, -218.7834354895107651 ) ) ;
#3291=CARTESIAN_POINT ( 'NONE',  ( 18.46552355142154411, 5.019711608606525211, -231.5099115070375433 ) ) ;
#3292=CARTESIAN_POINT ( 'NONE',  ( 8.958604797576050771, -20.52636309154128114, -232.6441826665315205 ) ) ;
#3293=CARTESIAN_POINT ( 'NONE',  ( -22.38347148959098121, 12.58966534755613687, -218.4978713241202399 ) ) ;
#3294=CARTESIAN_POINT ( 'NONE',  ( -4.583529401292260275, 28.77615850237956607, -226.7744741901706504 ) ) ;
#3295=CARTESIAN_POINT ( 'NONE',  ( -19.50907964299920039, -17.77536300509877876, -217.8007844881196320 ) ) ;
#3296=CARTESIAN_POINT ( 'NONE',  ( 20.13946171159960841, -0.1427001808266660232, -233.7987036390019853 ) ) ;
#3298=CARTESIAN_POINT ( 'NONE',  ( 10.82528077991200810, 8.849546035972329250, -221.2068619981234008 ) ) ;
#3300=CARTESIAN_POINT ( 'NONE',  ( -2.735889804569492600, 12.71735652435744512, -225.1194195722198117 ) ) ;
#3301=CARTESIAN_POINT ( 'NONE',  ( 16.50219604690516206, -6.005650786285340104, -230.9082164827931933 ) ) ;
#3302=CARTESIAN_POINT ( 'NONE',  ( 14.79879825009101069, -3.130997509566451953, -219.4569190381675696 ) ) ;
#3305=CARTESIAN_POINT ( 'NONE',  ( -3.855805549595750392, 26.68244055262801950, -232.4569730455296508 ) ) ;
#3306=CARTESIAN_POINT ( 'NONE',  ( -27.49927005802855717, -8.180762508579555004, -232.0193187950690970 ) ) ;
#3307=CARTESIAN_POINT ( 'NONE',  ( -15.48425879135615446, -25.29886615046042309, -220.6886037686364261 ) ) ;
#3308=CARTESIAN_POINT ( 'NONE',  ( 13.99926435381047618, -21.11851526759364006, -232.9234173943665951 ) ) ;
#3309=CARTESIAN_POINT ( 'NONE',  ( -11.07173923371951574, 9.938770595667456575, -229.9381419817434562 ) ) ;
#3310=CARTESIAN_POINT ( 'NONE',  ( 17.35243190875273811, 16.67741344734974263, -230.5744436858935558 ) ) ;
#3311=CARTESIAN_POINT ( 'NONE',  ( -18.08305592660031991, 4.022743421239192152, -217.2335041149100050 ) ) ;
#3312=CARTESIAN_POINT ( 'NONE',  ( -11.07173923371951574, 9.938770595667456575, -229.9381419817434562 ) ) ;
#3313=CARTESIAN_POINT ( 'NONE',  ( -12.03049011398204726, -11.12540611457240480, -223.2385418847515268 ) ) ;
#3317=CARTESIAN_POINT ( 'NONE',  ( -6.720912670637915198, 19.69156892798266512, -217.8848069150180891 ) ) ;
#3318=CARTESIAN_POINT ( 'NONE',  ( 28.65393683769942967, 4.398063292302325067, -219.1542358361629965 ) ) ;
#3319=CARTESIAN_POINT ( 'NONE',  ( 11.50837930502119733, 10.86662242793286381, -233.1728506169798436 ) ) ;
#3320=CARTESIAN_POINT ( 'NONE',  ( 12.31594623278127720, -7.047777776961618557, -228.0736214755532956 ) ) ;
#3323=CARTESIAN_POINT ( 'NONE',  ( -3.514547081416551588, 30.38636916157537016, -227.3529586180979436 ) ) ;
#3324=CARTESIAN_POINT ( 'NONE',  ( -22.78031074599627814, -9.151179398885634697, -235.0532497368941733 ) ) ;
#3326=CARTESIAN_POINT ( 'NONE',  ( 26.48990917286906921, 12.16675355942207659, -225.0153622588060216 ) ) ;
#3327=CARTESIAN_POINT ( 'NONE',  ( -18.46722752239034193, 0.9784074152395518809, -232.1633353206286188 ) ) ;
#3328=CARTESIAN_POINT ( 'NONE',  ( 21.05631363308661363, -21.50266115212419393, -222.6654548186096747 ) ) ;
#3329=CARTESIAN_POINT ( 'NONE',  ( -26.02440924314744919, 2.824604386891162111, -232.0644005296583430 ) ) ;
#3331=CARTESIAN_POINT ( 'NONE',  ( 24.60354977307301283, 7.993510024274534942, -218.5358880819990759 ) ) ;
#3332=CARTESIAN_POINT ( 'NONE',  ( 1.250172743705837641, -19.35180105203422940, -231.6553945523530729 ) ) ;
#3335=CARTESIAN_POINT ( 'NONE',  ( 15.42212722119060864, 5.401662248084913465, -220.8333402320903645 ) ) ;
#3336=CARTESIAN_POINT ( 'NONE',  ( -16.15126510923403202, -0.4755054218165427615, -219.3066569788202571 ) ) ;
#3337=CARTESIAN_POINT ( 'NONE',  ( 15.80653577316150837, -24.09293983082412893, -226.7583346419201575 ) ) ;
#3338=CARTESIAN_POINT ( 'NONE',  ( 14.80787930410854081, -2.237450434840648761, -227.0005678990481215 ) ) ;
#3340=CARTESIAN_POINT ( 'NONE',  ( 8.647507700742417924, 16.42978512283924175, -220.3082116258600536 ) ) ;
#3341=CARTESIAN_POINT ( 'NONE',  ( 10.01015180241662605, 20.19019600914695900, -219.1042218506083543 ) ) ;
#3342=CARTESIAN_POINT ( 'NONE',  ( 11.05135090310477786, -21.04892152267781569, -234.3520113253972568 ) ) ;
#3343=CARTESIAN_POINT ( 'NONE',  ( 9.584731462935641488, -12.36622837314704348, -230.4796538097028531 ) ) ;
#3345=CARTESIAN_POINT ( 'NONE',  ( -8.611121136347097860, 17.46802294375265419, -231.5575697815534113 ) ) ;
#3346=CARTESIAN_POINT ( 'NONE',  ( -14.47418542577149836, 8.806675964858893479, -228.0010566307936699 ) ) ;
#3347=CARTESIAN_POINT ( 'NONE',  ( 17.02590609996173754, 6.796709046606974169, -230.8496778635019098 ) ) ;
#3349=CARTESIAN_POINT ( 'NONE',  ( -5.110696651857618455, -18.61886646437566384, -231.2604145522360000 ) ) ;
#3354=CARTESIAN_POINT ( 'NONE',  ( 23.04342321161690776, 14.90264581583150694, -218.4777833225197412 ) ) ;
#3355=CARTESIAN_POINT ( 'NONE',  ( 13.80508996112396680, -23.93364289317450400, -226.6703843709330783 ) ) ;
#3356=CARTESIAN_POINT ( 'NONE',  ( 10.85888002857596923, 15.81835858589122878, -232.3913150909872627 ) ) ;
#3357=CARTESIAN_POINT ( 'NONE',  ( -17.75316132689678383, 25.03468689048078843, -222.1645193425721061 ) ) ;
#3359=CARTESIAN_POINT ( 'NONE',  ( 5.964915545484365644, 11.50358694729900577, -229.9646467236423462 ) ) ;
#3360=CARTESIAN_POINT ( 'NONE',  ( -19.27153818831731158, 23.75761453444584248, -221.9111479746408975 ) ) ;
#3362=CARTESIAN_POINT ( 'NONE',  ( 0.4042326456706432647, 15.50845657815858303, -219.2680337625893401 ) ) ;
#3363=CARTESIAN_POINT ( 'NONE',  ( 21.60524407607017849, 3.028118258437591415, -217.8361640396714449 ) ) ;
#3365=CARTESIAN_POINT ( 'NONE',  ( 7.437838793555467731, -20.85539581353325289, -233.9154700400843865 ) ) ;
#3366=CARTESIAN_POINT ( 'NONE',  ( 24.59129902578158067, -8.191391589517788674, -218.4338547727923299 ) ) ;
#3368=CARTESIAN_POINT ( 'NONE',  ( -15.15819830826754355, -2.370657588173597841, -221.8013720140894236 ) ) ;
#3369=CARTESIAN_POINT ( 'NONE',  ( -13.63292518690856170, 3.968236334994402981, -218.3158317831635316 ) ) ;
#3370=CARTESIAN_POINT ( 'NONE',  ( -10.64756522805915395, -11.91724881161430361, -221.7317784521105750 ) ) ;
#3372=CARTESIAN_POINT ( 'NONE',  ( 13.65368867897269389, -25.84127502057983605, -227.3223880387346867 ) ) ;
#3373=CARTESIAN_POINT ( 'NONE',  ( -24.15814485343234352, 4.373587128574028426, -232.6698675874553430 ) ) ;
#3374=CARTESIAN_POINT ( 'NONE',  ( 3.846342036506673612, 16.55327908958690131, -231.1358846258000597 ) ) ;
#3375=CARTESIAN_POINT ( 'NONE',  ( -4.558896566524145655, 13.01459016691503301, -228.3167740496058684 ) ) ;
#3377=CARTESIAN_POINT ( 'NONE',  ( 22.16968511661848495, 1.542591969257128826, -234.6098499860488857 ) ) ;
#3379=CARTESIAN_POINT ( 'NONE',  ( 10.50530447320976535, 20.19629329636330084, -217.1354359361034767 ) ) ;
#3380=CARTESIAN_POINT ( 'NONE',  ( -21.28804099221702018, -0.9277163183344186992, -219.0000000002572733 ) ) ;
#3381=CARTESIAN_POINT ( 'NONE',  ( -19.92987771446595957, 11.92619342620000999, -232.5382020162021206 ) ) ;
#3382=CARTESIAN_POINT ( 'NONE',  ( -14.03072379416114757, -18.13329758221107824, -232.5220584501505812 ) ) ;
#3384=APPLICATION_CONTEXT ( 'automotive_design' ) ;
#3387=CARTESIAN_POINT ( 'NONE',  ( -18.33565906012873725, 9.491905303418088025, -219.1855745749628568 ) ) ;
#3388=CARTESIAN_POINT ( 'NONE',  ( 2.892356176081334773, 24.03953794589038395, -215.3901262983647200 ) ) ;
#3389=CARTESIAN_POINT ( 'NONE',  ( 11.41911493375616260, 8.796695304819765582, -229.7440655656592412 ) ) ;
#3390=CARTESIAN_POINT ( 'NONE',  ( -3.174954051807135080, -13.80109495427747746, -226.5796556275459750 ) ) ;
#3392=CARTESIAN_POINT ( 'NONE',  ( -8.465333986790207987, -12.59497810381903982, -228.1424919783533198 ) ) ;
#3393=CARTESIAN_POINT ( 'NONE',  ( -16.96626096607909417, 26.06638125783293347, -227.3272535207661349 ) ) ;
#3394=CARTESIAN_POINT ( 'NONE',  ( 10.40291689048662782, -13.87512507945592333, -231.9656913702303029 ) ) ;
#3395=CARTESIAN_POINT ( 'NONE',  ( 0.9046320824004248085, 13.39785254849979701, -226.4815711199935890 ) ) ;
#3396=CARTESIAN_POINT ( 'NONE',  ( 10.56186985702850833, -7.684747726859879613, -229.4341029534429026 ) ) ;
#3397=CARTESIAN_POINT ( 'NONE',  ( -13.22951852716680676, -5.246159916193459338, -223.7538483380451453 ) ) ;
#3398=CARTESIAN_POINT ( 'NONE',  ( -20.45797657813638182, 1.164962349958370336, -217.1306074022350572 ) ) ;
#3401=CARTESIAN_POINT ( 'NONE',  ( -8.115738378024497379, 16.90402287339461296, -219.0833473190803034 ) ) ;
#3402=CARTESIAN_POINT ( 'NONE',  ( 18.75523091462765990, 19.46592657336209697, -230.4909883316157391 ) ) ;
#3404=CARTESIAN_POINT ( 'NONE',  ( 14.95414693437772868, 8.262206471704862665, -230.1862972580043163 ) ) ;
#3405=CARTESIAN_POINT ( 'NONE',  ( 20.47387447818710271, 7.390772095927000684, -234.0991886097562258 ) ) ;
#3406=CARTESIAN_POINT ( 'NONE',  ( -0.8305687497496098137, -27.95880702065288759, -232.3543905114424888 ) ) ;
#3408=CARTESIAN_POINT ( 'NONE',  ( -6.094651895680649467, 13.59752566126439177, -221.0608041154719103 ) ) ;
#3409=CARTESIAN_POINT ( 'NONE',  ( 16.64225601860865211, 1.926018578292457928, -220.2177910260893725 ) ) ;
#3410=CARTESIAN_POINT ( 'NONE',  ( 2.697602325873029727, -29.85947730167685421, -229.1126320946688111 ) ) ;
#3411=CARTESIAN_POINT ( 'NONE',  ( -22.13857085231108712, 6.545953331035805789, -217.2801712530867633 ) ) ;
#3412=CARTESIAN_POINT ( 'NONE',  ( -0.5888410438786807477, 14.99789765555501475, -227.7044550383138244 ) ) ;
#3413=CARTESIAN_POINT ( 'NONE',  ( -28.46519324992292965, -8.397260794665152517, -225.6705986409035347 ) ) ;
#3414=CARTESIAN_POINT ( 'NONE',  ( 14.46993441875745390, 0.2699826811589002284, -230.0986938382904157 ) ) ;
#3416=CARTESIAN_POINT ( 'NONE',  ( 17.81160404892403193, 9.939217752910943560, -216.9646549374535311 ) ) ;
#3418=CARTESIAN_POINT ( 'NONE',  ( 7.762960416026701616, 12.60702317161859121, -221.9096828323375235 ) ) ;
#3419=CARTESIAN_POINT ( 'NONE',  ( 15.40548389857710987, -8.435137368586953954, -220.3367290259554920 ) ) ;
#3420=CIRCLE ( 'NONE', #1632, 1.000000000000000888 ) ;
#3421=CARTESIAN_POINT ( 'NONE',  ( 12.44471834243122466, -10.90083019301730083, -219.2211511521849161 ) ) ;
#3422=CARTESIAN_POINT ( 'NONE',  ( 11.62313423782632782, 11.98467543564608029, -219.7293303032897995 ) ) ;
#3423=CARTESIAN_POINT ( 'NONE',  ( -16.38285517717123341, -14.67507636997927989, -214.6561055496966901 ) ) ;
#3424=CARTESIAN_POINT ( 'NONE',  ( -1.308474130992312023, -24.58654860180777391, -216.2430112183533026 ) ) ;
#3425=CARTESIAN_POINT ( 'NONE',  ( 9.358654279681809740, -11.94480763145079472, -229.8864256833185777 ) ) ;
#3426=CARTESIAN_POINT ( 'NONE',  ( -21.12280458060320498, 13.61074013710079988, -216.5529903464332335 ) ) ;
#3427=CARTESIAN_POINT ( 'NONE',  ( 8.856360819293511710, 14.24139612884802553, -227.7731680686805475 ) ) ;
#3428=CARTESIAN_POINT ( 'NONE',  ( -15.82069055112642353, 8.315535108674763976, -217.2800172218543935 ) ) ;
#3429=CARTESIAN_POINT ( 'NONE',  ( -7.366083718505351818, 19.86648438590005838, -231.8662444779758971 ) ) ;
#3430=CARTESIAN_POINT ( 'NONE',  ( 27.76845665997775114, -9.103683020204879739, -229.9743915588940979 ) ) ;
#3432=CARTESIAN_POINT ( 'NONE',  ( -16.84845737324940984, 22.31296517946017488, -228.8910390263689010 ) ) ;
#3433=CARTESIAN_POINT ( 'NONE',  ( 22.20554449732931346, 18.01468431515759860, -218.9348803756412849 ) ) ;
#3434=CARTESIAN_POINT ( 'NONE',  ( 6.523529190399725231, 13.69551997595937465, -217.3678933099786832 ) ) ;
#3435=CARTESIAN_POINT ( 'NONE',  ( 13.66436340482409761, -13.84785698770488871, -232.6553000701566134 ) ) ;
#3439=CARTESIAN_POINT ( 'NONE',  ( -10.84997096467605182, 25.01800101807719301, -232.4518260228253155 ) ) ;
#3440=CARTESIAN_POINT ( 'NONE',  ( -16.68014207497104451, -3.425858445063780788, -215.9332308579483595 ) ) ;
#3441=CARTESIAN_POINT ( 'NONE',  ( 13.55929460187270053, 0.3562519042583365270, -227.9787723277739246 ) ) ;
#3442=CARTESIAN_POINT ( 'NONE',  ( 28.51464931495100785, 5.422321182929326966, -223.8116416110474347 ) ) ;
#3443=CARTESIAN_POINT ( 'NONE',  ( -16.15126510923403202, -0.4755054218165427615, -219.3066569788202571 ) ) ;
#3444=CARTESIAN_POINT ( 'NONE',  ( 24.80560757033128993, -15.22139526172250079, -221.3338856610240271 ) ) ;
#3445=CARTESIAN_POINT ( 'NONE',  ( -16.65698539163286540, 11.03290537638306112, -233.6474915129378758 ) ) ;
#3446=CARTESIAN_POINT ( 'NONE',  ( -13.98136146596813845, 3.850743984385103680, -228.7620665878280590 ) ) ;
#3448=CARTESIAN_POINT ( 'NONE',  ( 0.7797512750231831991, -26.58197935702783354, -230.4407411870234625 ) ) ;
#3452=CARTESIAN_POINT ( 'NONE',  ( 13.39501375133567329, -10.34300172232987691, -228.1452887455185987 ) ) ;
#3454=CARTESIAN_POINT ( 'NONE',  ( 12.82662589338795556, -3.005951546645926786, -225.0248285060761759 ) ) ;
#3456=CARTESIAN_POINT ( 'NONE',  ( 9.653903571287008489, 19.16609876806546353, -219.1149796918802792 ) ) ;
#3457=CARTESIAN_POINT ( 'NONE',  ( 5.909674498212842408, 15.76475534640655773, -228.4922217450045139 ) ) ;
#3458=CARTESIAN_POINT ( 'NONE',  ( 20.52151979663716830, -23.02670487196117222, -229.5295066797569348 ) ) ;
#3459=CARTESIAN_POINT ( 'NONE',  ( 11.31395536621571019, -8.070181239749643964, -225.0898076798974614 ) ) ;
#3461=PRODUCT_DEFINITION_FORMATION_WITH_SPECIFIED_SOURCE ( 'ANY', '', #6909, .NOT_KNOWN. ) ;
#3462=CARTESIAN_POINT ( 'NONE',  ( -11.08731210905863840, 25.61052584666692766, -228.9953606804266997 ) ) ;
#3463=CARTESIAN_POINT ( 'NONE',  ( -15.47996233766743934, 8.203483081506188768, -221.0931279926996353 ) ) ;
#3464=CARTESIAN_POINT ( 'NONE',  ( -14.37318171526297483, 2.227741863946853140, -231.7654527934561202 ) ) ;
#3466=CARTESIAN_POINT ( 'NONE',  ( -1.044869047506413517, -25.54243019362050404, -231.6194713969048564 ) ) ;
#3469=CARTESIAN_POINT ( 'NONE',  ( 24.78377098693636427, 3.871650763546384155, -231.3521132786341923 ) ) ;
#3470=CARTESIAN_POINT ( 'NONE',  ( 13.61677703237491777, -11.64725695657166682, -220.6715806775949034 ) ) ;
#3471=CARTESIAN_POINT ( 'NONE',  ( 8.812073984913094904, 13.12649198322903210, -229.9172071780580495 ) ) ;
#3472=CARTESIAN_POINT ( 'NONE',  ( -24.02434186778878455, 18.57431834865475651, -228.2662945587547370 ) ) ;
#3473=CARTESIAN_POINT ( 'NONE',  ( 14.81251837262747983, -1.020578734748967209, -221.0290343291311785 ) ) ;
#3475=CARTESIAN_POINT ( 'NONE',  ( 6.093530912645064745, 16.79941505724243811, -232.1766444656230419 ) ) ;
#3476=CARTESIAN_POINT ( 'NONE',  ( 27.04607490430786854, 4.607450003618843049, -220.3758934308003461 ) ) ;
#3477=CARTESIAN_POINT ( 'NONE',  ( 1.752757082432757185, -17.15725705531007250, -232.7539178101738742 ) ) ;
#3478=CARTESIAN_POINT ( 'NONE',  ( 23.44296991241933981, -12.51566675729016964, -231.4065378011870564 ) ) ;
#3480=PRODUCT_DEFINITION_SHAPE ( 'NONE', 'NONE',  #6018 ) ;
#3482=CARTESIAN_POINT ( 'NONE',  ( -20.87212828950092813, -0.8819659211619411687, -215.0000000018925448 ) ) ;
#3483=CARTESIAN_POINT ( 'NONE',  ( -12.33332453308451804, -15.34461866416700282, -218.5928953102074388 ) ) ;
#3484=CARTESIAN_POINT ( 'NONE',  ( 7.680972971696337304, -18.49313070787806623, -217.8811398819712508 ) ) ;
#3486=CARTESIAN_POINT ( 'NONE',  ( -26.02492405343843984, 6.940268742526972900, -218.8798307745116460 ) ) ;
#3487=CARTESIAN_POINT ( 'NONE',  ( 10.25948093768852054, 28.38842464930171872, -224.3436940787075855 ) ) ;
#3488=CARTESIAN_POINT ( 'NONE',  ( -16.23478446547628096, 26.31175924651574149, -222.4178907105033431 ) ) ;
#3490=CARTESIAN_POINT ( 'NONE',  ( 18.01918173885548313, -1.728726289433203611, -215.5890043894241330 ) ) ;
#3491=ORIENTED_EDGE ( 'NONE', *, *, #7092, .F. ) ;
#3492=CARTESIAN_POINT ( 'NONE',  ( 23.04897566969193079, 17.95862962700741861, -223.6438515760422661 ) ) ;
#3493=CARTESIAN_POINT ( 'NONE',  ( -11.19223248830523332, 8.463078350427430507, -222.6400917074981578 ) ) ;
#3494=CARTESIAN_POINT ( 'NONE',  ( -18.63458318964815774, 8.046101765467303935, -217.8151248213926863 ) ) ;
#3495=CARTESIAN_POINT ( 'NONE',  ( -19.43452863239301820, -21.19996443032342626, -221.1427059245750399 ) ) ;
#3497=CARTESIAN_POINT ( 'NONE',  ( 13.86383614057800884, 4.939477956453596441, -219.6543243356308324 ) ) ;
#3498=CARTESIAN_POINT ( 'NONE',  ( -18.02718827071834085, 20.33515877052379395, -229.5060669840136143 ) ) ;
#3499=CARTESIAN_POINT ( 'NONE',  ( 22.66015888791822519, 10.43487984001084534, -234.3950629709119937 ) ) ;
#3500=CARTESIAN_POINT ( 'NONE',  ( 17.81160404892403193, 9.939217752910943560, -216.9646549374535311 ) ) ;
#3501=CARTESIAN_POINT ( 'NONE',  ( -30.53557093151922430, -9.496448454471346778, -222.0905184547210638 ) ) ;
#3503=CARTESIAN_POINT ( 'NONE',  ( -8.011291865669539547, -12.94570094964118923, -221.6322823144945744 ) ) ;
#3504=CARTESIAN_POINT ( 'NONE',  ( -6.331039912586185814, 17.62337457105953220, -233.2305561356360499 ) ) ;
#3505=CARTESIAN_POINT ( 'NONE',  ( 6.260999666360449467, -13.19315344885661645, -220.2890618333529744 ) ) ;
#3506=CARTESIAN_POINT ( 'NONE',  ( -3.643097910890548796, 22.16888955197135047, -233.9701981029593298 ) ) ;
#3507=CARTESIAN_POINT ( 'NONE',  ( 16.95735638057670869, -14.83641200555466355, -235.2222363121530293 ) ) ;
#3508=CARTESIAN_POINT ( 'NONE',  ( -16.21268175593173311, -5.852138355245464219, -231.1837890105803410 ) ) ;
#3509=CARTESIAN_POINT ( 'NONE',  ( 29.01678366425524658, 8.126504218505314014, -229.6975090854573125 ) ) ;
#3511=CARTESIAN_POINT ( 'NONE',  ( -6.208492967940078877, 16.71913201805454463, -230.4912298573936766 ) ) ;
#3512=CARTESIAN_POINT ( 'NONE',  ( -18.05576253097465766, 2.935622250037499104, -232.1557308718028594 ) ) ;
#3513=CARTESIAN_POINT ( 'NONE',  ( 7.995304978256253747, 13.28024228361502779, -220.6535174700288451 ) ) ;
#3514=CARTESIAN_POINT ( 'NONE',  ( 26.06405806384012536, 5.488112530166501024, -216.5020692413490622 ) ) ;
#3515=CARTESIAN_POINT ( 'NONE',  ( 4.525470981882147470, -27.64997114140619416, -217.1529231092339103 ) ) ;
#3516=CARTESIAN_POINT ( 'NONE',  ( 2.471991688031208945, 13.88348721647344419, -230.6707754746932437 ) ) ;
#3518=CARTESIAN_POINT ( 'NONE',  ( -8.215923615656011592, -19.99105411527736820, -235.1422105638354481 ) ) ;
#3519=CARTESIAN_POINT ( 'NONE',  ( -16.84845737324940984, 22.31296517946017488, -228.8910390263689010 ) ) ;
#3520=CARTESIAN_POINT ( 'NONE',  ( 2.535512286608554433, 13.86868953312499109, -224.9313928733152181 ) ) ;
#3521=CARTESIAN_POINT ( 'NONE',  ( -15.19144047750087267, -10.24270553329939304, -232.4311702607364793 ) ) ;
#3522=CARTESIAN_POINT ( 'NONE',  ( -21.18474081038989354, 8.486062504918864491, -230.7949373529753530 ) ) ;
#3524=CARTESIAN_POINT ( 'NONE',  ( 13.09827881591457022, 28.40264942367575784, -221.1045935444571455 ) ) ;
#3526=CARTESIAN_POINT ( 'NONE',  ( 4.730976410881341465, 17.65764351829336931, -217.6025626048331674 ) ) ;
#3527=CARTESIAN_POINT ( 'NONE',  ( 14.02135871364020936, -4.809710560857269002, -224.5109434094503911 ) ) ;
#3528=CARTESIAN_POINT ( 'NONE',  ( 16.18295504345472580, -4.390854861972272261, -232.0514848646187716 ) ) ;
#3529=CARTESIAN_POINT ( 'NONE',  ( -3.010752168931037698, 15.84372070116375575, -223.4060793985500482 ) ) ;
#3531=CARTESIAN_POINT ( 'NONE',  ( 15.89706143421296147, 10.57416387607782227, -218.3862415393350318 ) ) ;
#3532=CARTESIAN_POINT ( 'NONE',  ( -14.71809293534535534, -5.923356948231951691, -217.5005292165803041 ) ) ;
#3533=CARTESIAN_POINT ( 'NONE',  ( -0.1947256686167265494, -30.94043057420685727, -223.1178397439027492 ) ) ;
#3534=CARTESIAN_POINT ( 'NONE',  ( 21.39922646226391478, -21.53954253117021977, -224.1701659532164967 ) ) ;
#3535=CARTESIAN_POINT ( 'NONE',  ( -6.564517230509238743, 23.65597541655194647, -219.1225629381441991 ) ) ;
#3537=CARTESIAN_POINT ( 'NONE',  ( 24.14003655968566520, 13.76285650325712773, -228.1266575292093819 ) ) ;
#3539=CARTESIAN_POINT ( 'NONE',  ( -24.02434186778878455, 18.57431834865475651, -228.2662945587547370 ) ) ;
#3540=CARTESIAN_POINT ( 'NONE',  ( -15.72555926117677139, 17.60926865496976745, -217.2114552733360142 ) ) ;
#3541=CARTESIAN_POINT ( 'NONE',  ( 15.91397826126795323, -3.183288324723350549, -218.2846031002558504 ) ) ;
#3543=CARTESIAN_POINT ( 'NONE',  ( 5.955271202636533090, 21.50135983300913267, -233.0184468368920534 ) ) ;
#3544=CARTESIAN_POINT ( 'NONE',  ( 21.04928763009552384, -0.2309942901367783852, -233.9427286327411366 ) ) ;
#3545=CARTESIAN_POINT ( 'NONE',  ( 9.986779374595107228, 29.47523823012521049, -229.5287702428778687 ) ) ;
#3547=CARTESIAN_POINT ( 'NONE',  ( 8.158223302632384488, -13.44420475212243993, -229.3230086144918403 ) ) ;
#3550=CARTESIAN_POINT ( 'NONE',  ( -9.740348021262962064, 16.12529029871877384, -216.4361617420699702 ) ) ;
#3551=CARTESIAN_POINT ( 'NONE',  ( -25.64743926792790063, -18.08564893845128907, -228.9187414798782925 ) ) ;
#3553=CARTESIAN_POINT ( 'NONE',  ( 21.53262694368047647, 11.06794636811408594, -231.8394491640143826 ) ) ;
#3554=CARTESIAN_POINT ( 'NONE',  ( -21.08008464085897060, -0.9048411197481797119, -217.0000000010748522 ) ) ;
#3555=CARTESIAN_POINT ( 'NONE',  ( 14.68556740487494849, -6.365102927765655672, -229.6664356779805587 ) ) ;
#3557=CARTESIAN_POINT ( 'NONE',  ( -8.966714183099560032, 19.05224306381768073, -234.0879867025980445 ) ) ;
#3558=CARTESIAN_POINT ( 'NONE',  ( -20.54164754914381064, 7.122791156791981493, -233.5720402887671980 ) ) ;
#3559=CARTESIAN_POINT ( 'NONE',  ( -0.3025942668150596315, -28.96010673020088788, -223.5534481764385646 ) ) ;
#3562=CARTESIAN_POINT ( 'NONE',  ( -12.31207293045244988, 6.732038552366256923, -221.0952066824360713 ) ) ;
#3563=CARTESIAN_POINT ( 'NONE',  ( 13.96153919378708075, -19.04487818418218481, -231.5728976975466367 ) ) ;
#3564=CARTESIAN_POINT ( 'NONE',  ( 13.66359280701490420, -1.647215465832199355, -222.4923211118234008 ) ) ;
#3567=CARTESIAN_POINT ( 'NONE',  ( 13.72034832542693827, 10.98995328009155692, -220.6189139471235592 ) ) ;
#3568=CARTESIAN_POINT ( 'NONE',  ( -7.329856113536736828, 10.17606210583481818, -226.3085553030691415 ) ) ;
#3569=CARTESIAN_POINT ( 'NONE',  ( 19.59567110982616001, 18.11097967140601028, -228.7314497914969706 ) ) ;
#3570=CARTESIAN_POINT ( 'NONE',  ( -5.427686778165598191, -19.74436295060356272, -231.6150980610854901 ) ) ;
#3571=CARTESIAN_POINT ( 'NONE',  ( 11.88751558872989378, -3.770303194171726435, -225.3699946362665969 ) ) ;
#3573=CARTESIAN_POINT ( 'NONE',  ( -2.435715273212520238, 23.41098772907853132, -217.6796576669356966 ) ) ;
#3574=CARTESIAN_POINT ( 'NONE',  ( -18.92390258637512090, 12.75887082072172163, -230.9970325548277970 ) ) ;
#3575=CARTESIAN_POINT ( 'NONE',  ( -20.05025075566126702, 1.207204931470905018, -215.1628017022767949 ) ) ;
#3576=CARTESIAN_POINT ( 'NONE',  ( -8.785593564164850378, -26.69987990810942691, -222.9015467003982849 ) ) ;
#3579=CARTESIAN_POINT ( 'NONE',  ( 27.79670308438203108, 10.67628923451848877, -225.2981230784098727 ) ) ;
#3580=CARTESIAN_POINT ( 'NONE',  ( 21.81705645104102587, -16.14081802208856686, -221.4047148572338131 ) ) ;
#3581=CARTESIAN_POINT ( 'NONE',  ( 4.559463107227270662, 13.27337529356814017, -226.9596205199204633 ) ) ;
#3582=CARTESIAN_POINT ( 'NONE',  ( -13.55591840520136770, 8.363404288414606924, -231.2690188357804857 ) ) ;
#3583=CARTESIAN_POINT ( 'NONE',  ( 30.57915561709945251, 3.468229287067555067, -223.8876084027091906 ) ) ;
#3584=CARTESIAN_POINT ( 'NONE',  ( 8.979547488457603421, 23.24376652602565230, -232.6628827740196357 ) ) ;
#3585=CARTESIAN_POINT ( 'NONE',  ( 13.77325227673554942, 1.931642680738434148, -222.7035726732354703 ) ) ;
#3586=CARTESIAN_POINT ( 'NONE',  ( -0.6367083786117293531, -29.73461014436635708, -220.1383336929387724 ) ) ;
#3587=CARTESIAN_POINT ( 'NONE',  ( 15.54083024098960486, -10.44392130763852222, -217.6620978190037476 ) ) ;
#3590=CARTESIAN_POINT ( 'NONE',  ( -11.87391433320165746, 8.920676825367966245, -232.2044275666449096 ) ) ;
#3591=CARTESIAN_POINT ( 'NONE',  ( -18.09422283036245460, -3.216155923901089064, -229.6485988878351918 ) ) ;
#3592=CARTESIAN_POINT ( 'NONE',  ( 13.71882454279727526, 6.278400000045776252, -230.2269611870541723 ) ) ;
#3593=CARTESIAN_POINT ( 'NONE',  ( 8.674175678922351196, 20.85307874897338110, -216.6688793998777101 ) ) ;
#3594=CARTESIAN_POINT ( 'NONE',  ( 3.522445101072706475, 23.08420003150784439, -231.7850044194335055 ) ) ;
#3596=CARTESIAN_POINT ( 'NONE',  ( -24.19871179313096476, -3.348666575842360160, -230.4488973568908534 ) ) ;
#3597=CARTESIAN_POINT ( 'NONE',  ( 11.62313423782632782, 11.98467543564608029, -219.7293303032897995 ) ) ;
#3599=CARTESIAN_POINT ( 'NONE',  ( -24.33894786102607455, 16.69464852328507831, -227.6320542475859554 ) ) ;
#3600=CARTESIAN_POINT ( 'NONE',  ( -17.89085717681497201, 10.08962028281416856, -232.3705156551908431 ) ) ;
#3601=CARTESIAN_POINT ( 'NONE',  ( -22.54883021006152433, -16.50439104605484530, -230.5104955902558004 ) ) ;
#3602=CARTESIAN_POINT ( 'NONE',  ( -14.10849459794400751, -0.2436790717799666162, -223.1085195285415921 ) ) ;
#3603=DIRECTION ( 'NONE',  ( 0.1093404791528972547, -0.9940043559354329039, 0.000000000000000000 ) ) ;
#3604=CARTESIAN_POINT ( 'NONE',  ( 15.39025625686376841, 1.044190007782545226, -218.9203249718910911 ) ) ;
#3605=CARTESIAN_POINT ( 'NONE',  ( -17.07311071032027172, 18.59516984069744794, -230.9440421721702137 ) ) ;
#3606=CARTESIAN_POINT ( 'NONE',  ( 5.179557175392591972, 10.46258103618983881, -224.6216839350439614 ) ) ;
#3607=CARTESIAN_POINT ( 'NONE',  ( -14.29986196492902550, 0.06805469746732484282, -227.4167624117703213 ) ) ;
#3608=CARTESIAN_POINT ( 'NONE',  ( -14.38198375515248273, -6.747285987484331393, -233.1569015480179985 ) ) ;
#3610=CARTESIAN_POINT ( 'NONE',  ( -14.01584329375060456, -3.774282517739922405, -220.6818330080343173 ) ) ;
#3611=CARTESIAN_POINT ( 'NONE',  ( -4.591517861330576267, 12.55780501983563191, -223.5932882008353033 ) ) ;
#3612=CARTESIAN_POINT ( 'NONE',  ( -8.803769170443210612, -17.82266517633203406, -233.6972128408098683 ) ) ;
#3613=CARTESIAN_POINT ( 'NONE',  ( -5.807479211365208727, 19.77444019604324410, -216.0778658752277863 ) ) ;
#3614=CARTESIAN_POINT ( 'NONE',  ( 30.13983206778957324, -7.413543662652124944, -226.8644184361555745 ) ) ;
#3616=CARTESIAN_POINT ( 'NONE',  ( 15.14536540539411114, 2.907144070186200580, -217.8738854795238922 ) ) ;
#3618=CARTESIAN_POINT ( 'NONE',  ( 0.1979841192334154676, 16.22068729745496540, -223.9539336445596973 ) ) ;
#3619=CARTESIAN_POINT ( 'NONE',  ( -14.07336028695978314, 1.752429266630609828, -222.9750305084206161 ) ) ;
#3620=CARTESIAN_POINT ( 'NONE',  ( 18.54610009393809023, 0.6523581019769808531, -231.1787333216317677 ) ) ;
#3621=CARTESIAN_POINT ( 'NONE',  ( 25.85827166240959940, 13.84420748389600675, -220.2831452073696425 ) ) ;
#3622=CARTESIAN_POINT ( 'NONE',  ( -3.771778814064143504, -12.72945944931849915, -225.7745976896340778 ) ) ;
#3623=CARTESIAN_POINT ( 'NONE',  ( 1.833772325875588027, 13.50593961039006707, -219.8748197804281119 ) ) ;
#3624=CARTESIAN_POINT ( 'NONE',  ( 22.03647168420945590, 0.3315607655625663064, -232.0572713672586644 ) ) ;
#3625=CARTESIAN_POINT ( 'NONE',  ( -3.564252528062037406, -12.01378896085460291, -227.6748268428467270 ) ) ;
#3626=CARTESIAN_POINT ( 'NONE',  ( -11.48592899399814726, 13.65854631785387774, -230.8311022452805616 ) ) ;
#3627=CARTESIAN_POINT ( 'NONE',  ( 15.37089934297015503, 20.64239674606488961, -217.2018742121147170 ) ) ;
#3628=CARTESIAN_POINT ( 'NONE',  ( -28.55814054826834791, -1.660722980825670048, -228.2640858091212408 ) ) ;
#3629=CARTESIAN_POINT ( 'NONE',  ( -16.58624905143161143, 8.715293938925766426, -220.0618460037763384 ) ) ;
#3631=CARTESIAN_POINT ( 'NONE',  ( -5.373457274256926652, 30.83572167890261184, -229.2199105909169532 ) ) ;
#3632=CARTESIAN_POINT ( 'NONE',  ( 17.89221702206198117, 0.2742047965568425449, -220.2420650470893122 ) ) ;
#3634=CARTESIAN_POINT ( 'NONE',  ( 18.79065350309113214, -20.33706828427738600, -226.6662063318914591 ) ) ;
#3635=CARTESIAN_POINT ( 'NONE',  ( 4.725966861008204845, -14.24791254766627624, -227.2781441550517343 ) ) ;
#3636=CARTESIAN_POINT ( 'NONE',  ( -5.125319492185865577, 20.53749879880200524, -218.7557759432853288 ) ) ;
#3637=CARTESIAN_POINT ( 'NONE',  ( 14.39473142419577023, 15.98257177912839389, -217.4557725731239373 ) ) ;
#3638=CARTESIAN_POINT ( 'NONE',  ( -14.73876579896802141, -0.4225899574144328374, -230.2531052195884342 ) ) ;
#3639=CARTESIAN_POINT ( 'NONE',  ( -1.542335193334551491, -19.71915426430242135, -216.1352730594569209 ) ) ;
#3640=CARTESIAN_POINT ( 'NONE',  ( 6.166782020495575445, -26.61202787628535660, -217.6604608484729795 ) ) ;
#3641=CARTESIAN_POINT ( 'NONE',  ( -8.316066124693966444, 26.67103469786491843, -222.2304303634109885 ) ) ;
#3643=CARTESIAN_POINT ( 'NONE',  ( 21.07144422417032104, 18.33581350331571969, -223.6711752364813890 ) ) ;
#3644=CARTESIAN_POINT ( 'NONE',  ( -23.52999999174766543, 19.39566142560855866, -221.9446938626390704 ) ) ;
#3645=CARTESIAN_POINT ( 'NONE',  ( -5.764806379010653181, 14.19340719117484007, -223.8851086052821415 ) ) ;
#3646=CARTESIAN_POINT ( 'NONE',  ( -0.5888410438786807477, 14.99789765555501475, -227.7044550383138244 ) ) ;
#3647=CARTESIAN_POINT ( 'NONE',  ( 13.93840998928060415, 0.7705246578886114639, -220.8158265847476116 ) ) ;
#3648=CARTESIAN_POINT ( 'NONE',  ( 19.48863273024974418, 12.80680990455712909, -215.0408095016468053 ) ) ;
#3649=CARTESIAN_POINT ( 'NONE',  ( 9.835929410207317147, -16.71508016877321268, -232.2716196330763694 ) ) ;
#3652=CARTESIAN_POINT ( 'NONE',  ( -0.9414827276148034496, 23.96885519606619752, -216.4491898092606164 ) ) ;
#3653=CARTESIAN_POINT ( 'NONE',  ( 16.03897629125586377, -3.546747291816754633, -223.1229430630804700 ) ) ;
#3654=CARTESIAN_POINT ( 'NONE',  ( 20.15756451863428111, -2.090604891399794774, -217.8900786001194945 ) ) ;
#3655=CIRCLE ( 'NONE', #16244, 1.000000000000000888 ) ;
#3656=CARTESIAN_POINT ( 'NONE',  ( 23.04897566969193079, 17.95862962700741861, -223.6438515760422661 ) ) ;
#3657=CARTESIAN_POINT ( 'NONE',  ( -17.88126539071149779, 5.766250685202066961, -232.9050303536861293 ) ) ;
#3658=CARTESIAN_POINT ( 'NONE',  ( 8.510712203779903007, -27.79691582975998898, -230.5316902582456180 ) ) ;
#3659=CARTESIAN_POINT ( 'NONE',  ( -9.540790481621398200, 9.981116473660406996, -228.6478862620407995 ) ) ;
#3660=ORIENTED_EDGE ( 'NONE', *, *, #1264, .F. ) ;
#3661=CARTESIAN_POINT ( 'NONE',  ( -23.49379658590067876, 11.46840048879614393, -217.2519070826072323 ) ) ;
#3662=CARTESIAN_POINT ( 'NONE',  ( -10.94940667656068634, -10.80050631132953498, -220.7362776234490127 ) ) ;
#3665=CARTESIAN_POINT ( 'NONE',  ( -24.02434186778878455, 18.57431834865475651, -228.2662945587547370 ) ) ;
#3666=CARTESIAN_POINT ( 'NONE',  ( 13.82101996411362244, -10.82539765916244789, -229.0162845096555770 ) ) ;
#3670=CARTESIAN_POINT ( 'NONE',  ( 26.92457506054779515, 6.538608665672222209, -219.8654465082432807 ) ) ;
#3671=CARTESIAN_POINT ( 'NONE',  ( -16.23478446547628096, 26.31175924651574149, -222.4178907105033431 ) ) ;
#3673=CARTESIAN_POINT ( 'NONE',  ( 12.91676121433235913, 9.519065828383201477, -226.8102878246443765 ) ) ;
#3674=CARTESIAN_POINT ( 'NONE',  ( -3.373690338999510985, -20.30281967708846125, -218.2431319494177160 ) ) ;
#3675=CARTESIAN_POINT ( 'NONE',  ( -23.14980455159086503, 0.3541108476526578785, -217.8785187302087536 ) ) ;
#3677=CARTESIAN_POINT ( 'NONE',  ( -4.583529401292260275, 28.77615850237956607, -226.7744741901706504 ) ) ;
#3678=CARTESIAN_POINT ( 'NONE',  ( -22.38528940623734798, 16.50235888036280230, -227.1443357386333162 ) ) ;
#3679=CARTESIAN_POINT ( 'NONE',  ( 14.32363442937021425, 2.978337679677412808, -227.0386046113487453 ) ) ;
#3680=CARTESIAN_POINT ( 'NONE',  ( -21.81769295881711557, -14.18202798484824534, -220.2668003432649471 ) ) ;
#3683=CARTESIAN_POINT ( 'NONE',  ( 28.56567312134318826, 3.451746495494312672, -224.1550573921799412 ) ) ;
#3684=CARTESIAN_POINT ( 'NONE',  ( 0.5565384680698680642, -16.73444667301361122, -219.8404036742738015 ) ) ;
#3685=CARTESIAN_POINT ( 'NONE',  ( 11.87982377808925527, 10.85265283465803421, -229.5027252913499183 ) ) ;
#3686=CARTESIAN_POINT ( 'NONE',  ( -9.517741096562200909, 20.63709896626785678, -234.1036702156204967 ) ) ;
#3689=CARTESIAN_POINT ( 'NONE',  ( 18.03440114592047649, 4.755211820135348155, -216.3599228381250157 ) ) ;
#3690=CARTESIAN_POINT ( 'NONE',  ( 12.10245006109274080, 26.02147364279441888, -220.6079829738538649 ) ) ;
#3692=CARTESIAN_POINT ( 'NONE',  ( 2.178520447619924472, -13.56847537563065487, -221.4085897031499428 ) ) ;
#3693=CARTESIAN_POINT ( 'NONE',  ( 8.818493748348606331, -10.89961555176610375, -227.9481955143288303 ) ) ;
#3696=CARTESIAN_POINT ( 'NONE',  ( -8.653738780971721667, 11.12943719949617893, -219.7525355316396087 ) ) ;
#3697=CARTESIAN_POINT ( 'NONE',  ( -16.45250455720563210, -7.911775896682759601, -220.5271995834187067 ) ) ;
#3699=( BOUNDED_SURFACE ( )  B_SPLINE_SURFACE ( 3, 3, ( 
 ( #5962, #12839, #19683, #4600, #20119, #16993, #9682, #6295, #15316, #20458, #6752, #6406, #1575, #10017, #21927, #14861, #13620, #11923, #8110, #8447, #5046, #6635, #13169, #3136, #11702, #14976, #9790, #15200, #1120, #18789, #22163, #16541, #16881, #11477, #11584, #13276, #7996, #21704, #1456, #20014, #4707, #15091, #6517, #11815, #18344, #2905, #16655, #4825, #3244, #1236, #21817, #13506, #18458, #20343, #22046, #4939, #18682, #3021, #9906, #16769, #1348, #13386, #8219, #18572, #20230, #8329, #10128, #3582, #10572, #6861, #106, #335, #10459, #17213, #8999, #3472, #439, #15862, #17553, #17441, #5609, #8559, #1897, #18898, #2010, #17320, #13958, #14184, #3805, #20685, #15423, #8892, #8781, #15642, #7313, #21021, #14632, #2120, #6977, #13729, #222, #15756, #10689, #12489, #7091, #3357, #5491, #10240, #20794, #13848, #5374, #14069, #7203, #20905, #20569, #5267, #17106, #1685, #5157, #12037, #10350, #1787, #12147, #8662, #3686, #12258, #15524, #19003, #19109, #12375, #19226, #986, #16297, #548, #12814, #21342, #17774, #19437, #2553, #10792, #21562, #18098, #7860, #19658, #21127, #21233, #655, #3916, #6152, #11123, #14726, #7533, #2447, #9330, #21455, #17659, #19336, #12592, #14507, #12919, #10898, #9549, #873, #2339, #7751, #9437, #14621, #6044, #14401, #5823, #12702, #16410, #762, #2226, #5936, #19549, #5715, #16190, #4138, #4243, #7425, #16086, #19765, #11017, #9223, #2666, #4022, #9107, #15974, #11229, #17991, #14294, #17885, #7638, #4345, #20199, #4680, #1318, #1539, #13474, #8083, #18212, #18541, #13248, #11555, #2773, #13143, #19987, #6486, #16740, #1427, #9654, #16515, #4574, #1092, #11450, #13027, #8191, #21898, #15058, #11670, #11788, #18427, #7966, #14832, #16851, #21675, #6268, #18318, #2878, #9760, #9875, #21789, #4794, #18654, #16625, #1206, #20314, #20093, #2991, #4909, #13355, #3107, #3215, #10098, #14951, #19874, #11342, #15167, #9990, #6376, #8301, #22009, #16962, #6605, #8417, #15286, #22134, #4461, #3656, #2090, #5126, #8636, #19080, #8968, #22242, #10209, #12007, #15833, #3771, #20764, #5346, #7061, #302, #1762, #18758, #13592, #10322, #15610, #13929, #6833, #3553, #17077, #18867, #1656, #10431, #3326, #5019, #19194, #20873, #7172, #12119, #17291, #20537, #15496, #18974, #12228, #17185, #8530, #11894, #6723, #74, #1867, #13701, #20655, #10539, #8747, #12341, #14037, #20430, #190, #5459, #17408, #15394, #3442, #6945, #13816, #5238, #10657, #1980, #8861, #15725, #17523, #10764, #7284, #409, #5578, #14153, #20990, #17629, #12458, #3884, #19306, #2196, #9077, #16988 ),
 ( #16649, #1231, #8105, #11811, #18678, #4935, #13501, #13382, #1568, #4486, #20113, #14855, #6512, #13271, #9900, #10123, #22041, #14971, #11365, #4821, #21812, #4702, #18234, #21699, #6290, #15086, #3016, #10012, #2794, #9677, #13164, #16536, #20009, #21585, #16764, #8214, #1342, #20225, #20339, #3239, #8442, #1115, #6173, #2900, #7990, #18452, #11698, #6631, #13051, #11578, #19898, #1452, #4595, #21922, #9783, #6400, #16876, #18567, #3132, #11471, #8325, #18339, #15195, #7409, #17425, #8764, #12133, #16071, #318, #17538, #13944, #20889, #3900, #2104, #12578, #14279, #2323, #10674, #21113, #8985, #1881, #13833, #7187, #20669, #5253, #5699, #7075, #17644, #10776, #12244, #12475, #3568, #18988, #20778, #19421, #4007, #19094, #10883, #10445, #424, #17305, #19321, #9208, #14053, #10555, #3671, #14169, #5476, #17759, #6962, #21004, #5360, #1995, #8876, #15625, #12359, #15740, #19209, #205, #3790, #2210, #15848, #7299, #5594, #9092, #15959, #532, #9419, #7846, #6252, #2432, #19644, #4229, #12798, #14712, #14605, #4559, #7952, #21547, #747, #11108, #17977, #14817, #7735, #14492, #21440, #17870, #12687, #4444, #4121, #5806, #11002, #9315, #2540, #19751, #16283, #6138, #13127, #16176, #857, #1078, #6030, #12904, #21662, #4331, #11215, #19972, #11435, #7623, #7517, #21219, #2758, #13012, #19534, #19858, #18083, #18304, #21327, #2652, #9533, #2863, #9747, #11326, #641, #5921, #16393, #18195, #14386, #972, #9639, #16501, #11992, #13684, #8403, #15270, #16948, #10195, #11655, #6362, #1192, #20184, #3201, #1524, #16726, #13459, #20080, #6473, #4667, #20299, #13234, #14934, #6818, #8517, #17063, #21995, #4894, #21884, #18852, #11774, #1640, #4780, #18414, #21774, #3427, #9975, #18638, #1303, #8284, #13578, #10083, #22227, #15380, #16610, #22120, #20521, #6707, #11540, #8069, #16836, #2977, #9861, #5110, #8178, #5003, #20414, #13342, #11880, #15043, #18526, #3092, #1412, #15153, #6590, #18743, #3310, #3757, #1748, #15820, #5671, #3643, #12215, #507, #14024, #7383, #5444, #10524, #12106, #7158, #17394, #17509, #13801, #7045, #7268, #1968, #1852, #15929, #10417, #14251, #21084, #2182, #2076, #12549, #15483, #8846, #3537, #8956, #15712, #20860, #19396, #10750, #5333, #56, #396, #289, #12326, #6930, #17278, #8730, #10642, #19181, #20977, #20640, #5225, #15597, #18961, #176, #10307, #14138, #5565, #12443, #19293, #9063, #17170, #8622, #13917, #20752, #19068, #3870, #17616, #2620, #11296, #16474, #17947, #14787, #6109, #4413, #14575, #7592, #4201, #14683, #9502, #11185, #21191, #18051, #21629, #11080 ),
 ( #941, #21411, #9612, #18168, #6221, #7705, #2732, #6001, #5776, #10853, #2511, #17727, #2294, #1051, #4092, #21517, #7818, #9285, #16364, #614, #9179, #10969, #7924, #13096, #16146, #3979, #7489, #19723, #16042, #12980, #14358, #19616, #14461, #718, #19827, #9389, #12657, #19503, #17839, #2404, #21294, #5890, #12768, #16251, #826, #12873, #4303, #9833, #4868, #11627, #1613, #4980, #11747, #20053, #1276, #16694, #11855, #4748, #11513, #18499, #14904, #9720, #1495, #1162, #2838, #8037, #21745, #8150, #16809, #6444, #18613, #3284, #6335, #15015, #20387, #3061, #9950, #18720, #1385, #8260, #10169, #17038, #4640, #4532, #18277, #22089, #3174, #16581, #10058, #21855, #8492, #18383, #13314, #20155, #15356, #22203, #16922, #6792, #2946, #15127, #8375, #19943, #13208, #21966, #6559, #11408, #13431, #15244, #6680, #20272, #13552, #8699, #3401, #20496, #17251, #261, #20833, #13772, #10496, #17148, #3511, #1725, #17362, #10283, #11966, #3845, #5535, #14110, #19042, #1938, #18936, #15902, #8818, #20947, #1823, #15460, #18828, #481, #7014, #15683, #20611, #5305, #10611, #7131, #19265, #12413, #9037, #13997, #10725, #5415, #8599, #5085, #13888, #33, #6902, #17590, #5196, #2050, #17482, #10391, #19151, #12080, #15566, #146, #2157, #13660, #20725, #12187, #3618, #12297, #3729, #8928, #15795, #373, #7241, #7571, #21272, #12524, #7463, #14331, #804, #11056, #18030, #3954, #10829, #21165, #19373, #5752, #7356, #2488, #16228, #9368, #5980, #6085, #11274, #2709, #17700, #21495, #10943, #2268, #4180, #12855, #14662, #19805, #5863, #18143, #9480, #7797, #17924, #17815, #14437, #2599, #19697, #14552, #9151, #21388, #9592, #12744, #2380, #12961, #16455, #4389, #4067, #14223, #7683, #19591, #16013, #21059, #5647, #12632, #590, #19478, #4284, #9264, #11163, #16340, #16121, #695, #916, #14765, #3259, #22063, #11830, #16787, #2818, #2922, #4618, #7904, #10143, #15105, #18696, #11493, #6421, #13292, #3150, #21606, #4953, #16558, #18474, #16896, #14879, #13520, #20247, #6313, #11718, #6534, #4842, #13404, #18361, #9809, #16672, #20361, #4723, #1028, #3037, #1252, #9698, #20133, #8127, #8236, #4506, #20031, #18588, #14993, #21720, #6652, #1137, #6198, #13075, #15218, #21942, #19919, #11387, #21832, #8015, #10034, #11603, #9923, #13187, #18255, #1362, #1471, #8347, #3592, #12159, #15654, #15768, #20918, #12386, #6766, #8902, #20584, #22177, #13860, #234, #2022, #7215, #8674, #5507, #19121, #17453, #5278, #5170, #17225, #5384, #7104, #1911, #11939, #8793, #19236, #1798, #12052, #346, #3816, #14080, #13747 ),
 ( #20700, #17012, #19015, #18803, #1589, #15538, #8465, #15331, #13635, #17121, #12268, #20808, #6, #13968, #20470, #5062, #1699, #3373, #10254, #6875, #8571, #15436, #10469, #18909, #3701, #3486, #10362, #121, #6988, #10583, #17332, #14939, #18309, #18202, #10803, #14305, #561, #2869, #17787, #2240, #9237, #5621, #451, #14822, #14196, #15874, #21033, #12499, #7437, #7543, #19449, #2763, #16615, #19346, #21138, #11440, #2352, #16097, #9751, #668, #21552, #1197, #8074, #17669, #17563, #9009, #13132, #16506, #7328, #1083, #5725, #21780, #9122, #12605, #4036, #6367, #13239, #7957, #20084, #15984, #10915, #6143, #10699, #2132, #3928, #14717, #13017, #19863, #4449, #11331, #9644, #21667, #6257, #19978, #4565, #15385, #8521, #9980, #10200, #1308, #9865, #4785, #3432, #18857, #16841, #8627, #8182, #20419, #18418, #17067, #62, #20303, #8290, #1417, #11885, #18643, #15487, #11998, #18747, #11660, #15158, #22001, #10312, #11779, #18530, #3206, #21889, #16730, #22232, #15048, #6478, #13347, #20190, #6595, #1530, #13464, #3317, #17176, #3098, #4900, #5116, #10088, #16953, #1752, #8408, #15275, #6936, #13806, #22125, #11546, #2982, #6823, #1645, #6713, #13689, #13583, #4671, #5008, #20527, #1971, #10858, #617, #17620, #16046, #19071, #293, #10755, #7493, #13920, #1857, #3646, #20646, #17734, #12446, #19297, #20981, #14256, #15716, #10421, #5229, #8849, #7274, #5569, #20755, #17513, #8736, #10530, #15602, #2081, #17282, #18965, #2299, #12553, #21089, #3761, #8959, #17397, #12110, #15823, #5675, #7161, #180, #3543, #7050, #14028, #400, #5336, #12332, #2186, #20864, #19400, #5449, #12219, #19185, #10646, #14144, #9067, #3874, #15936, #511, #7387, #3983, #9183, #832, #21521, #19947, #16152, #11085, #14791, #21416, #6006, #6227, #4308, #2627, #13101, #4536, #14466, #21195, #12662, #16478, #19831, #4097, #4419, #9394, #11412, #21300, #16256, #17952, #18281, #16586, #11301, #9724, #12773, #7711, #18172, #1167, #7598, #17845, #19621, #14362, #2842, #6113, #12984, #14687, #7928, #14580, #10975, #5783, #2516, #946, #2736, #5896, #11190, #2409, #4206, #9291, #18056, #723, #19510, #12878, #19728, #21633, #9508, #16369, #7822, #9616, #1055, #2951, #6340, #21750, #8044, #14910, #18388, #9839, #4645, #16700, #13213, #20058, #11518, #1400, #11979, #20171, #4655, #15259, #11642, #13330, #18731, #11528, #15471, #18841, #1736, #6694, #15031, #15141, #16823, #20068, #44, #4991, #8610, #8273, #18626, #3188, #15368, #18399, #17160, #6461, #8390, #6805, #4765, #3414, #10182, #18513, #1626, #3296, #17050, #8505 ),
 ( #3079, #10071, #16712, #9963, #1291, #16936, #9849, #2963, #10295, #5098, #13672, #1511, #22106, #21982, #13222, #13566, #20509, #6576, #21872, #8165, #13446, #20286, #20401, #4882, #11761, #22214, #11867, #12534, #14235, #272, #16024, #7142, #21069, #1835, #13786, #14008, #20625, #5209, #5658, #7027, #17600, #10735, #12198, #12425, #3522, #12092, #13901, #19382, #3963, #19054, #10839, #10402, #383, #18947, #19278, #2279, #20844, #10510, #3629, #14123, #5427, #17713, #9162, #20958, #20736, #17375, #1951, #6916, #12310, #5316, #19165, #8713, #17262, #2167, #15580, #158, #8829, #15695, #3740, #10625, #17494, #5547, #2061, #8939, #15806, #7366, #7251, #3855, #9047, #15915, #493, #14776, #13085, #705, #7472, #21174, #2719, #6095, #12642, #12970, #17935, #6209, #7580, #2497, #4189, #19930, #2828, #19816, #18264, #21282, #9378, #4402, #9708, #16131, #4078, #5875, #600, #4516, #14671, #11396, #2388, #19602, #1039, #7694, #14563, #21617, #12864, #11172, #14342, #5762, #14447, #19491, #10953, #9602, #11284, #17826, #18154, #16237, #9273, #12754, #815, #11065, #21398, #5990, #16464, #19708, #4293, #18041, #7913, #2610, #9490, #16352, #927, #7806, #21506, #8361, #15232, #16908, #10156, #11614, #6322, #1149, #20143, #3163, #1484, #16683, #13419, #20041, #6433, #4628, #20259, #13196, #14891, #6778, #8479, #17026, #21954, #4855, #21841, #18816, #11732, #1601, #4736, #18371, #21731, #3388, #9935, #18600, #1262, #8248, #13537, #10047, #22190, #15342, #16797, #16568, #1372, #13647, #11502, #8026, #15116, #2933, #9821, #20483, #8138, #4966, #20374, #13302, #22077, #15003, #18486, #3048, #5074, #11952, #6546, #6666, #11843, #18708, #3271, #15784, #5636, #3606, #13874, #134, #17469, #1927, #14211, #17579, #2040, #10376, #20713, #7002, #2146, #17348, #1810, #8807, #5184, #19, #14097, #13759, #15449, #20598, #12067, #5294, #7118, #19029, #8917, #12401, #10714, #20822, #12175, #10483, #20935, #362, #7230, #18924, #5523, #12512, #15670, #249, #15889, #21046, #7344, #13984, #9026, #10600, #5400, #6889, #19361, #10270, #8687, #467, #12285, #17136, #17239, #1711, #19136, #15553, #3717, #19253, #8586, #3499, #3832, #14751, #19686, #5740, #5850, #7557, #10818, #13060, #18017, #21592, #14426, #9356, #16216, #6074, #2256, #7890, #19464, #21376, #19792, #17801, #16441, #903, #9250, #14649, #9466, #7783, #16326, #21259, #12732, #19577, #1014, #7669, #6183, #5967, #4165, #12619, #790, #11044, #11151, #7451, #683, #21481, #17910, #2368, #9578, #4053, #3942, #17687, #18128, #2584, #9138, #16001, #2475, #10929 ),
 ( #16110, #14539, #12843, #576, #14319, #12947, #21152, #4272, #4375, #11259, #2696, #13172, #1122, #18346, #15320, #16997, #11705, #18576, #20233, #13509, #14979, #9684, #4495, #1239, #6520, #4827, #20017, #16772, #7999, #4604, #13390, #1350, #8332, #16544, #14864, #11479, #2804, #2908, #19905, #15093, #3138, #21930, #10020, #18684, #1577, #22166, #21706, #11818, #8114, #6299, #8222, #16883, #4942, #10130, #11588, #8450, #22049, #20346, #1458, #21819, #20121, #15203, #6638, #3246, #9793, #6754, #11374, #4709, #6409, #18242, #16657, #13279, #18460, #3023, #9911, #3888, #18793, #17858, #16165, #12347, #12675, #2094, #19524, #20878, #5049, #15947, #19199, #14042, #19411, #11925, #735, #4110, #2421, #7401, #15729, #15837, #17527, #20460, #13624, #5688, #9304, #8973, #19310, #10767, #16061, #3360, #10242, #7177, #9081, #7507, #5464, #10989, #10871, #3779, #2311, #3995, #17747, #9196, #413, #7288, #14158, #17110, #17632, #1688, #523, #20994, #307, #2199, #5584, #21102, #8561, #10661, #631, #12464, #14270, #12566, #14374, #21208, #5795, #21762, #21648, #9850, #12787, #6125, #845, #14805, #21534, #18184, #18402, #8057, #2641, #19633, #13115, #7834, #12999, #4217, #7723, #14594, #11203, #19740, #14922, #14700, #21429, #19845, #2529, #11097, #11424, #17965, #9406, #16270, #6019, #4320, #4432, #16381, #6241, #13223, #12892, #18069, #6351, #11314, #2747, #20069, #9628, #16490, #4656, #11529, #9521, #14479, #5910, #9736, #19961, #960, #4548, #1067, #2964, #7941, #18293, #2852, #16715, #7611, #16598, #21313, #1179, #3189, #13673, #18948, #16824, #4767, #21984, #3524, #20626, #15369, #22216, #1628, #17161, #18627, #13331, #8166, #4883, #10183, #8506, #1401, #20403, #11643, #13448, #18515, #4992, #20173, #21873, #13787, #15472, #1738, #6695, #11868, #6577, #10404, #18732, #8612, #11763, #3081, #6462, #1292, #16937, #3298, #8274, #15260, #20510, #17051, #6918, #45, #1513, #15032, #8391, #5211, #9964, #15142, #22108, #20288, #10072, #12093, #13567, #11980, #5100, #6807, #18842, #3416, #10296, #17377, #16027, #9164, #275, #21178, #13903, #10738, #8715, #495, #12645, #10627, #20847, #7145, #2171, #8943, #5764, #2281, #9049, #15808, #160, #1953, #8831, #17603, #20961, #5660, #20738, #5319, #15698, #7030, #14010, #17265, #12427, #3857, #19280, #15917, #602, #19493, #4080, #12200, #7474, #5429, #19056, #14125, #7369, #14345, #1837, #385, #15582, #19384, #17715, #5549, #12313, #17496, #12537, #14237, #21071, #3632, #3967, #10512, #2063, #19167, #3742, #7253, #10841, #9275, #12756, #14449, #707, #10955 ),
 ( #17828, #7582, #2391, #16134, #21284, #19605, #5878, #13705, #15170, #15398, #6490, #15062, #9993, #8639, #1765, #22014, #13821, #13358, #3329, #1323, #22245, #5241, #3218, #13478, #6609, #17081, #1542, #20659, #17188, #1659, #16855, #20317, #4913, #15500, #16965, #1431, #8421, #4799, #21902, #20541, #20203, #11675, #18545, #3112, #11791, #6727, #18658, #8533, #78, #8304, #10102, #10325, #15289, #22138, #6949, #13595, #20433, #12122, #18978, #5022, #16743, #8194, #12012, #6836, #11898, #5129, #18760, #9878, #10213, #18870, #3445, #14268, #9080, #521, #15945, #20877, #5463, #12345, #16060, #7287, #630, #20992, #19197, #5349, #412, #3778, #10766, #7064, #306, #7400, #10660, #17413, #9195, #3659, #7506, #14373, #17745, #17631, #5794, #8752, #2093, #19084, #2198, #17526, #14156, #21207, #3994, #8971, #15613, #21101, #15836, #5583, #194, #10543, #1984, #19309, #12462, #5687, #13933, #20768, #8864, #12232, #15728, #3557, #3887, #12565, #19410, #10870, #2310, #12674, #10435, #7176, #17295, #14041, #1870, #16380, #18183, #4547, #9734, #11201, #8055, #21647, #19960, #7833, #843, #19739, #7940, #2746, #4431, #14478, #11313, #14920, #4319, #14593, #2851, #21761, #16596, #16269, #11423, #19844, #9519, #2420, #1178, #6350, #17964, #18292, #7721, #19522, #4216, #10988, #21533, #2528, #19632, #9627, #17857, #4108, #9303, #16164, #12997, #21311, #21428, #6017, #734, #7610, #16489, #5908, #12891, #2639, #958, #6239, #12786, #11096, #9405, #14699, #13113, #18068, #14803, #1066, #6124, #19020, #13527, #10474, #11944, #8680, #18702, #10040, #13409, #17338, #1593, #18808, #15224, #22183, #5176, #3379, #13865, #15544, #8470, #8242, #15336, #125, #3155, #15110, #6772, #21947, #6539, #6993, #8353, #18916, #12058, #20367, #13751, #4847, #20252, #22068, #20706, #5284, #4958, #12164, #11724, #1704, #18593, #20590, #3597, #13641, #11836, #3265, #15442, #20476, #16901, #1477, #12, #6658, #10149, #17018, #5068, #10260, #17128, #8577, #6881, #3492, #10368, #17231, #1803, #5390, #12274, #20924, #21038, #10705, #9128, #7549, #3707, #5513, #2357, #9015, #15880, #16102, #14202, #12505, #673, #14417, #2029, #8798, #240, #4041, #7443, #13973, #14310, #19242, #21249, #8908, #3823, #12392, #5841, #4155, #21143, #19568, #353, #17569, #5730, #11035, #17459, #19126, #7221, #1917, #12721, #15990, #567, #2246, #17792, #2138, #20813, #15659, #457, #10809, #12610, #15774, #5627, #10589, #14086, #7334, #19352, #3934, #7109, #17675, #19454, #10920, #9242, #2793, #1230, #19677, #14641, #18338, #2688, #9570, #9782, #7882 ) ),
 .UNSPECIFIED., .T., .F., .F. ) 
 B_SPLINE_SURFACE_WITH_KNOTS ( ( 4, 3, 4 ),
 ( 4, 2, 2, 2, 2, 2, 2, 2, 2, 2, 2, 2, 2, 2, 2, 2, 2, 2, 2, 2, 2, 2, 2, 2, 2, 2, 2, 2, 2, 2, 2, 2, 2, 2, 2, 2, 2, 2, 2, 2, 2, 2, 2, 2, 2, 2, 2, 2, 2, 2, 2, 2, 2, 2, 2, 2, 2, 2, 2, 2, 2, 2, 2, 2, 2, 2, 2, 2, 2, 2, 2, 2, 2, 2, 2, 2, 2, 2, 2, 2, 2, 2, 2, 2, 2, 2, 2, 2, 2, 2, 2, 2, 2, 2, 2, 2, 2, 2, 2, 2, 2, 2, 2, 2, 2, 2, 2, 2, 2, 2, 2, 2, 2, 2, 2, 2, 2, 2, 2, 2, 2, 2, 2, 2, 2, 2, 2, 2, 2, 2, 2, 2, 2, 2, 2, 2, 2, 2, 2, 2, 2, 2, 2, 2, 2, 2, 2, 2, 2, 2, 2, 2, 2, 2, 2, 2, 2, 2, 2, 2, 2, 2, 2, 2, 2, 2, 2, 4 ),
 ( 0.000000000000000000, 0.5000000000000000000, 1.000000000000000000 ),
 ( 0.000000000000000000, 0.001952908952989333875, 0.003905817905978667751, 0.007323408573709997045, 0.01074099924144132634, 0.01415858990917265650, 0.01586738524303832332, 0.01757618057690398666, 0.02099377124463531682, 0.02441136191236664699, 0.02782895258009797368, 0.03124654324782930384, 0.03466413391556063400, 0.03808172458329196070, 0.04149931525102329433, 0.04491690591875462102, 0.04662570125262028436, 0.04833449658648594771, 0.05175208725421727440, 0.05346088258808293775, 0.05516967792194860110, 0.05858726858967993473, 0.06200485925741126836, 0.06542244992514259505, 0.06884004059287393562, 0.07225763126060526231, 0.07567522192833658901, 0.07909281259606792958, 0.08251040326379925627, 0.08421919859766491268, 0.08592799393153058296, 0.08934558459926195129, 0.09276317526699331961, 0.09447197060085900377, 0.09618076593472468794, 0.09959835660245604239, 0.1030159472701873968, 0.1064335379379187652, 0.1098511286056501335, 0.1132687192733815018, 0.1166863099411127869, 0.1201039006088440858, 0.1235214912765753847, 0.1252302866104410273, 0.1269390819443066698, 0.1303566726120379826, 0.1320654679459036251, 0.1337742632797692677, 0.1371918539475005527, 0.1406094446152318378, 0.1440270352829631784, 0.1474446259506944912, 0.1508622166184258040, 0.1542798072861571446, 0.1576973979538884851, 0.1611149886216198257, 0.1645325792893511663, 0.1679501699570824791, 0.1713677606248137919, 0.1747853512925451325, 0.1764941466264108028, 0.1782029419602764730, 0.1816205326280078136, 0.1850381232957391542, 0.1884557139634704670, 0.1918733046312017798, 0.1952908952989331204, 0.1987084859666644610, 0.2021260766343957738, 0.2055436673021270866, 0.2072524626359927569, 0.2089612579698584272, 0.2123788486375897677, 0.2140876439714554380, 0.2157964393053211083, 0.2192140299730524489, 0.2226316206407837617, 0.2260492113085151300, 0.2294668019762464706, 0.2328843926439778111, 0.2363019833117091517, 0.2397195739794404923, 0.2431371646471718329, 0.2465547553149031734, 0.2499723459826345140, 0.2533899366503657991, 0.2568075273180971396, 0.2602251179858284802, 0.2636427086535597653, 0.2670602993212910503, 0.2704778899890223909, 0.2738954806567537315, 0.2773130713244850165, 0.2807306619922163571, 0.2841482526599476977, 0.2858570479938133957, 0.2875658433276790382, 0.2909834339954103788, 0.2926922293292760768, 0.2944010246631417194, 0.2978186153308730599, 0.3012362059986043450, 0.3046537966663356856, 0.3080713873340670261, 0.3114889780017983112, 0.3149065686695296518, 0.3183241593372609923, 0.3217417500049923329, 0.3234505453388579754, 0.3251593406727236735, 0.3285769313404549585, 0.3319945220081862991, 0.3354121126759176397, 0.3388297033436489247, 0.3422472940113802653, 0.3456648846791116059, 0.3490824753468429464, 0.3525000660145742870, 0.3559176566823056276, 0.3593352473500369682, 0.3627528380177683087, 0.3661704286854996493, 0.3695880193532309343, 0.3730056100209622749, 0.3747144053548279174, 0.3764232006886936155, 0.3798407913564249005, 0.3832583820241562411, 0.3866759726918875817, 0.3900935633596189223, 0.3935111540273502628, 0.3969287446950816034, 0.4003463353628129440, 0.4037639260305442845, 0.4054727213644099271, 0.4071815166982756251, 0.4105991073660069102, 0.4140166980337382507, 0.4157254933676038933, 0.4174342887014695913, 0.4208518793692008764, 0.4242694700369322169, 0.4276870607046635575, 0.4311046513723948981, 0.4345222420401262386, 0.4379398327078575237, 0.4413574233755888643, 0.4447750140433202048, 0.4464838093771859029, 0.4481926047110515454, 0.4516101953787828860, 0.4533189907126485840, 0.4550277860465142266, 0.4584453767142455671, 0.4618629673819769077, 0.4652805580497082483, 0.4686981487174395888, 0.4721157393851709294, 0.4755333300529022145, 0.4789509207206335550, 0.4823685113883648956, 0.4840773067222305381, 0.4857861020560961807, 0.4892036927238275212, 0.4926212833915588618, 0.4960388740592901469, 0.4979917830122794764, 0.4999446919652688059 ),
 .UNSPECIFIED. ) 
 GEOMETRIC_REPRESENTATION_ITEM ( )  RATIONAL_B_SPLINE_SURFACE ( (
 ( 1.000000000000000000, 1.000000000000000000, 1.000000000000000000, 1.000000000000000000, 1.000000000000000000, 1.000000000000000000, 1.000000000000000000, 1.000000000000000000, 1.000000000000000000, 1.000000000000000000, 1.000000000000000000, 1.000000000000000000, 1.000000000000000000, 1.000000000000000000, 1.000000000000000000, 1.000000000000000000, 1.000000000000000000, 1.000000000000000000, 1.000000000000000000, 1.000000000000000000, 1.000000000000000000, 1.000000000000000000, 1.000000000000000000, 1.000000000000000000, 1.000000000000000000, 1.000000000000000000, 1.000000000000000000, 1.000000000000000000, 1.000000000000000000, 1.000000000000000000, 1.000000000000000000, 1.000000000000000000, 1.000000000000000000, 1.000000000000000000, 1.000000000000000000, 1.000000000000000000, 1.000000000000000000, 1.000000000000000000, 1.000000000000000000, 1.000000000000000000, 1.000000000000000000, 1.000000000000000000, 1.000000000000000000, 1.000000000000000000, 1.000000000000000000, 1.000000000000000000, 1.000000000000000000, 1.000000000000000000, 1.000000000000000000, 1.000000000000000000, 1.000000000000000000, 1.000000000000000000, 1.000000000000000000, 1.000000000000000000, 1.000000000000000000, 1.000000000000000000, 1.000000000000000000, 1.000000000000000000, 1.000000000000000000, 1.000000000000000000, 1.000000000000000000, 1.000000000000000000, 1.000000000000000000, 1.000000000000000000, 1.000000000000000000, 1.000000000000000000, 1.000000000000000000, 1.000000000000000000, 1.000000000000000000, 1.000000000000000000, 1.000000000000000000, 1.000000000000000000, 1.000000000000000000, 1.000000000000000000, 1.000000000000000000, 1.000000000000000000, 1.000000000000000000, 1.000000000000000000, 1.000000000000000000, 1.000000000000000000, 1.000000000000000000, 1.000000000000000000, 1.000000000000000000, 1.000000000000000000, 1.000000000000000000, 1.000000000000000000, 1.000000000000000000, 1.000000000000000000, 1.000000000000000000, 1.000000000000000000, 1.000000000000000000, 1.000000000000000000, 1.000000000000000000, 1.000000000000000000, 1.000000000000000000, 1.000000000000000000, 1.000000000000000000, 1.000000000000000000, 1.000000000000000000, 1.000000000000000000, 1.000000000000000000, 1.000000000000000000, 1.000000000000000000, 1.000000000000000000, 1.000000000000000000, 1.000000000000000000, 1.000000000000000000, 1.000000000000000000, 1.000000000000000000, 1.000000000000000000, 1.000000000000000000, 1.000000000000000000, 1.000000000000000000, 1.000000000000000000, 1.000000000000000000, 1.000000000000000000, 1.000000000000000000, 1.000000000000000000, 1.000000000000000000, 1.000000000000000000, 1.000000000000000000, 1.000000000000000000, 1.000000000000000000, 1.000000000000000000, 1.000000000000000000, 1.000000000000000000, 1.000000000000000000, 1.000000000000000000, 1.000000000000000000, 1.000000000000000000, 1.000000000000000000, 1.000000000000000000, 1.000000000000000000, 1.000000000000000000, 1.000000000000000000, 1.000000000000000000, 1.000000000000000000, 1.000000000000000000, 1.000000000000000000, 1.000000000000000000, 1.000000000000000000, 1.000000000000000000, 1.000000000000000000, 1.000000000000000000, 1.000000000000000000, 1.000000000000000000, 1.000000000000000000, 1.000000000000000000, 1.000000000000000000, 1.000000000000000000, 1.000000000000000000, 1.000000000000000000, 1.000000000000000000, 1.000000000000000000, 1.000000000000000000, 1.000000000000000000, 1.000000000000000000, 1.000000000000000000, 1.000000000000000000, 1.000000000000000000, 1.000000000000000000, 1.000000000000000000, 1.000000000000000000, 1.000000000000000000, 1.000000000000000000, 1.000000000000000000, 1.000000000000000000, 1.000000000000000000, 1.000000000000000000, 1.000000000000000000, 1.000000000000000000, 1.000000000000000000, 1.000000000000000000, 1.000000000000000000, 1.000000000000000000, 1.000000000000000000, 1.000000000000000000, 1.000000000000000000, 1.000000000000000000, 1.000000000000000000, 1.000000000000000000, 1.000000000000000000, 1.000000000000000000, 1.000000000000000000, 1.000000000000000000, 1.000000000000000000, 1.000000000000000000, 1.000000000000000000, 1.000000000000000000, 1.000000000000000000, 1.000000000000000000, 1.000000000000000000, 1.000000000000000000, 1.000000000000000000, 1.000000000000000000, 1.000000000000000000, 1.000000000000000000, 1.000000000000000000, 1.000000000000000000, 1.000000000000000000, 1.000000000000000000, 1.000000000000000000, 1.000000000000000000, 1.000000000000000000, 1.000000000000000000, 1.000000000000000000, 1.000000000000000000, 1.000000000000000000, 1.000000000000000000, 1.000000000000000000, 1.000000000000000000, 1.000000000000000000, 1.000000000000000000, 1.000000000000000000, 1.000000000000000000, 1.000000000000000000, 1.000000000000000000, 1.000000000000000000, 1.000000000000000000, 1.000000000000000000, 1.000000000000000000, 1.000000000000000000, 1.000000000000000000, 1.000000000000000000, 1.000000000000000000, 1.000000000000000000, 1.000000000000000000, 1.000000000000000000, 1.000000000000000000, 1.000000000000000000, 1.000000000000000000, 1.000000000000000000, 1.000000000000000000, 1.000000000000000000, 1.000000000000000000, 1.000000000000000000, 1.000000000000000000, 1.000000000000000000, 1.000000000000000000, 1.000000000000000000, 1.000000000000000000, 1.000000000000000000, 1.000000000000000000, 1.000000000000000000, 1.000000000000000000, 1.000000000000000000, 1.000000000000000000, 1.000000000000000000, 1.000000000000000000, 1.000000000000000000, 1.000000000000000000, 1.000000000000000000, 1.000000000000000000, 1.000000000000000000, 1.000000000000000000, 1.000000000000000000, 1.000000000000000000, 1.000000000000000000, 1.000000000000000000, 1.000000000000000000, 1.000000000000000000, 1.000000000000000000, 1.000000000000000000, 1.000000000000000000, 1.000000000000000000, 1.000000000000000000, 1.000000000000000000, 1.000000000000000000, 1.000000000000000000, 1.000000000000000000, 1.000000000000000000, 1.000000000000000000, 1.000000000000000000, 1.000000000000000000, 1.000000000000000000, 1.000000000000000000, 1.000000000000000000, 1.000000000000000000, 1.000000000000000000, 1.000000000000000000, 1.000000000000000000, 1.000000000000000000, 1.000000000000000000, 1.000000000000000000, 1.000000000000000000, 1.000000000000000000, 1.000000000000000000, 1.000000000000000000, 1.000000000000000000, 1.000000000000000000, 1.000000000000000000, 1.000000000000000000, 1.000000000000000000, 1.000000000000000000, 1.000000000000000000, 1.000000000000000000, 1.000000000000000000, 1.000000000000000000, 1.000000000000000000, 1.000000000000000000, 1.000000000000000000, 1.000000000000000000, 1.000000000000000000, 1.000000000000000000, 1.000000000000000000, 1.000000000000000000, 1.000000000000000000, 1.000000000000000000, 1.000000000000000000, 1.000000000000000000, 1.000000000000000000, 1.000000000000000000, 1.000000000000000000, 1.000000000000000000, 1.000000000000000000, 1.000000000000000000, 1.000000000000000000, 1.000000000000000000, 1.000000000000000000, 1.000000000000000000, 1.000000000000000000, 1.000000000000000000, 1.000000000000000000, 1.000000000000000000, 1.000000000000000000, 1.000000000000000000, 1.000000000000000000, 1.000000000000000000, 1.000000000000000000, 1.000000000000000000, 1.000000000000000000, 1.000000000000000000, 1.000000000000000000, 1.000000000000000000, 1.000000000000000000, 1.000000000000000000),
 ( 0.3333333333333333703, 0.3333333333333333703, 0.3333333333333333703, 0.3333333333333333703, 0.3333333333333333703, 0.3333333333333333703, 0.3333333333333333703, 0.3333333333333333703, 0.3333333333333333703, 0.3333333333333333703, 0.3333333333333333703, 0.3333333333333333703, 0.3333333333333333703, 0.3333333333333333703, 0.3333333333333333703, 0.3333333333333333703, 0.3333333333333333703, 0.3333333333333333703, 0.3333333333333333703, 0.3333333333333333703, 0.3333333333333333703, 0.3333333333333333703, 0.3333333333333333703, 0.3333333333333333703, 0.3333333333333333703, 0.3333333333333333703, 0.3333333333333333703, 0.3333333333333333703, 0.3333333333333333703, 0.3333333333333333703, 0.3333333333333333703, 0.3333333333333333703, 0.3333333333333333703, 0.3333333333333333703, 0.3333333333333333703, 0.3333333333333333703, 0.3333333333333333703, 0.3333333333333333703, 0.3333333333333333703, 0.3333333333333333703, 0.3333333333333333703, 0.3333333333333333703, 0.3333333333333333703, 0.3333333333333333703, 0.3333333333333333703, 0.3333333333333333703, 0.3333333333333333703, 0.3333333333333333703, 0.3333333333333333703, 0.3333333333333333703, 0.3333333333333333703, 0.3333333333333333703, 0.3333333333333333703, 0.3333333333333333703, 0.3333333333333333703, 0.3333333333333333703, 0.3333333333333333703, 0.3333333333333333703, 0.3333333333333333703, 0.3333333333333333703, 0.3333333333333333703, 0.3333333333333333703, 0.3333333333333333703, 0.3333333333333333703, 0.3333333333333333703, 0.3333333333333333703, 0.3333333333333333703, 0.3333333333333333703, 0.3333333333333333703, 0.3333333333333333703, 0.3333333333333333703, 0.3333333333333333703, 0.3333333333333333703, 0.3333333333333333703, 0.3333333333333333703, 0.3333333333333333703, 0.3333333333333333703, 0.3333333333333333703, 0.3333333333333333703, 0.3333333333333333703, 0.3333333333333333703, 0.3333333333333333703, 0.3333333333333333703, 0.3333333333333333703, 0.3333333333333333703, 0.3333333333333333703, 0.3333333333333333703, 0.3333333333333333703, 0.3333333333333333703, 0.3333333333333333703, 0.3333333333333333703, 0.3333333333333333703, 0.3333333333333333703, 0.3333333333333333703, 0.3333333333333333703, 0.3333333333333333703, 0.3333333333333333703, 0.3333333333333333703, 0.3333333333333333703, 0.3333333333333333703, 0.3333333333333333703, 0.3333333333333333703, 0.3333333333333333703, 0.3333333333333333703, 0.3333333333333333703, 0.3333333333333333703, 0.3333333333333333703, 0.3333333333333333703, 0.3333333333333333703, 0.3333333333333333703, 0.3333333333333333703, 0.3333333333333333703, 0.3333333333333333703, 0.3333333333333333703, 0.3333333333333333703, 0.3333333333333333703, 0.3333333333333333703, 0.3333333333333333703, 0.3333333333333333703, 0.3333333333333333703, 0.3333333333333333703, 0.3333333333333333703, 0.3333333333333333703, 0.3333333333333333703, 0.3333333333333333703, 0.3333333333333333703, 0.3333333333333333703, 0.3333333333333333703, 0.3333333333333333703, 0.3333333333333333703, 0.3333333333333333703, 0.3333333333333333703, 0.3333333333333333703, 0.3333333333333333703, 0.3333333333333333703, 0.3333333333333333703, 0.3333333333333333703, 0.3333333333333333703, 0.3333333333333333703, 0.3333333333333333703, 0.3333333333333333703, 0.3333333333333333703, 0.3333333333333333703, 0.3333333333333333703, 0.3333333333333333703, 0.3333333333333333703, 0.3333333333333333703, 0.3333333333333333703, 0.3333333333333333703, 0.3333333333333333703, 0.3333333333333333703, 0.3333333333333333703, 0.3333333333333333703, 0.3333333333333333703, 0.3333333333333333703, 0.3333333333333333703, 0.3333333333333333703, 0.3333333333333333703, 0.3333333333333333703, 0.3333333333333333703, 0.3333333333333333703, 0.3333333333333333703, 0.3333333333333333703, 0.3333333333333333703, 0.3333333333333333703, 0.3333333333333333703, 0.3333333333333333703, 0.3333333333333333703, 0.3333333333333333703, 0.3333333333333333703, 0.3333333333333333703, 0.3333333333333333703, 0.3333333333333333703, 0.3333333333333333703, 0.3333333333333333703, 0.3333333333333333703, 0.3333333333333333703, 0.3333333333333333703, 0.3333333333333333703, 0.3333333333333333703, 0.3333333333333333703, 0.3333333333333333703, 0.3333333333333333703, 0.3333333333333333703, 0.3333333333333333703, 0.3333333333333333703, 0.3333333333333333703, 0.3333333333333333703, 0.3333333333333333703, 0.3333333333333333703, 0.3333333333333333703, 0.3333333333333333703, 0.3333333333333333703, 0.3333333333333333703, 0.3333333333333333703, 0.3333333333333333703, 0.3333333333333333703, 0.3333333333333333703, 0.3333333333333333703, 0.3333333333333333703, 0.3333333333333333703, 0.3333333333333333703, 0.3333333333333333703, 0.3333333333333333703, 0.3333333333333333703, 0.3333333333333333703, 0.3333333333333333703, 0.3333333333333333703, 0.3333333333333333703, 0.3333333333333333703, 0.3333333333333333703, 0.3333333333333333703, 0.3333333333333333703, 0.3333333333333333703, 0.3333333333333333703, 0.3333333333333333703, 0.3333333333333333703, 0.3333333333333333703, 0.3333333333333333703, 0.3333333333333333703, 0.3333333333333333703, 0.3333333333333333703, 0.3333333333333333703, 0.3333333333333333703, 0.3333333333333333703, 0.3333333333333333703, 0.3333333333333333703, 0.3333333333333333703, 0.3333333333333333703, 0.3333333333333333703, 0.3333333333333333703, 0.3333333333333333703, 0.3333333333333333703, 0.3333333333333333703, 0.3333333333333333703, 0.3333333333333333703, 0.3333333333333333703, 0.3333333333333333703, 0.3333333333333333703, 0.3333333333333333703, 0.3333333333333333703, 0.3333333333333333703, 0.3333333333333333703, 0.3333333333333333703, 0.3333333333333333703, 0.3333333333333333703, 0.3333333333333333703, 0.3333333333333333703, 0.3333333333333333703, 0.3333333333333333703, 0.3333333333333333703, 0.3333333333333333703, 0.3333333333333333703, 0.3333333333333333703, 0.3333333333333333703, 0.3333333333333333703, 0.3333333333333333703, 0.3333333333333333703, 0.3333333333333333703, 0.3333333333333333703, 0.3333333333333333703, 0.3333333333333333703, 0.3333333333333333703, 0.3333333333333333703, 0.3333333333333333703, 0.3333333333333333703, 0.3333333333333333703, 0.3333333333333333703, 0.3333333333333333703, 0.3333333333333333703, 0.3333333333333333703, 0.3333333333333333703, 0.3333333333333333703, 0.3333333333333333703, 0.3333333333333333703, 0.3333333333333333703, 0.3333333333333333703, 0.3333333333333333703, 0.3333333333333333703, 0.3333333333333333703, 0.3333333333333333703, 0.3333333333333333703, 0.3333333333333333703, 0.3333333333333333703, 0.3333333333333333703, 0.3333333333333333703, 0.3333333333333333703, 0.3333333333333333703, 0.3333333333333333703, 0.3333333333333333703, 0.3333333333333333703, 0.3333333333333333703, 0.3333333333333333703, 0.3333333333333333703, 0.3333333333333333703, 0.3333333333333333703, 0.3333333333333333703, 0.3333333333333333703, 0.3333333333333333703, 0.3333333333333333703, 0.3333333333333333703, 0.3333333333333333703, 0.3333333333333333703, 0.3333333333333333703, 0.3333333333333333703, 0.3333333333333333703, 0.3333333333333333703, 0.3333333333333333703, 0.3333333333333333703, 0.3333333333333333703, 0.3333333333333333703, 0.3333333333333333703, 0.3333333333333333703, 0.3333333333333333703, 0.3333333333333333703, 0.3333333333333333703, 0.3333333333333333703, 0.3333333333333333703, 0.3333333333333333703, 0.3333333333333333703, 0.3333333333333333703, 0.3333333333333333703, 0.3333333333333333703, 0.3333333333333333703, 0.3333333333333333703, 0.3333333333333333703, 0.3333333333333333703, 0.3333333333333333703, 0.3333333333333333703, 0.3333333333333333703, 0.3333333333333333703, 0.3333333333333333703, 0.3333333333333333703, 0.3333333333333333703, 0.3333333333333333703, 0.3333333333333333703),
 ( 0.3333333333333333703, 0.3333333333333333703, 0.3333333333333333703, 0.3333333333333333703, 0.3333333333333333703, 0.3333333333333333703, 0.3333333333333333703, 0.3333333333333333703, 0.3333333333333333703, 0.3333333333333333703, 0.3333333333333333703, 0.3333333333333333703, 0.3333333333333333703, 0.3333333333333333703, 0.3333333333333333703, 0.3333333333333333703, 0.3333333333333333703, 0.3333333333333333703, 0.3333333333333333703, 0.3333333333333333703, 0.3333333333333333703, 0.3333333333333333703, 0.3333333333333333703, 0.3333333333333333703, 0.3333333333333333703, 0.3333333333333333703, 0.3333333333333333703, 0.3333333333333333703, 0.3333333333333333703, 0.3333333333333333703, 0.3333333333333333703, 0.3333333333333333703, 0.3333333333333333703, 0.3333333333333333703, 0.3333333333333333703, 0.3333333333333333703, 0.3333333333333333703, 0.3333333333333333703, 0.3333333333333333703, 0.3333333333333333703, 0.3333333333333333703, 0.3333333333333333703, 0.3333333333333333703, 0.3333333333333333703, 0.3333333333333333703, 0.3333333333333333703, 0.3333333333333333703, 0.3333333333333333703, 0.3333333333333333703, 0.3333333333333333703, 0.3333333333333333703, 0.3333333333333333703, 0.3333333333333333703, 0.3333333333333333703, 0.3333333333333333703, 0.3333333333333333703, 0.3333333333333333703, 0.3333333333333333703, 0.3333333333333333703, 0.3333333333333333703, 0.3333333333333333703, 0.3333333333333333703, 0.3333333333333333703, 0.3333333333333333703, 0.3333333333333333703, 0.3333333333333333703, 0.3333333333333333703, 0.3333333333333333703, 0.3333333333333333703, 0.3333333333333333703, 0.3333333333333333703, 0.3333333333333333703, 0.3333333333333333703, 0.3333333333333333703, 0.3333333333333333703, 0.3333333333333333703, 0.3333333333333333703, 0.3333333333333333703, 0.3333333333333333703, 0.3333333333333333703, 0.3333333333333333703, 0.3333333333333333703, 0.3333333333333333703, 0.3333333333333333703, 0.3333333333333333703, 0.3333333333333333703, 0.3333333333333333703, 0.3333333333333333703, 0.3333333333333333703, 0.3333333333333333703, 0.3333333333333333703, 0.3333333333333333703, 0.3333333333333333703, 0.3333333333333333703, 0.3333333333333333703, 0.3333333333333333703, 0.3333333333333333703, 0.3333333333333333703, 0.3333333333333333703, 0.3333333333333333703, 0.3333333333333333703, 0.3333333333333333703, 0.3333333333333333703, 0.3333333333333333703, 0.3333333333333333703, 0.3333333333333333703, 0.3333333333333333703, 0.3333333333333333703, 0.3333333333333333703, 0.3333333333333333703, 0.3333333333333333703, 0.3333333333333333703, 0.3333333333333333703, 0.3333333333333333703, 0.3333333333333333703, 0.3333333333333333703, 0.3333333333333333703, 0.3333333333333333703, 0.3333333333333333703, 0.3333333333333333703, 0.3333333333333333703, 0.3333333333333333703, 0.3333333333333333703, 0.3333333333333333703, 0.3333333333333333703, 0.3333333333333333703, 0.3333333333333333703, 0.3333333333333333703, 0.3333333333333333703, 0.3333333333333333703, 0.3333333333333333703, 0.3333333333333333703, 0.3333333333333333703, 0.3333333333333333703, 0.3333333333333333703, 0.3333333333333333703, 0.3333333333333333703, 0.3333333333333333703, 0.3333333333333333703, 0.3333333333333333703, 0.3333333333333333703, 0.3333333333333333703, 0.3333333333333333703, 0.3333333333333333703, 0.3333333333333333703, 0.3333333333333333703, 0.3333333333333333703, 0.3333333333333333703, 0.3333333333333333703, 0.3333333333333333703, 0.3333333333333333703, 0.3333333333333333703, 0.3333333333333333703, 0.3333333333333333703, 0.3333333333333333703, 0.3333333333333333703, 0.3333333333333333703, 0.3333333333333333703, 0.3333333333333333703, 0.3333333333333333703, 0.3333333333333333703, 0.3333333333333333703, 0.3333333333333333703, 0.3333333333333333703, 0.3333333333333333703, 0.3333333333333333703, 0.3333333333333333703, 0.3333333333333333703, 0.3333333333333333703, 0.3333333333333333703, 0.3333333333333333703, 0.3333333333333333703, 0.3333333333333333703, 0.3333333333333333703, 0.3333333333333333703, 0.3333333333333333703, 0.3333333333333333703, 0.3333333333333333703, 0.3333333333333333703, 0.3333333333333333703, 0.3333333333333333703, 0.3333333333333333703, 0.3333333333333333703, 0.3333333333333333703, 0.3333333333333333703, 0.3333333333333333703, 0.3333333333333333703, 0.3333333333333333703, 0.3333333333333333703, 0.3333333333333333703, 0.3333333333333333703, 0.3333333333333333703, 0.3333333333333333703, 0.3333333333333333703, 0.3333333333333333703, 0.3333333333333333703, 0.3333333333333333703, 0.3333333333333333703, 0.3333333333333333703, 0.3333333333333333703, 0.3333333333333333703, 0.3333333333333333703, 0.3333333333333333703, 0.3333333333333333703, 0.3333333333333333703, 0.3333333333333333703, 0.3333333333333333703, 0.3333333333333333703, 0.3333333333333333703, 0.3333333333333333703, 0.3333333333333333703, 0.3333333333333333703, 0.3333333333333333703, 0.3333333333333333703, 0.3333333333333333703, 0.3333333333333333703, 0.3333333333333333703, 0.3333333333333333703, 0.3333333333333333703, 0.3333333333333333703, 0.3333333333333333703, 0.3333333333333333703, 0.3333333333333333703, 0.3333333333333333703, 0.3333333333333333703, 0.3333333333333333703, 0.3333333333333333703, 0.3333333333333333703, 0.3333333333333333703, 0.3333333333333333703, 0.3333333333333333703, 0.3333333333333333703, 0.3333333333333333703, 0.3333333333333333703, 0.3333333333333333703, 0.3333333333333333703, 0.3333333333333333703, 0.3333333333333333703, 0.3333333333333333703, 0.3333333333333333703, 0.3333333333333333703, 0.3333333333333333703, 0.3333333333333333703, 0.3333333333333333703, 0.3333333333333333703, 0.3333333333333333703, 0.3333333333333333703, 0.3333333333333333703, 0.3333333333333333703, 0.3333333333333333703, 0.3333333333333333703, 0.3333333333333333703, 0.3333333333333333703, 0.3333333333333333703, 0.3333333333333333703, 0.3333333333333333703, 0.3333333333333333703, 0.3333333333333333703, 0.3333333333333333703, 0.3333333333333333703, 0.3333333333333333703, 0.3333333333333333703, 0.3333333333333333703, 0.3333333333333333703, 0.3333333333333333703, 0.3333333333333333703, 0.3333333333333333703, 0.3333333333333333703, 0.3333333333333333703, 0.3333333333333333703, 0.3333333333333333703, 0.3333333333333333703, 0.3333333333333333703, 0.3333333333333333703, 0.3333333333333333703, 0.3333333333333333703, 0.3333333333333333703, 0.3333333333333333703, 0.3333333333333333703, 0.3333333333333333703, 0.3333333333333333703, 0.3333333333333333703, 0.3333333333333333703, 0.3333333333333333703, 0.3333333333333333703, 0.3333333333333333703, 0.3333333333333333703, 0.3333333333333333703, 0.3333333333333333703, 0.3333333333333333703, 0.3333333333333333703, 0.3333333333333333703, 0.3333333333333333703, 0.3333333333333333703, 0.3333333333333333703, 0.3333333333333333703, 0.3333333333333333703, 0.3333333333333333703, 0.3333333333333333703, 0.3333333333333333703, 0.3333333333333333703, 0.3333333333333333703, 0.3333333333333333703, 0.3333333333333333703, 0.3333333333333333703, 0.3333333333333333703, 0.3333333333333333703, 0.3333333333333333703, 0.3333333333333333703, 0.3333333333333333703, 0.3333333333333333703, 0.3333333333333333703, 0.3333333333333333703, 0.3333333333333333703, 0.3333333333333333703, 0.3333333333333333703, 0.3333333333333333703, 0.3333333333333333703, 0.3333333333333333703, 0.3333333333333333703, 0.3333333333333333703, 0.3333333333333333703, 0.3333333333333333703, 0.3333333333333333703, 0.3333333333333333703, 0.3333333333333333703, 0.3333333333333333703, 0.3333333333333333703, 0.3333333333333333703, 0.3333333333333333703, 0.3333333333333333703, 0.3333333333333333703, 0.3333333333333333703, 0.3333333333333333703, 0.3333333333333333703, 0.3333333333333333703),
 ( 1.000000000000000000, 1.000000000000000000, 1.000000000000000000, 1.000000000000000000, 1.000000000000000000, 1.000000000000000000, 1.000000000000000000, 1.000000000000000000, 1.000000000000000000, 1.000000000000000000, 1.000000000000000000, 1.000000000000000000, 1.000000000000000000, 1.000000000000000000, 1.000000000000000000, 1.000000000000000000, 1.000000000000000000, 1.000000000000000000, 1.000000000000000000, 1.000000000000000000, 1.000000000000000000, 1.000000000000000000, 1.000000000000000000, 1.000000000000000000, 1.000000000000000000, 1.000000000000000000, 1.000000000000000000, 1.000000000000000000, 1.000000000000000000, 1.000000000000000000, 1.000000000000000000, 1.000000000000000000, 1.000000000000000000, 1.000000000000000000, 1.000000000000000000, 1.000000000000000000, 1.000000000000000000, 1.000000000000000000, 1.000000000000000000, 1.000000000000000000, 1.000000000000000000, 1.000000000000000000, 1.000000000000000000, 1.000000000000000000, 1.000000000000000000, 1.000000000000000000, 1.000000000000000000, 1.000000000000000000, 1.000000000000000000, 1.000000000000000000, 1.000000000000000000, 1.000000000000000000, 1.000000000000000000, 1.000000000000000000, 1.000000000000000000, 1.000000000000000000, 1.000000000000000000, 1.000000000000000000, 1.000000000000000000, 1.000000000000000000, 1.000000000000000000, 1.000000000000000000, 1.000000000000000000, 1.000000000000000000, 1.000000000000000000, 1.000000000000000000, 1.000000000000000000, 1.000000000000000000, 1.000000000000000000, 1.000000000000000000, 1.000000000000000000, 1.000000000000000000, 1.000000000000000000, 1.000000000000000000, 1.000000000000000000, 1.000000000000000000, 1.000000000000000000, 1.000000000000000000, 1.000000000000000000, 1.000000000000000000, 1.000000000000000000, 1.000000000000000000, 1.000000000000000000, 1.000000000000000000, 1.000000000000000000, 1.000000000000000000, 1.000000000000000000, 1.000000000000000000, 1.000000000000000000, 1.000000000000000000, 1.000000000000000000, 1.000000000000000000, 1.000000000000000000, 1.000000000000000000, 1.000000000000000000, 1.000000000000000000, 1.000000000000000000, 1.000000000000000000, 1.000000000000000000, 1.000000000000000000, 1.000000000000000000, 1.000000000000000000, 1.000000000000000000, 1.000000000000000000, 1.000000000000000000, 1.000000000000000000, 1.000000000000000000, 1.000000000000000000, 1.000000000000000000, 1.000000000000000000, 1.000000000000000000, 1.000000000000000000, 1.000000000000000000, 1.000000000000000000, 1.000000000000000000, 1.000000000000000000, 1.000000000000000000, 1.000000000000000000, 1.000000000000000000, 1.000000000000000000, 1.000000000000000000, 1.000000000000000000, 1.000000000000000000, 1.000000000000000000, 1.000000000000000000, 1.000000000000000000, 1.000000000000000000, 1.000000000000000000, 1.000000000000000000, 1.000000000000000000, 1.000000000000000000, 1.000000000000000000, 1.000000000000000000, 1.000000000000000000, 1.000000000000000000, 1.000000000000000000, 1.000000000000000000, 1.000000000000000000, 1.000000000000000000, 1.000000000000000000, 1.000000000000000000, 1.000000000000000000, 1.000000000000000000, 1.000000000000000000, 1.000000000000000000, 1.000000000000000000, 1.000000000000000000, 1.000000000000000000, 1.000000000000000000, 1.000000000000000000, 1.000000000000000000, 1.000000000000000000, 1.000000000000000000, 1.000000000000000000, 1.000000000000000000, 1.000000000000000000, 1.000000000000000000, 1.000000000000000000, 1.000000000000000000, 1.000000000000000000, 1.000000000000000000, 1.000000000000000000, 1.000000000000000000, 1.000000000000000000, 1.000000000000000000, 1.000000000000000000, 1.000000000000000000, 1.000000000000000000, 1.000000000000000000, 1.000000000000000000, 1.000000000000000000, 1.000000000000000000, 1.000000000000000000, 1.000000000000000000, 1.000000000000000000, 1.000000000000000000, 1.000000000000000000, 1.000000000000000000, 1.000000000000000000, 1.000000000000000000, 1.000000000000000000, 1.000000000000000000, 1.000000000000000000, 1.000000000000000000, 1.000000000000000000, 1.000000000000000000, 1.000000000000000000, 1.000000000000000000, 1.000000000000000000, 1.000000000000000000, 1.000000000000000000, 1.000000000000000000, 1.000000000000000000, 1.000000000000000000, 1.000000000000000000, 1.000000000000000000, 1.000000000000000000, 1.000000000000000000, 1.000000000000000000, 1.000000000000000000, 1.000000000000000000, 1.000000000000000000, 1.000000000000000000, 1.000000000000000000, 1.000000000000000000, 1.000000000000000000, 1.000000000000000000, 1.000000000000000000, 1.000000000000000000, 1.000000000000000000, 1.000000000000000000, 1.000000000000000000, 1.000000000000000000, 1.000000000000000000, 1.000000000000000000, 1.000000000000000000, 1.000000000000000000, 1.000000000000000000, 1.000000000000000000, 1.000000000000000000, 1.000000000000000000, 1.000000000000000000, 1.000000000000000000, 1.000000000000000000, 1.000000000000000000, 1.000000000000000000, 1.000000000000000000, 1.000000000000000000, 1.000000000000000000, 1.000000000000000000, 1.000000000000000000, 1.000000000000000000, 1.000000000000000000, 1.000000000000000000, 1.000000000000000000, 1.000000000000000000, 1.000000000000000000, 1.000000000000000000, 1.000000000000000000, 1.000000000000000000, 1.000000000000000000, 1.000000000000000000, 1.000000000000000000, 1.000000000000000000, 1.000000000000000000, 1.000000000000000000, 1.000000000000000000, 1.000000000000000000, 1.000000000000000000, 1.000000000000000000, 1.000000000000000000, 1.000000000000000000, 1.000000000000000000, 1.000000000000000000, 1.000000000000000000, 1.000000000000000000, 1.000000000000000000, 1.000000000000000000, 1.000000000000000000, 1.000000000000000000, 1.000000000000000000, 1.000000000000000000, 1.000000000000000000, 1.000000000000000000, 1.000000000000000000, 1.000000000000000000, 1.000000000000000000, 1.000000000000000000, 1.000000000000000000, 1.000000000000000000, 1.000000000000000000, 1.000000000000000000, 1.000000000000000000, 1.000000000000000000, 1.000000000000000000, 1.000000000000000000, 1.000000000000000000, 1.000000000000000000, 1.000000000000000000, 1.000000000000000000, 1.000000000000000000, 1.000000000000000000, 1.000000000000000000, 1.000000000000000000, 1.000000000000000000, 1.000000000000000000, 1.000000000000000000, 1.000000000000000000, 1.000000000000000000, 1.000000000000000000, 1.000000000000000000, 1.000000000000000000, 1.000000000000000000, 1.000000000000000000, 1.000000000000000000, 1.000000000000000000, 1.000000000000000000, 1.000000000000000000, 1.000000000000000000, 1.000000000000000000, 1.000000000000000000, 1.000000000000000000, 1.000000000000000000, 1.000000000000000000, 1.000000000000000000, 1.000000000000000000, 1.000000000000000000, 1.000000000000000000, 1.000000000000000000, 1.000000000000000000, 1.000000000000000000, 1.000000000000000000, 1.000000000000000000, 1.000000000000000000, 1.000000000000000000, 1.000000000000000000, 1.000000000000000000, 1.000000000000000000, 1.000000000000000000, 1.000000000000000000, 1.000000000000000000, 1.000000000000000000, 1.000000000000000000, 1.000000000000000000, 1.000000000000000000, 1.000000000000000000, 1.000000000000000000, 1.000000000000000000, 1.000000000000000000, 1.000000000000000000, 1.000000000000000000, 1.000000000000000000, 1.000000000000000000, 1.000000000000000000, 1.000000000000000000, 1.000000000000000000),
 ( 0.3333333333333333703, 0.3333333333333333703, 0.3333333333333333703, 0.3333333333333333703, 0.3333333333333333703, 0.3333333333333333703, 0.3333333333333333703, 0.3333333333333333703, 0.3333333333333333703, 0.3333333333333333703, 0.3333333333333333703, 0.3333333333333333703, 0.3333333333333333703, 0.3333333333333333703, 0.3333333333333333703, 0.3333333333333333703, 0.3333333333333333703, 0.3333333333333333703, 0.3333333333333333703, 0.3333333333333333703, 0.3333333333333333703, 0.3333333333333333703, 0.3333333333333333703, 0.3333333333333333703, 0.3333333333333333703, 0.3333333333333333703, 0.3333333333333333703, 0.3333333333333333703, 0.3333333333333333703, 0.3333333333333333703, 0.3333333333333333703, 0.3333333333333333703, 0.3333333333333333703, 0.3333333333333333703, 0.3333333333333333703, 0.3333333333333333703, 0.3333333333333333703, 0.3333333333333333703, 0.3333333333333333703, 0.3333333333333333703, 0.3333333333333333703, 0.3333333333333333703, 0.3333333333333333703, 0.3333333333333333703, 0.3333333333333333703, 0.3333333333333333703, 0.3333333333333333703, 0.3333333333333333703, 0.3333333333333333703, 0.3333333333333333703, 0.3333333333333333703, 0.3333333333333333703, 0.3333333333333333703, 0.3333333333333333703, 0.3333333333333333703, 0.3333333333333333703, 0.3333333333333333703, 0.3333333333333333703, 0.3333333333333333703, 0.3333333333333333703, 0.3333333333333333703, 0.3333333333333333703, 0.3333333333333333703, 0.3333333333333333703, 0.3333333333333333703, 0.3333333333333333703, 0.3333333333333333703, 0.3333333333333333703, 0.3333333333333333703, 0.3333333333333333703, 0.3333333333333333703, 0.3333333333333333703, 0.3333333333333333703, 0.3333333333333333703, 0.3333333333333333703, 0.3333333333333333703, 0.3333333333333333703, 0.3333333333333333703, 0.3333333333333333703, 0.3333333333333333703, 0.3333333333333333703, 0.3333333333333333703, 0.3333333333333333703, 0.3333333333333333703, 0.3333333333333333703, 0.3333333333333333703, 0.3333333333333333703, 0.3333333333333333703, 0.3333333333333333703, 0.3333333333333333703, 0.3333333333333333703, 0.3333333333333333703, 0.3333333333333333703, 0.3333333333333333703, 0.3333333333333333703, 0.3333333333333333703, 0.3333333333333333703, 0.3333333333333333703, 0.3333333333333333703, 0.3333333333333333703, 0.3333333333333333703, 0.3333333333333333703, 0.3333333333333333703, 0.3333333333333333703, 0.3333333333333333703, 0.3333333333333333703, 0.3333333333333333703, 0.3333333333333333703, 0.3333333333333333703, 0.3333333333333333703, 0.3333333333333333703, 0.3333333333333333703, 0.3333333333333333703, 0.3333333333333333703, 0.3333333333333333703, 0.3333333333333333703, 0.3333333333333333703, 0.3333333333333333703, 0.3333333333333333703, 0.3333333333333333703, 0.3333333333333333703, 0.3333333333333333703, 0.3333333333333333703, 0.3333333333333333703, 0.3333333333333333703, 0.3333333333333333703, 0.3333333333333333703, 0.3333333333333333703, 0.3333333333333333703, 0.3333333333333333703, 0.3333333333333333703, 0.3333333333333333703, 0.3333333333333333703, 0.3333333333333333703, 0.3333333333333333703, 0.3333333333333333703, 0.3333333333333333703, 0.3333333333333333703, 0.3333333333333333703, 0.3333333333333333703, 0.3333333333333333703, 0.3333333333333333703, 0.3333333333333333703, 0.3333333333333333703, 0.3333333333333333703, 0.3333333333333333703, 0.3333333333333333703, 0.3333333333333333703, 0.3333333333333333703, 0.3333333333333333703, 0.3333333333333333703, 0.3333333333333333703, 0.3333333333333333703, 0.3333333333333333703, 0.3333333333333333703, 0.3333333333333333703, 0.3333333333333333703, 0.3333333333333333703, 0.3333333333333333703, 0.3333333333333333703, 0.3333333333333333703, 0.3333333333333333703, 0.3333333333333333703, 0.3333333333333333703, 0.3333333333333333703, 0.3333333333333333703, 0.3333333333333333703, 0.3333333333333333703, 0.3333333333333333703, 0.3333333333333333703, 0.3333333333333333703, 0.3333333333333333703, 0.3333333333333333703, 0.3333333333333333703, 0.3333333333333333703, 0.3333333333333333703, 0.3333333333333333703, 0.3333333333333333703, 0.3333333333333333703, 0.3333333333333333703, 0.3333333333333333703, 0.3333333333333333703, 0.3333333333333333703, 0.3333333333333333703, 0.3333333333333333703, 0.3333333333333333703, 0.3333333333333333703, 0.3333333333333333703, 0.3333333333333333703, 0.3333333333333333703, 0.3333333333333333703, 0.3333333333333333703, 0.3333333333333333703, 0.3333333333333333703, 0.3333333333333333703, 0.3333333333333333703, 0.3333333333333333703, 0.3333333333333333703, 0.3333333333333333703, 0.3333333333333333703, 0.3333333333333333703, 0.3333333333333333703, 0.3333333333333333703, 0.3333333333333333703, 0.3333333333333333703, 0.3333333333333333703, 0.3333333333333333703, 0.3333333333333333703, 0.3333333333333333703, 0.3333333333333333703, 0.3333333333333333703, 0.3333333333333333703, 0.3333333333333333703, 0.3333333333333333703, 0.3333333333333333703, 0.3333333333333333703, 0.3333333333333333703, 0.3333333333333333703, 0.3333333333333333703, 0.3333333333333333703, 0.3333333333333333703, 0.3333333333333333703, 0.3333333333333333703, 0.3333333333333333703, 0.3333333333333333703, 0.3333333333333333703, 0.3333333333333333703, 0.3333333333333333703, 0.3333333333333333703, 0.3333333333333333703, 0.3333333333333333703, 0.3333333333333333703, 0.3333333333333333703, 0.3333333333333333703, 0.3333333333333333703, 0.3333333333333333703, 0.3333333333333333703, 0.3333333333333333703, 0.3333333333333333703, 0.3333333333333333703, 0.3333333333333333703, 0.3333333333333333703, 0.3333333333333333703, 0.3333333333333333703, 0.3333333333333333703, 0.3333333333333333703, 0.3333333333333333703, 0.3333333333333333703, 0.3333333333333333703, 0.3333333333333333703, 0.3333333333333333703, 0.3333333333333333703, 0.3333333333333333703, 0.3333333333333333703, 0.3333333333333333703, 0.3333333333333333703, 0.3333333333333333703, 0.3333333333333333703, 0.3333333333333333703, 0.3333333333333333703, 0.3333333333333333703, 0.3333333333333333703, 0.3333333333333333703, 0.3333333333333333703, 0.3333333333333333703, 0.3333333333333333703, 0.3333333333333333703, 0.3333333333333333703, 0.3333333333333333703, 0.3333333333333333703, 0.3333333333333333703, 0.3333333333333333703, 0.3333333333333333703, 0.3333333333333333703, 0.3333333333333333703, 0.3333333333333333703, 0.3333333333333333703, 0.3333333333333333703, 0.3333333333333333703, 0.3333333333333333703, 0.3333333333333333703, 0.3333333333333333703, 0.3333333333333333703, 0.3333333333333333703, 0.3333333333333333703, 0.3333333333333333703, 0.3333333333333333703, 0.3333333333333333703, 0.3333333333333333703, 0.3333333333333333703, 0.3333333333333333703, 0.3333333333333333703, 0.3333333333333333703, 0.3333333333333333703, 0.3333333333333333703, 0.3333333333333333703, 0.3333333333333333703, 0.3333333333333333703, 0.3333333333333333703, 0.3333333333333333703, 0.3333333333333333703, 0.3333333333333333703, 0.3333333333333333703, 0.3333333333333333703, 0.3333333333333333703, 0.3333333333333333703, 0.3333333333333333703, 0.3333333333333333703, 0.3333333333333333703, 0.3333333333333333703, 0.3333333333333333703, 0.3333333333333333703, 0.3333333333333333703, 0.3333333333333333703, 0.3333333333333333703, 0.3333333333333333703, 0.3333333333333333703, 0.3333333333333333703, 0.3333333333333333703, 0.3333333333333333703, 0.3333333333333333703, 0.3333333333333333703, 0.3333333333333333703, 0.3333333333333333703, 0.3333333333333333703, 0.3333333333333333703, 0.3333333333333333703, 0.3333333333333333703, 0.3333333333333333703, 0.3333333333333333703, 0.3333333333333333703, 0.3333333333333333703, 0.3333333333333333703, 0.3333333333333333703, 0.3333333333333333703, 0.3333333333333333703),
 ( 0.3333333333333333703, 0.3333333333333333703, 0.3333333333333333703, 0.3333333333333333703, 0.3333333333333333703, 0.3333333333333333703, 0.3333333333333333703, 0.3333333333333333703, 0.3333333333333333703, 0.3333333333333333703, 0.3333333333333333703, 0.3333333333333333703, 0.3333333333333333703, 0.3333333333333333703, 0.3333333333333333703, 0.3333333333333333703, 0.3333333333333333703, 0.3333333333333333703, 0.3333333333333333703, 0.3333333333333333703, 0.3333333333333333703, 0.3333333333333333703, 0.3333333333333333703, 0.3333333333333333703, 0.3333333333333333703, 0.3333333333333333703, 0.3333333333333333703, 0.3333333333333333703, 0.3333333333333333703, 0.3333333333333333703, 0.3333333333333333703, 0.3333333333333333703, 0.3333333333333333703, 0.3333333333333333703, 0.3333333333333333703, 0.3333333333333333703, 0.3333333333333333703, 0.3333333333333333703, 0.3333333333333333703, 0.3333333333333333703, 0.3333333333333333703, 0.3333333333333333703, 0.3333333333333333703, 0.3333333333333333703, 0.3333333333333333703, 0.3333333333333333703, 0.3333333333333333703, 0.3333333333333333703, 0.3333333333333333703, 0.3333333333333333703, 0.3333333333333333703, 0.3333333333333333703, 0.3333333333333333703, 0.3333333333333333703, 0.3333333333333333703, 0.3333333333333333703, 0.3333333333333333703, 0.3333333333333333703, 0.3333333333333333703, 0.3333333333333333703, 0.3333333333333333703, 0.3333333333333333703, 0.3333333333333333703, 0.3333333333333333703, 0.3333333333333333703, 0.3333333333333333703, 0.3333333333333333703, 0.3333333333333333703, 0.3333333333333333703, 0.3333333333333333703, 0.3333333333333333703, 0.3333333333333333703, 0.3333333333333333703, 0.3333333333333333703, 0.3333333333333333703, 0.3333333333333333703, 0.3333333333333333703, 0.3333333333333333703, 0.3333333333333333703, 0.3333333333333333703, 0.3333333333333333703, 0.3333333333333333703, 0.3333333333333333703, 0.3333333333333333703, 0.3333333333333333703, 0.3333333333333333703, 0.3333333333333333703, 0.3333333333333333703, 0.3333333333333333703, 0.3333333333333333703, 0.3333333333333333703, 0.3333333333333333703, 0.3333333333333333703, 0.3333333333333333703, 0.3333333333333333703, 0.3333333333333333703, 0.3333333333333333703, 0.3333333333333333703, 0.3333333333333333703, 0.3333333333333333703, 0.3333333333333333703, 0.3333333333333333703, 0.3333333333333333703, 0.3333333333333333703, 0.3333333333333333703, 0.3333333333333333703, 0.3333333333333333703, 0.3333333333333333703, 0.3333333333333333703, 0.3333333333333333703, 0.3333333333333333703, 0.3333333333333333703, 0.3333333333333333703, 0.3333333333333333703, 0.3333333333333333703, 0.3333333333333333703, 0.3333333333333333703, 0.3333333333333333703, 0.3333333333333333703, 0.3333333333333333703, 0.3333333333333333703, 0.3333333333333333703, 0.3333333333333333703, 0.3333333333333333703, 0.3333333333333333703, 0.3333333333333333703, 0.3333333333333333703, 0.3333333333333333703, 0.3333333333333333703, 0.3333333333333333703, 0.3333333333333333703, 0.3333333333333333703, 0.3333333333333333703, 0.3333333333333333703, 0.3333333333333333703, 0.3333333333333333703, 0.3333333333333333703, 0.3333333333333333703, 0.3333333333333333703, 0.3333333333333333703, 0.3333333333333333703, 0.3333333333333333703, 0.3333333333333333703, 0.3333333333333333703, 0.3333333333333333703, 0.3333333333333333703, 0.3333333333333333703, 0.3333333333333333703, 0.3333333333333333703, 0.3333333333333333703, 0.3333333333333333703, 0.3333333333333333703, 0.3333333333333333703, 0.3333333333333333703, 0.3333333333333333703, 0.3333333333333333703, 0.3333333333333333703, 0.3333333333333333703, 0.3333333333333333703, 0.3333333333333333703, 0.3333333333333333703, 0.3333333333333333703, 0.3333333333333333703, 0.3333333333333333703, 0.3333333333333333703, 0.3333333333333333703, 0.3333333333333333703, 0.3333333333333333703, 0.3333333333333333703, 0.3333333333333333703, 0.3333333333333333703, 0.3333333333333333703, 0.3333333333333333703, 0.3333333333333333703, 0.3333333333333333703, 0.3333333333333333703, 0.3333333333333333703, 0.3333333333333333703, 0.3333333333333333703, 0.3333333333333333703, 0.3333333333333333703, 0.3333333333333333703, 0.3333333333333333703, 0.3333333333333333703, 0.3333333333333333703, 0.3333333333333333703, 0.3333333333333333703, 0.3333333333333333703, 0.3333333333333333703, 0.3333333333333333703, 0.3333333333333333703, 0.3333333333333333703, 0.3333333333333333703, 0.3333333333333333703, 0.3333333333333333703, 0.3333333333333333703, 0.3333333333333333703, 0.3333333333333333703, 0.3333333333333333703, 0.3333333333333333703, 0.3333333333333333703, 0.3333333333333333703, 0.3333333333333333703, 0.3333333333333333703, 0.3333333333333333703, 0.3333333333333333703, 0.3333333333333333703, 0.3333333333333333703, 0.3333333333333333703, 0.3333333333333333703, 0.3333333333333333703, 0.3333333333333333703, 0.3333333333333333703, 0.3333333333333333703, 0.3333333333333333703, 0.3333333333333333703, 0.3333333333333333703, 0.3333333333333333703, 0.3333333333333333703, 0.3333333333333333703, 0.3333333333333333703, 0.3333333333333333703, 0.3333333333333333703, 0.3333333333333333703, 0.3333333333333333703, 0.3333333333333333703, 0.3333333333333333703, 0.3333333333333333703, 0.3333333333333333703, 0.3333333333333333703, 0.3333333333333333703, 0.3333333333333333703, 0.3333333333333333703, 0.3333333333333333703, 0.3333333333333333703, 0.3333333333333333703, 0.3333333333333333703, 0.3333333333333333703, 0.3333333333333333703, 0.3333333333333333703, 0.3333333333333333703, 0.3333333333333333703, 0.3333333333333333703, 0.3333333333333333703, 0.3333333333333333703, 0.3333333333333333703, 0.3333333333333333703, 0.3333333333333333703, 0.3333333333333333703, 0.3333333333333333703, 0.3333333333333333703, 0.3333333333333333703, 0.3333333333333333703, 0.3333333333333333703, 0.3333333333333333703, 0.3333333333333333703, 0.3333333333333333703, 0.3333333333333333703, 0.3333333333333333703, 0.3333333333333333703, 0.3333333333333333703, 0.3333333333333333703, 0.3333333333333333703, 0.3333333333333333703, 0.3333333333333333703, 0.3333333333333333703, 0.3333333333333333703, 0.3333333333333333703, 0.3333333333333333703, 0.3333333333333333703, 0.3333333333333333703, 0.3333333333333333703, 0.3333333333333333703, 0.3333333333333333703, 0.3333333333333333703, 0.3333333333333333703, 0.3333333333333333703, 0.3333333333333333703, 0.3333333333333333703, 0.3333333333333333703, 0.3333333333333333703, 0.3333333333333333703, 0.3333333333333333703, 0.3333333333333333703, 0.3333333333333333703, 0.3333333333333333703, 0.3333333333333333703, 0.3333333333333333703, 0.3333333333333333703, 0.3333333333333333703, 0.3333333333333333703, 0.3333333333333333703, 0.3333333333333333703, 0.3333333333333333703, 0.3333333333333333703, 0.3333333333333333703, 0.3333333333333333703, 0.3333333333333333703, 0.3333333333333333703, 0.3333333333333333703, 0.3333333333333333703, 0.3333333333333333703, 0.3333333333333333703, 0.3333333333333333703, 0.3333333333333333703, 0.3333333333333333703, 0.3333333333333333703, 0.3333333333333333703, 0.3333333333333333703, 0.3333333333333333703, 0.3333333333333333703, 0.3333333333333333703, 0.3333333333333333703, 0.3333333333333333703, 0.3333333333333333703, 0.3333333333333333703, 0.3333333333333333703, 0.3333333333333333703, 0.3333333333333333703, 0.3333333333333333703, 0.3333333333333333703, 0.3333333333333333703, 0.3333333333333333703, 0.3333333333333333703, 0.3333333333333333703, 0.3333333333333333703, 0.3333333333333333703, 0.3333333333333333703, 0.3333333333333333703, 0.3333333333333333703, 0.3333333333333333703, 0.3333333333333333703, 0.3333333333333333703, 0.3333333333333333703, 0.3333333333333333703, 0.3333333333333333703),
 ( 1.000000000000000000, 1.000000000000000000, 1.000000000000000000, 1.000000000000000000, 1.000000000000000000, 1.000000000000000000, 1.000000000000000000, 1.000000000000000000, 1.000000000000000000, 1.000000000000000000, 1.000000000000000000, 1.000000000000000000, 1.000000000000000000, 1.000000000000000000, 1.000000000000000000, 1.000000000000000000, 1.000000000000000000, 1.000000000000000000, 1.000000000000000000, 1.000000000000000000, 1.000000000000000000, 1.000000000000000000, 1.000000000000000000, 1.000000000000000000, 1.000000000000000000, 1.000000000000000000, 1.000000000000000000, 1.000000000000000000, 1.000000000000000000, 1.000000000000000000, 1.000000000000000000, 1.000000000000000000, 1.000000000000000000, 1.000000000000000000, 1.000000000000000000, 1.000000000000000000, 1.000000000000000000, 1.000000000000000000, 1.000000000000000000, 1.000000000000000000, 1.000000000000000000, 1.000000000000000000, 1.000000000000000000, 1.000000000000000000, 1.000000000000000000, 1.000000000000000000, 1.000000000000000000, 1.000000000000000000, 1.000000000000000000, 1.000000000000000000, 1.000000000000000000, 1.000000000000000000, 1.000000000000000000, 1.000000000000000000, 1.000000000000000000, 1.000000000000000000, 1.000000000000000000, 1.000000000000000000, 1.000000000000000000, 1.000000000000000000, 1.000000000000000000, 1.000000000000000000, 1.000000000000000000, 1.000000000000000000, 1.000000000000000000, 1.000000000000000000, 1.000000000000000000, 1.000000000000000000, 1.000000000000000000, 1.000000000000000000, 1.000000000000000000, 1.000000000000000000, 1.000000000000000000, 1.000000000000000000, 1.000000000000000000, 1.000000000000000000, 1.000000000000000000, 1.000000000000000000, 1.000000000000000000, 1.000000000000000000, 1.000000000000000000, 1.000000000000000000, 1.000000000000000000, 1.000000000000000000, 1.000000000000000000, 1.000000000000000000, 1.000000000000000000, 1.000000000000000000, 1.000000000000000000, 1.000000000000000000, 1.000000000000000000, 1.000000000000000000, 1.000000000000000000, 1.000000000000000000, 1.000000000000000000, 1.000000000000000000, 1.000000000000000000, 1.000000000000000000, 1.000000000000000000, 1.000000000000000000, 1.000000000000000000, 1.000000000000000000, 1.000000000000000000, 1.000000000000000000, 1.000000000000000000, 1.000000000000000000, 1.000000000000000000, 1.000000000000000000, 1.000000000000000000, 1.000000000000000000, 1.000000000000000000, 1.000000000000000000, 1.000000000000000000, 1.000000000000000000, 1.000000000000000000, 1.000000000000000000, 1.000000000000000000, 1.000000000000000000, 1.000000000000000000, 1.000000000000000000, 1.000000000000000000, 1.000000000000000000, 1.000000000000000000, 1.000000000000000000, 1.000000000000000000, 1.000000000000000000, 1.000000000000000000, 1.000000000000000000, 1.000000000000000000, 1.000000000000000000, 1.000000000000000000, 1.000000000000000000, 1.000000000000000000, 1.000000000000000000, 1.000000000000000000, 1.000000000000000000, 1.000000000000000000, 1.000000000000000000, 1.000000000000000000, 1.000000000000000000, 1.000000000000000000, 1.000000000000000000, 1.000000000000000000, 1.000000000000000000, 1.000000000000000000, 1.000000000000000000, 1.000000000000000000, 1.000000000000000000, 1.000000000000000000, 1.000000000000000000, 1.000000000000000000, 1.000000000000000000, 1.000000000000000000, 1.000000000000000000, 1.000000000000000000, 1.000000000000000000, 1.000000000000000000, 1.000000000000000000, 1.000000000000000000, 1.000000000000000000, 1.000000000000000000, 1.000000000000000000, 1.000000000000000000, 1.000000000000000000, 1.000000000000000000, 1.000000000000000000, 1.000000000000000000, 1.000000000000000000, 1.000000000000000000, 1.000000000000000000, 1.000000000000000000, 1.000000000000000000, 1.000000000000000000, 1.000000000000000000, 1.000000000000000000, 1.000000000000000000, 1.000000000000000000, 1.000000000000000000, 1.000000000000000000, 1.000000000000000000, 1.000000000000000000, 1.000000000000000000, 1.000000000000000000, 1.000000000000000000, 1.000000000000000000, 1.000000000000000000, 1.000000000000000000, 1.000000000000000000, 1.000000000000000000, 1.000000000000000000, 1.000000000000000000, 1.000000000000000000, 1.000000000000000000, 1.000000000000000000, 1.000000000000000000, 1.000000000000000000, 1.000000000000000000, 1.000000000000000000, 1.000000000000000000, 1.000000000000000000, 1.000000000000000000, 1.000000000000000000, 1.000000000000000000, 1.000000000000000000, 1.000000000000000000, 1.000000000000000000, 1.000000000000000000, 1.000000000000000000, 1.000000000000000000, 1.000000000000000000, 1.000000000000000000, 1.000000000000000000, 1.000000000000000000, 1.000000000000000000, 1.000000000000000000, 1.000000000000000000, 1.000000000000000000, 1.000000000000000000, 1.000000000000000000, 1.000000000000000000, 1.000000000000000000, 1.000000000000000000, 1.000000000000000000, 1.000000000000000000, 1.000000000000000000, 1.000000000000000000, 1.000000000000000000, 1.000000000000000000, 1.000000000000000000, 1.000000000000000000, 1.000000000000000000, 1.000000000000000000, 1.000000000000000000, 1.000000000000000000, 1.000000000000000000, 1.000000000000000000, 1.000000000000000000, 1.000000000000000000, 1.000000000000000000, 1.000000000000000000, 1.000000000000000000, 1.000000000000000000, 1.000000000000000000, 1.000000000000000000, 1.000000000000000000, 1.000000000000000000, 1.000000000000000000, 1.000000000000000000, 1.000000000000000000, 1.000000000000000000, 1.000000000000000000, 1.000000000000000000, 1.000000000000000000, 1.000000000000000000, 1.000000000000000000, 1.000000000000000000, 1.000000000000000000, 1.000000000000000000, 1.000000000000000000, 1.000000000000000000, 1.000000000000000000, 1.000000000000000000, 1.000000000000000000, 1.000000000000000000, 1.000000000000000000, 1.000000000000000000, 1.000000000000000000, 1.000000000000000000, 1.000000000000000000, 1.000000000000000000, 1.000000000000000000, 1.000000000000000000, 1.000000000000000000, 1.000000000000000000, 1.000000000000000000, 1.000000000000000000, 1.000000000000000000, 1.000000000000000000, 1.000000000000000000, 1.000000000000000000, 1.000000000000000000, 1.000000000000000000, 1.000000000000000000, 1.000000000000000000, 1.000000000000000000, 1.000000000000000000, 1.000000000000000000, 1.000000000000000000, 1.000000000000000000, 1.000000000000000000, 1.000000000000000000, 1.000000000000000000, 1.000000000000000000, 1.000000000000000000, 1.000000000000000000, 1.000000000000000000, 1.000000000000000000, 1.000000000000000000, 1.000000000000000000, 1.000000000000000000, 1.000000000000000000, 1.000000000000000000, 1.000000000000000000, 1.000000000000000000, 1.000000000000000000, 1.000000000000000000, 1.000000000000000000, 1.000000000000000000, 1.000000000000000000, 1.000000000000000000, 1.000000000000000000, 1.000000000000000000, 1.000000000000000000, 1.000000000000000000, 1.000000000000000000, 1.000000000000000000, 1.000000000000000000, 1.000000000000000000, 1.000000000000000000, 1.000000000000000000, 1.000000000000000000, 1.000000000000000000, 1.000000000000000000, 1.000000000000000000, 1.000000000000000000, 1.000000000000000000, 1.000000000000000000, 1.000000000000000000, 1.000000000000000000, 1.000000000000000000, 1.000000000000000000, 1.000000000000000000, 1.000000000000000000, 1.000000000000000000, 1.000000000000000000, 1.000000000000000000) ) ) 
 REPRESENTATION_ITEM ( '' )  SURFACE ( )  );
#3701=CARTESIAN_POINT ( 'NONE',  ( -27.92885697401080591, 6.962042978589167319, -220.9552227796709190 ) ) ;
#3702=CARTESIAN_POINT ( 'NONE',  ( 6.566035546683759883, 15.06745272174450712, -218.8330720708048034 ) ) ;
#3703=CARTESIAN_POINT ( 'NONE',  ( -2.129100187576105530, 26.11057959790866789, -231.5939360033278547 ) ) ;
#3705=CARTESIAN_POINT ( 'NONE',  ( 23.82514222742702614, -14.35463969081363267, -233.5616060903067535 ) ) ;
#3707=CARTESIAN_POINT ( 'NONE',  ( 13.43730899468209294, 8.427513769504761498, -221.4030804848920297 ) ) ;
#3708=CARTESIAN_POINT ( 'NONE',  ( -8.005900519654911562, 11.01772743098285545, -228.7074549843708269 ) ) ;
#3709=CARTESIAN_POINT ( 'NONE',  ( -20.95553895916151177, 12.88782924195037438, -232.2493899712447956 ) ) ;
#3710=CARTESIAN_POINT ( 'NONE',  ( -8.326748185965973548, -13.59788789161040512, -220.4531618457016862 ) ) ;
#3711=CARTESIAN_POINT ( 'NONE',  ( -20.54164754914381064, 7.122791156791981493, -233.5720402887671980 ) ) ;
#3716=CARTESIAN_POINT ( 'NONE',  ( -11.55316006017064012, 19.79513644261079719, -232.3088878043970453 ) ) ;
#3717=CARTESIAN_POINT ( 'NONE',  ( 15.65443801613259467, 7.488839228060037989, -233.6469817377710569 ) ) ;
#3718=CARTESIAN_POINT ( 'NONE',  ( -20.94800339253696109, 4.477632454355491731, -216.5423208360950298 ) ) ;
#3720=CARTESIAN_POINT ( 'NONE',  ( -16.01199461824852932, -9.140529685459805265, -215.3147469429904106 ) ) ;
#3721=CARTESIAN_POINT ( 'NONE',  ( -20.63475909113443763, -3.483688486440585486, -233.7225001494461480 ) ) ;
#3722=CARTESIAN_POINT ( 'NONE',  ( -7.694246740028670928, 10.31295298368923063, -221.9989544301487001 ) ) ;
#3723=CARTESIAN_POINT ( 'NONE',  ( -12.42894476027428929, -17.97759322220185396, -216.3110355466728834 ) ) ;
#3724=CARTESIAN_POINT ( 'NONE',  ( 15.12287735332712835, 21.03907941686458116, -231.7894952627153202 ) ) ;
#3725=CARTESIAN_POINT ( 'NONE',  ( 15.44393261315032184, -28.37553556939610999, -226.2064134899511600 ) ) ;
#3727=CARTESIAN_POINT ( 'NONE',  ( 21.27683256847563698, 4.223177115764435108, -215.2584548172064842 ) ) ;
#3729=CARTESIAN_POINT ( 'NONE',  ( 0.6289891638115701067, 16.47510600144228832, -227.0521699048171342 ) ) ;
#3730=CARTESIAN_POINT ( 'NONE',  ( -29.22672729369577738, 6.588740615114764054, -224.9915299386302934 ) ) ;
#3731=CARTESIAN_POINT ( 'NONE',  ( 24.03642272140365677, 3.646960756862087205, -218.2320643939070806 ) ) ;
#3732=CARTESIAN_POINT ( 'NONE',  ( 24.52160379727246209, 5.049198597839295033, -215.7868787176665535 ) ) ;
#3733=CARTESIAN_POINT ( 'NONE',  ( 1.040523496405688642, -16.53460264249922318, -217.0944950338946455 ) ) ;
#3734=CARTESIAN_POINT ( 'NONE',  ( 2.469769522101480597, 18.85781121334172639, -215.5372409425634430 ) ) ;
#3736=CARTESIAN_POINT ( 'NONE',  ( -3.350277215847999202, -25.10023987965119119, -233.9767109426786647 ) ) ;
#3737=CARTESIAN_POINT ( 'NONE',  ( -16.50467377682197423, 21.56569464670658220, -229.9175202103629374 ) ) ;
#3738=CARTESIAN_POINT ( 'NONE',  ( 23.18902850759750933, 20.27908137164207147, -226.2847847834817117 ) ) ;
#3739=CARTESIAN_POINT ( 'NONE',  ( -28.87859926594958537, -0.8320174534291842061, -222.6356913548140142 ) ) ;
#3740=CARTESIAN_POINT ( 'NONE',  ( -22.03660207690921879, 17.07234836129451949, -222.7335359861421296 ) ) ;
#3741=CARTESIAN_POINT ( 'NONE',  ( -0.2758005215353623862, 11.79991891162212525, -226.8645588387054488 ) ) ;
#3742=CARTESIAN_POINT ( 'NONE',  ( 15.70515172005171323, -0.7403987186381333352, -226.4590404369862995 ) ) ;
#3745=CARTESIAN_POINT ( 'NONE',  ( 16.26678737605450564, -16.61684638199339048, -230.8698708339908308 ) ) ;
#3747=CARTESIAN_POINT ( 'NONE',  ( 14.68951511424354273, -18.85605729411972575, -217.5026406474102885 ) ) ;
#3748=CARTESIAN_POINT ( 'NONE',  ( -8.752190949579933488, 24.25633523490762755, -230.6624101830059885 ) ) ;
#3751=CARTESIAN_POINT ( 'NONE',  ( 12.53674998645855787, 17.96979015029927851, -232.8843215672231679 ) ) ;
#3752=CARTESIAN_POINT ( 'NONE',  ( -23.51371042417668633, 2.081716773471995463, -216.9231029201042418 ) ) ;
#3753=CARTESIAN_POINT ( 'NONE',  ( -18.64257584594551531, -16.66392856591270899, -217.1407738418131999 ) ) ;
#3754=CARTESIAN_POINT ( 'NONE',  ( -1.542335193334551491, -19.71915426430242135, -216.1352730594569209 ) ) ;
#3755=CARTESIAN_POINT ( 'NONE',  ( -6.573387563318148885, 17.69612765735440973, -231.1211991061559274 ) ) ;
#3757=CARTESIAN_POINT ( 'NONE',  ( 18.90025403853754327, 17.70150481658638952, -229.5234643039372315 ) ) ;
#3758=CARTESIAN_POINT ( 'NONE',  ( -8.823862513872974489, 14.92351368520778898, -217.1499513473673346 ) ) ;
#3759=CARTESIAN_POINT ( 'NONE',  ( -5.706122936196527107, 15.14201253431006045, -228.6865785740211550 ) ) ;
#3761=CARTESIAN_POINT ( 'NONE',  ( 2.535512286608554433, 13.86868953312499109, -224.9313928733152181 ) ) ;
#3762=CARTESIAN_POINT ( 'NONE',  ( -17.64438593497130370, 2.824953307685432069, -229.4443205246391813 ) ) ;
#3763=CARTESIAN_POINT ( 'NONE',  ( 22.69522586737246783, 3.669837464059151344, -234.0947686933411944 ) ) ;
#3765=CARTESIAN_POINT ( 'NONE',  ( 8.211296573249146746, -12.45047565346596130, -222.1279395315445413 ) ) ;
#3767=CARTESIAN_POINT ( 'NONE',  ( -22.00000000000137490, -2.602085213965210642E-15, -216.9999999999999716 ) ) ;
#3768=CARTESIAN_POINT ( 'NONE',  ( -3.501680520304516264, 14.31538576447642264, -219.8967178229432307 ) ) ;
#3769=CARTESIAN_POINT ( 'NONE',  ( 15.75976565806011465, -3.644771625422815298, -224.1463364774561740 ) ) ;
#3770=CARTESIAN_POINT ( 'NONE',  ( 29.17814965709308694, -1.309718763918959139, -225.2029557489520926 ) ) ;
#3771=CARTESIAN_POINT ( 'NONE',  ( 13.69275646168278371, 8.674223198772375909, -220.8699857572541987 ) ) ;
#3773=CARTESIAN_POINT ( 'NONE',  ( -17.96792326766206926, -0.6237852504629022299, -217.9759415197746932 ) ) ;
#3776=CARTESIAN_POINT ( 'NONE',  ( 2.178520447619924472, -13.56847537563065487, -221.4085897031499428 ) ) ;
#3778=CARTESIAN_POINT ( 'NONE',  ( -11.98736441306973077, 11.45674391201457176, -217.8252237716743025 ) ) ;
#3779=CARTESIAN_POINT ( 'NONE',  ( -8.929606928624414408, 11.65278034267609186, -219.1999234847403386 ) ) ;
#3781=CARTESIAN_POINT ( 'NONE',  ( -24.48580119005125866, 9.312492396273500006, -232.5498413856076070 ) ) ;
#3782=CARTESIAN_POINT ( 'NONE',  ( -19.98462433625633494, -12.30084073857678639, -216.8518508258974862 ) ) ;
#3785=CARTESIAN_POINT ( 'NONE',  ( -23.98802705797876200, 19.46654170242919690, -223.5293093576406989 ) ) ;
#3786=CARTESIAN_POINT ( 'NONE',  ( 0.3570725323625942860, -15.31465789365257102, -218.3993834748477525 ) ) ;
#3789=CARTESIAN_POINT ( 'NONE',  ( 18.14488609917747652, 6.993670804558928644, -231.4804853770579882 ) ) ;
#3790=CARTESIAN_POINT ( 'NONE',  ( -5.383332542724544645, 15.12651309054520432, -231.5699995578976313 ) ) ;
#3792=CARTESIAN_POINT ( 'NONE',  ( 17.35243190875273811, 16.67741344734974263, -230.5744436858935558 ) ) ;
#3793=CARTESIAN_POINT ( 'NONE',  ( 5.701450259358237460, -28.73672391946437088, -229.2085834618566196 ) ) ;
#3796=CARTESIAN_POINT ( 'NONE',  ( -4.080659539198054020, 15.43130099126780408, -228.8058965243247656 ) ) ;
#3797=CARTESIAN_POINT ( 'NONE',  ( -18.94009481283715957, 3.115208415279245191, -230.3622730452590588 ) ) ;
#3798=CARTESIAN_POINT ( 'NONE',  ( -27.17783334270200157, 15.20409188923851751, -223.6555185980277258 ) ) ;
#3799=CARTESIAN_POINT ( 'NONE',  ( -15.17770002056818868, -9.429316640439420638, -220.2566215541993699 ) ) ;
#3802=CARTESIAN_POINT ( 'NONE',  ( 25.02650711521362936, 17.58144575069911042, -223.6165279156031431 ) ) ;
#3803=CARTESIAN_POINT ( 'NONE',  ( 1.866975752136456279, -28.95217164724439840, -224.5474425503401221 ) ) ;
#3804=CARTESIAN_POINT ( 'NONE',  ( 19.72515656911863147, 14.02277373989196541, -218.0718040828188009 ) ) ;
#3805=CARTESIAN_POINT ( 'NONE',  ( -10.30050448363967419, 10.07750059423401190, -220.1837019037183723 ) ) ;
#3807=CARTESIAN_POINT ( 'NONE',  ( 17.98589043827631428, 2.945998030785370592, -233.4030907785035538 ) ) ;
#3808=CARTESIAN_POINT ( 'NONE',  ( 4.301648988406530094, 13.23079486486395240, -223.2766268961034655 ) ) ;
#3810=CARTESIAN_POINT ( 'NONE',  ( -5.240862053303020573, -11.96147391800445270, -224.1453450823045443 ) ) ;
#3811=CARTESIAN_POINT ( 'NONE',  ( 12.84024077373997841, -14.50125846907313054, -216.8496453050001946 ) ) ;
#3814=CARTESIAN_POINT ( 'NONE',  ( -12.38801939673351704, 9.361418580567464787, -232.8075769614211765 ) ) ;
#3815=CARTESIAN_POINT ( 'NONE',  ( -15.27576489228250090, -6.235258113955679526, -227.2120396213316553 ) ) ;
#3816=CARTESIAN_POINT ( 'NONE',  ( 20.18206873099720156, 1.748383523995667987, -234.4526011791959661 ) ) ;
#3817=CARTESIAN_POINT ( 'NONE',  ( -0.5888410438786807477, 14.99789765555501475, -227.7044550383138244 ) ) ;
#3818=CARTESIAN_POINT ( 'NONE',  ( 5.064106757301036765, 16.06517852189101703, -221.6413221086847329 ) ) ;
#3820=CARTESIAN_POINT ( 'NONE',  ( 11.96323484613444599, -17.37820513000257350, -215.5071828020160183 ) ) ;
#3823=CARTESIAN_POINT ( 'NONE',  ( 23.49048926389013658, 9.645778135078892035, -218.7307869890797463 ) ) ;
#3824=CARTESIAN_POINT ( 'NONE',  ( -10.01410430826631170, 16.10970239316000630, -233.6135099156378203 ) ) ;
#3825=CARTESIAN_POINT ( 'NONE',  ( -16.48591407464216729, 7.092323989942422635, -218.8909951703408012 ) ) ;
#3826=CARTESIAN_POINT ( 'NONE',  ( -20.63475909113443763, -3.483688486440585486, -233.7225001494461480 ) ) ;
#3827=CARTESIAN_POINT ( 'NONE',  ( -14.07917727715460821, 7.534853284453274291, -218.6337090155677458 ) ) ;
#3831=CARTESIAN_POINT ( 'NONE',  ( -18.92390258637512090, 12.75887082072172163, -230.9970325548277970 ) ) ;
#3832=CARTESIAN_POINT ( 'NONE',  ( 24.19672885113291727, 10.99915907690374439, -233.6834417629405891 ) ) ;
#3833=CARTESIAN_POINT ( 'NONE',  ( -28.99926036811508467, 3.909990568804979194, -228.9613767892386988 ) ) ;
#3835=CARTESIAN_POINT ( 'NONE',  ( -26.48368569639269055, -17.40725828600530534, -221.7871577296580199 ) ) ;
#3836=CARTESIAN_POINT ( 'NONE',  ( -27.10757994293576800, -10.52107906247675473, -229.7403242048749519 ) ) ;
#3837=CARTESIAN_POINT ( 'NONE',  ( -11.23881320317003407, 15.84151802331611236, -234.2799649731619809 ) ) ;
#3838=CARTESIAN_POINT ( 'NONE',  ( -9.625604265899946554, -19.21123364792547505, -233.9327940972253259 ) ) ;
#3839=CARTESIAN_POINT ( 'NONE',  ( 4.603870848087811218, 30.13529352683433515, -225.9623629403671430 ) ) ;
#3840=CARTESIAN_POINT ( 'NONE',  ( 5.535251771770903773, -29.91249465213552128, -219.7039649384792028 ) ) ;
#3843=CARTESIAN_POINT ( 'NONE',  ( -22.10934047915427314, 0.9940043559354312386, -216.9999999999999716 ) ) ;
#3844=( NAMED_UNIT ( * ) SI_UNIT ( $, .STERADIAN. ) SOLID_ANGLE_UNIT ( ) );
#3845=CARTESIAN_POINT ( 'NONE',  ( -8.467651734177735534, 23.23776955534497546, -231.2693664226804913 ) ) ;
#3846=CARTESIAN_POINT ( 'NONE',  ( -20.71192633727912380, 6.339941255257877550, -217.2401662359725094 ) ) ;
#3847=CARTESIAN_POINT ( 'NONE',  ( 22.18132842682159733, 5.591149267797686839, -232.0584733989884114 ) ) ;
#3848=CARTESIAN_POINT ( 'NONE',  ( 14.87635807518583775, 11.13002414557121789, -232.1789382499626981 ) ) ;
#3849=CARTESIAN_POINT ( 'NONE',  ( -11.03528491614390994, -18.43141318057359612, -232.7233776306152038 ) ) ;
#3850=CARTESIAN_POINT ( 'NONE',  ( 15.79748369401691122, 19.19631269170049137, -215.0096632418193963 ) ) ;
#3852=CARTESIAN_POINT ( 'NONE',  ( -9.794218246645117532, -15.26311849320921255, -215.4893187949746505 ) ) ;
#3853=CARTESIAN_POINT ( 'NONE',  ( -4.130417896617784912, 16.21758012034559826, -229.8171973319304584 ) ) ;
#3854=CARTESIAN_POINT ( 'NONE',  ( 22.20554449732931346, 18.01468431515759860, -218.9348803756412849 ) ) ;
#3855=CARTESIAN_POINT ( 'NONE',  ( -12.96364545172611571, 10.77137376900670063, -221.1208843751685720 ) ) ;
#3856=CARTESIAN_POINT ( 'NONE',  ( -4.877547524699579640, 12.94924496403020697, -219.3991240521417581 ) ) ;
#3857=CARTESIAN_POINT ( 'NONE',  ( 14.68015846516680867, 2.651775288685355836, -224.1317433549420173 ) ) ;
#3858=CARTESIAN_POINT ( 'NONE',  ( 8.129749879387842881, -22.89596468334109147, -230.6606593278197295 ) ) ;
#3859=ORIENTED_EDGE ( 'NONE', *, *, #13136, .F. ) ;
#3860=CARTESIAN_POINT ( 'NONE',  ( 10.08089751255479527, -9.763210684072014089, -226.4220581413412390 ) ) ;
#3861=CARTESIAN_POINT ( 'NONE',  ( -0.3589900283600636066, 18.35437183075527656, -220.3960288481451357 ) ) ;
#3864=CARTESIAN_POINT ( 'NONE',  ( 10.55627441269396094, 10.31758739525044888, -223.1990319438957613 ) ) ;
#3865=CARTESIAN_POINT ( 'NONE',  ( 17.43540344723615476, -3.335533435063737340, -230.8961756483947738 ) ) ;
#3866=CARTESIAN_POINT ( 'NONE',  ( -15.19144047750087267, -10.24270553329939304, -232.4311702607364793 ) ) ;
#3867=CARTESIAN_POINT ( 'NONE',  ( -6.163092920833200594, -27.00835405423771007, -232.1022292408408987 ) ) ;
#3868=CARTESIAN_POINT ( 'NONE',  ( -2.723069588102707606, 15.58614045890443833, -225.0254611642426141 ) ) ;
#3870=CARTESIAN_POINT ( 'NONE',  ( 24.96615890023450035, 5.871290975262302148, -218.1661911638112201 ) ) ;
#3871=CARTESIAN_POINT ( 'NONE',  ( -6.474151797443945533, 21.29193859232740138, -215.9573456447696458 ) ) ;
#3872=CARTESIAN_POINT ( 'NONE',  ( -9.746008880186941781, 12.96562886885531896, -220.1990846131056401 ) ) ;
#3874=CARTESIAN_POINT ( 'NONE',  ( 6.771176146757415637, 15.60014285904435027, -218.3493856697694753 ) ) ;
#3875=CARTESIAN_POINT ( 'NONE',  ( -23.52458685063474420, 4.195399146287285497, -230.7490123595086970 ) ) ;
#3876=CARTESIAN_POINT ( 'NONE',  ( 16.67941620816951698, 4.093285459228785506, -217.1675623234529269 ) ) ;
#3877=CARTESIAN_POINT ( 'NONE',  ( 13.38323588254664642, -24.59169381177348157, -229.6955247737395780 ) ) ;
#3881=CARTESIAN_POINT ( 'NONE',  ( 9.333020543840051531, 16.91085096921651143, -217.7308990335875762 ) ) ;
#3882=CARTESIAN_POINT ( 'NONE',  ( -13.09367826499460818, -1.871088059101057244, -230.2970504731880510 ) ) ;
#3884=CARTESIAN_POINT ( 'NONE',  ( 18.54610009393809023, 0.6523581019769808531, -231.1787333216317677 ) ) ;
#3885=CARTESIAN_POINT ( 'NONE',  ( 3.342529885312644833, -17.78621320651278737, -216.7788622297345853 ) ) ;
#3887=CARTESIAN_POINT ( 'NONE',  ( -9.517741096562200909, 20.63709896626785678, -234.1036702156204967 ) ) ;
#3888=CARTESIAN_POINT ( 'NONE',  ( -24.33894786102607455, 16.69464852328507831, -227.6320542475859554 ) ) ;
#3890=CARTESIAN_POINT ( 'NONE',  ( -21.93900267957129557, 7.862893636934532360, -233.4951761057262161 ) ) ;
#3891=CARTESIAN_POINT ( 'NONE',  ( -19.75205891382245227, -22.10994567413457546, -223.7241504221178729 ) ) ;
#3895=CARTESIAN_POINT ( 'NONE',  ( -14.07917727715460821, 7.534853284453274291, -218.6337090155677458 ) ) ;
#3896=CARTESIAN_POINT ( 'NONE',  ( 0.3659801352207852077, -13.50984377477715093, -221.1746532791751463 ) ) ;
#3899=CARTESIAN_POINT ( 'NONE',  ( 15.33128967029630729, 6.504525012335983902, -229.0514072561169883 ) ) ;
#3900=CARTESIAN_POINT ( 'NONE',  ( -19.40752943788874774, 15.61499612050012864, -234.7624367253776541 ) ) ;
#3903=CARTESIAN_POINT ( 'NONE',  ( 12.00334754111224100, 12.62951371569041115, -228.5814949098771649 ) ) ;
#3904=CARTESIAN_POINT ( 'NONE',  ( -1.178362239076253370, -26.64461120719161613, -230.8441371545519019 ) ) ;
#3906=CARTESIAN_POINT ( 'NONE',  ( 2.703362520412529779, 29.60004130108520215, -225.6165589735000481 ) ) ;
#3907=CARTESIAN_POINT ( 'NONE',  ( -18.59263364681495290, 22.28600439725833482, -224.9897462721271779 ) ) ;
#3908=CARTESIAN_POINT ( 'NONE',  ( -13.63442241228529994, 1.608023091903783008, -219.2326980015357094 ) ) ;
#3910=CARTESIAN_POINT ( 'NONE',  ( -10.61621529918308227, -15.65610094335291969, -220.0975530242428420 ) ) ;
#3913=CARTESIAN_POINT ( 'NONE',  ( -16.15126510923403202, -0.4755054218165427615, -219.3066569788202571 ) ) ;
#3914=CARTESIAN_POINT ( 'NONE',  ( 3.323726671003152777, -15.99176757603385823, -228.1400570273458186 ) ) ;
#3915=CARTESIAN_POINT ( 'NONE',  ( 23.04897566969193079, 17.95862962700741861, -223.6438515760422661 ) ) ;
#3916=CARTESIAN_POINT ( 'NONE',  ( -2.934221234790329369, 15.07857928364152222, -230.9558365497803720 ) ) ;
#3917=CARTESIAN_POINT ( 'NONE',  ( 16.67941620816951698, 4.093285459228785506, -217.1675623234529269 ) ) ;
#3919=CARTESIAN_POINT ( 'NONE',  ( 10.50530447320976535, 20.19629329636330084, -217.1354359361034767 ) ) ;
#3921=CARTESIAN_POINT ( 'NONE',  ( -5.804961988600464196, -12.67915086496026511, -228.7923277404792088 ) ) ;
#3922=CARTESIAN_POINT ( 'NONE',  ( 25.83609367470520723, -15.13481494965009411, -225.4685613576401124 ) ) ;
#3923=B_SPLINE_CURVE_WITH_KNOTS ( 'NONE', 3,
 ( #19992, #11347, #18218, #13254, #7972, #2777, #21906, #20098, #8308, #18436, #2999, #1326, #14839, #6049, #2884, #16746, #9661, #15176 ),
 .UNSPECIFIED., .F., .F.,
 ( 4, 2, 2, 2, 2, 2, 2, 2, 4 ),
 ( 4.470280076681872704E-18, 0.0004125412386659448559, 0.0008250824773318852666, 0.001237623715997825677, 0.001650164954663766196, 0.002062706193329706499, 0.002475247431995646584, 0.002887788670661587103, 0.003300329909327527622 ),
 .UNSPECIFIED. ) ;
#3926=CARTESIAN_POINT ( 'NONE',  ( -28.12586305337175219, 12.75764838638491305, -230.3810511299127768 ) ) ;
#3927=CARTESIAN_POINT ( 'NONE',  ( -16.27785121718144623, -3.187812258433146084, -227.1052622255949132 ) ) ;
#3928=CARTESIAN_POINT ( 'NONE',  ( -13.70798801564395752, 13.71024986321384809, -218.3360451569033955 ) ) ;
#3929=CARTESIAN_POINT ( 'NONE',  ( 25.62718606866737403, 13.33219119508369310, -230.9315691959737933 ) ) ;
#3930=CARTESIAN_POINT ( 'NONE',  ( 5.909674498212842408, 15.76475534640655773, -228.4922217450045139 ) ) ;
#3932=CARTESIAN_POINT ( 'NONE',  ( 10.87654225111433526, -5.446269956799608458, -227.9455542281931741 ) ) ;
#3934=CARTESIAN_POINT ( 'NONE',  ( 18.60971343765040942, 2.368090295052050820, -218.6871071987073094 ) ) ;
#3935=CARTESIAN_POINT ( 'NONE',  ( -17.94782256308196366, 19.07396065564992682, -232.7143578890335220 ) ) ;
#3936=CARTESIAN_POINT ( 'NONE',  ( -13.31245686955614005, 26.96290519511623174, -230.1796856776773836 ) ) ;
#3937=CARTESIAN_POINT ( 'NONE',  ( -14.01584329375060456, -3.774282517739922405, -220.6818330080343173 ) ) ;
#3938=CARTESIAN_POINT ( 'NONE',  ( -27.90314475660494153, 12.48829126175061077, -223.3300566725355338 ) ) ;
#3940=CARTESIAN_POINT ( 'NONE',  ( 14.64930099072384095, -2.233284345536625803, -226.6630761355773984 ) ) ;
#3941=CARTESIAN_POINT ( 'NONE',  ( -10.07004052286948337, 22.64471483900350179, -217.4645417110143626 ) ) ;
#3942=CARTESIAN_POINT ( 'NONE',  ( 13.85822045549773129, -1.469587484828172919, -226.8778453516271156 ) ) ;
#3943=CARTESIAN_POINT ( 'NONE',  ( -17.84981083811007707, 0.8485253248287054628, -231.8041300026935119 ) ) ;
#3944=CARTESIAN_POINT ( 'NONE',  ( 12.18657022793382794, 26.76558097653315471, -221.8882195427397335 ) ) ;
#3945=CARTESIAN_POINT ( 'NONE',  ( -13.44605823798860200, -7.860403065310468840, -219.7865185367595586 ) ) ;
#3946=CARTESIAN_POINT ( 'NONE',  ( 5.248013545904832711, 18.51731616863089158, -219.3673127389703552 ) ) ;
#3947=CARTESIAN_POINT ( 'NONE',  ( -1.643553855084622928, -13.05119293000219294, -222.7191902239112551 ) ) ;
#3948=CARTESIAN_POINT ( 'NONE',  ( 10.66614775643814994, 26.29080367171353672, -230.0818785118670178 ) ) ;
#3949=CARTESIAN_POINT ( 'NONE',  ( 10.15560415551905749, -12.94826033684588928, -216.3500876866647502 ) ) ;
#3951=CARTESIAN_POINT ( 'NONE',  ( -19.65084584916038324, 18.01805631773661176, -219.5040736310571106 ) ) ;
#3953=CARTESIAN_POINT ( 'NONE',  ( 14.58943670538545412, -3.864781073802256550, -230.4050158740328129 ) ) ;
#3954=CARTESIAN_POINT ( 'NONE',  ( 3.746955526231565248, 25.82691596581962656, -220.7780764774678062 ) ) ;
#3955=CARTESIAN_POINT ( 'NONE',  ( -26.19327040236159831, 13.44417515682194875, -223.7810975255189874 ) ) ;
#3956=CARTESIAN_POINT ( 'NONE',  ( 25.69300549816939494, 5.947472783069708946, -230.6131061331718115 ) ) ;
#3957=CARTESIAN_POINT ( 'NONE',  ( -15.02551512915570697, -20.93241195546420741, -218.9083119944682778 ) ) ;
#3958=CARTESIAN_POINT ( 'NONE',  ( 20.82555317450757215, 14.06078233701296476, -215.4201375757437802 ) ) ;
#3960=CARTESIAN_POINT ( 'NONE',  ( -6.645226799955220365, -27.24439832571371767, -217.1032720093393493 ) ) ;
#3961=CARTESIAN_POINT ( 'NONE',  ( -9.988594796049140356, 11.34066464990972811, -226.6453149279956563 ) ) ;
#3962=CARTESIAN_POINT ( 'NONE',  ( 12.95792863868717149, 16.83236386576623644, -216.3406066345214356 ) ) ;
#3963=CARTESIAN_POINT ( 'NONE',  ( -25.17056316833229701, 11.10725809642625705, -227.0225660235207386 ) ) ;
#3965=CARTESIAN_POINT ( 'NONE',  ( -12.98662328632235585, 28.83726371277012035, -223.5970274767108776 ) ) ;
#3967=CARTESIAN_POINT ( 'NONE',  ( 17.47660375112063491, 0.1533180678384444551, -220.6249646429494931 ) ) ;
#3968=CARTESIAN_POINT ( 'NONE',  ( 7.144583572002897398, -18.19063289417396945, -230.4059351064080658 ) ) ;
#3970=CARTESIAN_POINT ( 'NONE',  ( 13.66436340482409761, -13.84785698770488871, -232.6553000701566134 ) ) ;
#3971=CARTESIAN_POINT ( 'NONE',  ( -2.806347010929339802, 19.90767250424812573, -230.9206976900916004 ) ) ;
#3973=CARTESIAN_POINT ( 'NONE',  ( 16.07305932912010960, 0.9253679043337685872, -229.0409936706996064 ) ) ;
#3974=CARTESIAN_POINT ( 'NONE',  ( -22.30463520409893263, -0.6981587008078518064, -233.9491726243120127 ) ) ;
#3975=CARTESIAN_POINT ( 'NONE',  ( -22.51170993270524789, -14.32174306031543054, -231.7292175355062795 ) ) ;
#3976=CARTESIAN_POINT ( 'NONE',  ( -7.832594822155400927, -23.57318293858060088, -216.4298491688572028 ) ) ;
#3977=CARTESIAN_POINT ( 'NONE',  ( -6.901278853520646628, 15.41233971300566807, -220.5972764307651346 ) ) ;
#3979=CARTESIAN_POINT ( 'NONE',  ( -27.12694304224540076, 7.756125161462346540, -217.3817363082233101 ) ) ;
#3980=CARTESIAN_POINT ( 'NONE',  ( -2.958555384449997661, 13.07587799061801093, -222.7767538261418565 ) ) ;
#3981=CARTESIAN_POINT ( 'NONE',  ( 3.746955526231565248, 25.82691596581962656, -220.7780764774678062 ) ) ;
#3983=CARTESIAN_POINT ( 'NONE',  ( 5.702651035983461902, 12.42242820409033222, -224.7304266323218656 ) ) ;
#3984=CARTESIAN_POINT ( 'NONE',  ( -15.83894155097017631, 1.950284868793920712, -224.5615909987450038 ) ) ;
#3985=CARTESIAN_POINT ( 'NONE',  ( 30.57915561709945251, 3.468229287067555067, -223.8876084027091906 ) ) ;
#3986=CARTESIAN_POINT ( 'NONE',  ( 19.57710422433000019, -21.48596639614413562, -228.6055549924913635 ) ) ;
#3989=CARTESIAN_POINT ( 'NONE',  ( 8.689059922489732912, 15.18271246186214363, -218.7354841152034908 ) ) ;
#3990=CARTESIAN_POINT ( 'NONE',  ( 26.08609146265030176, -9.082777145696592669, -223.3125241607380360 ) ) ;
#3991=CARTESIAN_POINT ( 'NONE',  ( 28.78651053433536333, -0.9604905981993369091, -227.3547688931310233 ) ) ;
#3992=CARTESIAN_POINT ( 'NONE',  ( 6.374306683232226156, -13.38367253400339330, -219.9651431149896723 ) ) ;
#3994=CARTESIAN_POINT ( 'NONE',  ( -17.17400284685640344, 24.63223427531467280, -220.6313524368512162 ) ) ;
#3995=CARTESIAN_POINT ( 'NONE',  ( -7.812160407601123069, 10.19183344000749081, -223.8148904943605828 ) ) ;
#3997=CARTESIAN_POINT ( 'NONE',  ( -11.46843428684449151, 6.508406145394057596, -225.7212143570321814 ) ) ;
#3998=CARTESIAN_POINT ( 'NONE',  ( -23.08212926897555306, -14.71479305961103101, -218.7697472404056214 ) ) ;
#4001=CARTESIAN_POINT ( 'NONE',  ( -13.93333636822611155, 3.327141996558931947, -221.4468162587888287 ) ) ;
#4002=CARTESIAN_POINT ( 'NONE',  ( 9.678950682101415737, -24.51930918146190663, -231.5088683414745105 ) ) ;
#4004=CARTESIAN_POINT ( 'NONE',  ( -28.13472254077564116, 12.33996625515159629, -224.9141344439281909 ) ) ;
#4006=CARTESIAN_POINT ( 'NONE',  ( 14.68130101653174613, 6.427210486143660084, -228.0153742661088074 ) ) ;
#4007=CARTESIAN_POINT ( 'NONE',  ( -8.716816145717144693, 12.22834664005217675, -231.7124508691059646 ) ) ;
#4009=CARTESIAN_POINT ( 'NONE',  ( 18.90025403853754327, 17.70150481658638952, -229.5234643039372315 ) ) ;
#4010=CARTESIAN_POINT ( 'NONE',  ( 1.038689920556553847, -18.98022482494055652, -217.9213632692622866 ) ) ;
#4012=CARTESIAN_POINT ( 'NONE',  ( -0.3197916200495275474, 16.38897215927557482, -229.9606066735827028 ) ) ;
#4013=CARTESIAN_POINT ( 'NONE',  ( -18.36252859017411510, 21.06344830687906367, -228.5073589488702623 ) ) ;
#4014=CARTESIAN_POINT ( 'NONE',  ( -14.83806045519817829, 13.18806197935771074, -233.4179411789645542 ) ) ;
#4016=CARTESIAN_POINT ( 'NONE',  ( -17.87876569233342749, -13.82805272504658944, -230.9569051913176168 ) ) ;
#4018=VERTEX_POINT ( 'NONE', #1861 ) ;
#4019=CARTESIAN_POINT ( 'NONE',  ( -17.88126539071149779, 5.766250685202066961, -232.9050303536861293 ) ) ;
#4020=CARTESIAN_POINT ( 'NONE',  ( 3.208289162541382300, -18.46136333555241293, -230.6641274008648850 ) ) ;
#4021=CARTESIAN_POINT ( 'NONE',  ( 24.57222455393806015, 12.08236629421828212, -229.7319216558644541 ) ) ;
#4022=CARTESIAN_POINT ( 'NONE',  ( 5.141746912158045468, 22.01688500372448232, -216.6678693612369386 ) ) ;
#4025=CARTESIAN_POINT ( 'NONE',  ( -27.11599398522282911, 10.60460483532474996, -224.7310548435675912 ) ) ;
#4026=CARTESIAN_POINT ( 'NONE',  ( 14.28815361401014172, 13.86049093364188778, -216.0585456615740156 ) ) ;
#4028=CARTESIAN_POINT ( 'NONE',  ( 13.03557269046774714, 7.519834803053426775, -226.9490612297269081 ) ) ;
#4030=CARTESIAN_POINT ( 'NONE',  ( -5.279374154171231126, -12.28263746854076466, -222.5283095625445640 ) ) ;
#4031=CARTESIAN_POINT ( 'NONE',  ( 8.115778909262310492, -29.92983049028717346, -224.5060555478150377 ) ) ;
#4034=CARTESIAN_POINT ( 'NONE',  ( -10.49339404011726984, 12.66576824096800991, -217.2681947942554643 ) ) ;
#4035=CARTESIAN_POINT ( 'NONE',  ( -16.47483915600249205, -3.991485801086211538, -222.0851216934102297 ) ) ;
#4036=CARTESIAN_POINT ( 'NONE',  ( -21.23733589435050817, 17.25275849955597351, -229.9547908233139708 ) ) ;
#4037=CARTESIAN_POINT ( 'NONE',  ( 12.08198696763335178, 15.54678077493410981, -216.6084679670902631 ) ) ;
#4038=CARTESIAN_POINT ( 'NONE',  ( -1.946052076048385482, 22.23149728939677061, -232.8927760318659068 ) ) ;
#4040=CARTESIAN_POINT ( 'NONE',  ( 25.79180107113126397, -16.09695083256378112, -231.0225534820104656 ) ) ;
#4041=CARTESIAN_POINT ( 'NONE',  ( 24.57222455393806015, 12.08236629421828212, -229.7319216558644541 ) ) ;
#4044=CARTESIAN_POINT ( 'NONE',  ( 0.6332696906856497554, 18.74964962670039625, -234.8596399859513042 ) ) ;
#4045=CARTESIAN_POINT ( 'NONE',  ( -16.28135616697389310, 20.98764039357472200, -216.9434553755565958 ) ) ;
#4046=CARTESIAN_POINT ( 'NONE',  ( -29.05925532287432489, -3.238226816112620199, -230.1495230746535867 ) ) ;
#4048=CARTESIAN_POINT ( 'NONE',  ( -12.78558550453068854, 7.693178343823584342, -230.0800953344970878 ) ) ;
#4052=CARTESIAN_POINT ( 'NONE',  ( 2.068961274655788607, 15.13167107497539376, -217.8084559455312501 ) ) ;
#4053=CARTESIAN_POINT ( 'NONE',  ( 13.70635042947887428, -1.390919209824193592, -225.3477037409554953 ) ) ;
#4054=CARTESIAN_POINT ( 'NONE',  ( 17.89221702206198117, 0.2742047965568425449, -220.2420650470893122 ) ) ;
#4055=CARTESIAN_POINT ( 'NONE',  ( 14.31308345469695453, 12.76656023072872159, -231.9445021321040770 ) ) ;
#4058=CARTESIAN_POINT ( 'NONE',  ( -22.19673167533144564, -9.562764463827019057, -233.1557790568585062 ) ) ;
#4059=CARTESIAN_POINT ( 'NONE',  ( -9.060295054034883222, 29.20313342278041802, -224.2979742714222482 ) ) ;
#4060=CARTESIAN_POINT ( 'NONE',  ( -0.8413160509385254615, -28.71376977722865931, -218.8117683208458288 ) ) ;
#4061=CARTESIAN_POINT ( 'NONE',  ( 4.883314309504700468, 19.06839645569368358, -217.0171359871271193 ) ) ;
#4062=CARTESIAN_POINT ( 'NONE',  ( 5.982199551433209805, -30.67818700677413091, -221.2919386232889849 ) ) ;
#4063=CARTESIAN_POINT ( 'NONE',  ( 15.37450427861381286, -5.898921106289613847E-14, -228.0000000000000853 ) ) ;
#4064=CARTESIAN_POINT ( 'NONE',  ( -11.35482716595652875, 11.86850131893102223, -220.6599844941370350 ) ) ;
#4066=CARTESIAN_POINT ( 'NONE',  ( -18.30524310960561252, -4.731645231655051909, -231.4308113063693781 ) ) ;
#4067=CARTESIAN_POINT ( 'NONE',  ( 6.402706778685327116, 14.41397785959879307, -226.0127495172349086 ) ) ;
#4068=CARTESIAN_POINT ( 'NONE',  ( -17.39737143130126285, 7.531548707695031375, -232.0788227848755696 ) ) ;
#4069=CARTESIAN_POINT ( 'NONE',  ( -16.99821283087967672, -0.5135051709387361552, -216.2173766440975555 ) ) ;
#4070=CARTESIAN_POINT ( 'NONE',  ( -19.73058714482073128, -19.33240507441191625, -228.8766180877602494 ) ) ;
#4071=CARTESIAN_POINT ( 'NONE',  ( 26.56239871811266440, 9.439457669498057868, -217.7226690415261885 ) ) ;
#4075=CARTESIAN_POINT ( 'NONE',  ( -6.608244874605412100, -9.640126028631323507, -223.8427097396816805 ) ) ;
#4076=CARTESIAN_POINT ( 'NONE',  ( 9.336393807558161839, 27.79372469574263960, -228.5913636680961361 ) ) ;
#4077=CARTESIAN_POINT ( 'NONE',  ( 21.38922145650625239, 17.10616209967719215, -217.8354246241890451 ) ) ;
#4078=CARTESIAN_POINT ( 'NONE',  ( -9.523248388595575875, 12.31121908620753125, -221.6288572946744182 ) ) ;
#4079=CARTESIAN_POINT ( 'NONE',  ( -5.543543819386913540, 14.51457927969963713, -217.3847528063896846 ) ) ;
#4080=CARTESIAN_POINT ( 'NONE',  ( 16.31458447723494132, 2.619382102851042671, -229.5862799001085364 ) ) ;
#4081=CARTESIAN_POINT ( 'NONE',  ( 14.18740332497314149, -14.20295060558812672, -230.7262566610843351 ) ) ;
#4082=CARTESIAN_POINT ( 'NONE',  ( 4.999282783285113219, -13.99249059192112021, -223.3817383379047214 ) ) ;
#4085=CARTESIAN_POINT ( 'NONE',  ( 15.05360126642391450, 1.481754003466396963, -222.9454997252120734 ) ) ;
#4086=CARTESIAN_POINT ( 'NONE',  ( 23.36729170583618398, -5.500043712341283531, -232.1593072787115375 ) ) ;
#4087=CARTESIAN_POINT ( 'NONE',  ( -18.75993824683981970, -9.028840681436806292, -217.1556094966459227 ) ) ;
#4089=CARTESIAN_POINT ( 'NONE',  ( -0.1947256686167265494, -30.94043057420685727, -223.1178397439027492 ) ) ;
#4090=CARTESIAN_POINT ( 'NONE',  ( 7.017641603801325623, 14.96204511409594673, -228.1064041248110073 ) ) ;
#4092=CARTESIAN_POINT ( 'NONE',  ( -17.17143024911216287, 2.756036084795755681, -233.9491886983466316 ) ) ;
#4094=CARTESIAN_POINT ( 'NONE',  ( -10.24288955603410933, 28.30762631303078791, -220.8855665231519083 ) ) ;
#4095=CARTESIAN_POINT ( 'NONE',  ( 1.455106383990497187, 21.12056149333958999, -230.8076663600630241 ) ) ;
#4096=CARTESIAN_POINT ( 'NONE',  ( 13.49429091642815770, -0.3433647160923702368, -223.9641315955981895 ) ) ;
#4097=CARTESIAN_POINT ( 'NONE',  ( 10.49811526528768368, 13.26166588535847701, -217.9009921269571919 ) ) ;
#4098=CARTESIAN_POINT ( 'NONE',  ( -22.03660207690921879, 17.07234836129451949, -222.7335359861421296 ) ) ;
#4099=CARTESIAN_POINT ( 'NONE',  ( 14.81251837262747983, -1.020578734748967209, -221.0290343291311785 ) ) ;
#4100=CARTESIAN_POINT ( 'NONE',  ( 1.874647746501092893, -15.20125101474619633, -222.7462710229423521 ) ) ;
#4103=CARTESIAN_POINT ( 'NONE',  ( 4.907833106823921376, 13.98151846258800290, -229.0190609869640923 ) ) ;
#4104=CARTESIAN_POINT ( 'NONE',  ( -20.47121909278842722, -2.147015668718357695, -235.2226201655121258 ) ) ;
#4105=CARTESIAN_POINT ( 'NONE',  ( -17.43458823433387650, 2.804998135793385750, -231.8077100320880959 ) ) ;
#4106=CARTESIAN_POINT ( 'NONE',  ( 7.021536848793814123, -14.49751826649810482, -218.4909385705359455 ) ) ;
#4108=CARTESIAN_POINT ( 'NONE',  ( 2.539761864897490007, 23.64215977235053501, -233.4645566207487661 ) ) ;
#4110=CARTESIAN_POINT ( 'NONE',  ( -11.01414002179357610, 8.614420160880040811, -226.3770540798392972 ) ) ;
#4112=CARTESIAN_POINT ( 'NONE',  ( -10.30050448363967419, 10.07750059423401190, -220.1837019037183723 ) ) ;
#4113=CARTESIAN_POINT ( 'NONE',  ( -19.02606456345395358, -20.49905271945607055, -219.9673098173381902 ) ) ;
#4116=CARTESIAN_POINT ( 'NONE',  ( -4.104500432947460808, 15.73223271406093460, -218.0734292856946297 ) ) ;
#4117=CARTESIAN_POINT ( 'NONE',  ( 3.881011284096109293, -13.04786028604701187, -224.6787317506201589 ) ) ;
#4119=CARTESIAN_POINT ( 'NONE',  ( -13.56774755469388616, 7.311522441667196226, -219.1912666243428021 ) ) ;
#4120=CARTESIAN_POINT ( 'NONE',  ( -31.04267853410473421, 7.029517189377418873, -226.8060334161593516 ) ) ;
#4121=CARTESIAN_POINT ( 'NONE',  ( -1.565160934061885500, 18.19073094521525391, -232.0278805765578909 ) ) ;
#4123=CARTESIAN_POINT ( 'NONE',  ( 18.39384604806649648, 2.566915855367216004, -231.7421336352533103 ) ) ;
#4124=CARTESIAN_POINT ( 'NONE',  ( -15.65248652229887405, -15.36320747609890169, -219.0899148657056230 ) ) ;
#4125=B_SPLINE_CURVE_WITH_KNOTS ( 'NONE', 3,
 ( #12184, #21160, #259, #19474, #20944, #17696, #12294, #19038, #7011, #4063 ),
 .UNSPECIFIED., .F., .F.,
 ( 4, 2, 2, 2, 4 ),
 ( 0.003847469879456770925, 0.004275615195033988063, 0.004703760510611204766, 0.005131905826188422337, 0.005560051141765639041 ),
 .UNSPECIFIED. ) ;
#4127=CARTESIAN_POINT ( 'NONE',  ( 7.213476267053916757, 16.78447451494783138, -217.5857052077849687 ) ) ;
#4128=CARTESIAN_POINT ( 'NONE',  ( -7.266348978356541366, 16.38312187400933340, -217.9429203627011873 ) ) ;
#4129=CARTESIAN_POINT ( 'NONE',  ( -8.308618357598591686, 12.44656112581930785, -228.0014162119141474 ) ) ;
#4130=CARTESIAN_POINT ( 'NONE',  ( -18.95931133506032040, -20.40484553783743138, -225.1835090426186525 ) ) ;
#4135=CARTESIAN_POINT ( 'NONE',  ( -13.11494368899652052, 3.355507568391938200, -225.9121440085824304 ) ) ;
#4136=CARTESIAN_POINT ( 'NONE',  ( -1.602612909676673469, -20.69807258397210248, -232.3153362903766492 ) ) ;
#4137=CARTESIAN_POINT ( 'NONE',  ( 21.25094435758043332, 17.68230636442804027, -229.7964888993842010 ) ) ;
#4138=CARTESIAN_POINT ( 'NONE',  ( 3.763426558366607111, 28.60172112197566818, -230.1816715025297526 ) ) ;
#4140=CARTESIAN_POINT ( 'NONE',  ( -27.01279207917464475, 4.316569700791554887, -221.4451031230926219 ) ) ;
#4141=CARTESIAN_POINT ( 'NONE',  ( 19.97628502126439187, 24.50819884991013708, -224.8824979922784735 ) ) ;
#4142=CARTESIAN_POINT ( 'NONE',  ( 11.57669841200422134, 10.63052136557218574, -228.9489978335593889 ) ) ;
#4144=CARTESIAN_POINT ( 'NONE',  ( -13.13432812001650341, -19.42279346457301514, -216.4126494286626610 ) ) ;
#4145=CARTESIAN_POINT ( 'NONE',  ( 6.374306683232226156, -13.38367253400339330, -219.9651431149896723 ) ) ;
#4148=CARTESIAN_POINT ( 'NONE',  ( -4.591517861330576267, 12.55780501983563191, -223.5932882008353033 ) ) ;
#4149=CARTESIAN_POINT ( 'NONE',  ( 18.01918173885548313, -1.728726289433203611, -215.5890043894241330 ) ) ;
#4150=CARTESIAN_POINT ( 'NONE',  ( 20.80196158924851701, -7.261721507697286526, -217.3074963141844194 ) ) ;
#4151=CARTESIAN_POINT ( 'NONE',  ( 10.49811526528768368, 13.26166588535847701, -217.9009921269571919 ) ) ;
#4152=CARTESIAN_POINT ( 'NONE',  ( 10.90137817157632227, 16.64712710991609868, -230.5401786220292593 ) ) ;
#4154=CARTESIAN_POINT ( 'NONE',  ( 13.42370487565828796, -6.089723759188163221, -217.7532606872487406 ) ) ;
#4155=CARTESIAN_POINT ( 'NONE',  ( 18.04365516558436866, 6.721233635139160612, -218.4376093631473168 ) ) ;
#4156=CARTESIAN_POINT ( 'NONE',  ( 0.9169988354999972779, 20.59043933275470550, -235.2854195559275752 ) ) ;
#4157=CARTESIAN_POINT ( 'NONE',  ( -5.028549462823471039, 18.55099042571767143, -234.6264744246184648 ) ) ;
#4158=CARTESIAN_POINT ( 'NONE',  ( -23.30703516638871875, -0.6243632158918477337, -216.1214812734271220 ) ) ;
#4159=CARTESIAN_POINT ( 'NONE',  ( -24.24202834850560606, 19.05981756344202438, -226.6980666352953335 ) ) ;
#4161=EDGE_CURVE ( 'NONE', #5173, #161, #15697, .T. ) ;
#4162=STYLED_ITEM ( 'NONE', ( #20832 ), #21952 ) ;
#4163=CARTESIAN_POINT ( 'NONE',  ( 27.96460686140487084, -1.872811165202790340, -220.9791906660856000 ) ) ;
#4164=CARTESIAN_POINT ( 'NONE',  ( -1.806671251568986669, 13.52068930966770388, -228.3567401718105430 ) ) ;
#4165=CARTESIAN_POINT ( 'NONE',  ( 28.77543668145700195, 2.466904630248945907, -219.6646827587300947 ) ) ;
#4166=CARTESIAN_POINT ( 'NONE',  ( -14.07917727715460821, 7.534853284453274291, -218.6337090155677458 ) ) ;
#4167=CARTESIAN_POINT ( 'NONE',  ( 17.99029889091409018, 9.613712288440757092, -232.0298403238024036 ) ) ;
#4168=CARTESIAN_POINT ( 'NONE',  ( 15.58734083230706524, 0.8631096974226073471, -227.8746545404512744 ) ) ;
#4171=CARTESIAN_POINT ( 'NONE',  ( -1.837924626891132229, 29.27703531260187475, -227.2344808100871774 ) ) ;
#4172=CARTESIAN_POINT ( 'NONE',  ( -13.72709560065558421, -5.132649126379569715, -227.9317987811764965 ) ) ;
#4173=CARTESIAN_POINT ( 'NONE',  ( 5.343558017910363667, 26.29639771561252459, -218.1010331760174665 ) ) ;
#4174=CARTESIAN_POINT ( 'NONE',  ( -7.753256282497156704, -15.05334625439219565, -219.2728364670455221 ) ) ;
#4177=CARTESIAN_POINT ( 'NONE',  ( -13.31590776630363315, 5.340120742929252096, -225.6956515496373186 ) ) ;
#4179=CARTESIAN_POINT ( 'NONE',  ( 12.99512476935412231, -3.120572961704727977, -223.7636045402963987 ) ) ;
#4180=CARTESIAN_POINT ( 'NONE',  ( 4.894897393135387631, 18.48819632322109996, -230.2131424875790628 ) ) ;
#4181=CARTESIAN_POINT ( 'NONE',  ( -22.24722865165759345, 18.77558306771206986, -226.5077042908023941 ) ) ;
#4182=CARTESIAN_POINT ( 'NONE',  ( -29.65068623107463708, 4.004319520977249525, -231.5200339834770773 ) ) ;
#4183=CARTESIAN_POINT ( 'NONE',  ( -13.15060755141140980, -21.73659206351220519, -231.8601396556976226 ) ) ;
#4184=CARTESIAN_POINT ( 'NONE',  ( 13.85207896949186335, 7.847214149978243292, -217.3457543576531066 ) ) ;
#4186=CARTESIAN_POINT ( 'NONE',  ( -12.86575055733568540, -10.70886189207742589, -216.1397835820578450 ) ) ;
#4187=CARTESIAN_POINT ( 'NONE',  ( -2.435715273212520238, 23.41098772907853132, -217.6796576669356966 ) ) ;
#4188=CARTESIAN_POINT ( 'NONE',  ( 17.23498165643884761, 6.576565757823654934, -216.5785374982484655 ) ) ;
#4189=CARTESIAN_POINT ( 'NONE',  ( -18.59263364681495290, 22.28600439725833482, -224.9897462721271779 ) ) ;
#4190=CARTESIAN_POINT ( 'NONE',  ( 19.29971334243027314, 24.42889259816135095, -228.2141526116784291 ) ) ;
#4192=CARTESIAN_POINT ( 'NONE',  ( -3.368184987477955694, -15.91886893360235078, -219.1066823976216256 ) ) ;
#4193=CARTESIAN_POINT ( 'NONE',  ( 6.250374750423979719, -27.98416211894771521, -222.2453514702945085 ) ) ;
#4195=CARTESIAN_POINT ( 'NONE',  ( 18.04365516558436866, 6.721233635139160612, -218.4376093631473168 ) ) ;
#4196=CARTESIAN_POINT ( 'NONE',  ( 12.13827923251525220, -9.172799829723585319, -229.1860353116090891 ) ) ;
#4197=CARTESIAN_POINT ( 'NONE',  ( -17.42499862437977853, -18.98713029041037004, -232.7811807006768845 ) ) ;
#4198=CARTESIAN_POINT ( 'NONE',  ( -19.50907964299920039, -17.77536300509877876, -217.8007844881196320 ) ) ;
#4199=CARTESIAN_POINT ( 'NONE',  ( 3.388180927852674884, 15.71154068801650538, -224.9339660840813053 ) ) ;
#4201=CARTESIAN_POINT ( 'NONE',  ( 14.32363442937021425, 2.978337679677412808, -227.0386046113487453 ) ) ;
#4202=CARTESIAN_POINT ( 'NONE',  ( -3.501680520304516264, 14.31538576447642264, -219.8967178229432307 ) ) ;
#4203=CARTESIAN_POINT ( 'NONE',  ( -3.130917144532865848, 26.01013079854885390, -229.4331404728494874 ) ) ;
#4204=CARTESIAN_POINT ( 'NONE',  ( 29.83024462204712179, 0.7507192471929857724, -227.4186229137179396 ) ) ;
#4206=CARTESIAN_POINT ( 'NONE',  ( 11.64932556965463561, 7.668732705389711413, -229.0406978839571366 ) ) ;
#4207=CARTESIAN_POINT ( 'NONE',  ( -14.59766675578715223, 7.926254675926275972, -222.3706877972550444 ) ) ;
#4208=CARTESIAN_POINT ( 'NONE',  ( 19.49137065790598555, 9.165486118354671419, -234.8706749352814995 ) ) ;
#4209=CARTESIAN_POINT ( 'NONE',  ( 0.7797512750231831991, -26.58197935702783354, -230.4407411870234625 ) ) ;
#4212=CARTESIAN_POINT ( 'NONE',  ( 12.04687593227112430, 27.54339840196571743, -224.6466266724203820 ) ) ;
#4213=CARTESIAN_POINT ( 'NONE',  ( 22.59847068942421444, -14.29990159211854106, -221.3422834976353499 ) ) ;
#4215=CARTESIAN_POINT ( 'NONE',  ( -6.722478243781921492, -14.20656108661463612, -231.4169491518476889 ) ) ;
#4216=CARTESIAN_POINT ( 'NONE',  ( 0.7245137624042983227, 13.44764381486384330, -223.4043886706536455 ) ) ;
#4217=CARTESIAN_POINT ( 'NONE',  ( -5.373457274256926652, 30.83572167890261184, -229.2199105909169532 ) ) ;
#4219=CARTESIAN_POINT ( 'NONE',  ( -9.250876228778270871, 9.538614635316015722, -227.1332118982684563 ) ) ;
#4220=CARTESIAN_POINT ( 'NONE',  ( -20.63475909113443763, -3.483688486440585486, -233.7225001494461480 ) ) ;
#4224=CARTESIAN_POINT ( 'NONE',  ( -9.443239614166923701, 9.388015667058336788, -222.3195230688234290 ) ) ;
#4225=CARTESIAN_POINT ( 'NONE',  ( 8.990474075060864934, -28.03008174514034678, -221.5310560963409330 ) ) ;
#4226=CARTESIAN_POINT ( 'NONE',  ( 24.59129902578158067, -8.191391589517788674, -218.4338547727923299 ) ) ;
#4227=CARTESIAN_POINT ( 'NONE',  ( -25.80904414196669450, 12.19501778665756220, -219.1732313092283846 ) ) ;
#4228=CARTESIAN_POINT ( 'NONE',  ( 15.80790828609669951, 3.698719088746416972, -219.8106174092292804 ) ) ;
#4229=CARTESIAN_POINT ( 'NONE',  ( -7.834600152078401436, 27.83486203824852012, -220.1209588485844222 ) ) ;
#4230=CARTESIAN_POINT ( 'NONE',  ( 13.75457993763798648, 0.05083669377823854529, -228.0000000000000853 ) ) ;
#4231=CARTESIAN_POINT ( 'NONE',  ( 17.32394486779715592, 4.028159306070694612, -218.4253989884176690 ) ) ;
#4232=CARTESIAN_POINT ( 'NONE',  ( -11.18644257538908526, -20.90776414258732174, -230.8249452324125173 ) ) ;
#4234=CARTESIAN_POINT ( 'NONE',  ( 9.527502190795640757, 23.55559004943647139, -217.4101659741468211 ) ) ;
#4235=CARTESIAN_POINT ( 'NONE',  ( -11.13829636790841704, 14.30978168460582189, -218.6922574227322400 ) ) ;
#4236=CARTESIAN_POINT ( 'NONE',  ( -12.33997807949817904, 15.01940705987184188, -217.6798968600957380 ) ) ;
#4237=CARTESIAN_POINT ( 'NONE',  ( 23.84888352507021736, -3.411310983279423947, -216.3556234003997645 ) ) ;
#4240=CARTESIAN_POINT ( 'NONE',  ( 18.79638869589749461, 0.4878066561304963966, -219.5712168927955759 ) ) ;
#4241=CARTESIAN_POINT ( 'NONE',  ( -5.474373895759362618, -29.29005893717160092, -223.2371403555430334 ) ) ;
#4242=CARTESIAN_POINT ( 'NONE',  ( 15.15867943830037134, 1.437942759855808772, -227.6349539663164876 ) ) ;
#4243=CARTESIAN_POINT ( 'NONE',  ( 4.340445191644851874, 29.86837761166362881, -227.4879512554873315 ) ) ;
#4244=CARTESIAN_POINT ( 'NONE',  ( 14.87215633904093082, -2.419155424398304888, -226.7769793042785125 ) ) ;
#4245=CARTESIAN_POINT ( 'NONE',  ( -25.06333669508177309, 2.553070212212491530, -230.2963116797556893 ) ) ;
#4246=CARTESIAN_POINT ( 'NONE',  ( 23.83082175545800752, 15.77842900014857896, -219.5351905769044834 ) ) ;
#4248=CARTESIAN_POINT ( 'NONE',  ( 21.35706335192880445, 15.67286272432725092, -219.2578158352350783 ) ) ;
#4251=CARTESIAN_POINT ( 'NONE',  ( -26.69331514234889013, -17.84497232456928373, -223.5918739730229845 ) ) ;
#4252=CARTESIAN_POINT ( 'NONE',  ( -20.11874861854083463, -21.11755179634840474, -229.7504124090357323 ) ) ;
#4253=CARTESIAN_POINT ( 'NONE',  ( 5.451525948382545117, -12.45300865616632713, -227.8545162512558306 ) ) ;
#4256=CARTESIAN_POINT ( 'NONE',  ( -16.23478446547628096, 26.31175924651574149, -222.4178907105033431 ) ) ;
#4257=CARTESIAN_POINT ( 'NONE',  ( 24.13177372007769961, -1.862525787088729956, -215.1116454360890202 ) ) ;
#4258=CARTESIAN_POINT ( 'NONE',  ( 25.69761320619099720, -8.403105518750903613, -219.2599777650661110 ) ) ;
#4259=CARTESIAN_POINT ( 'NONE',  ( -26.38808873681881906, 13.30696350521622939, -225.1492950792419663 ) ) ;
#4260=CARTESIAN_POINT ( 'NONE',  ( 18.23116248274160256, 13.99874872632082123, -216.0593560670294835 ) ) ;
#4261=CARTESIAN_POINT ( 'NONE',  ( 12.60818910183731489, 13.02403301690871729, -229.3305689548085695 ) ) ;
#4263=CARTESIAN_POINT ( 'NONE',  ( 5.517988016436452980, -29.70724229459007759, -226.4438119151823514 ) ) ;
#4265=CARTESIAN_POINT ( 'NONE',  ( -8.123851230256436295, 20.56863949923577550, -215.0796075421103239 ) ) ;
#4266=CARTESIAN_POINT ( 'NONE',  ( -12.80532875684362715, 24.61139456694233374, -232.5885756414849084 ) ) ;
#4267=CARTESIAN_POINT ( 'NONE',  ( -16.38803511840525218, -9.809678413005567421, -217.1940421839195494 ) ) ;
#4268=CARTESIAN_POINT ( 'NONE',  ( -15.66530208164916260, 23.23467148471576849, -218.1250122661128046 ) ) ;
#4270=CARTESIAN_POINT ( 'NONE',  ( 29.12543877365354916, -1.475122899492763873, -224.0746120762670444 ) ) ;
#4271=CARTESIAN_POINT ( 'NONE',  ( -4.651113456395510326, 27.58151660986499110, -218.3072938287727141 ) ) ;
#4272=CARTESIAN_POINT ( 'NONE',  ( -16.08005950484750102, -0.1764640578214327904, -223.5999988222837942 ) ) ;
#4273=CARTESIAN_POINT ( 'NONE',  ( -16.65698539163286540, 11.03290537638306112, -233.6474915129378758 ) ) ;
#4274=CARTESIAN_POINT ( 'NONE',  ( 17.00168025137501004, 6.212099629982537508, -219.0548246536471595 ) ) ;
#4276=CARTESIAN_POINT ( 'NONE',  ( 5.064106757301036765, 16.06517852189101703, -221.6413221086847329 ) ) ;
#4277=CARTESIAN_POINT ( 'NONE',  ( -24.15031621174628285, -13.05338392360020627, -219.0842748323915714 ) ) ;
#4278=CARTESIAN_POINT ( 'NONE',  ( 15.87442104186276381, 8.674488492264579520, -230.9702037640878416 ) ) ;
#4279=CARTESIAN_POINT ( 'NONE',  ( 1.040523496405688642, -16.53460264249922318, -217.0944950338946455 ) ) ;
#4282=CARTESIAN_POINT ( 'NONE',  ( -13.96147744945181124, 5.260363697127891314, -222.3342733685200301 ) ) ;
#4283=CARTESIAN_POINT ( 'NONE',  ( 15.56514059923893178, -9.210181625211102840, -232.5361143517874325 ) ) ;
#4284=CARTESIAN_POINT ( 'NONE',  ( 15.03112630398312177, 24.11065413595933293, -226.8236212149936080 ) ) ;
#4285=CARTESIAN_POINT ( 'NONE',  ( -24.39036648059286350, 13.21953970265592027, -220.1632778389106591 ) ) ;
#4286=CARTESIAN_POINT ( 'NONE',  ( -16.81617677814535128, 0.6259372974186930838, -233.5115673467681745 ) ) ;
#4287=CARTESIAN_POINT ( 'NONE',  ( -22.88587990158785601, -12.52061884883742238, -220.5813279352508687 ) ) ;
#4288=CARTESIAN_POINT ( 'NONE',  ( 11.75404126451729070, 5.688294280104953415, -229.3533586468489602 ) ) ;
#4290=CARTESIAN_POINT ( 'NONE',  ( -11.72787654052445028, -3.882995534642332824, -226.9210218758430244 ) ) ;
#4291=CARTESIAN_POINT ( 'NONE',  ( 2.951582164238582440, 19.39026647431845873, -217.4356918981242472 ) ) ;
#4292=CARTESIAN_POINT ( 'NONE',  ( -16.98287383830707142, 1.584866439881522648, -221.5391863673846444 ) ) ;
#4293=CARTESIAN_POINT ( 'NONE',  ( -5.629016366058284149, 14.31889596247328633, -229.4177297515988414 ) ) ;
#4294=CARTESIAN_POINT ( 'NONE',  ( 11.84598249547323690, 10.36127485500543699, -218.5481300776139904 ) ) ;
#4295=CARTESIAN_POINT ( 'NONE',  ( -4.782174899302804150, -29.09898918907212817, -227.3916599557566940 ) ) ;
#4296=CARTESIAN_POINT ( 'NONE',  ( -1.339836966046043631, -21.49735173129188581, -217.9043760890963313 ) ) ;
#4297=CARTESIAN_POINT ( 'NONE',  ( 16.91879448796214191, 0.8271603773820436212, -230.0510230802265710 ) ) ;
#4298=CARTESIAN_POINT ( 'NONE',  ( 11.78320976064766690, -8.193118641535518165, -222.2581747538435479 ) ) ;
#4299=CARTESIAN_POINT ( 'NONE',  ( 16.22685372911609036, -0.3790667790403521309, -218.4894315352551644 ) ) ;
#4300=CARTESIAN_POINT ( 'NONE',  ( -5.525229149912007642, -13.32411127922494742, -220.4018445532201440 ) ) ;
#4301=CARTESIAN_POINT ( 'NONE',  ( 15.50648685944955218, 24.16641006378193168, -224.4827813270165393 ) ) ;
#4303=CARTESIAN_POINT ( 'NONE',  ( -24.69837543585720141, 12.57569301576483589, -232.4521327773205428 ) ) ;
#4304=CARTESIAN_POINT ( 'NONE',  ( 4.389496648589924277, 14.47660514356954131, -220.6151178996808540 ) ) ;
#4305=CARTESIAN_POINT ( 'NONE',  ( 4.894897393135387631, 18.48819632322109996, -230.2131424875790628 ) ) ;
#4306=CARTESIAN_POINT ( 'NONE',  ( 29.31647908907816102, 0.9594737942742700421, -228.5782466420670858 ) ) ;
#4308=CARTESIAN_POINT ( 'NONE',  ( 16.64575860537911112, 25.12688477742292648, -227.5050599151411745 ) ) ;
#4309=CARTESIAN_POINT ( 'NONE',  ( -13.58070052954164275, 11.19572749768420650, -220.2511552028196604 ) ) ;
#4310=CARTESIAN_POINT ( 'NONE',  ( -25.94982248293519689, 10.67899231259548287, -221.1273147719203962 ) ) ;
#4311=CARTESIAN_POINT ( 'NONE',  ( 5.191785474240024456, -25.78595846473334419, -219.2330600099714673 ) ) ;
#4314=CARTESIAN_POINT ( 'NONE',  ( 5.169766346882679997, 29.28517558595074988, -221.5178724947562614 ) ) ;
#4315=CARTESIAN_POINT ( 'NONE',  ( 12.91525526572063853, -9.549346049255611035, -226.1928206613168584 ) ) ;
#4318=CARTESIAN_POINT ( 'NONE',  ( -7.832594822155400927, -23.57318293858060088, -216.4298491688572028 ) ) ;
#4319=CARTESIAN_POINT ( 'NONE',  ( -3.755296588130283553, 23.77975947300719284, -233.7323173085780752 ) ) ;
#4320=CARTESIAN_POINT ( 'NONE',  ( -0.04850409037381671340, 14.20520396026658716, -231.8092226852533031 ) ) ;
#4322=CARTESIAN_POINT ( 'NONE',  ( -18.47334320050258327, 24.79293862780133040, -226.9986786077537317 ) ) ;
#4323=CARTESIAN_POINT ( 'NONE',  ( -25.34460520202507539, -7.988444519707189606, -217.6292756219348234 ) ) ;
#4326=CARTESIAN_POINT ( 'NONE',  ( -11.02345917017863464, 29.02019856777526741, -223.9475008740665771 ) ) ;
#4327=CARTESIAN_POINT ( 'NONE',  ( -6.183400735100206269, -24.17720054222102277, -215.4627583112813625 ) ) ;
#4329=CARTESIAN_POINT ( 'NONE',  ( -12.44873260470819787, 7.411970124596155785, -229.4214091473984070 ) ) ;
#4330=CARTESIAN_POINT ( 'NONE',  ( -11.78887577478644566, 1.715692547334320084, -224.3106172711415525 ) ) ;
#4331=CARTESIAN_POINT ( 'NONE',  ( 0.9879969248128627202, 20.02408072508558945, -218.2055348255049410 ) ) ;
#4333=CARTESIAN_POINT ( 'NONE',  ( 23.24653631066306048, 11.83805845626388020, -219.6020901153134162 ) ) ;
#4334=CARTESIAN_POINT ( 'NONE',  ( -12.75670220164522384, -23.12103459569904373, -229.1084755445707799 ) ) ;
#4336=CARTESIAN_POINT ( 'NONE',  ( 10.25948093768852054, 28.38842464930171872, -224.3436940787075855 ) ) ;
#4337=CARTESIAN_POINT ( 'NONE',  ( 1.833772325875588027, 13.50593961039006707, -219.8748197804281119 ) ) ;
#4338=CARTESIAN_POINT ( 'NONE',  ( -9.734169867326336600, 14.53420431798807755, -231.2442251076483046 ) ) ;
#4339=CARTESIAN_POINT ( 'NONE',  ( -16.02921639098982709, -5.689335215210093999, -220.0011032104688979 ) ) ;
#4342=CARTESIAN_POINT ( 'NONE',  ( -16.63766460830045091, 5.158675778507696208, -232.1659425527909093 ) ) ;
#4343=CARTESIAN_POINT ( 'NONE',  ( -13.40300228573463848, -19.05792172404923690, -234.2100255530988306 ) ) ;
#4344=CARTESIAN_POINT ( 'NONE',  ( 22.18132842682159733, 5.591149267797686839, -232.0584733989884114 ) ) ;
#4345=CARTESIAN_POINT ( 'NONE',  ( 4.343013938751969505, 13.02036404005131587, -224.7825435359082178 ) ) ;
#4347=CARTESIAN_POINT ( 'NONE',  ( -16.66929017373293931, 3.065794289431343689, -220.7800282905443794 ) ) ;
#4348=CARTESIAN_POINT ( 'NONE',  ( 9.253342549662157523, 15.33540844142859605, -216.2601104504267937 ) ) ;
#4350=CARTESIAN_POINT ( 'NONE',  ( 22.86997486125673618, 17.56009411325475966, -222.3578648042903296 ) ) ;
#4352=CARTESIAN_POINT ( 'NONE',  ( 24.96598054343045447, -3.653363829669123319, -219.8248103142179559 ) ) ;
#4353=CARTESIAN_POINT ( 'NONE',  ( -19.31342342724724759, -3.870051895940637365, -217.8584481481169348 ) ) ;
#4358=CARTESIAN_POINT ( 'NONE',  ( -8.201407585998298444, 17.38801480109368924, -216.6295241303755006 ) ) ;
#4359=CARTESIAN_POINT ( 'NONE',  ( 15.13468687495441323, -1.603572186776826447, -217.3101985623318626 ) ) ;
#4360=CARTESIAN_POINT ( 'NONE',  ( 14.64930099072384095, -2.233284345536625803, -226.6630761355773984 ) ) ;
#4361=CARTESIAN_POINT ( 'NONE',  ( -25.64868633208605786, 12.30364128039660798, -229.0020209687957049 ) ) ;
#4362=CARTESIAN_POINT ( 'NONE',  ( 9.211411085256067111, 16.86455563410128633, -232.8411836211112700 ) ) ;
#4363=CARTESIAN_POINT ( 'NONE',  ( 20.90058474538433231, 18.60939544422136294, -225.8027644507526475 ) ) ;
#4365=CARTESIAN_POINT ( 'NONE',  ( 3.303203443418958773, -15.45560242990989686, -230.9065799468681917 ) ) ;
#4368=CARTESIAN_POINT ( 'NONE',  ( 4.213939275857851108, 16.79797086795582928, -215.8378124706958943 ) ) ;
#4369=CARTESIAN_POINT ( 'NONE',  ( -4.424820997438546399, 11.84746159238278373, -221.7815792475208525 ) ) ;
#4370=CARTESIAN_POINT ( 'NONE',  ( 15.03150297321239925, -8.313127316319620874, -220.7815108570360394 ) ) ;
#4371=CARTESIAN_POINT ( 'NONE',  ( -0.9414827276148034496, 23.96885519606619752, -216.4491898092606164 ) ) ;
#4374=CARTESIAN_POINT ( 'NONE',  ( 2.631948090663005946, 31.21493676147814611, -222.3107766067421380 ) ) ;
#4375=CARTESIAN_POINT ( 'NONE',  ( -15.94549496081242346, -0.04271059606100771622, -224.7066567765017169 ) ) ;
#4376=CARTESIAN_POINT ( 'NONE',  ( -11.24282496690421596, 12.44430180464951086, -232.4405891940542404 ) ) ;
#4377=CARTESIAN_POINT ( 'NONE',  ( 20.89184612657454920, 5.404957034965973683, -232.0952743654565609 ) ) ;
#4378=CARTESIAN_POINT ( 'NONE',  ( 3.673290835002071653, 15.92545533070904895, -226.4848186297188022 ) ) ;
#4381=CARTESIAN_POINT ( 'NONE',  ( -1.696080206444520844, 14.74162257415073540, -222.2455536759108838 ) ) ;
#4382=CARTESIAN_POINT ( 'NONE',  ( -18.64257584594551531, -16.66392856591270899, -217.1407738418131999 ) ) ;
#4383=CARTESIAN_POINT ( 'NONE',  ( 14.73698509926073186, 4.443590625350892331, -227.4062002049096236 ) ) ;
#4384=CARTESIAN_POINT ( 'NONE',  ( -9.870642741937645681, -28.68889699630894441, -223.8025096038410879 ) ) ;
#4387=CARTESIAN_POINT ( 'NONE',  ( -22.04240660558204823, 19.10355008918698871, -223.9524535985323723 ) ) ;
#4388=CARTESIAN_POINT ( 'NONE',  ( 23.27685575300125720, -16.81362096763192326, -220.1650456318757563 ) ) ;
#4389=CARTESIAN_POINT ( 'NONE',  ( 6.225744896574323839, 14.38227537199079720, -224.8391693295998266 ) ) ;
#4390=CARTESIAN_POINT ( 'NONE',  ( -13.75208518020500748, 5.661250135068270239, -227.6647651141479685 ) ) ;
#4391=CARTESIAN_POINT ( 'NONE',  ( -11.10543627608095285, 3.497967533612860613, -224.1342318769322617 ) ) ;
#4392=CARTESIAN_POINT ( 'NONE',  ( -13.72723917162997154, -9.146515947596070006, -227.8820830806802746 ) ) ;
#4393=B_SPLINE_CURVE_WITH_KNOTS ( 'NONE', 3,
 ( #19986, #871, #11449, #4242, #21340, #18317, #19657, #5935, #17990, #2552, #6043, #2877, #16624, #9436, #16296, #7750, #14620, #21454 ),
 .UNSPECIFIED., .F., .F.,
 ( 4, 2, 2, 2, 2, 2, 2, 2, 4 ),
 ( 2.482325801946720893E-17, 0.0004266872910318495827, 0.0008533745820636743371, 0.001280061873095498983, 0.001706749164127323738, 0.002133436455159148492, 0.002560123746190973246, 0.002986811037222798001, 0.003413498328254622755 ),
 .UNSPECIFIED. ) ;
#4394=CARTESIAN_POINT ( 'NONE',  ( 14.81258087342262364, 2.398747990731791013, -230.9000679928271040 ) ) ;
#4396=CARTESIAN_POINT ( 'NONE',  ( -9.864471611369220128, -7.448779108659549841, -221.8449511945744064 ) ) ;
#4397=CARTESIAN_POINT ( 'NONE',  ( 4.303123380281038024, 17.66787810618728827, -231.9745698734655832 ) ) ;
#4399=CARTESIAN_POINT ( 'NONE',  ( 22.42925200799500729, 5.652256920629083581, -234.0734181799116698 ) ) ;
#4402=CARTESIAN_POINT ( 'NONE',  ( -11.86888352782322897, 15.29489941890347282, -218.1379771575364259 ) ) ;
#4403=CARTESIAN_POINT ( 'NONE',  ( 3.490829917597003895, 11.40812925993816229, -222.8973702487053004 ) ) ;
#4405=CARTESIAN_POINT ( 'NONE',  ( 0.6532050297617689738, -21.40793743009686878, -217.7635283671393722 ) ) ;
#4406=CARTESIAN_POINT ( 'NONE',  ( 0.4703770282364683197, -28.19050476347214484, -228.5103440588500519 ) ) ;
#4407=CARTESIAN_POINT ( 'NONE',  ( 14.73698509926073186, 4.443590625350892331, -227.4062002049096236 ) ) ;
#4408=CARTESIAN_POINT ( 'NONE',  ( 14.68556740487494849, -6.365102927765655672, -229.6664356779805587 ) ) ;
#4409=CARTESIAN_POINT ( 'NONE',  ( -29.22168435891936156, -1.352755938724206519, -225.9547066689444250 ) ) ;
#4410=CARTESIAN_POINT ( 'NONE',  ( -5.279374154171231126, -12.28263746854076466, -222.5283095625445640 ) ) ;
#4411=CARTESIAN_POINT ( 'NONE',  ( 14.02816775221371337, 20.58276248714641810, -218.7180790146936999 ) ) ;
#4413=CARTESIAN_POINT ( 'NONE',  ( 14.65309016725241698, 3.424799466898550637, -221.5217808432381048 ) ) ;
#4414=CARTESIAN_POINT ( 'NONE',  ( 5.169766346882679997, 29.28517558595074988, -221.5178724947562614 ) ) ;
#4415=CARTESIAN_POINT ( 'NONE',  ( -1.158668551263366986, 23.31492692626720853, -219.2372600964201865 ) ) ;
#4416=CARTESIAN_POINT ( 'NONE',  ( 7.144703960786618957, -9.913249271193393497, -228.5244988832443198 ) ) ;
#4419=CARTESIAN_POINT ( 'NONE',  ( 9.798337081649805214, 12.27506320122302697, -218.9346733583377613 ) ) ;
#4420=CARTESIAN_POINT ( 'NONE',  ( -20.29166677327761903, 16.18344358422343632, -220.0060062064338524 ) ) ;
#4421=CARTESIAN_POINT ( 'NONE',  ( -18.04102731735134313, 0.8647102676311391178, -229.4625228093430849 ) ) ;
#4422=CARTESIAN_POINT ( 'NONE',  ( 1.632321987819951969, -14.78074153629778387, -224.5834756332612301 ) ) ;
#4425=CARTESIAN_POINT ( 'NONE',  ( 26.29894631880581812, 12.29609390142961090, -226.3100047295820332 ) ) ;
#4426=CARTESIAN_POINT ( 'NONE',  ( 10.81635663018848525, -11.46278932037511566, -222.6527676248099681 ) ) ;
#4429=CARTESIAN_POINT ( 'NONE',  ( -5.636842872076440081, -13.76003991320737541, -219.7405193562604495 ) ) ;
#4431=CARTESIAN_POINT ( 'NONE',  ( -3.003186468682855104, 15.63968344752823469, -231.5301608670590667 ) ) ;
#4432=CARTESIAN_POINT ( 'NONE',  ( 0.1645309800062008665, 15.56029994314186382, -233.1129172884685943 ) ) ;
#4434=CARTESIAN_POINT ( 'NONE',  ( -17.75316132689678383, 25.03468689048078843, -222.1645193425721061 ) ) ;
#4435=CARTESIAN_POINT ( 'NONE',  ( -19.29805292978571885, -8.785194383212417080, -233.3520286081516133 ) ) ;
#4438=CARTESIAN_POINT ( 'NONE',  ( -10.24288955603410933, 28.30762631303078791, -220.8855665231519083 ) ) ;
#4439=CARTESIAN_POINT ( 'NONE',  ( -6.646164377397596468, -30.92684034042379437, -222.9942643485979374 ) ) ;
#4440=CARTESIAN_POINT ( 'NONE',  ( 15.84759643368428428, -7.142586963752317608, -231.1761396821659673 ) ) ;
#4441=CARTESIAN_POINT ( 'NONE',  ( -14.83974801774860630, 13.71714848582103485, -216.0935642439352762 ) ) ;
#4442=CARTESIAN_POINT ( 'NONE',  ( -30.35034897870229287, 7.696526532841741819, -221.5749790623549416 ) ) ;
#4444=CARTESIAN_POINT ( 'NONE',  ( -1.386728072030569692, 16.52832439466973824, -230.7516952943509807 ) ) ;
#4446=CARTESIAN_POINT ( 'NONE',  ( -17.17981675979428147, 1.478343374046288128, -216.2419730925687418 ) ) ;
#4447=CARTESIAN_POINT ( 'NONE',  ( -7.069738587058329138, -16.45101055981254845, -220.5392980307454138 ) ) ;
#4449=CARTESIAN_POINT ( 'NONE',  ( -11.05032764129755840, 11.65053160594169945, -221.1796278216217218 ) ) ;
#4450=CARTESIAN_POINT ( 'NONE',  ( 7.450672702945051462, 17.42371045663376705, -217.2894981592719432 ) ) ;
#4451=CARTESIAN_POINT ( 'NONE',  ( -5.566280468132954518, 29.91920859341914962, -222.2705790733167817 ) ) ;
#4453=CARTESIAN_POINT ( 'NONE',  ( 26.38334502096500245, -3.352420239867627494, -217.3603908026431384 ) ) ;
#4457=CARTESIAN_POINT ( 'NONE',  ( -27.82842955277035202, 11.70195273568964112, -227.9294339757464911 ) ) ;
#4458=CARTESIAN_POINT ( 'NONE',  ( -20.34211109426514597, -24.21145056749966074, -225.0780941718357724 ) ) ;
#4459=CARTESIAN_POINT ( 'NONE',  ( 28.51464931495100785, 5.422321182929326966, -223.8116416110474347 ) ) ;
#4461=CARTESIAN_POINT ( 'NONE',  ( 22.84140515590350518, 18.29101041979067332, -226.2334522600520472 ) ) ;
#4462=CARTESIAN_POINT ( 'NONE',  ( 14.67485956688574689, -3.005730394301288744, -224.9297226343007594 ) ) ;
#4464=CARTESIAN_POINT ( 'NONE',  ( -19.50431861204945605, -0.7624880359591150736, -219.4666829195064395 ) ) ;
#4465=CARTESIAN_POINT ( 'NONE',  ( 17.04685026979186446, 18.05617612716381970, -216.0910122987878310 ) ) ;
#4466=FILL_AREA_STYLE_COLOUR ( '', #11691 ) ;
#4468=CARTESIAN_POINT ( 'NONE',  ( 17.00168025137501004, 6.212099629982537508, -219.0548246536471595 ) ) ;
#4470=CARTESIAN_POINT ( 'NONE',  ( 21.58416078958130413, -8.344710983103166058, -219.2549068428508861 ) ) ;
#4472=CARTESIAN_POINT ( 'NONE',  ( -18.53787071664277519, -6.556543064843903146, -232.5192140591401824 ) ) ;
#4476=CARTESIAN_POINT ( 'NONE',  ( -1.973645837583506424, 28.78841935349527503, -228.5341874691134763 ) ) ;
#4477=CARTESIAN_POINT ( 'NONE',  ( 15.86371404000427887, -2.776058937659206638, -233.1947532464443213 ) ) ;
#4478=CARTESIAN_POINT ( 'NONE',  ( 14.62702828724412285, -1.994068170757606673, -224.0552340365271959 ) ) ;
#4480=CARTESIAN_POINT ( 'NONE',  ( -20.45797657813638182, 1.164962349958370336, -217.1306074022350572 ) ) ;
#4481=CARTESIAN_POINT ( 'NONE',  ( 28.65393683769942967, 4.398063292302325067, -219.1542358361629965 ) ) ;
#4482=CARTESIAN_POINT ( 'NONE',  ( 10.79895562092076844, 12.01490073542734116, -225.7380208924852809 ) ) ;
#4484=CARTESIAN_POINT ( 'NONE',  ( 3.099569060413221333, -25.61866983817578713, -217.9657659276338677 ) ) ;
#4486=CARTESIAN_POINT ( 'NONE',  ( -12.36382104905844592, -0.1264132474004772688, -228.0034406263598896 ) ) ;
#4487=CARTESIAN_POINT ( 'NONE',  ( -4.154119475380428916, 11.54776298361823095, -227.0876712548254943 ) ) ;
#4488=CARTESIAN_POINT ( 'NONE',  ( 7.587775680576782200, 20.81864918083767435, -235.2547171215352364 ) ) ;
#4489=CARTESIAN_POINT ( 'NONE',  ( 13.37416304104233333, -8.359606308866407431, -226.7674924273047452 ) ) ;
#4490=CARTESIAN_POINT ( 'NONE',  ( -0.3969026096611234511, 20.89748314411456676, -216.3289738411752978 ) ) ;
#4493=CARTESIAN_POINT ( 'NONE',  ( -6.260151855817680300, 29.88549235135308635, -226.8929519981915064 ) ) ;
#4495=CARTESIAN_POINT ( 'NONE',  ( -28.05279008194460744, 4.018900919424986284, -224.6698354068587662 ) ) ;
#4496=CARTESIAN_POINT ( 'NONE',  ( -16.39453490553961856, 20.24836633112041184, -233.1722131570092245 ) ) ;
#4497=CARTESIAN_POINT ( 'NONE',  ( 13.43730899468209294, 8.427513769504761498, -221.4030804848920297 ) ) ;
#4498=CARTESIAN_POINT ( 'NONE',  ( 3.182992543297812560, 16.68308636702302650, -221.9272281984358415 ) ) ;
#4500=CARTESIAN_POINT ( 'NONE',  ( 8.858651440950676914, 22.47383302477780376, -230.7859943773311215 ) ) ;
#4501=CARTESIAN_POINT ( 'NONE',  ( -14.13781561609191328, -15.90667165809925621, -233.6615929499251649 ) ) ;
#4502=CARTESIAN_POINT ( 'NONE',  ( 18.04365516558436866, 6.721233635139160612, -218.4376093631473168 ) ) ;
#4503=CARTESIAN_POINT ( 'NONE',  ( -3.300732473188277005, -24.68991359470437175, -216.3853901891898488 ) ) ;
#4504=CARTESIAN_POINT ( 'NONE',  ( -7.464187997994982560, 14.20693289415472016, -228.8865298551900764 ) ) ;
#4505=CARTESIAN_POINT ( 'NONE',  ( 25.09678678204237201, -16.96620885351193309, -225.7902784465786965 ) ) ;
#4506=CARTESIAN_POINT ( 'NONE',  ( 18.13412043358480474, 12.55378873098427128, -233.2186159706515696 ) ) ;
#4507=CARTESIAN_POINT ( 'NONE',  ( -8.435479365662203577, 14.12888021429238528, -220.5365774424437859 ) ) ;
#4508=CARTESIAN_POINT ( 'NONE',  ( -18.07648963816576781, 14.36622924931724654, -235.1425738388569187 ) ) ;
#4509=CARTESIAN_POINT ( 'NONE',  ( -21.34127571194312623, -5.850660018714998856, -219.1209233896074977 ) ) ;
#4511=CARTESIAN_POINT ( 'NONE',  ( -16.66921372850992000, 0.4301828684420727078, -227.8397539831347842 ) ) ;
#4513=CARTESIAN_POINT ( 'NONE',  ( -24.74482344071061135, -7.641957171360318490, -233.9284114646162891 ) ) ;
#4514=CARTESIAN_POINT ( 'NONE',  ( 2.808299412262623473, 18.06245856371233316, -217.9832661743849656 ) ) ;
#4515=CARTESIAN_POINT ( 'NONE',  ( 29.55842656951424985, 4.785221541509360854, -220.5134865854112718 ) ) ;
#4516=CARTESIAN_POINT ( 'NONE',  ( -9.007976471255481954, 12.60968992764439633, -227.9367755778692981 ) ) ;
#4517=CARTESIAN_POINT ( 'NONE',  ( 3.982203626615636427, 14.63895582687697150, -217.4952312584269123 ) ) ;
#4520=CARTESIAN_POINT ( 'NONE',  ( -3.664580975482237157, -26.87662451849047329, -230.7630177344243236 ) ) ;
#4522=EDGE_LOOP ( 'NONE', ( #7478, #7056, #20532, #1416, #18568 ) ) ;
#4523=CARTESIAN_POINT ( 'NONE',  ( 0.9095753368782393267, -25.50589708844611891, -231.1945442011520697 ) ) ;
#4524=CARTESIAN_POINT ( 'NONE',  ( -27.68973657932738064, 5.930811633061950694, -216.7842770206311513 ) ) ;
#4525=CARTESIAN_POINT ( 'NONE',  ( 13.49882595795384255, -9.201056071450322449, -219.2439763087855908 ) ) ;
#4526=CARTESIAN_POINT ( 'NONE',  ( -26.43144772945995413, -6.745116643720071359, -219.5134289301136050 ) ) ;
#4527=CARTESIAN_POINT ( 'NONE',  ( -11.39823187951283501, -7.998194509987097689, -226.8062974464413912 ) ) ;
#4529=CARTESIAN_POINT ( 'NONE',  ( 9.214796078729456497, 26.59493510027307650, -225.5796848805584318 ) ) ;
#4532=CARTESIAN_POINT ( 'NONE',  ( -13.44241955326339166, 15.88952131657459965, -217.2587743382015901 ) ) ;
#4533=CARTESIAN_POINT ( 'NONE',  ( 5.248230734842167955, 23.54336384919183445, -216.8914391693808739 ) ) ;
#4534=CARTESIAN_POINT ( 'NONE',  ( 8.632180352507942800, 16.83956698119041917, -230.4752415867875186 ) ) ;
#4535=CARTESIAN_POINT ( 'NONE',  ( 17.05764047735875266, -11.29112887239367424, -214.9748062598841898 ) ) ;
#4536=CARTESIAN_POINT ( 'NONE',  ( 16.96779410054824666, 23.69881408353223406, -220.2174342377987841 ) ) ;
#4537=CARTESIAN_POINT ( 'NONE',  ( -17.00819119081011266, 8.904695857470725784, -219.7915043529501133 ) ) ;
#4538=CARTESIAN_POINT ( 'NONE',  ( -25.48569860171343748, 4.299098795181173216, -219.7804659532078801 ) ) ;
#4539=CARTESIAN_POINT ( 'NONE',  ( 3.619268272960482591, -21.10655420957111517, -217.8630709410095108 ) ) ;
#4542=CARTESIAN_POINT ( 'NONE',  ( 14.32085100525799248, 9.220655089380342062, -219.9006227404039464 ) ) ;
#4543=CARTESIAN_POINT ( 'NONE',  ( 15.00179858758994911, -7.185045179863253750, -227.1671253934038077 ) ) ;
#4545=CARTESIAN_POINT ( 'NONE',  ( -8.803769170443210612, -17.82266517633203406, -233.6972128408098683 ) ) ;
#4547=CARTESIAN_POINT ( 'NONE',  ( -4.620781219515533778, 16.99182040716223696, -217.1278208835672672 ) ) ;
#4548=CARTESIAN_POINT ( 'NONE',  ( 3.641537757978871248, 12.43698445400491437, -220.3805014257186485 ) ) ;
#4550=CARTESIAN_POINT ( 'NONE',  ( -3.514547081416551588, 30.38636916157537016, -227.3529586180979436 ) ) ;
#4551=CARTESIAN_POINT ( 'NONE',  ( -22.25980993584449408, -3.522148912989541802, -233.7954546715351398 ) ) ;
#4554=CARTESIAN_POINT ( 'NONE',  ( 3.763426558366607111, 28.60172112197566818, -230.1816715025297526 ) ) ;
#4555=CARTESIAN_POINT ( 'NONE',  ( -4.110806133445755961, -12.94090688063470473, -230.1197724001632992 ) ) ;
#4556=CARTESIAN_POINT ( 'NONE',  ( 15.33694643395292090, -2.540932720676567502, -228.3777194553126435 ) ) ;
#4557=CARTESIAN_POINT ( 'NONE',  ( -9.716674560061926869, 27.56227806819028103, -219.4917914922789919 ) ) ;
#4558=CARTESIAN_POINT ( 'NONE',  ( 14.32363442937021425, 2.978337679677412808, -227.0386046113487453 ) ) ;
#4559=CARTESIAN_POINT ( 'NONE',  ( -4.211886032913159106, 20.62037006687756602, -216.9488349035050305 ) ) ;
#4560=CARTESIAN_POINT ( 'NONE',  ( -16.71711190488355570, 0.6105529133557690002, -230.9511258789794681 ) ) ;
#4561=CARTESIAN_POINT ( 'NONE',  ( 27.30736127486511577, 7.960716467858479639, -228.6121938484450595 ) ) ;
#4562=CARTESIAN_POINT ( 'NONE',  ( -13.78780214743967214, -7.867619234746639378, -226.3818292120506044 ) ) ;
#4565=CARTESIAN_POINT ( 'NONE',  ( -10.30870167223346456, 11.95603877111467561, -228.4123369090513336 ) ) ;
#4566=CARTESIAN_POINT ( 'NONE',  ( 5.359747511823000465, 20.14556701535824601, -232.9094821222151381 ) ) ;
#4567=CARTESIAN_POINT ( 'NONE',  ( -6.127117917506272882, 18.94558806480136681, -232.9763641438055117 ) ) ;
#4568=CARTESIAN_POINT ( 'NONE',  ( 13.37423534347618670, -3.100899090186935325, -222.2483675785374260 ) ) ;
#4571=CARTESIAN_POINT ( 'NONE',  ( -11.24282496690421596, 12.44430180464951086, -232.4405891940542404 ) ) ;
#4572=CARTESIAN_POINT ( 'NONE',  ( -4.241635020808209866, -19.61639137582426429, -216.9458228475819226 ) ) ;
#4573=CARTESIAN_POINT ( 'NONE',  ( 17.07668571305246985, 2.037405138410691485, -219.7626854147787867 ) ) ;
#4574=CARTESIAN_POINT ( 'NONE',  ( 10.50530447320976535, 20.19629329636330084, -217.1354359361034767 ) ) ;
#4577=CARTESIAN_POINT ( 'NONE',  ( -19.18087294808806931, 21.32275554655070593, -230.8558978902391061 ) ) ;
#4578=CARTESIAN_POINT ( 'NONE',  ( 17.66865342763861690, 2.849170916951684784, -230.9175656266857004 ) ) ;
#4580=CARTESIAN_POINT ( 'NONE',  ( 20.58703255433590940, 0.4816031003617209372, -231.9427175861361263 ) ) ;
#4582=CARTESIAN_POINT ( 'NONE',  ( 28.03541074264261113, -3.118360251426135488, -224.4433144283077581 ) ) ;
#4583=CARTESIAN_POINT ( 'NONE',  ( -13.33530847390368024, -5.065163879519744228, -226.5386329521395226 ) ) ;
#4586=CARTESIAN_POINT ( 'NONE',  ( -15.64710113362562183, 25.90300453978063189, -220.8637308366217269 ) ) ;
#4587=CARTESIAN_POINT ( 'NONE',  ( 28.26377063890550190, -1.722554810693586180, -217.1290174754948623 ) ) ;
#4588=CARTESIAN_POINT ( 'NONE',  ( 19.63495056682994289, -4.096126682090319271, -232.1271738766904207 ) ) ;
#4589=CARTESIAN_POINT ( 'NONE',  ( -20.00523085820573499, 3.356386534894876927, -232.9491364426554298 ) ) ;
#4590=CARTESIAN_POINT ( 'NONE',  ( -16.04492519386327487, 1.819644280589142626, -223.4665098021627614 ) ) ;
#4591=CARTESIAN_POINT ( 'NONE',  ( 16.48099188159542194, 16.04875567542346815, -230.8408106201084706 ) ) ;
#4593=CARTESIAN_POINT ( 'NONE',  ( 12.79824285610881063, -25.13061632922516253, -232.1172912921500426 ) ) ;
#4595=CARTESIAN_POINT ( 'NONE',  ( -26.42613204384124259, 13.88327151024443395, -218.2510073314678323 ) ) ;
#4596=CARTESIAN_POINT ( 'NONE',  ( 7.587775680576782200, 20.81864918083767435, -235.2547171215352364 ) ) ;
#4597=CARTESIAN_POINT ( 'NONE',  ( 3.714886539878811789, 12.88803176524806560, -219.5889136906770034 ) ) ;
#4598=CARTESIAN_POINT ( 'NONE',  ( 15.59528062753244804, -5.679035096727840681, -230.0190217829878918 ) ) ;
#4599=CARTESIAN_POINT ( 'NONE',  ( -17.17400284685640344, 24.63223427531467280, -220.6313524368512162 ) ) ;
#4600=CARTESIAN_POINT ( 'NONE',  ( -18.71530386740073126, -0.6857509888707814527, -217.6195632122020527 ) ) ;
#4603=CARTESIAN_POINT ( 'NONE',  ( 5.264801124131998300, 10.54092478143144795, -226.4890466082630098 ) ) ;
#4604=CARTESIAN_POINT ( 'NONE',  ( -18.94444594796027914, 3.458349568010113728, -218.9807021659310635 ) ) ;
#4605=CARTESIAN_POINT ( 'NONE',  ( -14.70651859537745487, 4.211702956367679107, -230.0357207626005334 ) ) ;
#4606=CARTESIAN_POINT ( 'NONE',  ( 28.57344184061583192, 5.631897254180425527, -225.1192013637692355 ) ) ;
#4607=CARTESIAN_POINT ( 'NONE',  ( 3.786538429322381383, 16.06208591393598084, -226.9891439814428793 ) ) ;
#4610=CARTESIAN_POINT ( 'NONE',  ( 10.73846460100926592, 12.62787417135106161, -222.6344468496098159 ) ) ;
#4611=CARTESIAN_POINT ( 'NONE',  ( -12.44777057840899559, -8.577008958641105352, -229.4809580173677830 ) ) ;
#4612=CARTESIAN_POINT ( 'NONE',  ( 14.54149994592679107, 8.070685273005897997, -229.7292930672863349 ) ) ;
#4613=CARTESIAN_POINT ( 'NONE',  ( 4.525470981882147470, -27.64997114140619416, -217.1529231092339103 ) ) ;
#4615=CARTESIAN_POINT ( 'NONE',  ( -14.22255565734842619, 21.32307452572284134, -218.8849463683180261 ) ) ;
#4617=CARTESIAN_POINT ( 'NONE',  ( 16.26147397530412420, -13.20473954510486081, -216.9283256773164794 ) ) ;
#4618=CARTESIAN_POINT ( 'NONE',  ( 9.125049424194871861, 12.37796447639467523, -227.2539065556229332 ) ) ;
#4619=CARTESIAN_POINT ( 'NONE',  ( -14.87932799058895128, 18.71706570923887369, -231.8731726670167745 ) ) ;
#4620=CARTESIAN_POINT ( 'NONE',  ( -22.61701582078733708, 5.416317966792455252, -214.6955127214549748 ) ) ;
#4622=CARTESIAN_POINT ( 'NONE',  ( -15.27576489228250090, -6.235258113955679526, -227.2120396213316553 ) ) ;
#4623=CARTESIAN_POINT ( 'NONE',  ( -19.50431861204945605, -0.7624880359591150736, -219.4666829195064395 ) ) ;
#4625=CARTESIAN_POINT ( 'NONE',  ( -14.44949936980387584, -0.9990553581641278269, -220.3450678990494964 ) ) ;
#4626=CARTESIAN_POINT ( 'NONE',  ( 14.20064147608437821, 14.63411858269657806, -233.6150408276221242 ) ) ;
#4627=CARTESIAN_POINT ( 'NONE',  ( 25.38325563848796662, 11.05100313887457553, -217.8685524735130628 ) ) ;
#4628=CARTESIAN_POINT ( 'NONE',  ( -1.884624261322229266, 13.00421381464247084, -226.7648460381863345 ) ) ;
#4629=CARTESIAN_POINT ( 'NONE',  ( 4.849508625227819003, 24.02665844953846275, -214.9607406399067315 ) ) ;
#4630=B_SPLINE_CURVE_WITH_KNOTS ( 'NONE', 3,
 ( #5807, #16284, #21114, #533, #4230, #9420 ),
 .UNSPECIFIED., .F., .F.,
 ( 4, 2, 4 ),
 ( 0.003413498328254622755, 0.003630484103855696840, 0.003847469879456770925 ),
 .UNSPECIFIED. ) ;
#4631=CARTESIAN_POINT ( 'NONE',  ( 6.833096512853454207, -24.74801519961247465, -219.7405977492105364 ) ) ;
#4633=CARTESIAN_POINT ( 'NONE',  ( 1.268102448827562068, -18.18084990330622830, -231.0699201170278911 ) ) ;
#4634=CARTESIAN_POINT ( 'NONE',  ( -9.924247690135956645, 7.079756654796299564, -222.1205998075789694 ) ) ;
#4635=CARTESIAN_POINT ( 'NONE',  ( 25.46470895113276711, -14.41152162994631070, -228.1811935238409035 ) ) ;
#4636=CARTESIAN_POINT ( 'NONE',  ( 27.83450977899788370, 1.364662819714677511, -230.5442677252456463 ) ) ;
#4637=CARTESIAN_POINT ( 'NONE',  ( -20.11874861854083463, -21.11755179634840474, -229.7504124090357323 ) ) ;
#4638=CARTESIAN_POINT ( 'NONE',  ( 14.19979467405507556, 6.351366891014061267, -230.8614099669030679 ) ) ;
#4640=CARTESIAN_POINT ( 'NONE',  ( -15.72555926117677139, 17.60926865496976745, -217.2114552733360142 ) ) ;
#4641=CARTESIAN_POINT ( 'NONE',  ( 20.54489901492447501, 10.52141067440427591, -216.2005526543161693 ) ) ;
#4642=CARTESIAN_POINT ( 'NONE',  ( 5.343558017910363667, 26.29639771561252459, -218.1010331760174665 ) ) ;
#4643=CARTESIAN_POINT ( 'NONE',  ( 13.88312867625433711, 12.44451767566605760, -217.7066242262208391 ) ) ;
#4644=CARTESIAN_POINT ( 'NONE',  ( 6.910796951316678260, -9.495606915386650471, -226.6778026831113380 ) ) ;
#4645=CARTESIAN_POINT ( 'NONE',  ( 15.91624278015930649, 5.932232821383347954, -217.3600859879243217 ) ) ;
#4646=CARTESIAN_POINT ( 'NONE',  ( -6.581016643627174645, 27.50493254600863935, -230.8763182197739070 ) ) ;
#4647=CARTESIAN_POINT ( 'NONE',  ( -12.58820391453271093, -22.27128923838312247, -218.3899974299303324 ) ) ;
#4650=CARTESIAN_POINT ( 'NONE',  ( 18.04365516558436866, 6.721233635139160612, -218.4376093631473168 ) ) ;
#4651=CARTESIAN_POINT ( 'NONE',  ( 23.68557655437113141, -13.81416892717991551, -227.4080549258873987 ) ) ;
#4653=CARTESIAN_POINT ( 'NONE',  ( -13.88743542672353826, 10.36310385030668613, -230.6144170796622745 ) ) ;
#4654=CARTESIAN_POINT ( 'NONE',  ( -4.670971249126254499, -22.80666086768999890, -234.0323572959307512 ) ) ;
#4655=CARTESIAN_POINT ( 'NONE',  ( 13.19406830060760605, 4.163358546877222288, -228.8532745215267425 ) ) ;
#4656=CARTESIAN_POINT ( 'NONE',  ( 4.966801760238292118, 27.41406605988239420, -216.4490579899774900 ) ) ;
#4658=CARTESIAN_POINT ( 'NONE',  ( -2.958555384449997661, 13.07587799061801093, -222.7767538261418565 ) ) ;
#4659=CARTESIAN_POINT ( 'NONE',  ( -17.04082806826102470, -4.797954729550726327, -217.3726213297937306 ) ) ;
#4662=CARTESIAN_POINT ( 'NONE',  ( -2.772442535524381579, 13.75675912271027457, -228.9770533867650215 ) ) ;
#4663=CARTESIAN_POINT ( 'NONE',  ( -7.876537541093066253, -10.96045937405908965, -230.9151686379251487 ) ) ;
#4664=CARTESIAN_POINT ( 'NONE',  ( 12.02378739738799140, -16.98783239109716092, -233.4545636224233931 ) ) ;
#4665=CARTESIAN_POINT ( 'NONE',  ( 28.36095019830170472, -8.296631283839911220, -225.2861439608085448 ) ) ;
#4666=CARTESIAN_POINT ( 'NONE',  ( -19.94037810645588138, 20.40093185429846656, -220.0593903119159620 ) ) ;
#4667=CARTESIAN_POINT ( 'NONE',  ( 11.00580183749007190, 25.74996642444834904, -225.8602305833924788 ) ) ;
#4668=CARTESIAN_POINT ( 'NONE',  ( -29.88125065636863198, 4.504452993877526623, -226.2048141718237275 ) ) ;
#4669=CARTESIAN_POINT ( 'NONE',  ( -15.00242079508237936, 7.335218745534954898, -232.9526071471669013 ) ) ;
#4670=CARTESIAN_POINT ( 'NONE',  ( -13.11077419447928349, -11.05578789306379406, -228.2719546787038212 ) ) ;
#4671=CARTESIAN_POINT ( 'NONE',  ( -4.583529401292260275, 28.77615850237956607, -226.7744741901706504 ) ) ;
#4672=CARTESIAN_POINT ( 'NONE',  ( 13.10956039622986324, 4.581323766968698585, -221.0328522389722252 ) ) ;
#4673=CARTESIAN_POINT ( 'NONE',  ( 2.471991688031208945, 13.88348721647344419, -230.6707754746932437 ) ) ;
#4674=CARTESIAN_POINT ( 'NONE',  ( 24.64273247744971229, -10.07127014888436278, -217.7281412196979602 ) ) ;
#4677=CARTESIAN_POINT ( 'NONE',  ( -23.49379658590067876, 11.46840048879614393, -217.2519070826072323 ) ) ;
#4678=CARTESIAN_POINT ( 'NONE',  ( -11.17605908769978740, -26.51801958233905765, -230.6004191093659301 ) ) ;
#4679=CARTESIAN_POINT ( 'NONE',  ( 14.63113973005795643, 4.926264598692385199, -222.4866305912601945 ) ) ;
#4680=CARTESIAN_POINT ( 'NONE',  ( 4.656903975822286768, 13.45000048768594780, -227.6722060245555497 ) ) ;
#4684=CARTESIAN_POINT ( 'NONE',  ( -17.20794623181132721, 21.97849129791581291, -217.9187454682870850 ) ) ;
#4686=CARTESIAN_POINT ( 'NONE',  ( 16.10828274231666768, 3.530956590605524692, -220.6574330336208050 ) ) ;
#4689=CARTESIAN_POINT ( 'NONE',  ( -21.08008464085897060, -0.9048411197481797119, -217.0000000010748522 ) ) ;
#4690=CARTESIAN_POINT ( 'NONE',  ( 26.31881739696682843, -8.664992621510689830, -226.4435203923285655 ) ) ;
#4691=CARTESIAN_POINT ( 'NONE',  ( -16.20471097821853235, -2.781505378741172319, -220.1484675126197317 ) ) ;
#4694=CARTESIAN_POINT ( 'NONE',  ( 1.847452069095833593, 15.11597492720254543, -223.6261404253179421 ) ) ;
#4695=CARTESIAN_POINT ( 'NONE',  ( 12.44757525125794118, -27.84495572490402182, -221.5053358145852656 ) ) ;
#4696=CARTESIAN_POINT ( 'NONE',  ( 15.60497028854143764, -26.39208911975253002, -225.8550158017044112 ) ) ;
#4697=CARTESIAN_POINT ( 'NONE',  ( -18.88895772509644644, 1.306698388790553444, -217.6272550812279292 ) ) ;
#4698=CARTESIAN_POINT ( 'NONE',  ( 21.96352831578506937, -0.3315607655626218175, -233.9427286327412787 ) ) ;
#4699=CARTESIAN_POINT ( 'NONE',  ( 27.30736127486511577, 7.960716467858479639, -228.6121938484450595 ) ) ;
#4700=CARTESIAN_POINT ( 'NONE',  ( 2.980115756258533644, -14.12936798750240008, -229.0659090661425807 ) ) ;
#4702=CARTESIAN_POINT ( 'NONE',  ( -31.76239872120898511, 5.177298019713663990, -226.5714959923072342 ) ) ;
#4703=CARTESIAN_POINT ( 'NONE',  ( 12.92410717862594893, 29.37236178718849189, -224.5435071569520744 ) ) ;
#4704=CARTESIAN_POINT ( 'NONE',  ( 3.764125772070460396, 11.78312483992801596, -228.3484643988637970 ) ) ;
#4705=CARTESIAN_POINT ( 'NONE',  ( 22.30453140437255044, -8.121595866981794032, -232.1448055058014575 ) ) ;
#4706=CARTESIAN_POINT ( 'NONE',  ( -11.42613629117093765, 28.09170287990588832, -228.7150250545069241 ) ) ;
#4707=CARTESIAN_POINT ( 'NONE',  ( -15.15434969228324924, 4.423874646950748613, -230.6144467931089821 ) ) ;
#4708=CARTESIAN_POINT ( 'NONE',  ( 14.75291830987536557, 13.43762972591284033, -235.1407057970265839 ) ) ;
#4709=CARTESIAN_POINT ( 'NONE',  ( -15.23792247720107440, 7.806131751461257373, -230.3336101049160902 ) ) ;
#4710=CARTESIAN_POINT ( 'NONE',  ( -11.69688825528096388, 18.63404371591177622, -215.8612738028812714 ) ) ;
#4712=CARTESIAN_POINT ( 'NONE',  ( 3.388180927852674884, 15.71154068801650538, -224.9339660840813053 ) ) ;
#4713=CARTESIAN_POINT ( 'NONE',  ( 27.32546652195855685, -7.354568365469916991, -229.0866163655393279 ) ) ;
#4715=CARTESIAN_POINT ( 'NONE',  ( -23.14980455159086503, 0.3541108476526578785, -217.8785187302087536 ) ) ;
#4716=CARTESIAN_POINT ( 'NONE',  ( 25.33562512631297281, 12.25422971834577268, -228.6777356031426791 ) ) ;
#4717=CARTESIAN_POINT ( 'NONE',  ( -18.40842514464981861, -18.33793064768350334, -230.6214457472987931 ) ) ;
#4719=CARTESIAN_POINT ( 'NONE',  ( -4.142636420702924482, 14.17169704882741321, -225.1666440184957310 ) ) ;
#4721=CARTESIAN_POINT ( 'NONE',  ( 19.66153801111809685, -22.47763448259700780, -224.4992982350615023 ) ) ;
#4723=CARTESIAN_POINT ( 'NONE',  ( 10.49810582199713416, 9.357428619962972149, -224.5466107281195605 ) ) ;
#4724=CARTESIAN_POINT ( 'NONE',  ( -4.170472558179216804, 16.67407401355319152, -230.2690496885289804 ) ) ;
#4725=CARTESIAN_POINT ( 'NONE',  ( -13.17897211815351000, 23.48099580033777301, -217.3415693533541173 ) ) ;
#4727=CARTESIAN_POINT ( 'NONE',  ( -14.91191843134457784, -11.59770670008449756, -219.5316993567479642 ) ) ;
#4729=CARTESIAN_POINT ( 'NONE',  ( 13.85822045549773129, -1.469587484828172919, -226.8778453516271156 ) ) ;
#4733=CARTESIAN_POINT ( 'NONE',  ( -27.49927005802855717, -8.180762508579555004, -232.0193187950690970 ) ) ;
#4734=CARTESIAN_POINT ( 'NONE',  ( 16.96779410054824666, 23.69881408353223406, -220.2174342377987841 ) ) ;
#4735=CARTESIAN_POINT ( 'NONE',  ( -14.59766675578715223, 7.926254675926275972, -222.3706877972550444 ) ) ;
#4736=CARTESIAN_POINT ( 'NONE',  ( 2.804048525646705148, 30.59371477727813726, -220.6614663749232363 ) ) ;
#4737=CARTESIAN_POINT ( 'NONE',  ( 25.02650711521362936, 17.58144575069911042, -223.6165279156031431 ) ) ;
#4739=CARTESIAN_POINT ( 'NONE',  ( -18.06397433365231819, -19.82544507610489859, -216.4780239895989951 ) ) ;
#4740=ORIENTED_EDGE ( 'NONE', *, *, #18322, .F. ) ;
#4741=CARTESIAN_POINT ( 'NONE',  ( -7.972347216402701164, -18.74702622849856937, -232.1058264431568148 ) ) ;
#4742=CARTESIAN_POINT ( 'NONE',  ( -29.65068623107463708, 4.004319520977249525, -231.5200339834770773 ) ) ;
#4743=CARTESIAN_POINT ( 'NONE',  ( 8.332496243628455090, -29.79192972398156769, -226.1452587264855367 ) ) ;
#4744=CARTESIAN_POINT ( 'NONE',  ( -14.93108815068229589, -1.792787290847115633, -227.6165763581034582 ) ) ;
#4745=CARTESIAN_POINT ( 'NONE',  ( -23.10791503177032880, -5.282985115830100220, -217.6364121950018671 ) ) ;
#4746=CARTESIAN_POINT ( 'NONE',  ( 19.61276001257277102, 19.97122404150989894, -229.5162757829903342 ) ) ;
#4748=CARTESIAN_POINT ( 'NONE',  ( -14.64425879132321384, 10.88727730234500868, -217.2315376225554644 ) ) ;
#4749=CARTESIAN_POINT ( 'NONE',  ( 12.79953165872901266, 10.20044330008568778, -230.3912386799665626 ) ) ;
#4750=CARTESIAN_POINT ( 'NONE',  ( -1.249406995060579062, 25.48934319316224162, -216.9406480707515072 ) ) ;
#4751=CARTESIAN_POINT ( 'NONE',  ( 8.645835506124264214, 12.38899589144949687, -223.4673650485651990 ) ) ;
#4752=CARTESIAN_POINT ( 'NONE',  ( 9.191046577198441980, -13.34937224525895161, -233.4761082295262611 ) ) ;
#4754=CARTESIAN_POINT ( 'NONE',  ( -6.496078068315311427, 23.46891392553531119, -233.1042179568201220 ) ) ;
#4755=CARTESIAN_POINT ( 'NONE',  ( -6.266309075335420253, -15.78290365675015572, -230.2363798222519051 ) ) ;
#4756=CARTESIAN_POINT ( 'NONE',  ( -13.65925618638770800, 3.289586759644148817, -222.1579143493116533 ) ) ;
#4760=CARTESIAN_POINT ( 'NONE',  ( 14.22574309452842733, 4.476723532073429546, -225.5862451792618231 ) ) ;
#4761=CARTESIAN_POINT ( 'NONE',  ( 8.625046000483031605, -27.40455649025574303, -220.2318935480384710 ) ) ;
#4762=CARTESIAN_POINT ( 'NONE',  ( -26.02492405343843984, 6.940268742526972900, -218.8798307745116460 ) ) ;
#4763=CARTESIAN_POINT ( 'NONE',  ( 7.163080459435270164, 24.05253566895842354, -232.4475987112033408 ) ) ;
#4764=CARTESIAN_POINT ( 'NONE',  ( -13.22951852716680676, -5.246159916193459338, -223.7538483380451453 ) ) ;
#4765=CARTESIAN_POINT ( 'NONE',  ( 13.16746181015946959, 0.3897807143096829741, -227.1676274388083243 ) ) ;
#4767=CARTESIAN_POINT ( 'NONE',  ( 12.65306858828212810, 29.42930486385247590, -226.3758484992818012 ) ) ;
#4769=CARTESIAN_POINT ( 'NONE',  ( -3.673551555920188783, 29.81207051619892923, -228.8770490300152005 ) ) ;
#4770=CARTESIAN_POINT ( 'NONE',  ( 13.21219219391003818, -8.064832675337259005, -225.0434479037668041 ) ) ;
#4773=CARTESIAN_POINT ( 'NONE',  ( 5.141746912158045468, 22.01688500372448232, -216.6678693612369386 ) ) ;
#4774=CARTESIAN_POINT ( 'NONE',  ( -5.787689185779406387, -30.68964578337966387, -228.1462806397894383 ) ) ;
#4775=CARTESIAN_POINT ( 'NONE',  ( 5.434900225474387447, -11.93567727083262042, -224.7511004068755369 ) ) ;
#4777=CARTESIAN_POINT ( 'NONE',  ( 17.02763684969102798, -14.67205317233652195, -233.2001291093645818 ) ) ;
#4779=CARTESIAN_POINT ( 'NONE',  ( -11.05707385098054729, 9.265475627845670914, -220.9763772784480693 ) ) ;
#4780=CARTESIAN_POINT ( 'NONE',  ( 8.132753622789847370, 14.44084924206385701, -222.7013822740049704 ) ) ;
#4782=CARTESIAN_POINT ( 'NONE',  ( -22.57344584932824105, 14.14390280519600473, -217.2212543695777924 ) ) ;
#4783=CARTESIAN_POINT ( 'NONE',  ( -14.27150057966913721, -8.785576370668652046, -221.5154223125717579 ) ) ;
#4785=CARTESIAN_POINT ( 'NONE',  ( -16.50467377682197423, 21.56569464670658220, -229.9175202103629374 ) ) ;
#4786=CARTESIAN_POINT ( 'NONE',  ( 23.22505041959077232, 19.39625294115234055, -221.5972645870541555 ) ) ;
#4787=CARTESIAN_POINT ( 'NONE',  ( 1.682843645364419993, 12.02583837823347679, -224.9288196625490457 ) ) ;
#4788=CARTESIAN_POINT ( 'NONE',  ( 14.58943670538545412, -3.864781073802256550, -230.4050158740328129 ) ) ;
#4791=CARTESIAN_POINT ( 'NONE',  ( -28.13472254077564116, 12.33996625515159629, -224.9141344439281909 ) ) ;
#4792=CARTESIAN_POINT ( 'NONE',  ( -30.36433721104044992, -10.30696067327809651, -227.5875578433412159 ) ) ;
#4794=CARTESIAN_POINT ( 'NONE',  ( 18.23324537670537993, 23.47692953258263771, -224.8333321331434433 ) ) ;
#4798=CARTESIAN_POINT ( 'NONE',  ( 12.31511859722645852, -8.491226738247512174, -220.9006323875693738 ) ) ;
#4799=CARTESIAN_POINT ( 'NONE',  ( -13.69675006931110417, 3.702342960760605539, -228.0723273272095355 ) ) ;
#4800=CARTESIAN_POINT ( 'NONE',  ( -19.90771709537278156, 23.83218599423810602, -225.0439263757368735 ) ) ;
#4801=CARTESIAN_POINT ( 'NONE',  ( 15.18181359483165949, 6.369295616116027681, -230.7949408486033462 ) ) ;
#4802=( NAMED_UNIT ( * ) SI_UNIT ( $, .STERADIAN. ) SOLID_ANGLE_UNIT ( ) );
#4804=CARTESIAN_POINT ( 'NONE',  ( 28.57344184061583192, 5.631897254180425527, -225.1192013637692355 ) ) ;
#4806=CARTESIAN_POINT ( 'NONE',  ( 27.35305420947085153, -2.513179086165481912, -228.1718430395816881 ) ) ;
#4807=CARTESIAN_POINT ( 'NONE',  ( -15.19144047750087267, -10.24270553329939304, -232.4311702607364793 ) ) ;
#4810=CARTESIAN_POINT ( 'NONE',  ( 0.3355639943343493026, 23.87279439325363128, -218.0067922387550823 ) ) ;
#4811=CARTESIAN_POINT ( 'NONE',  ( 6.264370104348762069, -18.85623240742893714, -216.4903287596617076 ) ) ;
#4812=CARTESIAN_POINT ( 'NONE',  ( 13.36656406724190305, -19.73987914515934960, -233.3798509643240209 ) ) ;
#4814=CARTESIAN_POINT ( 'NONE',  ( -17.14223598032838325, 23.31797360549976261, -226.5771676936548431 ) ) ;
#4815=CARTESIAN_POINT ( 'NONE',  ( -15.99768154740552717, 2.245235659047613908, -226.7015216759272107 ) ) ;
#4816=CARTESIAN_POINT ( 'NONE',  ( 25.18311526135610734, 13.65721788432563955, -224.7326014392022273 ) ) ;
#4819=CARTESIAN_POINT ( 'NONE',  ( -8.126933673790581736, -26.89509779614531126, -227.4795931708183048 ) ) ;
#4821=CARTESIAN_POINT ( 'NONE',  ( -29.65068623107463708, 4.004319520977249525, -231.5200339834770773 ) ) ;
#4822=CARTESIAN_POINT ( 'NONE',  ( 10.61539692146153691, 8.157890242340682718, -227.5705019877536301 ) ) ;
#4823=CARTESIAN_POINT ( 'NONE',  ( 29.72361553920624999, -4.223772423702004453, -224.3921473884441866 ) ) ;
#4824=CARTESIAN_POINT ( 'NONE',  ( 0.9908753270255351575, 13.79205759140780430, -228.0165926715089881 ) ) ;
#4825=CARTESIAN_POINT ( 'NONE',  ( -27.29953305526601426, 11.21644211419729054, -229.3676346105362995 ) ) ;
#4826=CARTESIAN_POINT ( 'NONE',  ( 10.00603923119254723, 9.610873433734882454, -231.2388095806506669 ) ) ;
#4827=CARTESIAN_POINT ( 'NONE',  ( -25.48569860171343748, 4.299098795181173216, -219.7804659532078801 ) ) ;
#4829=CARTESIAN_POINT ( 'NONE',  ( -15.66530208164916260, 23.23467148471576849, -218.1250122661128046 ) ) ;
#4832=CARTESIAN_POINT ( 'NONE',  ( 3.241594727517011609, 27.64703009302456138, -225.5540025036233374 ) ) ;
#4833=CARTESIAN_POINT ( 'NONE',  ( 20.80196158924851701, -7.261721507697286526, -217.3074963141844194 ) ) ;
#4835=CARTESIAN_POINT ( 'NONE',  ( -18.34948365288241590, -1.907751280579004893, -231.5848060246952116 ) ) ;
#4836=CARTESIAN_POINT ( 'NONE',  ( -14.74212732455322161, 0.2624230007780231633, -231.8143822214177874 ) ) ;
#4837=CARTESIAN_POINT ( 'NONE',  ( -11.81856518996410088, -14.35937779267807279, -219.1576658967449305 ) ) ;
#4839=CARTESIAN_POINT ( 'NONE',  ( -4.334015487506815312, 18.19775486192265390, -231.4387392399519285 ) ) ;
#4841=CARTESIAN_POINT ( 'NONE',  ( 5.191785474240024456, -25.78595846473334419, -219.2330600099714673 ) ) ;
#4842=CARTESIAN_POINT ( 'NONE',  ( 13.88312867625433711, 12.44451767566605760, -217.7066242262208391 ) ) ;
#4843=CARTESIAN_POINT ( 'NONE',  ( -6.720912670637915198, 19.69156892798266512, -217.8848069150180891 ) ) ;
#4844=CARTESIAN_POINT ( 'NONE',  ( -7.686214453470440411, 10.71593237010305444, -228.8058998235944159 ) ) ;
#4846=CARTESIAN_POINT ( 'NONE',  ( -27.21693968233852701, -2.213369147249347524, -221.9579181326467392 ) ) ;
#4847=CARTESIAN_POINT ( 'NONE',  ( 17.19674704922021391, 23.07334190050143974, -228.8256488842130238 ) ) ;
#4849=CARTESIAN_POINT ( 'NONE',  ( 14.95834318372430083, -1.617016552789838801, -229.6306532055809271 ) ) ;
#4852=CARTESIAN_POINT ( 'NONE',  ( 26.16486877413895584, -0.2437668799822691745, -230.8325409000573814 ) ) ;
#4853=CARTESIAN_POINT ( 'NONE',  ( 10.49811526528768368, 13.26166588535847701, -217.9009921269571919 ) ) ;
#4854=CARTESIAN_POINT ( 'NONE',  ( -14.20363567091065349, 7.857660128015216294, -223.4151327167956822 ) ) ;
#4855=CARTESIAN_POINT ( 'NONE',  ( 0.8673818989965740300, 28.69424263383094598, -231.7310846804014659 ) ) ;
#4857=CARTESIAN_POINT ( 'NONE',  ( 15.21408433160105034, 3.021350230896802103, -222.3056493717910769 ) ) ;
#4859=CARTESIAN_POINT ( 'NONE',  ( -13.74974073587016576, -14.61773948691506142, -215.3128624239759290 ) ) ;
#4861=CARTESIAN_POINT ( 'NONE',  ( -11.82217545354207644, -11.78227988727524966, -219.0934395369134506 ) ) ;
#4862=CARTESIAN_POINT ( 'NONE',  ( -16.99821283087967672, -0.5135051709387361552, -216.2173766440975555 ) ) ;
#4863=CARTESIAN_POINT ( 'NONE',  ( 5.668262076144046979, -25.28042871382391965, -216.8182873783340483 ) ) ;
#4864=CARTESIAN_POINT ( 'NONE',  ( 13.34086609499694553, -4.728578536804411314, -230.1381470621469134 ) ) ;
#4865=CARTESIAN_POINT ( 'NONE',  ( -22.53818779203657741, -7.663114047788936567, -232.6164956747681458 ) ) ;
#4867=CARTESIAN_POINT ( 'NONE',  ( 13.17768061945195157, 6.810183613937965674, -219.8302315341053657 ) ) ;
#4868=CARTESIAN_POINT ( 'NONE',  ( -27.05172747931452903, 14.36075930490012276, -228.5082213655825853 ) ) ;
#4869=CARTESIAN_POINT ( 'NONE',  ( 20.40268796714816801, 18.65534563792085621, -219.5587498978784993 ) ) ;
#4870=CARTESIAN_POINT ( 'NONE',  ( 10.55627441269396094, 10.31758739525044888, -223.1990319438957613 ) ) ;
#4871=CARTESIAN_POINT ( 'NONE',  ( 8.812670488384366507, 12.21486833790445914, -225.9961634525829197 ) ) ;
#4872=CARTESIAN_POINT ( 'NONE',  ( 25.51806929334465934, -15.64550748320022144, -218.8629450469393589 ) ) ;
#4873=CARTESIAN_POINT ( 'NONE',  ( -10.65640919150578192, 23.79238421564942740, -218.1088542024188826 ) ) ;
#4874=CARTESIAN_POINT ( 'NONE',  ( -24.68906941503829700, 2.445024713909649705, -232.6803430500543755 ) ) ;
#4875=DIRECTION ( 'NONE',  ( -0.9940043559354330149, -0.1093404791528966163, -6.737719923507020479E-14 ) ) ;
#4876=CARTESIAN_POINT ( 'NONE',  ( 15.33737796850231305, 13.57479350230705428, -232.3313557812109025 ) ) ;
#4877=CARTESIAN_POINT ( 'NONE',  ( 14.99967020447171784, -24.16696097797641940, -221.8072564961694297 ) ) ;
#4878=CARTESIAN_POINT ( 'NONE',  ( -12.43544732248594720, 12.69828336922617318, -219.3367909706387877 ) ) ;
#4879=AXIS2_PLACEMENT_3D ( 'NONE', #12519, #1819, #14328 ) ;
#4880=CARTESIAN_POINT ( 'NONE',  ( 5.955271202636533090, 21.50135983300913267, -233.0184468368920534 ) ) ;
#4881=CARTESIAN_POINT ( 'NONE',  ( -20.18470553695442860, -13.13924840112635195, -232.9662461559857718 ) ) ;
#4882=CARTESIAN_POINT ( 'NONE',  ( -26.87016840655871874, 6.086699737350822481, -222.9228935003981746 ) ) ;
#4883=CARTESIAN_POINT ( 'NONE',  ( 8.454338299486085617, 13.28844197278511530, -217.6979371188311632 ) ) ;
#4885=CARTESIAN_POINT ( 'NONE',  ( 0.9046320824004248085, 13.39785254849979701, -226.4815711199935890 ) ) ;
#4886=CARTESIAN_POINT ( 'NONE',  ( 11.63667859525082093, -10.90089931597979600, -224.9413544669828013 ) ) ;
#4887=CARTESIAN_POINT ( 'NONE',  ( 18.43413881788024611, -3.292634616013774274, -216.7808090690139409 ) ) ;
#4889=CARTESIAN_POINT ( 'NONE',  ( 5.169766346882679997, 29.28517558595074988, -221.5178724947562614 ) ) ;
#4890=CARTESIAN_POINT ( 'NONE',  ( -15.25474278246548643, -4.999135024540048988, -232.7276810733381183 ) ) ;
#4891=CARTESIAN_POINT ( 'NONE',  ( -12.11864581566431553, -23.10742878804749978, -232.9192999331436909 ) ) ;
#4892=CARTESIAN_POINT ( 'NONE',  ( 15.60497028854143764, -26.39208911975253002, -225.8550158017044112 ) ) ;
#4893=CARTESIAN_POINT ( 'NONE',  ( -14.98215928292561294, 22.79623052288931362, -230.3289734367122890 ) ) ;
#4894=CARTESIAN_POINT ( 'NONE',  ( 9.132190541728901323, 17.73033835127231939, -219.5524510795130766 ) ) ;
#4895=CARTESIAN_POINT ( 'NONE',  ( -13.10651848559790444, 3.262242204071156948, -224.3513854875720597 ) ) ;
#4896=CARTESIAN_POINT ( 'NONE',  ( -20.80338291456855870, 18.97067006663518995, -230.9007617602332516 ) ) ;
#4897=CARTESIAN_POINT ( 'NONE',  ( -22.39763175122653038, -14.70415172796113623, -221.0757120432126612 ) ) ;
#4900=CARTESIAN_POINT ( 'NONE',  ( -4.879985665934096772, 15.33285679834440174, -220.9402849574511833 ) ) ;
#4901=CARTESIAN_POINT ( 'NONE',  ( 15.91624278015930649, 5.932232821383347954, -217.3600859879243217 ) ) ;
#4902=CARTESIAN_POINT ( 'NONE',  ( 18.99256614858759207, 26.22894869843687715, -224.5811130452664202 ) ) ;
#4903=CARTESIAN_POINT ( 'NONE',  ( 13.93061470302797389, -11.80544459979379646, -217.9389246709861538 ) ) ;
#4906=CARTESIAN_POINT ( 'NONE',  ( -19.25929423112888017, 9.818144317380269825, -216.1837936240308409 ) ) ;
#4907=CARTESIAN_POINT ( 'NONE',  ( -11.89542047990565266, -6.454581786823162304, -219.2692666839191133 ) ) ;
#4909=CARTESIAN_POINT ( 'NONE',  ( 13.61707622192329481, 14.84143455326118932, -217.6958999636067063 ) ) ;
#4911=CARTESIAN_POINT ( 'NONE',  ( 14.34945462593695531, -6.128426910066905542, -229.1128190117150041 ) ) ;
#4913=CARTESIAN_POINT ( 'NONE',  ( -14.68037037322036475, 3.441677802729143920, -220.1396515630443389 ) ) ;
#4916=CARTESIAN_POINT ( 'NONE',  ( -7.812160407601123069, 10.19183344000749081, -223.8148904943605828 ) ) ;
#4917=CARTESIAN_POINT ( 'NONE',  ( 15.92396645628901020, -0.3225394686005420009, -223.0199929375764327 ) ) ;
#4918=CARTESIAN_POINT ( 'NONE',  ( -13.29422863469367577, -26.11207831950312652, -226.3284374130324750 ) ) ;
#4920=CARTESIAN_POINT ( 'NONE',  ( 24.58316096239279602, 5.861425670879941485, -231.3104446318280623 ) ) ;
#4922=CARTESIAN_POINT ( 'NONE',  ( 14.64841443880303373, -15.14843974207636101, -218.3573740752273125 ) ) ;
#4923=CARTESIAN_POINT ( 'NONE',  ( 12.84273949316563801, -2.956482729363947737, -224.4564014745444638 ) ) ;
#4925=CARTESIAN_POINT ( 'NONE',  ( 9.653903571287008489, 19.16609876806546353, -219.1149796918802792 ) ) ;
#4926=CARTESIAN_POINT ( 'NONE',  ( 20.78003164828882632, -23.67023879211220461, -227.8573985392403074 ) ) ;
#4927=CARTESIAN_POINT ( 'NONE',  ( 9.918856707546316542, -11.48950767347732871, -219.9734948840342668 ) ) ;
#4929=CARTESIAN_POINT ( 'NONE',  ( -10.29720673141181209, 11.14783905173092649, -222.8560683878917530 ) ) ;
#4930=CARTESIAN_POINT ( 'NONE',  ( 14.00715608756928532, 4.299235856235253728, -230.2440235370780215 ) ) ;
#4931=CARTESIAN_POINT ( 'NONE',  ( 20.64430047260004031, 12.67811357335941480, -231.0449411089858813 ) ) ;
#4932=VERTEX_POINT ( 'NONE', #19024 ) ;
#4933=CARTESIAN_POINT ( 'NONE',  ( -3.424405916006480144, -18.03457810294644403, -219.2650390415759318 ) ) ;
#4935=CARTESIAN_POINT ( 'NONE',  ( -14.70339349403010942, -0.4153334646997780544, -217.8790668391084466 ) ) ;
#4936=CARTESIAN_POINT ( 'NONE',  ( 9.851209273476317918, 25.48401176094959553, -233.7173763849377792 ) ) ;
#4937=CARTESIAN_POINT ( 'NONE',  ( 10.85023464552735462, -16.86364573545779777, -230.5238403791007045 ) ) ;
#4938=CARTESIAN_POINT ( 'NONE',  ( 12.18657022793382794, 26.76558097653315471, -221.8882195427397335 ) ) ;
#4939=CARTESIAN_POINT ( 'NONE',  ( -19.25929423112888017, 9.818144317380269825, -216.1837936240308409 ) ) ;
#4941=CARTESIAN_POINT ( 'NONE',  ( 10.86206282953156510, 30.27427353967719981, -226.0953027964478110 ) ) ;
#4942=CARTESIAN_POINT ( 'NONE',  ( -25.19195624009214640, 10.50676406307063182, -220.0954552869889937 ) ) ;
#4943=CARTESIAN_POINT ( 'NONE',  ( -3.643097910890548796, 22.16888955197135047, -233.9701981029593298 ) ) ;
#4945=CARTESIAN_POINT ( 'NONE',  ( 1.127544764349826867, -27.89617517048659323, -231.9509945439240823 ) ) ;
#4946=CARTESIAN_POINT ( 'NONE',  ( 25.54997870115619207, -2.097555195297153841, -218.7002440566220400 ) ) ;
#4949=CARTESIAN_POINT ( 'NONE',  ( 25.18785298611088308, 3.974282393449815931, -218.7636041058819956 ) ) ;
#4950=CARTESIAN_POINT ( 'NONE',  ( -16.08069336251900339, -10.46797077187589231, -230.6200287382480383 ) ) ;
#4952=CARTESIAN_POINT ( 'NONE',  ( 1.525817648051120967, -14.82969601928396841, -225.8796824437346515 ) ) ;
#4953=CARTESIAN_POINT ( 'NONE',  ( 19.61276001257277102, 19.97122404150989894, -229.5162757829903342 ) ) ;
#4954=CARTESIAN_POINT ( 'NONE',  ( -4.583529401292260275, 28.77615850237956607, -226.7744741901706504 ) ) ;
#4955=CARTESIAN_POINT ( 'NONE',  ( -6.331039912586185814, 17.62337457105953220, -233.2305561356360499 ) ) ;
#4956=CARTESIAN_POINT ( 'NONE',  ( -18.09422283036245460, -3.216155923901089064, -229.6485988878351918 ) ) ;
#4958=CARTESIAN_POINT ( 'NONE',  ( 17.60676319847677007, 21.31475060840986302, -219.8266339603936785 ) ) ;
#4959=CARTESIAN_POINT ( 'NONE',  ( -15.94549496081242346, -0.04271059606100771622, -224.7066567765017169 ) ) ;
#4960=CARTESIAN_POINT ( 'NONE',  ( -18.94444594796027914, 3.458349568010113728, -218.9807021659310635 ) ) ;
#4963=CARTESIAN_POINT ( 'NONE',  ( -13.58432508418311180, -0.3977623232610293935, -228.1278904906119465 ) ) ;
#4964=CARTESIAN_POINT ( 'NONE',  ( 16.10596270516584028, 24.75152718569329835, -228.9330127594856492 ) ) ;
#4965=CARTESIAN_POINT ( 'NONE',  ( -14.01525440049806193, 8.239250543314939890, -226.5804714421811070 ) ) ;
#4966=CARTESIAN_POINT ( 'NONE',  ( 9.400341091271927851, 28.64465517894215196, -231.0823126271420165 ) ) ;
#4967=CARTESIAN_POINT ( 'NONE',  ( 25.70381634773192658, 10.55338509461953400, -230.3576492130207782 ) ) ;
#4968=EDGE_CURVE ( 'NONE', #8552, #8796, #7346, .T. ) ;
#4969=CARTESIAN_POINT ( 'NONE',  ( -19.52111408301234974, -15.33805657151784985, -234.6553009392178808 ) ) ;
#4971=CARTESIAN_POINT ( 'NONE',  ( -11.24961133108761935, -10.18645864713539950, -228.7780882195199013 ) ) ;
#4973=CARTESIAN_POINT ( 'NONE',  ( -17.58289524052909414, 0.7988212499981205417, -233.9567931471624149 ) ) ;
#4974=CARTESIAN_POINT ( 'NONE',  ( 15.65513449100897780, -26.00057195821942457, -227.4103383097017570 ) ) ;
#4975=CARTESIAN_POINT ( 'NONE',  ( -3.060450601941519189, 13.29454208326677289, -222.0135664617158682 ) ) ;
#4976=CARTESIAN_POINT ( 'NONE',  ( 16.37256825621668099, -5.086412116083368851, -216.7246661941694867 ) ) ;
#4977=CARTESIAN_POINT ( 'NONE',  ( -26.43144772945995413, -6.745116643720071359, -219.5134289301136050 ) ) ;
#4978=CARTESIAN_POINT ( 'NONE',  ( 12.54860906168727652, 6.077542143275485031, -228.1605930327268368 ) ) ;
#4980=CARTESIAN_POINT ( 'NONE',  ( -25.98311979368102342, 15.13734258059737670, -220.6162231662327429 ) ) ;
#4981=CARTESIAN_POINT ( 'NONE',  ( 11.54460987479198053, 9.649171130674412566, -228.7280371210653698 ) ) ;
#4982=CARTESIAN_POINT ( 'NONE',  ( 16.54345861550681107, 19.37554510112122230, -218.2240151908141002 ) ) ;
#4983=CARTESIAN_POINT ( 'NONE',  ( 6.225744896574323839, 14.38227537199079720, -224.8391693295998266 ) ) ;
#4984=CARTESIAN_POINT ( 'NONE',  ( -1.453954827973251929, -30.77017545459721859, -228.2950292831040713 ) ) ;
#4985=CARTESIAN_POINT ( 'NONE',  ( -5.727886109716582297, 15.25217619989539486, -230.5419623196804650 ) ) ;
#4986=CARTESIAN_POINT ( 'NONE',  ( 15.61962121506769385, 4.525360868525488911, -229.0684696061408090 ) ) ;
#4987=CARTESIAN_POINT ( 'NONE',  ( 3.671249956548685578, -18.86103685443826805, -233.0640024924723548 ) ) ;
#4988=CARTESIAN_POINT ( 'NONE',  ( -18.04772061096520375, 5.916925414182395038, -217.8829197293425750 ) ) ;
#4989=CARTESIAN_POINT ( 'NONE',  ( 3.846342036506673612, 16.55327908958690131, -231.1358846258000597 ) ) ;
#4990=CARTESIAN_POINT ( 'NONE',  ( -18.89430729770302975, -12.42271633246521212, -233.2230176520695295 ) ) ;
#4991=CARTESIAN_POINT ( 'NONE',  ( 26.28575214971901630, 3.591103948354015696, -217.0994821834097763 ) ) ;
#4992=CARTESIAN_POINT ( 'NONE',  ( 10.81638188557560731, 14.98959006186633403, -234.2424515599453514 ) ) ;
#4994=CARTESIAN_POINT ( 'NONE',  ( -10.24288955603410933, 28.30762631303078791, -220.8855665231519083 ) ) ;
#4995=CARTESIAN_POINT ( 'NONE',  ( 14.09645999499448088, -9.025099991742237648, -228.8994629750086744 ) ) ;
#4996=CARTESIAN_POINT ( 'NONE',  ( 12.85536293311005451, -7.423602990911125410, -229.4216632760384300 ) ) ;
#4998=CARTESIAN_POINT ( 'NONE',  ( 12.04687593227112430, 27.54339840196571743, -224.6466266724203820 ) ) ;
#4999=CARTESIAN_POINT ( 'NONE',  ( -14.02432777873800518, -4.625777501976016559, -231.5673840409723709 ) ) ;
#5000=CARTESIAN_POINT ( 'NONE',  ( -7.531388159411753769, -21.98719092781708540, -216.0713624712111312 ) ) ;
#5001=CARTESIAN_POINT ( 'NONE',  ( 7.021536848793814123, -14.49751826649810482, -218.4909385705359455 ) ) ;
#5002=CARTESIAN_POINT ( 'NONE',  ( -21.95649697515285581, 20.70968357470995258, -226.9638023349746447 ) ) ;
#5003=CARTESIAN_POINT ( 'NONE',  ( 10.73846460100926592, 12.62787417135106161, -222.6344468496098159 ) ) ;
#5004=CARTESIAN_POINT ( 'NONE',  ( -23.98802705797876200, 19.46654170242919690, -223.5293093576406989 ) ) ;
#5005=CARTESIAN_POINT ( 'NONE',  ( -22.28357709049062407, 7.264818440526320309, -215.3877468064711707 ) ) ;
#5006=CARTESIAN_POINT ( 'NONE',  ( -17.40151406155100844, -6.170051014037699844, -218.8120118016391871 ) ) ;
#5008=CARTESIAN_POINT ( 'NONE',  ( -4.224287562409271501, 29.03635716824519264, -224.1823526280761882 ) ) ;
#5009=CARTESIAN_POINT ( 'NONE',  ( 24.19635128940818447, 10.31396593861802380, -216.9479509989864425 ) ) ;
#5010=CARTESIAN_POINT ( 'NONE',  ( 9.616550234602936342, 9.263684773868845923, -230.4827401731016607 ) ) ;
#5012=CARTESIAN_POINT ( 'NONE',  ( 13.20312407767240614, -7.650902547765872086, -230.0578600405493717 ) ) ;
#5015=CARTESIAN_POINT ( 'NONE',  ( -3.368164009525018265, 19.03203264544105622, -233.5986411977714567 ) ) ;
#5017=CARTESIAN_POINT ( 'NONE',  ( -27.99742768613627319, -7.906662303124995184, -217.4094589651611216 ) ) ;
#5019=CARTESIAN_POINT ( 'NONE',  ( 26.24002132888527328, 11.62331517472360964, -222.5300873157218859 ) ) ;
#5021=CARTESIAN_POINT ( 'NONE',  ( 13.04434844185555420, -10.19049307777131297, -230.8679447648462713 ) ) ;
#5022=CARTESIAN_POINT ( 'NONE',  ( -14.07917727715460821, 7.534853284453274291, -218.6337090155677458 ) ) ;
#5023=CARTESIAN_POINT ( 'NONE',  ( 26.53121369294028042, 10.74560293343441586, -229.2288136770759195 ) ) ;
#5024=CARTESIAN_POINT ( 'NONE',  ( -1.827935560680505445, -14.81092009092713369, -225.7372845858837707 ) ) ;
#5026=CARTESIAN_POINT ( 'NONE',  ( 17.34727976380017722, 4.822939981779328811, -230.8836217450937909 ) ) ;
#5028=CARTESIAN_POINT ( 'NONE',  ( 15.55571562362403704, -22.93410568583619025, -228.9591035895856805 ) ) ;
#5031=CARTESIAN_POINT ( 'NONE',  ( 13.96918721733258195, 14.12724320058294403, -230.4946432816737172 ) ) ;
#5032=CARTESIAN_POINT ( 'NONE',  ( 4.482815116226093188, 26.97722808566452812, -229.2080185206130238 ) ) ;
#5033=CARTESIAN_POINT ( 'NONE',  ( 7.797975340826715396, -14.61189063385648623, -232.7894517818505733 ) ) ;
#5034=CARTESIAN_POINT ( 'NONE',  ( 16.07085865561684201, -17.65509622858733252, -216.6880805489183501 ) ) ;
#5036=CARTESIAN_POINT ( 'NONE',  ( -7.873497077133136735, 15.44270125396616677, -230.2562282217168672 ) ) ;
#5037=CARTESIAN_POINT ( 'NONE',  ( -23.67953786836281083, 9.946055673977088674, -229.5560005648173671 ) ) ;
#5038=CARTESIAN_POINT ( 'NONE',  ( 18.51425713624010427, 11.82474821235740592, -231.3645840199355632 ) ) ;
#5040=CARTESIAN_POINT ( 'NONE',  ( -4.358491045216396742, -15.83376542237952300, -229.0450454480885583 ) ) ;
#5043=CARTESIAN_POINT ( 'NONE',  ( 25.60482246989237609, 8.614967517510873307, -219.3103232513597618 ) ) ;
#5044=CARTESIAN_POINT ( 'NONE',  ( 13.35408364068459619, -22.25650632745845314, -229.3239852056058226 ) ) ;
#5045=CARTESIAN_POINT ( 'NONE',  ( 8.979547488457603421, 23.24376652602565230, -232.6628827740196357 ) ) ;
#5046=CARTESIAN_POINT ( 'NONE',  ( -28.99926036811508467, 3.909990568804979194, -228.9613767892386988 ) ) ;
#5048=CARTESIAN_POINT ( 'NONE',  ( 7.651502705057454889, 16.60422307457919544, -215.4679461133464144 ) ) ;
#5049=CARTESIAN_POINT ( 'NONE',  ( -14.95675039876920032, 11.42095949000369259, -217.2220932760075129 ) ) ;
#5051=CARTESIAN_POINT ( 'NONE',  ( -7.189383125363055349, 14.28512618638020548, -231.7475838278701303 ) ) ;
#5052=CARTESIAN_POINT ( 'NONE',  ( 18.54610009393809023, 0.6523581019769808531, -231.1787333216317677 ) ) ;
#5053=CARTESIAN_POINT ( 'NONE',  ( 8.510712203779903007, -27.79691582975998898, -230.5316902582456180 ) ) ;
#5057=CARTESIAN_POINT ( 'NONE',  ( -26.98548179121306845, 3.096138561569834913, -233.8324893795610251 ) ) ;
#5058=CARTESIAN_POINT ( 'NONE',  ( -8.537495277687638051, -14.12518193842558212, -230.5589415009361858 ) ) ;
#5061=CARTESIAN_POINT ( 'NONE',  ( 7.074707374710634156, -26.72731565888815553, -229.5909540767539738 ) ) ;
#5062=CARTESIAN_POINT ( 'NONE',  ( -20.00523085820573499, 3.356386534894876927, -232.9491364426554298 ) ) ;
#5063=CARTESIAN_POINT ( 'NONE',  ( 2.485733319737138736, 14.76073968410796056, -221.5245536174130905 ) ) ;
#5064=CARTESIAN_POINT ( 'NONE',  ( -11.19105919052231179, 21.17456633634251872, -216.2128528132037957 ) ) ;
#5066=CARTESIAN_POINT ( 'NONE',  ( -27.87965705189043675, -2.801641921304233840, -225.5825458398584260 ) ) ;
#5068=CARTESIAN_POINT ( 'NONE',  ( 18.50911814746675788, 15.92944434255054453, -232.0449215596906072 ) ) ;
#5069=CARTESIAN_POINT ( 'NONE',  ( -16.66921372850992000, 0.4301828684420727078, -227.8397539831347842 ) ) ;
#5070=CARTESIAN_POINT ( 'NONE',  ( -18.41237742040652847, 14.06446039901721790, -216.7469276929859632 ) ) ;
#5072=CARTESIAN_POINT ( 'NONE',  ( 17.24952650401854370, 25.19767938110938843, -224.5319471861414797 ) ) ;
#5073=CARTESIAN_POINT ( 'NONE',  ( -14.47418542577149836, 8.806675964858893479, -228.0010566307936699 ) ) ;
#5074=CARTESIAN_POINT ( 'NONE',  ( 10.22554538262735413, 24.20440706210576209, -215.6176527921760737 ) ) ;
#5075=CARTESIAN_POINT ( 'NONE',  ( 22.44730228620155899, 3.608729811217749717, -232.0798239124179645 ) ) ;
#5076=CARTESIAN_POINT ( 'NONE',  ( -2.916193397327769166, -13.79856165086501107, -222.9033574188488842 ) ) ;
#5078=CARTESIAN_POINT ( 'NONE',  ( -9.225692202065292946, -15.38374647092247116, -218.6784895636799320 ) ) ;
#5079=CARTESIAN_POINT ( 'NONE',  ( -16.13584396029534318, 23.78382729893626646, -231.6788043429177435 ) ) ;
#5080=CARTESIAN_POINT ( 'NONE',  ( 1.752757082432757185, -17.15725705531007250, -232.7539178101738742 ) ) ;
#5081=CARTESIAN_POINT ( 'NONE',  ( -6.855867220396999251, 12.17758473459128332, -220.6375607554995213 ) ) ;
#5082=CARTESIAN_POINT ( 'NONE',  ( 21.68440970896747544, -13.87065835575754846, -215.6285083892243790 ) ) ;
#5083=CARTESIAN_POINT ( 'NONE',  ( -27.85133024402786006, -1.794102530182491773, -229.4204807338591081 ) ) ;
#5084=CARTESIAN_POINT ( 'NONE',  ( 13.64836464229338198, 15.83060743948028737, -232.0893758582176929 ) ) ;
#5085=CARTESIAN_POINT ( 'NONE',  ( -2.993956627714193353, 22.04778837082692178, -231.1741803919495339 ) ) ;
#5086=CARTESIAN_POINT ( 'NONE',  ( 19.70286159681817750, 17.87637900817293612, -218.6154571368943493 ) ) ;
#5088=CARTESIAN_POINT ( 'NONE',  ( 18.23324537670537993, 23.47692953258263771, -224.8333321331434433 ) ) ;
#5089=CARTESIAN_POINT ( 'NONE',  ( 14.29768887814754663, 10.87030385293788548, -231.8067013864770161 ) ) ;
#5090=CARTESIAN_POINT ( 'NONE',  ( -0.2114165566986584699, -18.43750818655219703, -233.9360633499430833 ) ) ;
#5091=CARTESIAN_POINT ( 'NONE',  ( -1.806671251568986669, 13.52068930966770388, -228.3567401718105430 ) ) ;
#5093=CARTESIAN_POINT ( 'NONE',  ( 27.04607490430786854, 4.607450003618843049, -220.3758934308003461 ) ) ;
#5094=CARTESIAN_POINT ( 'NONE',  ( 3.085658278449291192, -27.83354332032029888, -231.5475985764057043 ) ) ;
#5095=CARTESIAN_POINT ( 'NONE',  ( -12.82737030338386219, 8.595865151885988098, -221.6735325378515142 ) ) ;
#5096=CARTESIAN_POINT ( 'NONE',  ( -1.433739110790628102, 17.19322394474796667, -219.1420620387681879 ) ) ;
#5097=CARTESIAN_POINT ( 'NONE',  ( -17.42499862437977853, -18.98713029041037004, -232.7811807006768845 ) ) ;
#5098=CARTESIAN_POINT ( 'NONE',  ( -15.99768154740552717, 2.245235659047613908, -226.7015216759272107 ) ) ;
#5100=CARTESIAN_POINT ( 'NONE',  ( 23.04342321161690776, 14.90264581583150694, -218.4777833225197412 ) ) ;
#5102=CARTESIAN_POINT ( 'NONE',  ( 17.68508104102419409, 23.41266195669770767, -227.5327139115408954 ) ) ;
#5103=CARTESIAN_POINT ( 'NONE',  ( 21.28979032490934031, -14.07620925358629727, -230.4022181401844875 ) ) ;
#5104=CARTESIAN_POINT ( 'NONE',  ( 24.68599888815047194, -16.20242508705913309, -228.6174911781957633 ) ) ;
#5105=CARTESIAN_POINT ( 'NONE',  ( 10.02513374692848913, 18.81568788741115128, -217.1505009242214612 ) ) ;
#5106=CARTESIAN_POINT ( 'NONE',  ( -15.95680269303277221, -1.471987722620473615, -218.5035227479738751 ) ) ;
#5107=CARTESIAN_POINT ( 'NONE',  ( -8.258403559667634397, -29.80786866836635696, -223.3983869762195127 ) ) ;
#5108=CARTESIAN_POINT ( 'NONE',  ( 11.39114332821395692, -8.257479203742953189, -226.5648397932267528 ) ) ;
#5109=CARTESIAN_POINT ( 'NONE',  ( -11.88513743913613752, 17.65694776598872195, -232.6054623148957035 ) ) ;
#5110=CARTESIAN_POINT ( 'NONE',  ( 11.87550186346493497, 14.27797038184677270, -220.2068243228838185 ) ) ;
#5111=CARTESIAN_POINT ( 'NONE',  ( -15.15434969228324924, 4.423874646950748613, -230.6144467931089821 ) ) ;
#5112=CARTESIAN_POINT ( 'NONE',  ( -11.84805200323110164, 5.835720598137266180, -228.2740675967047537 ) ) ;
#5113=CARTESIAN_POINT ( 'NONE',  ( 13.39541376241636783, -3.462025909069690321, -228.4300562622815391 ) ) ;
#5116=CARTESIAN_POINT ( 'NONE',  ( -4.742143146070755932, 15.01230778631049567, -221.4832709320255049 ) ) ;
#5117=CARTESIAN_POINT ( 'NONE',  ( 11.09231067055629616, 7.417581979752235100, -227.5152062457793534 ) ) ;
#5118=CARTESIAN_POINT ( 'NONE',  ( 25.12984891811676036, 19.96069634721137476, -226.7154725927711070 ) ) ;
#5119=CARTESIAN_POINT ( 'NONE',  ( 10.08089751255479527, -9.763210684072014089, -226.4220581413412390 ) ) ;
#5123=CARTESIAN_POINT ( 'NONE',  ( -3.060450601941519189, 13.29454208326677289, -222.0135664617158682 ) ) ;
#5124=CARTESIAN_POINT ( 'NONE',  ( -30.74480097515601074, -10.13586512673612106, -225.7096819839593707 ) ) ;
#5126=CARTESIAN_POINT ( 'NONE',  ( 22.02796522526679723, 16.41909032291435366, -220.1590600991317217 ) ) ;
#5127=CARTESIAN_POINT ( 'NONE',  ( -16.74550766701807447, 3.787526820511904813, -217.9802846976114381 ) ) ;
#5128=CARTESIAN_POINT ( 'NONE',  ( 11.32394539683753720, -15.63383003174572572, -233.0723040138117881 ) ) ;
#5129=CARTESIAN_POINT ( 'NONE',  ( -12.44873260470819787, 7.411970124596155785, -229.4214091473984070 ) ) ;
#5130=CARTESIAN_POINT ( 'NONE',  ( -15.15110768032078070, 3.517015312212880218, -219.5479300368539270 ) ) ;
#5131=CARTESIAN_POINT ( 'NONE',  ( -1.434166139689934338, -16.90223958437590213, -219.9603817157532433 ) ) ;
#5134=EDGE_CURVE ( 'NONE', #2027, #5173, #4393, .T. ) ;
#5137=CARTESIAN_POINT ( 'NONE',  ( 23.84477361619719105, -14.51625201957343592, -224.2863126538025540 ) ) ;
#5138=CARTESIAN_POINT ( 'NONE',  ( 12.80332909036350308, -2.946706566599696320, -225.5941091591410839 ) ) ;
#5140=CARTESIAN_POINT ( 'NONE',  ( 18.90025403853754327, 17.70150481658638952, -229.5234643039372315 ) ) ;
#5141=CARTESIAN_POINT ( 'NONE',  ( 0.9879969248128627202, 20.02408072508558945, -218.2055348255049410 ) ) ;
#5143=CARTESIAN_POINT ( 'NONE',  ( 7.462112298232926655, -14.04285870004232528, -232.2430251799377174 ) ) ;
#5144=CARTESIAN_POINT ( 'NONE',  ( 17.15627899979664051, -18.64955541608202694, -217.1729447097152388 ) ) ;
#5146=CARTESIAN_POINT ( 'NONE',  ( -9.661739055621840322, 20.41227307912577871, -232.0920144483423257 ) ) ;
#5147=CARTESIAN_POINT ( 'NONE',  ( -25.36936018126600345, 11.57160208538938306, -224.9662154788713622 ) ) ;
#5148=CARTESIAN_POINT ( 'NONE',  ( 14.23294950300690331, 6.961167337017927892, -222.0879133937260974 ) ) ;
#5149=CARTESIAN_POINT ( 'NONE',  ( -8.698852260299409167, -27.05211559305675451, -224.0453856107860986 ) ) ;
#5154=CARTESIAN_POINT ( 'NONE',  ( 20.02669998934234741, 11.93441252203826508, -216.7824909737982182 ) ) ;
#5155=CARTESIAN_POINT ( 'NONE',  ( 10.74448773353722686, -20.82765299830942851, -219.2305132457354659 ) ) ;
#5156=CARTESIAN_POINT ( 'NONE',  ( 4.343013938751969505, 13.02036404005131587, -224.7825435359082178 ) ) ;
#5157=CARTESIAN_POINT ( 'NONE',  ( -6.571166997218196748, 12.74865329367398736, -229.9840124400968762 ) ) ;
#5158=CARTESIAN_POINT ( 'NONE',  ( 13.72784977962315267, 2.687686193488206143, -220.8507880271885995 ) ) ;
#5159=CARTESIAN_POINT ( 'NONE',  ( -2.772442535524381579, 13.75675912271027457, -228.9770533867650215 ) ) ;
#5162=CARTESIAN_POINT ( 'NONE',  ( 1.836136847161299990, -12.84546502099244591, -226.1727064218434293 ) ) ;
#5163=CARTESIAN_POINT ( 'NONE',  ( 16.06750045776299629, -1.909440863493336860, -220.4398626676318713 ) ) ;
#5166=CARTESIAN_POINT ( 'NONE',  ( -17.21167111787709914, -1.850592482912338799, -230.8442569545952665 ) ) ;
#5167=CARTESIAN_POINT ( 'NONE',  ( -27.68973657932738064, 5.930811633061950694, -216.7842770206311513 ) ) ;
#5168=CARTESIAN_POINT ( 'NONE',  ( -15.71547198132422984, -24.70787285779005060, -226.7356521228395536 ) ) ;
#5169=CARTESIAN_POINT ( 'NONE',  ( 12.78854151797817451, -25.92021405714643123, -222.0152117995072842 ) ) ;
#5170=CARTESIAN_POINT ( 'NONE',  ( 16.48801037644500056, 3.165716804515234628, -216.8169430726136113 ) ) ;
#5171=CARTESIAN_POINT ( 'NONE',  ( 5.359747511823000465, 20.14556701535824601, -232.9094821222151381 ) ) ;
#5172=CARTESIAN_POINT ( 'NONE',  ( -23.16143087541734502, 21.36835206473086046, -221.8715256527013651 ) ) ;
#5173=VERTEX_POINT ( 'NONE', #3441 ) ;
#5174=CARTESIAN_POINT ( 'NONE',  ( 11.86238739854314872, -1.469869507039519130, -223.6725020993723660 ) ) ;
#5176=CARTESIAN_POINT ( 'NONE',  ( 11.33210854356620523, 22.81476816607802149, -217.8536224460118262 ) ) ;
#5177=CARTESIAN_POINT ( 'NONE',  ( -19.92987771446595957, 11.92619342620000999, -232.5382020162021206 ) ) ;
#5178=CARTESIAN_POINT ( 'NONE',  ( -24.30769394037691100, 17.48612956801762053, -223.4340414801748693 ) ) ;
#5179=CARTESIAN_POINT ( 'NONE',  ( -10.95598939193837928, -18.74794674280272488, -217.4432683290776538 ) ) ;
#5183=CARTESIAN_POINT ( 'NONE',  ( -24.48812334466693486, 4.469247780253509106, -230.3044243311433945 ) ) ;
#5184=CARTESIAN_POINT ( 'NONE',  ( 18.15173157547545557, 23.32481284044927961, -217.8532150843729482 ) ) ;
#5186=CARTESIAN_POINT ( 'NONE',  ( 22.90621760533471019, 17.25363305745006670, -230.8615280072714597 ) ) ;
#5187=CARTESIAN_POINT ( 'NONE',  ( -13.06588638656279322, -26.69120070130052014, -220.2265807429280642 ) ) ;
#5189=CARTESIAN_POINT ( 'NONE',  ( -5.688232406366994454, -14.80527619068227629, -228.6723097085491645 ) ) ;
#5190=CARTESIAN_POINT ( 'NONE',  ( -7.099035520468861549, 19.73710792467281649, -233.8745459908100770 ) ) ;
#5191=CARTESIAN_POINT ( 'NONE',  ( 12.73130673999417795, -23.76414828096303467, -217.7386337832039942 ) ) ;
#5192=CARTESIAN_POINT ( 'NONE',  ( -2.772442535524381579, 13.75675912271027457, -228.9770533867650215 ) ) ;
#5193=CARTESIAN_POINT ( 'NONE',  ( 10.88154471369483112, -8.002597937117323923, -230.2267818776996080 ) ) ;
#5194=CARTESIAN_POINT ( 'NONE',  ( -21.08965452150356867, -10.66825825602615296, -217.1903588586143314 ) ) ;
#5195=CARTESIAN_POINT ( 'NONE',  ( 15.89621445970763070, 6.639162626453350313, -232.5295318698041456 ) ) ;
#5196=CARTESIAN_POINT ( 'NONE',  ( -2.906906946766868227, 27.66682465340607422, -226.6559963821499082 ) ) ;
#5197=CARTESIAN_POINT ( 'NONE',  ( -18.88895772509644644, 1.306698388790553444, -217.6272550812279292 ) ) ;
#5199=CARTESIAN_POINT ( 'NONE',  ( 13.49011766416699842, 7.659170998773840111, -228.1905628957712793 ) ) ;
#5200=CARTESIAN_POINT ( 'NONE',  ( 17.41909632439413969, 2.006477695503792624, -233.4081875040758121 ) ) ;
#5201=CARTESIAN_POINT ( 'NONE',  ( 4.449544252370068342, -12.87211356511098082, -219.5022864574935113 ) ) ;
#5202=CARTESIAN_POINT ( 'NONE',  ( 18.65058977333779211, 24.40868228550881014, -219.3406275662563303 ) ) ;
#5204=CARTESIAN_POINT ( 'NONE',  ( 13.43185000535467211, -22.27464880184020757, -218.9084381759842870 ) ) ;
#5205=CARTESIAN_POINT ( 'NONE',  ( -12.78923236353123727, 15.53885160143439315, -231.8946633672937878 ) ) ;
#5206=CARTESIAN_POINT ( 'NONE',  ( -4.691002462566371101, 21.98518063340150164, -232.2516024630330094 ) ) ;
#5208=CARTESIAN_POINT ( 'NONE',  ( -18.75993824683981970, -9.028840681436806292, -217.1556094966459227 ) ) ;
#5209=CARTESIAN_POINT ( 'NONE',  ( -15.65611835717891687, 5.486779671999271635, -227.0554626315911264 ) ) ;
#5211=CARTESIAN_POINT ( 'NONE',  ( 18.39533937270110187, 14.26564464607222504, -233.9088367426310242 ) ) ;
#5213=CARTESIAN_POINT ( 'NONE',  ( 8.329997790135040603, 12.51216704542961899, -228.7022893680961602 ) ) ;
#5214=CARTESIAN_POINT ( 'NONE',  ( 24.55456120837795808, -10.86188008310946351, -220.0712554825904590 ) ) ;
#5217=CARTESIAN_POINT ( 'NONE',  ( 12.94117841657163126, -3.283311917827119064, -226.8844617769393039 ) ) ;
#5219=CARTESIAN_POINT ( 'NONE',  ( 22.86997486125673618, 17.56009411325475966, -222.3578648042903296 ) ) ;
#5220=CARTESIAN_POINT ( 'NONE',  ( -15.30224200789663946, -6.308083384910589508, -216.9633489813582514 ) ) ;
#5221=CARTESIAN_POINT ( 'NONE',  ( -1.890995374385051608, -13.09686096954197509, -227.5694739903412085 ) ) ;
#5222=CARTESIAN_POINT ( 'NONE',  ( 9.918856707546316542, -11.48950767347732871, -219.9734948840342668 ) ) ;
#5223=CARTESIAN_POINT ( 'NONE',  ( 0.4762409465891800919, 16.20008108839776284, -225.9988706007428050 ) ) ;
#5225=CARTESIAN_POINT ( 'NONE',  ( 14.68130101653174613, 6.427210486143660084, -228.0153742661088074 ) ) ;
#5226=CARTESIAN_POINT ( 'NONE',  ( -13.56774755469388616, 7.311522441667196226, -219.1912666243428021 ) ) ;
#5227=CARTESIAN_POINT ( 'NONE',  ( -3.389634396460917465, 16.42708991135657115, -221.9057377485790994 ) ) ;
#5228=CARTESIAN_POINT ( 'NONE',  ( 18.43413881788024611, -3.292634616013774274, -216.7808090690139409 ) ) ;
#5229=CARTESIAN_POINT ( 'NONE',  ( 2.464084843620814702, 29.35663482419208492, -227.0015060686748143 ) ) ;
#5230=CARTESIAN_POINT ( 'NONE',  ( -17.55809605150417951, 6.636094600389130349, -229.8856864643722986 ) ) ;
#5231=CARTESIAN_POINT ( 'NONE',  ( 10.66732316618037402, 25.78610527446713263, -216.5597036843431624 ) ) ;
#5232=CARTESIAN_POINT ( 'NONE',  ( 5.719431426348611680, -15.09047950350996281, -220.7788505835459318 ) ) ;
#5235=CARTESIAN_POINT ( 'NONE',  ( 1.382955251742491898, 16.46353944795171032, -231.7743150979565030 ) ) ;
#5236=CARTESIAN_POINT ( 'NONE',  ( -8.465184826868526358, -8.692222964613778302, -225.5402182279159149 ) ) ;
#5238=CARTESIAN_POINT ( 'NONE',  ( 25.18785298611088308, 3.974282393449815931, -218.7636041058819956 ) ) ;
#5239=CARTESIAN_POINT ( 'NONE',  ( -20.54164754914381064, 7.122791156791981493, -233.5720402887671980 ) ) ;
#5240=CARTESIAN_POINT ( 'NONE',  ( 17.28140336138120858, -11.48510652344925020, -216.9852223368602893 ) ) ;
#5241=CARTESIAN_POINT ( 'NONE',  ( -29.88125065636863198, 4.504452993877526623, -226.2048141718237275 ) ) ;
#5242=CARTESIAN_POINT ( 'NONE',  ( -14.10849459794400751, -0.2436790717799666162, -223.1085195285415921 ) ) ;
#5243=CARTESIAN_POINT ( 'NONE',  ( -8.652743106909156268, -19.89692808811530966, -232.3032230114403376 ) ) ;
#5246=CARTESIAN_POINT ( 'NONE',  ( -23.49379658590067876, 11.46840048879614393, -217.2519070826072323 ) ) ;
#5247=CARTESIAN_POINT ( 'NONE',  ( 19.11859169356911536, -17.02155004481861411, -230.1485466288596911 ) ) ;
#5252=CARTESIAN_POINT ( 'NONE',  ( 15.99247752609008444, 10.72268246046808216, -230.5614800526110173 ) ) ;
#5253=CARTESIAN_POINT ( 'NONE',  ( -12.22073052649759184, 14.03927388329973525, -215.9097966823721606 ) ) ;
#5254=CARTESIAN_POINT ( 'NONE',  ( 10.90137817157632227, 16.64712710991609868, -230.5401786220292593 ) ) ;
#5255=CARTESIAN_POINT ( 'NONE',  ( -1.044869047506413517, -25.54243019362050404, -231.6194713969048564 ) ) ;
#5256=CARTESIAN_POINT ( 'NONE',  ( 21.04926289057418742, -6.455467962217539934, -215.4677037730695872 ) ) ;
#5258=CARTESIAN_POINT ( 'NONE',  ( -12.87285471141929172, 9.485162256560764504, -229.1865421006261840 ) ) ;
#5259=CARTESIAN_POINT ( 'NONE',  ( -16.51501534778698854, 10.61825396983174485, -230.5082364903317966 ) ) ;
#5260=CARTESIAN_POINT ( 'NONE',  ( -31.04267853410473421, 7.029517189377418873, -226.8060334161593516 ) ) ;
#5261=CARTESIAN_POINT ( 'NONE',  ( -1.494569538902034145, -28.29191435206508487, -228.8702894339512852 ) ) ;
#5264=CARTESIAN_POINT ( 'NONE',  ( 22.90621760533471019, 17.25363305745006670, -230.8615280072714597 ) ) ;
#5265=CARTESIAN_POINT ( 'NONE',  ( 7.764422566766373990, -15.81008911711046672, -220.9836405809557220 ) ) ;
#5266=CARTESIAN_POINT ( 'NONE',  ( 18.23324537670537993, 23.47692953258263771, -224.8333321331434433 ) ) ;
#5267=CARTESIAN_POINT ( 'NONE',  ( -6.201839134465864767, 11.37481922992157379, -223.7040893475979146 ) ) ;
#5268=CARTESIAN_POINT ( 'NONE',  ( 24.19672885113291727, 10.99915907690374439, -233.6834417629405891 ) ) ;
#5269=CARTESIAN_POINT ( 'NONE',  ( 5.331555957413248059, 27.50712867803999728, -219.0801070358024276 ) ) ;
#5270=CARTESIAN_POINT ( 'NONE',  ( 13.43288712491620629, 0.9237972417345811094, -222.1423753579431946 ) ) ;
#5271=CARTESIAN_POINT ( 'NONE',  ( -6.642805165258356404, -28.12267032419628521, -230.9452027245340560 ) ) ;
#5272=CARTESIAN_POINT ( 'NONE',  ( 11.78320976064766690, -8.193118641535518165, -222.2581747538435479 ) ) ;
#5275=CARTESIAN_POINT ( 'NONE',  ( 28.02123297569005089, 5.903198806000402143, -227.5759114383273811 ) ) ;
#5276=CARTESIAN_POINT ( 'NONE',  ( -15.79547310275335725, -3.553268508742920773, -224.0225025563328813 ) ) ;
#5278=CARTESIAN_POINT ( 'NONE',  ( 17.23039831256031817, 3.331158952577910615, -216.4027685342793461 ) ) ;
#5279=CARTESIAN_POINT ( 'NONE',  ( 0.1556102272723409452, 19.71550568250159685, -232.1993058477363547 ) ) ;
#5280=CARTESIAN_POINT ( 'NONE',  ( 2.208705534715813101, 15.26926593729510984, -227.3643075380122980 ) ) ;
#5282=CARTESIAN_POINT ( 'NONE',  ( -25.18517655442826353, -3.313270981248286340, -229.9274946033256697 ) ) ;
#5284=CARTESIAN_POINT ( 'NONE',  ( 17.97843143658897347, 22.12221935793617078, -220.9346589834416079 ) ) ;
#5285=CARTESIAN_POINT ( 'NONE',  ( -16.09559989144903369, 12.31939076846282966, -216.7948290530243298 ) ) ;
#5286=CARTESIAN_POINT ( 'NONE',  ( -14.58670098223046629, 7.239570004716886942, -229.3284954533748135 ) ) ;
#5287=CARTESIAN_POINT ( 'NONE',  ( -15.28220591200235390, -15.65475725988279443, -217.1155325995422913 ) ) ;
#5289=CARTESIAN_POINT ( 'NONE',  ( -14.70651859537745487, 4.211702956367679107, -230.0357207626005334 ) ) ;
#5290=CARTESIAN_POINT ( 'NONE',  ( -22.00000000000137490, -2.602085213965210642E-15, -216.9999999999999716 ) ) ;
#5292=CARTESIAN_POINT ( 'NONE',  ( 21.72366288329714834, 2.385777479048636351, -215.9150265590827757 ) ) ;
#5293=CARTESIAN_POINT ( 'NONE',  ( -9.007976471255481954, 12.60968992764439633, -227.9367755778692981 ) ) ;
#5294=CARTESIAN_POINT ( 'NONE',  ( 8.865150807857233417, 8.939496441981303221, -220.7647208555746090 ) ) ;
#5295=CARTESIAN_POINT ( 'NONE',  ( 21.19180206786061405, -1.472355559550188264, -231.3901500139509722 ) ) ;
#5296=CARTESIAN_POINT ( 'NONE',  ( -29.95626564321166541, -9.027512590954497540, -220.3228832733970819 ) ) ;
#5297=CARTESIAN_POINT ( 'NONE',  ( -24.95227886253013239, -16.82584358170602101, -223.8363818545792299 ) ) ;
#5298=CARTESIAN_POINT ( 'NONE',  ( -16.58369694688956741, 24.75758513462668375, -230.3405478298966784 ) ) ;
#5299=CARTESIAN_POINT ( 'NONE',  ( -1.778254167844783851, -12.78790610364390012, -225.9413532495922254 ) ) ;
#5300=CARTESIAN_POINT ( 'NONE',  ( -6.101488798441174310, 11.33371047077072369, -225.3616985956418546 ) ) ;
#5301=CARTESIAN_POINT ( 'NONE',  ( 12.37876697492742650, -4.127359938151530905, -227.8507160500782618 ) ) ;
#5302=CARTESIAN_POINT ( 'NONE',  ( -28.87859926594958537, -0.8320174534291842061, -222.6356913548140142 ) ) ;
#5303=CARTESIAN_POINT ( 'NONE',  ( -21.28183200535960040, 1.085030287403131233, -217.0000000015322712 ) ) ;
#5305=CARTESIAN_POINT ( 'NONE',  ( -3.125843203957122896, 15.99774916147792680, -222.8808123721668721 ) ) ;
#5306=CARTESIAN_POINT ( 'NONE',  ( 26.75666476377482539, 8.100664119735744961, -232.1611550320539834 ) ) ;
#5307=CARTESIAN_POINT ( 'NONE',  ( 18.46552355142154411, 5.019711608606525211, -231.5099115070375433 ) ) ;
#5308=CARTESIAN_POINT ( 'NONE',  ( 13.71882454279727526, 6.278400000045776252, -230.2269611870541723 ) ) ;
#5309=CARTESIAN_POINT ( 'NONE',  ( 6.571750410407496190, -24.62545695199335682, -234.5391748598602248 ) ) ;
#5310=CARTESIAN_POINT ( 'NONE',  ( 5.030854775705693172, 19.94152319263364603, -234.9034581965229336 ) ) ;
#5311=CARTESIAN_POINT ( 'NONE',  ( 17.34727976380017722, 4.822939981779328811, -230.8836217450937909 ) ) ;
#5312=CARTESIAN_POINT ( 'NONE',  ( -14.63769981573866552, -28.59145599960802642, -226.8825043222271631 ) ) ;
#5313=CARTESIAN_POINT ( 'NONE',  ( -8.435479365662203577, 14.12888021429238528, -220.5365774424437859 ) ) ;
#5314=CARTESIAN_POINT ( 'NONE',  ( 11.01659168199870287, 19.17922986229587323, -233.3715978632214387 ) ) ;
#5315=CARTESIAN_POINT ( 'NONE',  ( -23.10791503177032880, -5.282985115830100220, -217.6364121950018671 ) ) ;
#5316=CARTESIAN_POINT ( 'NONE',  ( -16.51501534778698854, 10.61825396983174485, -230.5082364903317966 ) ) ;
#5318=CARTESIAN_POINT ( 'NONE',  ( -23.89856910807799295, 17.42297078648622843, -222.0178620725767757 ) ) ;
#5319=CARTESIAN_POINT ( 'NONE',  ( 18.84307465506600465, 4.899879697440840509, -218.2189947030338715 ) ) ;
#5321=CARTESIAN_POINT ( 'NONE',  ( 4.484811161826725900, 15.38298568785217313, -219.4617573400562662 ) ) ;
#5322=CARTESIAN_POINT ( 'NONE',  ( 13.59384321027942910, -22.95766697980085169, -228.5239052398278830 ) ) ;
#5324=CARTESIAN_POINT ( 'NONE',  ( 14.41459438711767760, -7.262430563887544821, -219.0449948566021021 ) ) ;
#5325=CARTESIAN_POINT ( 'NONE',  ( -9.106229537879125147, 25.89784491087598184, -228.9807674929363372 ) ) ;
#5327=CARTESIAN_POINT ( 'NONE',  ( 9.107417252317809186, 16.30291009569977234, -218.0131178633739921 ) ) ;
#5328=CARTESIAN_POINT ( 'NONE',  ( -10.70714119831929168, -8.316548062297686172, -219.3892619542279192 ) ) ;
#5329=CARTESIAN_POINT ( 'NONE',  ( -3.300598509645395584, -18.18730530649546395, -233.4303386612170925 ) ) ;
#5330=CARTESIAN_POINT ( 'NONE',  ( -1.643553855084622928, -13.05119293000219294, -222.7191902239112551 ) ) ;
#5331=CARTESIAN_POINT ( 'NONE',  ( 0.04449911090679885967, 16.51968908208873899, -222.9067194156212111 ) ) ;
#5333=CARTESIAN_POINT ( 'NONE',  ( 22.37742875470728876, 11.29804624588327577, -218.9256858961603882 ) ) ;
#5334=CARTESIAN_POINT ( 'NONE',  ( -28.59157645096996347, 5.137867505054540374, -220.4667042235044505 ) ) ;
#5335=CARTESIAN_POINT ( 'NONE',  ( -7.928079932584687128, 26.12067226064367986, -221.2051195461628197 ) ) ;
#5336=CARTESIAN_POINT ( 'NONE',  ( 9.336393807558161839, 27.79372469574263960, -228.5913636680961361 ) ) ;
#5337=CARTESIAN_POINT ( 'NONE',  ( -26.64664107080812627, 5.256684826493772000, -228.0533579629717735 ) ) ;
#5338=CARTESIAN_POINT ( 'NONE',  ( 16.84354851290083133, 10.42424693870724361, -215.2582953371023109 ) ) ;
#5340=CARTESIAN_POINT ( 'NONE',  ( 15.50624253654579654, -15.96056326703506478, -233.0338314371582840 ) ) ;
#5343=CARTESIAN_POINT ( 'NONE',  ( -2.817219543927646175, 14.13981714106644993, -229.6779615865167443 ) ) ;
#5344=CARTESIAN_POINT ( 'NONE',  ( -23.67094103897667523, 1.103242709927489740, -215.1660654633311935 ) ) ;
#5345=CARTESIAN_POINT ( 'NONE',  ( 22.36788034568564854, -2.140002702436959225, -217.7104380410378610 ) ) ;
#5346=CARTESIAN_POINT ( 'NONE',  ( 12.85408565574548412, 7.821283853063205171, -223.1248833997948111 ) ) ;
#5347=CARTESIAN_POINT ( 'NONE',  ( -16.71711190488355570, 0.6105529133557690002, -230.9511258789794681 ) ) ;
#5348=CARTESIAN_POINT ( 'NONE',  ( 15.65513449100897780, -26.00057195821942457, -227.4103383097017570 ) ) ;
#5349=CARTESIAN_POINT ( 'NONE',  ( -14.83974801774860630, 13.71714848582103485, -216.0935642439352762 ) ) ;
#5351=CARTESIAN_POINT ( 'NONE',  ( -25.80904414196669450, 12.19501778665756220, -219.1732313092283846 ) ) ;
#5352=CARTESIAN_POINT ( 'NONE',  ( -16.87231408860552051, -20.68405295654727993, -231.0270656955280515 ) ) ;
#5355=CARTESIAN_POINT ( 'NONE',  ( -20.54164754914381064, 7.122791156791981493, -233.5720402887671980 ) ) ;
#5356=CARTESIAN_POINT ( 'NONE',  ( 15.78601976571614962, -10.64697985159532401, -219.7411765650222151 ) ) ;
#5357=CARTESIAN_POINT ( 'NONE',  ( -28.55814054826834791, -1.660722980825670048, -228.2640858091212408 ) ) ;
#5359=CARTESIAN_POINT ( 'NONE',  ( 14.04819512851487673, 6.831178966487911453, -222.6676118107292552 ) ) ;
#5360=CARTESIAN_POINT ( 'NONE',  ( -8.201407585998298444, 17.38801480109368924, -216.6295241303755006 ) ) ;
#5361=CARTESIAN_POINT ( 'NONE',  ( 25.18311526135610734, 13.65721788432563955, -224.7326014392022273 ) ) ;
#5362=CARTESIAN_POINT ( 'NONE',  ( -0.004649462380863607185, -15.32103018016390017, -221.8331694311728484 ) ) ;
#5363=CARTESIAN_POINT ( 'NONE',  ( 13.04627209130898002, -4.074791396861574988, -220.3858784301183675 ) ) ;
#5365=CARTESIAN_POINT ( 'NONE',  ( -4.130417896617784912, 16.21758012034559826, -229.8171973319304584 ) ) ;
#5366=CARTESIAN_POINT ( 'NONE',  ( -26.35007260221545877, 6.140745174321167177, -221.9336216792591188 ) ) ;
#5367=CARTESIAN_POINT ( 'NONE',  ( 20.62963957373278134, 2.372686805184054837, -232.5966151263358483 ) ) ;
#5368=CARTESIAN_POINT ( 'NONE',  ( -22.93762879021373280, -16.04239672171475206, -226.2337446402420653 ) ) ;
#5371=CARTESIAN_POINT ( 'NONE',  ( 28.62253243811995418, 3.652502539191337494, -225.4068779441649326 ) ) ;
#5372=CARTESIAN_POINT ( 'NONE',  ( 3.608972370552595343, -15.05750810295313435, -224.7555151483228713 ) ) ;
#5373=CARTESIAN_POINT ( 'NONE',  ( 13.61707622192329481, 14.84143455326118932, -217.6958999636067063 ) ) ;
#5374=CARTESIAN_POINT ( 'NONE',  ( -11.69688825528096388, 18.63404371591177622, -215.8612738028812714 ) ) ;
#5376=CARTESIAN_POINT ( 'NONE',  ( 15.65443801613259467, 7.488839228060037989, -233.6469817377710569 ) ) ;
#5377=CARTESIAN_POINT ( 'NONE',  ( 7.769483725421269860, 20.68783433326350263, -233.2348178266662728 ) ) ;
#5378=CARTESIAN_POINT ( 'NONE',  ( 14.01840907662334956, 2.035826308177659083, -222.7954063512536038 ) ) ;
#5379=CARTESIAN_POINT ( 'NONE',  ( 1.799766247726228174, -14.75051420185460849, -230.6199496058247291 ) ) ;
#5380=CARTESIAN_POINT ( 'NONE',  ( 8.785770181087007913, -10.38731345016515917, -223.4272116603623317 ) ) ;
#5382=CARTESIAN_POINT ( 'NONE',  ( -9.045741320599788082, 11.46901338045063312, -219.0588111342715365 ) ) ;
#5383=CARTESIAN_POINT ( 'NONE',  ( -24.91054099106560926, -7.366054470814448862, -220.6971974931307159 ) ) ;
#5384=CARTESIAN_POINT ( 'NONE',  ( 14.55590852435181226, 2.816890518231522034, -218.5131513550309990 ) ) ;
#5385=CARTESIAN_POINT ( 'NONE',  ( 7.450672702945051462, 17.42371045663376705, -217.2894981592719432 ) ) ;
#5386=CARTESIAN_POINT ( 'NONE',  ( -1.470815287892122125, 29.54293232078718745, -224.5855911371830302 ) ) ;
#5388=CARTESIAN_POINT ( 'NONE',  ( 15.19497947618244460, -8.176986896541109218, -234.2449823452919304 ) ) ;
#5390=CARTESIAN_POINT ( 'NONE',  ( 19.72515656911863147, 14.02277373989196541, -218.0718040828188009 ) ) ;
#5391=CARTESIAN_POINT ( 'NONE',  ( -8.929606928624414408, 11.65278034267609186, -219.1999234847403386 ) ) ;
#5392=CARTESIAN_POINT ( 'NONE',  ( -15.10945752141584464, 6.470132813599071220, -220.1568141593501764 ) ) ;
#5393=CARTESIAN_POINT ( 'NONE',  ( -5.688232406366994454, -14.80527619068227629, -228.6723097085491645 ) ) ;
#5398=CARTESIAN_POINT ( 'NONE',  ( 15.91624278015930649, 5.932232821383347954, -217.3600859879243217 ) ) ;
#5399=CARTESIAN_POINT ( 'NONE',  ( -9.222253059793434460, 13.27185325399938165, -229.0864811363590547 ) ) ;
#5400=CARTESIAN_POINT ( 'NONE',  ( 15.51445714770079931, 9.275596138242290678, -215.8565574371285436 ) ) ;
#5401=CARTESIAN_POINT ( 'NONE',  ( -29.95012366401462955, 4.746560250930182967, -224.6954343660969471 ) ) ;
#5402=( BOUNDED_SURFACE ( )  B_SPLINE_SURFACE ( 3, 3, ( 
 ( #7847, #7953, #2864, #14818, #8179, #1413, #11656, #21441, #15044, #21663, #6253, #20185, #4560, #9748, #18415, #9976, #16611, #14935, #21775, #6363, #13235, #4668, #21885, #14606, #5334, #57, #6931, #8623, #1853, #3311, #20300, #15154, #11775, #18853, #12217, #4895, #10196, #8404, #17279, #17172, #5111, #18639, #6591, #20753, #17064, #8285, #22228, #18962, #13579, #10525, #11993, #8731, #18744, #10084, #13460, #17395, #1641, #3428, #15271, #6819, #5226, #10308, #13918, #15598, #8518, #21996, #15381, #177, #10418, #3202, #13685, #7046, #16949, #19069, #22121, #3539, #20522, #5004, #3644, #6708, #1525, #20415, #11881, #1749, #15484, #13802, #20641, #12107, #15713, #7490, #19617, #17617, #5566, #14139, #9180, #15931, #2183, #14359, #17510, #21295, #12444, #20978, #9286, #9064, #15821, #508, #19182, #14025, #5777, #5445, #7159, #12327, #3758, #19294, #21085, #10751, #19504, #11081, #14462, #8847, #2405, #7384, #14252, #16147, #5672, #12550, #719, #5892, #2077, #290, #20862, #4094, #21192, #10643, #12658, #3871, #12769, #16043, #19397, #4202, #1969, #8957, #3980, #10854, #7593, #397, #7270, #17728, #2296, #10970, #17840, #615, #8039, #12981, #21857, #2839, #7925, #13316, #8152, #20157, #14907, #4750, #1052, #19724, #11298, #827, #11186, #21412, #16365, #17948, #15017, #9721, #16583, #18278, #11515, #19828, #7707, #2512, #6002, #6222, #6446, #14576, #4414, #18052, #4642, #4533, #14788, #12874, #16252, #9390, #18169, #4304, #9613, #6337, #942, #2621, #21630, #18385, #6110, #9504, #7819, #14684, #2733, #13098, #21518, #16475, #21747, #19944, #1278, #2948, #11409, #1164, #13210, #9835, #20055, #16697, #20389, #20613, #9952, #3513, #11749, #35, #17040, #8377, #1825, #3176, #16811, #18615, #10393, #17253, #16924, #15568, #8262, #5088, #3063, #17150, #7016, #4982, #15246, #1498, #18830, #3287, #11857, #1727, #4870, #8702, #22092, #6682, #18938, #18722, #10060, #10171, #6561, #1387, #15462, #15129, #21968, #13433, #20275, #13554, #8494, #1616, #6905, #20727, #148, #18502, #12082, #15358, #22205, #13890, #6794, #11629, #13662, #20498, #5199, #11968, #3404, #8601, #10285, #13774, #14439, #8930, #10831, #375, #7243, #14113, #17817, #9039, #2382, #483, #20949, #7133, #2159, #5537, #12526, #8820, #2052, #2270, #7573, #10613, #5417, #17484, #9266, #10945, #19481, #19375, #5307, #10499, #3847, #20835, #3956, #19267, #15905, #16123, #5754, #12415, #17364, #17703, #3731, #12300, #15797, #12189, #19153, #21061, #7358, #16015, #10727, #19044, #697, #5649, #17592, #3620, #14225, #9153, #592, #7465 ),
 ( #1940, #14333, #21167, #12634, #4069, #15685, #263, #13999, #11495, #7799, #21274, #12963, #9700, #4286, #1254, #2711, #21722, #9482, #806, #4182, #8129, #14664, #9594, #5982, #19807, #18257, #16457, #4620, #6315, #21497, #5865, #6087, #13189, #1139, #12746, #4391, #8017, #19593, #20033, #21390, #16560, #11276, #18032, #18363, #12857, #11058, #19699, #2924, #9811, #11165, #16674, #17926, #18145, #11389, #2490, #9370, #13077, #16230, #16342, #1030, #7906, #14881, #7685, #14554, #2601, #14767, #918, #21608, #6200, #2820, #19921, #4508, #1800, #18590, #20472, #10036, #16898, #1473, #5172, #18698, #12054, #10145, #8349, #16789, #11832, #15220, #22179, #18476, #11720, #11941, #17227, #20249, #15107, #4844, #18911, #20586, #6877, #6768, #14995, #20135, #13522, #8238, #13637, #6654, #3261, #3488, #15438, #22065, #4725, #5064, #13406, #21944, #3152, #21834, #6536, #8467, #17014, #3375, #20363, #6423, #10364, #15333, #4955, #13294, #1591, #18805, #10256, #17123, #13749, #11605, #3039, #9925, #1364, #1701, #8573, #8, #15986, #13862, #10585, #453, #20810, #17789, #9124, #19238, #12270, #8904, #7330, #15656, #8676, #21140, #15876, #4038, #15770, #3703, #14307, #19451, #5727, #5386, #563, #9011, #20920, #20702, #12607, #10917, #7106, #7439, #19123, #15540, #236, #123, #5280, #6990, #5509, #19017, #12161, #3594, #10471, #17334, #10701, #1913, #2024, #8795, #10805, #13970, #17455, #17671, #348, #7217, #14082, #19348, #12388, #3818, #17565, #2134, #14198, #21035, #5623, #12501, #3930, #2242, #21246, #18118, #16099, #7879, #20006, #18007, #5954, #14528, #9567, #16316, #2571, #14741, #17899, #21695, #12831, #21362, #9673, #9455, #16204, #892, #19565, #14414, #6169, #5838, #7545, #12718, #4152, #19674, #21470, #11139, #19893, #11467, #14851, #9239, #2790, #7768, #14638, #16532, #6062, #12936, #1111, #6286, #2462, #670, #11032, #4482, #21581, #9345, #13046, #4261, #13160, #16429, #19782, #4591, #2354, #776, #11361, #7656, #4363, #11246, #2685, #1004, #18230, #7986, #16760, #13722, #15415, #10119, #16984, #18674, #11915, #13378, #8101, #2897, #21808, #6626, #22259, #14968, #20220, #18448, #5038, #4931, #15191, #6396, #16645, #8551, #4816, #18336, #10009, #6744, #1339, #20561, #22035, #18781, #6508, #20111, #1227, #5148, #11694, #13497, #3011, #16872, #15307, #20335, #1677, #3347, #18564, #9780, #11807, #3235, #13267, #4699, #6854, #3129, #11574, #1449, #13612, #8210, #9896, #1563, #10230, #8321, #15082, #21918, #8437, #22155, #20449, #17099, #3679, #8992, #7195, #17652, #19329, #5367, #21120, #12251 ),
 ( #8771, #2217, #3575, #17206, #12140, #10784, #3908, #17313, #15966, #8655, #5483, #3464, #17545, #7418, #19102, #15633, #1888, #19216, #10563, #17433, #2113, #5260, #9099, #214, #7083, #539, #2003, #10452, #8885, #6968, #1780, #15855, #15516, #98, #13840, #20678, #13951, #15749, #20786, #7306, #12029, #14286, #18890, #12482, #327, #14062, #10342, #20897, #12367, #18995, #3798, #10682, #431, #14176, #21011, #5601, #10890, #14614, #17877, #8155, #9427, #5928, #21860, #1281, #6449, #21448, #13319, #21334, #16079, #16183, #4014, #7525, #2330, #5814, #5708, #15020, #7742, #6037, #16290, #18090, #9323, #17766, #19430, #9216, #4236, #12585, #12694, #19651, #2439, #648, #21226, #14394, #19541, #4129, #11010, #11116, #4338, #754, #14500, #7630, #12807, #17984, #2546, #865, #12911, #19758, #2952, #11222, #9840, #16701, #19388, #17383, #16033, #499, #5434, #9169, #12951, #7150, #9053, #20852, #12318, #19171, #606, #7258, #7480, #20967, #3748, #5325, #389, #10633, #10742, #7037, #280, #7374, #5767, #8837, #3636, #15703, #14350, #21182, #17719, #17607, #3529, #8721, #2067, #19061, #2174, #17500, #14130, #10409, #3971, #8947, #15588, #15921, #1958, #10517, #14015, #17270, #15813, #19284, #5554, #14242, #12434, #1843, #166, #3861, #21075, #13908, #5663, #12541, #10844, #2284, #20744, #12206, #15207, #9581, #11708, #1125, #22053, #8336, #4832, #2699, #21710, #11591, #9687, #6642, #20237, #8117, #8002, #20020, #18464, #4498, #19795, #10024, #4712, #4378, #4607, #14868, #3141, #11263, #16886, #16547, #18579, #20124, #9796, #16444, #1461, #18132, #18245, #1017, #6302, #7893, #11377, #14754, #18349, #3027, #1243, #21595, #6186, #13282, #13064, #9914, #19909, #13176, #11482, #2911, #16777, #16661, #14982, #1353, #2807, #21822, #6412, #8225, #15096, #21933, #6523, #13393, #9951, #16810, #18384, #13432, #1386, #1496, #20054, #13315, #13553, #18829, #21856, #16695, #6445, #13661, #22204, #8493, #8376, #3402, #21746, #15128, #9834, #15245, #8261, #4869, #5086, #17039, #11628, #6336, #22090, #15016, #1277, #20156, #16582, #8151, #10059, #20273, #4981, #4749, #1163, #11967, #16923, #18500, #8038, #11748, #3175, #18614, #6681, #15357, #20497, #14905, #13209, #6793, #3062, #4641, #11514, #1614, #2947, #21967, #20388, #6560, #11856, #18721, #3285, #10170, #10497, #8929, #17252, #10284, #482, #17483, #5648, #17363, #5306, #15903, #21060, #7357, #7015, #17591, #10612, #262, #15461, #14224, #12525, #8700, #9038, #20726, #19374, #1824, #1726, #8819, #15796, #13998, #17149, #8600, #34, #6903, #13773, #12298 ),
 ( #7242, #12188, #20612, #5197, #13889, #374, #19043, #3619, #1939, #12081, #18937, #15567, #15684, #7132, #3512, #20834, #5416, #2051, #10392, #19152, #14111, #147, #3730, #20948, #5536, #12414, #19266, #2158, #3846, #10726, #9152, #2489, #19479, #11164, #17925, #14553, #14766, #4390, #21273, #16014, #9481, #2381, #4068, #16122, #6199, #10944, #19698, #7684, #14663, #9265, #3955, #21607, #4285, #696, #10830, #21389, #12856, #5981, #2600, #2710, #7905, #13076, #591, #18144, #7572, #17701, #2269, #11275, #7464, #5864, #18031, #14438, #14332, #9593, #16341, #12745, #4181, #917, #17816, #21166, #16456, #7798, #5753, #11057, #19592, #1029, #12633, #9369, #16229, #805, #21496, #6086, #12962, #19806, #22178, #18362, #18697, #8128, #3260, #4619, #11388, #18475, #3151, #1363, #6767, #18256, #19920, #10144, #8466, #21943, #8016, #6422, #10035, #4507, #2819, #11719, #15332, #14994, #3038, #9924, #22064, #9699, #1590, #13188, #15106, #13521, #11494, #17013, #16559, #1138, #6653, #16897, #14880, #1472, #21833, #21721, #4843, #16788, #6314, #20032, #2923, #8348, #9810, #8237, #16673, #13293, #1253, #20134, #4724, #11604, #6535, #13405, #18589, #15219, #20248, #20362, #4954, #11831, #20471, #17122, #1912, #17564, #10255, #8675, #13748, #347, #235, #10470, #1700, #11940, #3817, #122, #13636, #5279, #2023, #18910, #15875, #17333, #14081, #1799, #15437, #18804, #452, #6989, #8794, #20585, #12160, #10584, #15655, #19237, #20919, #13861, #5063, #20701, #5508, #7105, #12387, #13969, #2133, #3374, #10700, #5171, #8903, #19016, #10363, #9010, #12053, #8572, #3487, #7, #6876, #17226, #15539, #3593, #20809, #5385, #19122, #12269, #3702, #17454, #15769, #7216, #21245, #7544, #12830, #562, #4362, #10916, #19450, #14637, #14413, #9238, #11138, #19781, #21361, #18006, #10804, #12500, #17670, #2241, #4037, #4151, #16098, #2570, #16428, #11245, #14197, #7767, #5837, #12717, #21469, #19564, #17898, #6061, #18117, #7438, #19673, #2684, #669, #17788, #2353, #14527, #11031, #2461, #4260, #14306, #9566, #9344, #16203, #12935, #775, #7655, #9454, #7329, #5953, #16315, #9123, #19347, #15985, #21139, #891, #21034, #5622, #3929, #5726, #12606, #7878, #1448, #8100, #14967, #15190, #13266, #11573, #22034, #13496, #1110, #14740, #21580, #3128, #6507, #13045, #13377, #18335, #4930, #8209, #20110, #18673, #20334, #3234, #20219, #10118, #6395, #2789, #16644, #6168, #16531, #4481, #21694, #1003, #11806, #15081, #21917, #1338, #16871, #2896, #19892, #11360, #18229, #18447, #9672, #7985, #9779, #14850, #10008, #9895, #4698 ),
 ( #8320, #11466, #6285, #13159, #20005, #1226, #3010, #4590, #21807, #4815, #16759, #6625, #11693, #18563, #3797, #10341, #8884, #12139, #15748, #20677, #20896, #15306, #326, #17098, #5366, #97, #13721, #7194, #8550, #22154, #1676, #14061, #5482, #22258, #12366, #13611, #10451, #8436, #19215, #16983, #6853, #1562, #20448, #17312, #6743, #213, #5037, #17205, #20560, #5147, #1887, #8654, #1779, #7082, #10229, #11914, #12028, #18889, #2002, #15515, #3463, #20785, #18780, #8770, #12250, #3346, #15414, #6967, #13839, #5259, #18994, #3574, #19101, #15632, #13950, #3678, #17432, #10562, #17765, #2545, #647, #21225, #9426, #864, #10783, #17544, #8991, #12806, #16182, #430, #753, #5707, #14613, #17876, #7524, #6036, #7741, #12910, #7629, #19757, #16078, #12481, #4013, #15854, #3907, #14175, #9098, #10681, #21447, #2438, #9322, #11009, #4235, #12584, #7305, #2112, #21010, #5813, #5600, #19328, #19429, #17651, #19650, #19540, #14393, #2216, #15965, #538, #10889, #7417, #2329, #21333, #14285, #21119, #12693, #11115, #9215, #4128, #14499, #5927, #17983, #16289, #11333, #18311, #1310, #21782, #9982, #11662, #19980, #13466, #4567, #18532, #6369, #3100, #8076, #8292, #2658, #16843, #4451, #15050, #9753, #1085, #1419, #18204, #9540, #2765, #7959, #16508, #11548, #2871, #11442, #9867, #19865, #15160, #14824, #21669, #22003, #16617, #6259, #8184, #6598, #18420, #21891, #7853, #16401, #14719, #21554, #13134, #1199, #14941, #6480, #4337, #11221, #18089, #4787, #13241, #20086, #978, #4673, #2984, #6145, #13019, #9646, #16732, #13349, #20192, #3545, #10090, #10423, #15387, #1973, #5231, #10315, #15718, #10532, #295, #17284, #7163, #3434, #22127, #13691, #3208, #13585, #1532, #18749, #20305, #17399, #12112, #18968, #20648, #13922, #22234, #16955, #4902, #8410, #8629, #8851, #15278, #6825, #20421, #7052, #6938, #17178, #6715, #18645, #11781, #20529, #5010, #12000, #8738, #3319, #11887, #1754, #20757, #8523, #10202, #17069, #1648, #5118, #15489, #18859, #64, #1859, #13808, #3648, #5338, #15604, #182, #12221, #19073, #9185, #5899, #17736, #17954, #12334, #12775, #14146, #2411, #19402, #10757, #4208, #5571, #19187, #20983, #19623, #11087, #19299, #2518, #10648, #7495, #5451, #19512, #9396, #7389, #3876, #834, #14468, #2301, #17622, #14258, #12664, #12448, #14030, #16258, #21197, #20866, #21091, #9069, #3763, #17515, #2083, #2188, #21302, #14364, #3985, #8961, #15825, #402, #15938, #7276, #513, #5677, #12555, #10860, #16048, #4099, #619, #5785, #10977, #17847, #9293, #16154, #725, #7600, #16480, #20368 ),
 ( #13530, #3380, #1057, #11303, #19833, #15225, #21635, #7930, #4959, #948, #5069, #18174, #4421, #15338, #14793, #9618, #11838, #20478, #22069, #18703, #11192, #12880, #18058, #2629, #2738, #4538, #6229, #3266, #17129, #11945, #14583, #8471, #13103, #19949, #22185, #11726, #18594, #6773, #18809, #7824, #21418, #6008, #10150, #17019, #19730, #1594, #3157, #10261, #6659, #10041, #7713, #4310, #9510, #13642, #16371, #16902, #14689, #1478, #21523, #6115, #12986, #8354, #19353, #21039, #15775, #354, #2030, #17570, #19021, #13752, #8579, #5177, #12276, #5628, #20591, #3599, #1804, #15547, #14203, #20927, #10475, #7336, #10810, #5285, #7222, #17340, #1918, #8799, #6883, #3493, #126, #15660, #241, #10369, #20814, #7110, #8909, #12059, #20707, #5514, #3935, #6994, #8681, #13866, #12506, #1705, #15881, #14087, #15443, #18917, #13974, #17233, #12393, #5391, #19128, #13, #2139, #3708, #12165, #19243, #10590, #17460, #3824, #10706, #9016, #459, #21366, #6068, #674, #17677, #13054, #11143, #16103, #2249, #12835, #4265, #19679, #16320, #16433, #21586, #19899, #7444, #9571, #21251, #4487, #6175, #2689, #568, #19569, #9460, #7550, #9129, #18122, #5958, #5843, #17903, #896, #2359, #15992, #7883, #2577, #14311, #2467, #12722, #1008, #21144, #14745, #14418, #5731, #18011, #7662, #12611, #19456, #4044, #4156, #10921, #11037, #17793, #9243, #9349, #16209, #7773, #14643, #781, #14532, #21474, #12940, #19785, #4368, #11252, #20114, #1453, #18235, #20455, #3133, #6749, #21813, #16765, #1344, #13503, #9678, #15313, #4596, #6513, #4936, #13617, #8215, #13165, #4703, #16537, #11472, #14857, #9786, #11366, #8444, #10014, #16878, #11699, #11812, #6402, #1116, #2795, #21700, #21923, #22160, #7992, #13272, #18340, #20340, #20227, #15087, #6291, #20010, #1571, #11580, #2901, #3017, #22043, #16651, #1232, #13383, #18679, #18454, #8106, #14972, #9902, #4822, #18569, #8326, #15196, #6632, #3241, #16990, #10125, #20682, #14181, #5264, #19222, #219, #3802, #8778, #8996, #3354, #10686, #5154, #15753, #10456, #1784, #17550, #18894, #10236, #12034, #2117, #15859, #10347, #436, #1682, #20791, #18786, #10568, #7310, #12144, #8659, #17210, #12255, #19000, #3579, #17438, #20566, #5043, #15520, #103, #12372, #17317, #6974, #8889, #11920, #19106, #332, #8556, #17103, #15420, #22263, #13845, #1893, #15639, #7200, #6858, #13726, #3469, #5488, #7088, #13955, #5371, #3683, #2007, #14066, #20902, #21124, #5605, #19333, #869, #4240, #10789, #11120, #16083, #2662, #5933, #11014, #16406, #11226, #982, #17988, #7857, #19762, #9546 ),
 ( #21018, #17656, #14504, #12486, #2550, #3913, #14398, #2336, #10895, #12811, #12699, #21230, #9434, #14291, #18095, #9220, #17770, #6041, #5820, #652, #16294, #2223, #19655, #7748, #9104, #15971, #545, #7422, #7530, #17882, #19545, #14618, #5712, #12589, #19434, #21452, #4135, #2444, #12916, #9327, #16187, #4342, #4019, #759, #7635, #21338, #16848, #20196, #4457, #4791, #9757, #18651, #21895, #4677, #10095, #4906, #16959, #11666, #1536, #20090, #16512, #8080, #19871, #7963, #18209, #13140, #14723, #11785, #6483, #13353, #15055, #8298, #16622, #11339, #21559, #2770, #2988, #3212, #9651, #1203, #14829, #1424, #1315, #11552, #1089, #13024, #6149, #14948, #21673, #6373, #3104, #19984, #6264, #18424, #15164, #2875, #4571, #11447, #18315, #21786, #9871, #13245, #16737, #18538, #8188, #20310, #22006, #9987, #6602, #13470, #299, #3550, #7169, #12116, #12338, #14034, #187, #10654, #13589, #6942, #1653, #15608, #69, #18971, #19191, #8858, #3439, #20427, #13926, #6830, #8527, #20533, #17520, #15391, #1863, #10427, #19077, #13697, #8414, #3768, #8743, #5123, #15282, #17288, #7058, #20761, #5343, #20870, #22131, #6719, #5015, #5455, #12004, #11891, #18754, #15722, #3323, #10319, #12225, #18863, #10206, #17073, #3652, #17182, #8633, #10536, #22239, #1759, #15493, #17404, #13813, #20652, #5235, #1977, #12884, #21423, #21096, #9400, #2415, #14368, #7280, #6012, #4314, #517, #838, #12560, #7717, #9073, #15830, #624, #7605, #5789, #11197, #406, #2087, #14587, #19734, #4103, #12455, #10865, #14473, #8965, #14150, #16159, #20987, #19406, #7500, #21202, #4212, #5575, #19303, #17626, #19517, #17958, #15941, #3881, #21306, #3989, #10761, #2193, #5681, #5903, #17740, #2305, #9189, #7393, #14263, #16053, #12669, #10981, #17852, #9297, #729, #12779, #19628, #11091, #2523, #16264, #1061, #18178, #7934, #15135, #1394, #9958, #21640, #13441, #6570, #3070, #953, #19954, #9845, #14798, #4876, #18508, #6346, #6234, #18286, #16706, #2742, #18062, #8268, #2959, #20281, #2847, #13107, #21976, #2634, #9514, #4542, #16817, #18394, #8049, #7828, #16374, #14693, #16484, #21528, #11418, #6118, #9622, #12990, #16592, #1286, #21755, #19839, #4425, #11308, #9729, #1174, #20063, #14916, #13218, #8160, #4650, #11524, #15026, #21865, #6455, #13324, #20166, #4760, #11637, #15689, #4986, #6910, #5311, #3291, #1945, #8707, #13666, #17370, #20839, #15363, #17257, #6799, #20502, #5093, #16930, #13561, #10176, #11974, #18835, #20395, #8605, #3409, #18942, #15253, #8498, #15574, #14003, #17045, #11861, #1621, #8824, #267, #3624 ) ),
 .UNSPECIFIED., .T., .F., .F. ) 
 B_SPLINE_SURFACE_WITH_KNOTS ( ( 4, 3, 4 ),
 ( 4, 2, 2, 2, 2, 2, 2, 2, 2, 2, 2, 2, 2, 2, 2, 2, 2, 2, 2, 2, 2, 2, 2, 2, 2, 2, 2, 2, 2, 2, 2, 2, 2, 2, 2, 2, 2, 2, 2, 2, 2, 2, 2, 2, 2, 2, 2, 2, 2, 2, 2, 2, 2, 2, 2, 2, 2, 2, 2, 2, 2, 2, 2, 2, 2, 2, 2, 2, 2, 2, 2, 2, 2, 2, 2, 2, 2, 2, 2, 2, 2, 2, 2, 2, 2, 2, 2, 2, 2, 2, 2, 2, 2, 2, 2, 2, 2, 2, 2, 2, 2, 2, 2, 2, 2, 2, 2, 2, 2, 2, 2, 2, 2, 2, 2, 2, 2, 2, 2, 2, 2, 2, 2, 2, 2, 2, 2, 2, 2, 2, 2, 2, 2, 2, 2, 2, 2, 2, 2, 2, 2, 2, 2, 2, 2, 2, 2, 2, 2, 2, 2, 2, 2, 2, 2, 2, 2, 2, 2, 2, 2, 2, 2, 2, 2, 2, 2, 4 ),
 ( 0.000000000000000000, 0.5000000000000000000, 1.000000000000000000 ),
 ( 0.000000000000000000, 0.001952908952989333875, 0.003905817905978667751, 0.007323408573709997045, 0.01074099924144132634, 0.01415858990917265650, 0.01586738524303832332, 0.01757618057690398666, 0.02099377124463531682, 0.02441136191236664699, 0.02782895258009797368, 0.03124654324782930384, 0.03466413391556063400, 0.03808172458329196070, 0.04149931525102329433, 0.04491690591875462102, 0.04662570125262028436, 0.04833449658648594771, 0.05175208725421727440, 0.05346088258808293775, 0.05516967792194860110, 0.05858726858967993473, 0.06200485925741126836, 0.06542244992514259505, 0.06884004059287393562, 0.07225763126060526231, 0.07567522192833658901, 0.07909281259606792958, 0.08251040326379925627, 0.08421919859766491268, 0.08592799393153058296, 0.08934558459926195129, 0.09276317526699331961, 0.09447197060085900377, 0.09618076593472468794, 0.09959835660245604239, 0.1030159472701873968, 0.1064335379379187652, 0.1098511286056501335, 0.1132687192733815018, 0.1166863099411127869, 0.1201039006088440858, 0.1235214912765753847, 0.1252302866104410273, 0.1269390819443066698, 0.1303566726120379826, 0.1320654679459036251, 0.1337742632797692677, 0.1371918539475005527, 0.1406094446152318378, 0.1440270352829631784, 0.1474446259506944912, 0.1508622166184258040, 0.1542798072861571446, 0.1576973979538884851, 0.1611149886216198257, 0.1645325792893511663, 0.1679501699570824791, 0.1713677606248137919, 0.1747853512925451325, 0.1764941466264108028, 0.1782029419602764730, 0.1816205326280078136, 0.1850381232957391542, 0.1884557139634704670, 0.1918733046312017798, 0.1952908952989331204, 0.1987084859666644610, 0.2021260766343957738, 0.2055436673021270866, 0.2072524626359927569, 0.2089612579698584272, 0.2123788486375897677, 0.2140876439714554380, 0.2157964393053211083, 0.2192140299730524489, 0.2226316206407837617, 0.2260492113085151300, 0.2294668019762464706, 0.2328843926439778111, 0.2363019833117091517, 0.2397195739794404923, 0.2431371646471718329, 0.2465547553149031734, 0.2499723459826345140, 0.2533899366503657991, 0.2568075273180971396, 0.2602251179858284802, 0.2636427086535597653, 0.2670602993212910503, 0.2704778899890223909, 0.2738954806567537315, 0.2773130713244850165, 0.2807306619922163571, 0.2841482526599476977, 0.2858570479938133957, 0.2875658433276790382, 0.2909834339954103788, 0.2926922293292760768, 0.2944010246631417194, 0.2978186153308730599, 0.3012362059986043450, 0.3046537966663356856, 0.3080713873340670261, 0.3114889780017983112, 0.3149065686695296518, 0.3183241593372609923, 0.3217417500049923329, 0.3234505453388579754, 0.3251593406727236735, 0.3285769313404549585, 0.3319945220081862991, 0.3354121126759176397, 0.3388297033436489247, 0.3422472940113802653, 0.3456648846791116059, 0.3490824753468429464, 0.3525000660145742870, 0.3559176566823056276, 0.3593352473500369682, 0.3627528380177683087, 0.3661704286854996493, 0.3695880193532309343, 0.3730056100209622749, 0.3747144053548279174, 0.3764232006886936155, 0.3798407913564249005, 0.3832583820241562411, 0.3866759726918875817, 0.3900935633596189223, 0.3935111540273502628, 0.3969287446950816034, 0.4003463353628129440, 0.4037639260305442845, 0.4054727213644099271, 0.4071815166982756251, 0.4105991073660069102, 0.4140166980337382507, 0.4157254933676038933, 0.4174342887014695913, 0.4208518793692008764, 0.4242694700369322169, 0.4276870607046635575, 0.4311046513723948981, 0.4345222420401262386, 0.4379398327078575237, 0.4413574233755888643, 0.4447750140433202048, 0.4464838093771859029, 0.4481926047110515454, 0.4516101953787828860, 0.4533189907126485840, 0.4550277860465142266, 0.4584453767142455671, 0.4618629673819769077, 0.4652805580497082483, 0.4686981487174395888, 0.4721157393851709294, 0.4755333300529022145, 0.4789509207206335550, 0.4823685113883648956, 0.4840773067222305381, 0.4857861020560961807, 0.4892036927238275212, 0.4926212833915588618, 0.4960388740592901469, 0.4979917830122794764, 0.4999446919652688059 ),
 .UNSPECIFIED. ) 
 GEOMETRIC_REPRESENTATION_ITEM ( )  RATIONAL_B_SPLINE_SURFACE ( (
 ( 1.000000000000000000, 1.000000000000000000, 1.000000000000000000, 1.000000000000000000, 1.000000000000000000, 1.000000000000000000, 1.000000000000000000, 1.000000000000000000, 1.000000000000000000, 1.000000000000000000, 1.000000000000000000, 1.000000000000000000, 1.000000000000000000, 1.000000000000000000, 1.000000000000000000, 1.000000000000000000, 1.000000000000000000, 1.000000000000000000, 1.000000000000000000, 1.000000000000000000, 1.000000000000000000, 1.000000000000000000, 1.000000000000000000, 1.000000000000000000, 1.000000000000000000, 1.000000000000000000, 1.000000000000000000, 1.000000000000000000, 1.000000000000000000, 1.000000000000000000, 1.000000000000000000, 1.000000000000000000, 1.000000000000000000, 1.000000000000000000, 1.000000000000000000, 1.000000000000000000, 1.000000000000000000, 1.000000000000000000, 1.000000000000000000, 1.000000000000000000, 1.000000000000000000, 1.000000000000000000, 1.000000000000000000, 1.000000000000000000, 1.000000000000000000, 1.000000000000000000, 1.000000000000000000, 1.000000000000000000, 1.000000000000000000, 1.000000000000000000, 1.000000000000000000, 1.000000000000000000, 1.000000000000000000, 1.000000000000000000, 1.000000000000000000, 1.000000000000000000, 1.000000000000000000, 1.000000000000000000, 1.000000000000000000, 1.000000000000000000, 1.000000000000000000, 1.000000000000000000, 1.000000000000000000, 1.000000000000000000, 1.000000000000000000, 1.000000000000000000, 1.000000000000000000, 1.000000000000000000, 1.000000000000000000, 1.000000000000000000, 1.000000000000000000, 1.000000000000000000, 1.000000000000000000, 1.000000000000000000, 1.000000000000000000, 1.000000000000000000, 1.000000000000000000, 1.000000000000000000, 1.000000000000000000, 1.000000000000000000, 1.000000000000000000, 1.000000000000000000, 1.000000000000000000, 1.000000000000000000, 1.000000000000000000, 1.000000000000000000, 1.000000000000000000, 1.000000000000000000, 1.000000000000000000, 1.000000000000000000, 1.000000000000000000, 1.000000000000000000, 1.000000000000000000, 1.000000000000000000, 1.000000000000000000, 1.000000000000000000, 1.000000000000000000, 1.000000000000000000, 1.000000000000000000, 1.000000000000000000, 1.000000000000000000, 1.000000000000000000, 1.000000000000000000, 1.000000000000000000, 1.000000000000000000, 1.000000000000000000, 1.000000000000000000, 1.000000000000000000, 1.000000000000000000, 1.000000000000000000, 1.000000000000000000, 1.000000000000000000, 1.000000000000000000, 1.000000000000000000, 1.000000000000000000, 1.000000000000000000, 1.000000000000000000, 1.000000000000000000, 1.000000000000000000, 1.000000000000000000, 1.000000000000000000, 1.000000000000000000, 1.000000000000000000, 1.000000000000000000, 1.000000000000000000, 1.000000000000000000, 1.000000000000000000, 1.000000000000000000, 1.000000000000000000, 1.000000000000000000, 1.000000000000000000, 1.000000000000000000, 1.000000000000000000, 1.000000000000000000, 1.000000000000000000, 1.000000000000000000, 1.000000000000000000, 1.000000000000000000, 1.000000000000000000, 1.000000000000000000, 1.000000000000000000, 1.000000000000000000, 1.000000000000000000, 1.000000000000000000, 1.000000000000000000, 1.000000000000000000, 1.000000000000000000, 1.000000000000000000, 1.000000000000000000, 1.000000000000000000, 1.000000000000000000, 1.000000000000000000, 1.000000000000000000, 1.000000000000000000, 1.000000000000000000, 1.000000000000000000, 1.000000000000000000, 1.000000000000000000, 1.000000000000000000, 1.000000000000000000, 1.000000000000000000, 1.000000000000000000, 1.000000000000000000, 1.000000000000000000, 1.000000000000000000, 1.000000000000000000, 1.000000000000000000, 1.000000000000000000, 1.000000000000000000, 1.000000000000000000, 1.000000000000000000, 1.000000000000000000, 1.000000000000000000, 1.000000000000000000, 1.000000000000000000, 1.000000000000000000, 1.000000000000000000, 1.000000000000000000, 1.000000000000000000, 1.000000000000000000, 1.000000000000000000, 1.000000000000000000, 1.000000000000000000, 1.000000000000000000, 1.000000000000000000, 1.000000000000000000, 1.000000000000000000, 1.000000000000000000, 1.000000000000000000, 1.000000000000000000, 1.000000000000000000, 1.000000000000000000, 1.000000000000000000, 1.000000000000000000, 1.000000000000000000, 1.000000000000000000, 1.000000000000000000, 1.000000000000000000, 1.000000000000000000, 1.000000000000000000, 1.000000000000000000, 1.000000000000000000, 1.000000000000000000, 1.000000000000000000, 1.000000000000000000, 1.000000000000000000, 1.000000000000000000, 1.000000000000000000, 1.000000000000000000, 1.000000000000000000, 1.000000000000000000, 1.000000000000000000, 1.000000000000000000, 1.000000000000000000, 1.000000000000000000, 1.000000000000000000, 1.000000000000000000, 1.000000000000000000, 1.000000000000000000, 1.000000000000000000, 1.000000000000000000, 1.000000000000000000, 1.000000000000000000, 1.000000000000000000, 1.000000000000000000, 1.000000000000000000, 1.000000000000000000, 1.000000000000000000, 1.000000000000000000, 1.000000000000000000, 1.000000000000000000, 1.000000000000000000, 1.000000000000000000, 1.000000000000000000, 1.000000000000000000, 1.000000000000000000, 1.000000000000000000, 1.000000000000000000, 1.000000000000000000, 1.000000000000000000, 1.000000000000000000, 1.000000000000000000, 1.000000000000000000, 1.000000000000000000, 1.000000000000000000, 1.000000000000000000, 1.000000000000000000, 1.000000000000000000, 1.000000000000000000, 1.000000000000000000, 1.000000000000000000, 1.000000000000000000, 1.000000000000000000, 1.000000000000000000, 1.000000000000000000, 1.000000000000000000, 1.000000000000000000, 1.000000000000000000, 1.000000000000000000, 1.000000000000000000, 1.000000000000000000, 1.000000000000000000, 1.000000000000000000, 1.000000000000000000, 1.000000000000000000, 1.000000000000000000, 1.000000000000000000, 1.000000000000000000, 1.000000000000000000, 1.000000000000000000, 1.000000000000000000, 1.000000000000000000, 1.000000000000000000, 1.000000000000000000, 1.000000000000000000, 1.000000000000000000, 1.000000000000000000, 1.000000000000000000, 1.000000000000000000, 1.000000000000000000, 1.000000000000000000, 1.000000000000000000, 1.000000000000000000, 1.000000000000000000, 1.000000000000000000, 1.000000000000000000, 1.000000000000000000, 1.000000000000000000, 1.000000000000000000, 1.000000000000000000, 1.000000000000000000, 1.000000000000000000, 1.000000000000000000, 1.000000000000000000, 1.000000000000000000, 1.000000000000000000, 1.000000000000000000, 1.000000000000000000, 1.000000000000000000, 1.000000000000000000, 1.000000000000000000, 1.000000000000000000, 1.000000000000000000, 1.000000000000000000, 1.000000000000000000, 1.000000000000000000, 1.000000000000000000, 1.000000000000000000, 1.000000000000000000, 1.000000000000000000, 1.000000000000000000, 1.000000000000000000, 1.000000000000000000, 1.000000000000000000, 1.000000000000000000, 1.000000000000000000, 1.000000000000000000, 1.000000000000000000, 1.000000000000000000, 1.000000000000000000, 1.000000000000000000, 1.000000000000000000, 1.000000000000000000, 1.000000000000000000, 1.000000000000000000, 1.000000000000000000, 1.000000000000000000, 1.000000000000000000, 1.000000000000000000, 1.000000000000000000, 1.000000000000000000, 1.000000000000000000, 1.000000000000000000, 1.000000000000000000, 1.000000000000000000, 1.000000000000000000),
 ( 0.3333333333333333703, 0.3333333333333333703, 0.3333333333333333703, 0.3333333333333333703, 0.3333333333333333703, 0.3333333333333333703, 0.3333333333333333703, 0.3333333333333333703, 0.3333333333333333703, 0.3333333333333333703, 0.3333333333333333703, 0.3333333333333333703, 0.3333333333333333703, 0.3333333333333333703, 0.3333333333333333703, 0.3333333333333333703, 0.3333333333333333703, 0.3333333333333333703, 0.3333333333333333703, 0.3333333333333333703, 0.3333333333333333703, 0.3333333333333333703, 0.3333333333333333703, 0.3333333333333333703, 0.3333333333333333703, 0.3333333333333333703, 0.3333333333333333703, 0.3333333333333333703, 0.3333333333333333703, 0.3333333333333333703, 0.3333333333333333703, 0.3333333333333333703, 0.3333333333333333703, 0.3333333333333333703, 0.3333333333333333703, 0.3333333333333333703, 0.3333333333333333703, 0.3333333333333333703, 0.3333333333333333703, 0.3333333333333333703, 0.3333333333333333703, 0.3333333333333333703, 0.3333333333333333703, 0.3333333333333333703, 0.3333333333333333703, 0.3333333333333333703, 0.3333333333333333703, 0.3333333333333333703, 0.3333333333333333703, 0.3333333333333333703, 0.3333333333333333703, 0.3333333333333333703, 0.3333333333333333703, 0.3333333333333333703, 0.3333333333333333703, 0.3333333333333333703, 0.3333333333333333703, 0.3333333333333333703, 0.3333333333333333703, 0.3333333333333333703, 0.3333333333333333703, 0.3333333333333333703, 0.3333333333333333703, 0.3333333333333333703, 0.3333333333333333703, 0.3333333333333333703, 0.3333333333333333703, 0.3333333333333333703, 0.3333333333333333703, 0.3333333333333333703, 0.3333333333333333703, 0.3333333333333333703, 0.3333333333333333703, 0.3333333333333333703, 0.3333333333333333703, 0.3333333333333333703, 0.3333333333333333703, 0.3333333333333333703, 0.3333333333333333703, 0.3333333333333333703, 0.3333333333333333703, 0.3333333333333333703, 0.3333333333333333703, 0.3333333333333333703, 0.3333333333333333703, 0.3333333333333333703, 0.3333333333333333703, 0.3333333333333333703, 0.3333333333333333703, 0.3333333333333333703, 0.3333333333333333703, 0.3333333333333333703, 0.3333333333333333703, 0.3333333333333333703, 0.3333333333333333703, 0.3333333333333333703, 0.3333333333333333703, 0.3333333333333333703, 0.3333333333333333703, 0.3333333333333333703, 0.3333333333333333703, 0.3333333333333333703, 0.3333333333333333703, 0.3333333333333333703, 0.3333333333333333703, 0.3333333333333333703, 0.3333333333333333703, 0.3333333333333333703, 0.3333333333333333703, 0.3333333333333333703, 0.3333333333333333703, 0.3333333333333333703, 0.3333333333333333703, 0.3333333333333333703, 0.3333333333333333703, 0.3333333333333333703, 0.3333333333333333703, 0.3333333333333333703, 0.3333333333333333703, 0.3333333333333333703, 0.3333333333333333703, 0.3333333333333333703, 0.3333333333333333703, 0.3333333333333333703, 0.3333333333333333703, 0.3333333333333333703, 0.3333333333333333703, 0.3333333333333333703, 0.3333333333333333703, 0.3333333333333333703, 0.3333333333333333703, 0.3333333333333333703, 0.3333333333333333703, 0.3333333333333333703, 0.3333333333333333703, 0.3333333333333333703, 0.3333333333333333703, 0.3333333333333333703, 0.3333333333333333703, 0.3333333333333333703, 0.3333333333333333703, 0.3333333333333333703, 0.3333333333333333703, 0.3333333333333333703, 0.3333333333333333703, 0.3333333333333333703, 0.3333333333333333703, 0.3333333333333333703, 0.3333333333333333703, 0.3333333333333333703, 0.3333333333333333703, 0.3333333333333333703, 0.3333333333333333703, 0.3333333333333333703, 0.3333333333333333703, 0.3333333333333333703, 0.3333333333333333703, 0.3333333333333333703, 0.3333333333333333703, 0.3333333333333333703, 0.3333333333333333703, 0.3333333333333333703, 0.3333333333333333703, 0.3333333333333333703, 0.3333333333333333703, 0.3333333333333333703, 0.3333333333333333703, 0.3333333333333333703, 0.3333333333333333703, 0.3333333333333333703, 0.3333333333333333703, 0.3333333333333333703, 0.3333333333333333703, 0.3333333333333333703, 0.3333333333333333703, 0.3333333333333333703, 0.3333333333333333703, 0.3333333333333333703, 0.3333333333333333703, 0.3333333333333333703, 0.3333333333333333703, 0.3333333333333333703, 0.3333333333333333703, 0.3333333333333333703, 0.3333333333333333703, 0.3333333333333333703, 0.3333333333333333703, 0.3333333333333333703, 0.3333333333333333703, 0.3333333333333333703, 0.3333333333333333703, 0.3333333333333333703, 0.3333333333333333703, 0.3333333333333333703, 0.3333333333333333703, 0.3333333333333333703, 0.3333333333333333703, 0.3333333333333333703, 0.3333333333333333703, 0.3333333333333333703, 0.3333333333333333703, 0.3333333333333333703, 0.3333333333333333703, 0.3333333333333333703, 0.3333333333333333703, 0.3333333333333333703, 0.3333333333333333703, 0.3333333333333333703, 0.3333333333333333703, 0.3333333333333333703, 0.3333333333333333703, 0.3333333333333333703, 0.3333333333333333703, 0.3333333333333333703, 0.3333333333333333703, 0.3333333333333333703, 0.3333333333333333703, 0.3333333333333333703, 0.3333333333333333703, 0.3333333333333333703, 0.3333333333333333703, 0.3333333333333333703, 0.3333333333333333703, 0.3333333333333333703, 0.3333333333333333703, 0.3333333333333333703, 0.3333333333333333703, 0.3333333333333333703, 0.3333333333333333703, 0.3333333333333333703, 0.3333333333333333703, 0.3333333333333333703, 0.3333333333333333703, 0.3333333333333333703, 0.3333333333333333703, 0.3333333333333333703, 0.3333333333333333703, 0.3333333333333333703, 0.3333333333333333703, 0.3333333333333333703, 0.3333333333333333703, 0.3333333333333333703, 0.3333333333333333703, 0.3333333333333333703, 0.3333333333333333703, 0.3333333333333333703, 0.3333333333333333703, 0.3333333333333333703, 0.3333333333333333703, 0.3333333333333333703, 0.3333333333333333703, 0.3333333333333333703, 0.3333333333333333703, 0.3333333333333333703, 0.3333333333333333703, 0.3333333333333333703, 0.3333333333333333703, 0.3333333333333333703, 0.3333333333333333703, 0.3333333333333333703, 0.3333333333333333703, 0.3333333333333333703, 0.3333333333333333703, 0.3333333333333333703, 0.3333333333333333703, 0.3333333333333333703, 0.3333333333333333703, 0.3333333333333333703, 0.3333333333333333703, 0.3333333333333333703, 0.3333333333333333703, 0.3333333333333333703, 0.3333333333333333703, 0.3333333333333333703, 0.3333333333333333703, 0.3333333333333333703, 0.3333333333333333703, 0.3333333333333333703, 0.3333333333333333703, 0.3333333333333333703, 0.3333333333333333703, 0.3333333333333333703, 0.3333333333333333703, 0.3333333333333333703, 0.3333333333333333703, 0.3333333333333333703, 0.3333333333333333703, 0.3333333333333333703, 0.3333333333333333703, 0.3333333333333333703, 0.3333333333333333703, 0.3333333333333333703, 0.3333333333333333703, 0.3333333333333333703, 0.3333333333333333703, 0.3333333333333333703, 0.3333333333333333703, 0.3333333333333333703, 0.3333333333333333703, 0.3333333333333333703, 0.3333333333333333703, 0.3333333333333333703, 0.3333333333333333703, 0.3333333333333333703, 0.3333333333333333703, 0.3333333333333333703, 0.3333333333333333703, 0.3333333333333333703, 0.3333333333333333703, 0.3333333333333333703, 0.3333333333333333703, 0.3333333333333333703, 0.3333333333333333703, 0.3333333333333333703, 0.3333333333333333703, 0.3333333333333333703, 0.3333333333333333703, 0.3333333333333333703, 0.3333333333333333703, 0.3333333333333333703, 0.3333333333333333703, 0.3333333333333333703, 0.3333333333333333703, 0.3333333333333333703, 0.3333333333333333703, 0.3333333333333333703, 0.3333333333333333703, 0.3333333333333333703, 0.3333333333333333703, 0.3333333333333333703, 0.3333333333333333703, 0.3333333333333333703, 0.3333333333333333703, 0.3333333333333333703, 0.3333333333333333703, 0.3333333333333333703),
 ( 0.3333333333333333703, 0.3333333333333333703, 0.3333333333333333703, 0.3333333333333333703, 0.3333333333333333703, 0.3333333333333333703, 0.3333333333333333703, 0.3333333333333333703, 0.3333333333333333703, 0.3333333333333333703, 0.3333333333333333703, 0.3333333333333333703, 0.3333333333333333703, 0.3333333333333333703, 0.3333333333333333703, 0.3333333333333333703, 0.3333333333333333703, 0.3333333333333333703, 0.3333333333333333703, 0.3333333333333333703, 0.3333333333333333703, 0.3333333333333333703, 0.3333333333333333703, 0.3333333333333333703, 0.3333333333333333703, 0.3333333333333333703, 0.3333333333333333703, 0.3333333333333333703, 0.3333333333333333703, 0.3333333333333333703, 0.3333333333333333703, 0.3333333333333333703, 0.3333333333333333703, 0.3333333333333333703, 0.3333333333333333703, 0.3333333333333333703, 0.3333333333333333703, 0.3333333333333333703, 0.3333333333333333703, 0.3333333333333333703, 0.3333333333333333703, 0.3333333333333333703, 0.3333333333333333703, 0.3333333333333333703, 0.3333333333333333703, 0.3333333333333333703, 0.3333333333333333703, 0.3333333333333333703, 0.3333333333333333703, 0.3333333333333333703, 0.3333333333333333703, 0.3333333333333333703, 0.3333333333333333703, 0.3333333333333333703, 0.3333333333333333703, 0.3333333333333333703, 0.3333333333333333703, 0.3333333333333333703, 0.3333333333333333703, 0.3333333333333333703, 0.3333333333333333703, 0.3333333333333333703, 0.3333333333333333703, 0.3333333333333333703, 0.3333333333333333703, 0.3333333333333333703, 0.3333333333333333703, 0.3333333333333333703, 0.3333333333333333703, 0.3333333333333333703, 0.3333333333333333703, 0.3333333333333333703, 0.3333333333333333703, 0.3333333333333333703, 0.3333333333333333703, 0.3333333333333333703, 0.3333333333333333703, 0.3333333333333333703, 0.3333333333333333703, 0.3333333333333333703, 0.3333333333333333703, 0.3333333333333333703, 0.3333333333333333703, 0.3333333333333333703, 0.3333333333333333703, 0.3333333333333333703, 0.3333333333333333703, 0.3333333333333333703, 0.3333333333333333703, 0.3333333333333333703, 0.3333333333333333703, 0.3333333333333333703, 0.3333333333333333703, 0.3333333333333333703, 0.3333333333333333703, 0.3333333333333333703, 0.3333333333333333703, 0.3333333333333333703, 0.3333333333333333703, 0.3333333333333333703, 0.3333333333333333703, 0.3333333333333333703, 0.3333333333333333703, 0.3333333333333333703, 0.3333333333333333703, 0.3333333333333333703, 0.3333333333333333703, 0.3333333333333333703, 0.3333333333333333703, 0.3333333333333333703, 0.3333333333333333703, 0.3333333333333333703, 0.3333333333333333703, 0.3333333333333333703, 0.3333333333333333703, 0.3333333333333333703, 0.3333333333333333703, 0.3333333333333333703, 0.3333333333333333703, 0.3333333333333333703, 0.3333333333333333703, 0.3333333333333333703, 0.3333333333333333703, 0.3333333333333333703, 0.3333333333333333703, 0.3333333333333333703, 0.3333333333333333703, 0.3333333333333333703, 0.3333333333333333703, 0.3333333333333333703, 0.3333333333333333703, 0.3333333333333333703, 0.3333333333333333703, 0.3333333333333333703, 0.3333333333333333703, 0.3333333333333333703, 0.3333333333333333703, 0.3333333333333333703, 0.3333333333333333703, 0.3333333333333333703, 0.3333333333333333703, 0.3333333333333333703, 0.3333333333333333703, 0.3333333333333333703, 0.3333333333333333703, 0.3333333333333333703, 0.3333333333333333703, 0.3333333333333333703, 0.3333333333333333703, 0.3333333333333333703, 0.3333333333333333703, 0.3333333333333333703, 0.3333333333333333703, 0.3333333333333333703, 0.3333333333333333703, 0.3333333333333333703, 0.3333333333333333703, 0.3333333333333333703, 0.3333333333333333703, 0.3333333333333333703, 0.3333333333333333703, 0.3333333333333333703, 0.3333333333333333703, 0.3333333333333333703, 0.3333333333333333703, 0.3333333333333333703, 0.3333333333333333703, 0.3333333333333333703, 0.3333333333333333703, 0.3333333333333333703, 0.3333333333333333703, 0.3333333333333333703, 0.3333333333333333703, 0.3333333333333333703, 0.3333333333333333703, 0.3333333333333333703, 0.3333333333333333703, 0.3333333333333333703, 0.3333333333333333703, 0.3333333333333333703, 0.3333333333333333703, 0.3333333333333333703, 0.3333333333333333703, 0.3333333333333333703, 0.3333333333333333703, 0.3333333333333333703, 0.3333333333333333703, 0.3333333333333333703, 0.3333333333333333703, 0.3333333333333333703, 0.3333333333333333703, 0.3333333333333333703, 0.3333333333333333703, 0.3333333333333333703, 0.3333333333333333703, 0.3333333333333333703, 0.3333333333333333703, 0.3333333333333333703, 0.3333333333333333703, 0.3333333333333333703, 0.3333333333333333703, 0.3333333333333333703, 0.3333333333333333703, 0.3333333333333333703, 0.3333333333333333703, 0.3333333333333333703, 0.3333333333333333703, 0.3333333333333333703, 0.3333333333333333703, 0.3333333333333333703, 0.3333333333333333703, 0.3333333333333333703, 0.3333333333333333703, 0.3333333333333333703, 0.3333333333333333703, 0.3333333333333333703, 0.3333333333333333703, 0.3333333333333333703, 0.3333333333333333703, 0.3333333333333333703, 0.3333333333333333703, 0.3333333333333333703, 0.3333333333333333703, 0.3333333333333333703, 0.3333333333333333703, 0.3333333333333333703, 0.3333333333333333703, 0.3333333333333333703, 0.3333333333333333703, 0.3333333333333333703, 0.3333333333333333703, 0.3333333333333333703, 0.3333333333333333703, 0.3333333333333333703, 0.3333333333333333703, 0.3333333333333333703, 0.3333333333333333703, 0.3333333333333333703, 0.3333333333333333703, 0.3333333333333333703, 0.3333333333333333703, 0.3333333333333333703, 0.3333333333333333703, 0.3333333333333333703, 0.3333333333333333703, 0.3333333333333333703, 0.3333333333333333703, 0.3333333333333333703, 0.3333333333333333703, 0.3333333333333333703, 0.3333333333333333703, 0.3333333333333333703, 0.3333333333333333703, 0.3333333333333333703, 0.3333333333333333703, 0.3333333333333333703, 0.3333333333333333703, 0.3333333333333333703, 0.3333333333333333703, 0.3333333333333333703, 0.3333333333333333703, 0.3333333333333333703, 0.3333333333333333703, 0.3333333333333333703, 0.3333333333333333703, 0.3333333333333333703, 0.3333333333333333703, 0.3333333333333333703, 0.3333333333333333703, 0.3333333333333333703, 0.3333333333333333703, 0.3333333333333333703, 0.3333333333333333703, 0.3333333333333333703, 0.3333333333333333703, 0.3333333333333333703, 0.3333333333333333703, 0.3333333333333333703, 0.3333333333333333703, 0.3333333333333333703, 0.3333333333333333703, 0.3333333333333333703, 0.3333333333333333703, 0.3333333333333333703, 0.3333333333333333703, 0.3333333333333333703, 0.3333333333333333703, 0.3333333333333333703, 0.3333333333333333703, 0.3333333333333333703, 0.3333333333333333703, 0.3333333333333333703, 0.3333333333333333703, 0.3333333333333333703, 0.3333333333333333703, 0.3333333333333333703, 0.3333333333333333703, 0.3333333333333333703, 0.3333333333333333703, 0.3333333333333333703, 0.3333333333333333703, 0.3333333333333333703, 0.3333333333333333703, 0.3333333333333333703, 0.3333333333333333703, 0.3333333333333333703, 0.3333333333333333703, 0.3333333333333333703, 0.3333333333333333703, 0.3333333333333333703, 0.3333333333333333703, 0.3333333333333333703, 0.3333333333333333703, 0.3333333333333333703, 0.3333333333333333703, 0.3333333333333333703, 0.3333333333333333703, 0.3333333333333333703, 0.3333333333333333703, 0.3333333333333333703, 0.3333333333333333703, 0.3333333333333333703, 0.3333333333333333703, 0.3333333333333333703, 0.3333333333333333703, 0.3333333333333333703, 0.3333333333333333703, 0.3333333333333333703, 0.3333333333333333703, 0.3333333333333333703, 0.3333333333333333703, 0.3333333333333333703, 0.3333333333333333703, 0.3333333333333333703, 0.3333333333333333703, 0.3333333333333333703),
 ( 1.000000000000000000, 1.000000000000000000, 1.000000000000000000, 1.000000000000000000, 1.000000000000000000, 1.000000000000000000, 1.000000000000000000, 1.000000000000000000, 1.000000000000000000, 1.000000000000000000, 1.000000000000000000, 1.000000000000000000, 1.000000000000000000, 1.000000000000000000, 1.000000000000000000, 1.000000000000000000, 1.000000000000000000, 1.000000000000000000, 1.000000000000000000, 1.000000000000000000, 1.000000000000000000, 1.000000000000000000, 1.000000000000000000, 1.000000000000000000, 1.000000000000000000, 1.000000000000000000, 1.000000000000000000, 1.000000000000000000, 1.000000000000000000, 1.000000000000000000, 1.000000000000000000, 1.000000000000000000, 1.000000000000000000, 1.000000000000000000, 1.000000000000000000, 1.000000000000000000, 1.000000000000000000, 1.000000000000000000, 1.000000000000000000, 1.000000000000000000, 1.000000000000000000, 1.000000000000000000, 1.000000000000000000, 1.000000000000000000, 1.000000000000000000, 1.000000000000000000, 1.000000000000000000, 1.000000000000000000, 1.000000000000000000, 1.000000000000000000, 1.000000000000000000, 1.000000000000000000, 1.000000000000000000, 1.000000000000000000, 1.000000000000000000, 1.000000000000000000, 1.000000000000000000, 1.000000000000000000, 1.000000000000000000, 1.000000000000000000, 1.000000000000000000, 1.000000000000000000, 1.000000000000000000, 1.000000000000000000, 1.000000000000000000, 1.000000000000000000, 1.000000000000000000, 1.000000000000000000, 1.000000000000000000, 1.000000000000000000, 1.000000000000000000, 1.000000000000000000, 1.000000000000000000, 1.000000000000000000, 1.000000000000000000, 1.000000000000000000, 1.000000000000000000, 1.000000000000000000, 1.000000000000000000, 1.000000000000000000, 1.000000000000000000, 1.000000000000000000, 1.000000000000000000, 1.000000000000000000, 1.000000000000000000, 1.000000000000000000, 1.000000000000000000, 1.000000000000000000, 1.000000000000000000, 1.000000000000000000, 1.000000000000000000, 1.000000000000000000, 1.000000000000000000, 1.000000000000000000, 1.000000000000000000, 1.000000000000000000, 1.000000000000000000, 1.000000000000000000, 1.000000000000000000, 1.000000000000000000, 1.000000000000000000, 1.000000000000000000, 1.000000000000000000, 1.000000000000000000, 1.000000000000000000, 1.000000000000000000, 1.000000000000000000, 1.000000000000000000, 1.000000000000000000, 1.000000000000000000, 1.000000000000000000, 1.000000000000000000, 1.000000000000000000, 1.000000000000000000, 1.000000000000000000, 1.000000000000000000, 1.000000000000000000, 1.000000000000000000, 1.000000000000000000, 1.000000000000000000, 1.000000000000000000, 1.000000000000000000, 1.000000000000000000, 1.000000000000000000, 1.000000000000000000, 1.000000000000000000, 1.000000000000000000, 1.000000000000000000, 1.000000000000000000, 1.000000000000000000, 1.000000000000000000, 1.000000000000000000, 1.000000000000000000, 1.000000000000000000, 1.000000000000000000, 1.000000000000000000, 1.000000000000000000, 1.000000000000000000, 1.000000000000000000, 1.000000000000000000, 1.000000000000000000, 1.000000000000000000, 1.000000000000000000, 1.000000000000000000, 1.000000000000000000, 1.000000000000000000, 1.000000000000000000, 1.000000000000000000, 1.000000000000000000, 1.000000000000000000, 1.000000000000000000, 1.000000000000000000, 1.000000000000000000, 1.000000000000000000, 1.000000000000000000, 1.000000000000000000, 1.000000000000000000, 1.000000000000000000, 1.000000000000000000, 1.000000000000000000, 1.000000000000000000, 1.000000000000000000, 1.000000000000000000, 1.000000000000000000, 1.000000000000000000, 1.000000000000000000, 1.000000000000000000, 1.000000000000000000, 1.000000000000000000, 1.000000000000000000, 1.000000000000000000, 1.000000000000000000, 1.000000000000000000, 1.000000000000000000, 1.000000000000000000, 1.000000000000000000, 1.000000000000000000, 1.000000000000000000, 1.000000000000000000, 1.000000000000000000, 1.000000000000000000, 1.000000000000000000, 1.000000000000000000, 1.000000000000000000, 1.000000000000000000, 1.000000000000000000, 1.000000000000000000, 1.000000000000000000, 1.000000000000000000, 1.000000000000000000, 1.000000000000000000, 1.000000000000000000, 1.000000000000000000, 1.000000000000000000, 1.000000000000000000, 1.000000000000000000, 1.000000000000000000, 1.000000000000000000, 1.000000000000000000, 1.000000000000000000, 1.000000000000000000, 1.000000000000000000, 1.000000000000000000, 1.000000000000000000, 1.000000000000000000, 1.000000000000000000, 1.000000000000000000, 1.000000000000000000, 1.000000000000000000, 1.000000000000000000, 1.000000000000000000, 1.000000000000000000, 1.000000000000000000, 1.000000000000000000, 1.000000000000000000, 1.000000000000000000, 1.000000000000000000, 1.000000000000000000, 1.000000000000000000, 1.000000000000000000, 1.000000000000000000, 1.000000000000000000, 1.000000000000000000, 1.000000000000000000, 1.000000000000000000, 1.000000000000000000, 1.000000000000000000, 1.000000000000000000, 1.000000000000000000, 1.000000000000000000, 1.000000000000000000, 1.000000000000000000, 1.000000000000000000, 1.000000000000000000, 1.000000000000000000, 1.000000000000000000, 1.000000000000000000, 1.000000000000000000, 1.000000000000000000, 1.000000000000000000, 1.000000000000000000, 1.000000000000000000, 1.000000000000000000, 1.000000000000000000, 1.000000000000000000, 1.000000000000000000, 1.000000000000000000, 1.000000000000000000, 1.000000000000000000, 1.000000000000000000, 1.000000000000000000, 1.000000000000000000, 1.000000000000000000, 1.000000000000000000, 1.000000000000000000, 1.000000000000000000, 1.000000000000000000, 1.000000000000000000, 1.000000000000000000, 1.000000000000000000, 1.000000000000000000, 1.000000000000000000, 1.000000000000000000, 1.000000000000000000, 1.000000000000000000, 1.000000000000000000, 1.000000000000000000, 1.000000000000000000, 1.000000000000000000, 1.000000000000000000, 1.000000000000000000, 1.000000000000000000, 1.000000000000000000, 1.000000000000000000, 1.000000000000000000, 1.000000000000000000, 1.000000000000000000, 1.000000000000000000, 1.000000000000000000, 1.000000000000000000, 1.000000000000000000, 1.000000000000000000, 1.000000000000000000, 1.000000000000000000, 1.000000000000000000, 1.000000000000000000, 1.000000000000000000, 1.000000000000000000, 1.000000000000000000, 1.000000000000000000, 1.000000000000000000, 1.000000000000000000, 1.000000000000000000, 1.000000000000000000, 1.000000000000000000, 1.000000000000000000, 1.000000000000000000, 1.000000000000000000, 1.000000000000000000, 1.000000000000000000, 1.000000000000000000, 1.000000000000000000, 1.000000000000000000, 1.000000000000000000, 1.000000000000000000, 1.000000000000000000, 1.000000000000000000, 1.000000000000000000, 1.000000000000000000, 1.000000000000000000, 1.000000000000000000, 1.000000000000000000, 1.000000000000000000, 1.000000000000000000, 1.000000000000000000, 1.000000000000000000, 1.000000000000000000, 1.000000000000000000, 1.000000000000000000, 1.000000000000000000, 1.000000000000000000, 1.000000000000000000, 1.000000000000000000, 1.000000000000000000, 1.000000000000000000, 1.000000000000000000, 1.000000000000000000, 1.000000000000000000, 1.000000000000000000, 1.000000000000000000, 1.000000000000000000, 1.000000000000000000, 1.000000000000000000, 1.000000000000000000, 1.000000000000000000, 1.000000000000000000),
 ( 0.3333333333333333703, 0.3333333333333333703, 0.3333333333333333703, 0.3333333333333333703, 0.3333333333333333703, 0.3333333333333333703, 0.3333333333333333703, 0.3333333333333333703, 0.3333333333333333703, 0.3333333333333333703, 0.3333333333333333703, 0.3333333333333333703, 0.3333333333333333703, 0.3333333333333333703, 0.3333333333333333703, 0.3333333333333333703, 0.3333333333333333703, 0.3333333333333333703, 0.3333333333333333703, 0.3333333333333333703, 0.3333333333333333703, 0.3333333333333333703, 0.3333333333333333703, 0.3333333333333333703, 0.3333333333333333703, 0.3333333333333333703, 0.3333333333333333703, 0.3333333333333333703, 0.3333333333333333703, 0.3333333333333333703, 0.3333333333333333703, 0.3333333333333333703, 0.3333333333333333703, 0.3333333333333333703, 0.3333333333333333703, 0.3333333333333333703, 0.3333333333333333703, 0.3333333333333333703, 0.3333333333333333703, 0.3333333333333333703, 0.3333333333333333703, 0.3333333333333333703, 0.3333333333333333703, 0.3333333333333333703, 0.3333333333333333703, 0.3333333333333333703, 0.3333333333333333703, 0.3333333333333333703, 0.3333333333333333703, 0.3333333333333333703, 0.3333333333333333703, 0.3333333333333333703, 0.3333333333333333703, 0.3333333333333333703, 0.3333333333333333703, 0.3333333333333333703, 0.3333333333333333703, 0.3333333333333333703, 0.3333333333333333703, 0.3333333333333333703, 0.3333333333333333703, 0.3333333333333333703, 0.3333333333333333703, 0.3333333333333333703, 0.3333333333333333703, 0.3333333333333333703, 0.3333333333333333703, 0.3333333333333333703, 0.3333333333333333703, 0.3333333333333333703, 0.3333333333333333703, 0.3333333333333333703, 0.3333333333333333703, 0.3333333333333333703, 0.3333333333333333703, 0.3333333333333333703, 0.3333333333333333703, 0.3333333333333333703, 0.3333333333333333703, 0.3333333333333333703, 0.3333333333333333703, 0.3333333333333333703, 0.3333333333333333703, 0.3333333333333333703, 0.3333333333333333703, 0.3333333333333333703, 0.3333333333333333703, 0.3333333333333333703, 0.3333333333333333703, 0.3333333333333333703, 0.3333333333333333703, 0.3333333333333333703, 0.3333333333333333703, 0.3333333333333333703, 0.3333333333333333703, 0.3333333333333333703, 0.3333333333333333703, 0.3333333333333333703, 0.3333333333333333703, 0.3333333333333333703, 0.3333333333333333703, 0.3333333333333333703, 0.3333333333333333703, 0.3333333333333333703, 0.3333333333333333703, 0.3333333333333333703, 0.3333333333333333703, 0.3333333333333333703, 0.3333333333333333703, 0.3333333333333333703, 0.3333333333333333703, 0.3333333333333333703, 0.3333333333333333703, 0.3333333333333333703, 0.3333333333333333703, 0.3333333333333333703, 0.3333333333333333703, 0.3333333333333333703, 0.3333333333333333703, 0.3333333333333333703, 0.3333333333333333703, 0.3333333333333333703, 0.3333333333333333703, 0.3333333333333333703, 0.3333333333333333703, 0.3333333333333333703, 0.3333333333333333703, 0.3333333333333333703, 0.3333333333333333703, 0.3333333333333333703, 0.3333333333333333703, 0.3333333333333333703, 0.3333333333333333703, 0.3333333333333333703, 0.3333333333333333703, 0.3333333333333333703, 0.3333333333333333703, 0.3333333333333333703, 0.3333333333333333703, 0.3333333333333333703, 0.3333333333333333703, 0.3333333333333333703, 0.3333333333333333703, 0.3333333333333333703, 0.3333333333333333703, 0.3333333333333333703, 0.3333333333333333703, 0.3333333333333333703, 0.3333333333333333703, 0.3333333333333333703, 0.3333333333333333703, 0.3333333333333333703, 0.3333333333333333703, 0.3333333333333333703, 0.3333333333333333703, 0.3333333333333333703, 0.3333333333333333703, 0.3333333333333333703, 0.3333333333333333703, 0.3333333333333333703, 0.3333333333333333703, 0.3333333333333333703, 0.3333333333333333703, 0.3333333333333333703, 0.3333333333333333703, 0.3333333333333333703, 0.3333333333333333703, 0.3333333333333333703, 0.3333333333333333703, 0.3333333333333333703, 0.3333333333333333703, 0.3333333333333333703, 0.3333333333333333703, 0.3333333333333333703, 0.3333333333333333703, 0.3333333333333333703, 0.3333333333333333703, 0.3333333333333333703, 0.3333333333333333703, 0.3333333333333333703, 0.3333333333333333703, 0.3333333333333333703, 0.3333333333333333703, 0.3333333333333333703, 0.3333333333333333703, 0.3333333333333333703, 0.3333333333333333703, 0.3333333333333333703, 0.3333333333333333703, 0.3333333333333333703, 0.3333333333333333703, 0.3333333333333333703, 0.3333333333333333703, 0.3333333333333333703, 0.3333333333333333703, 0.3333333333333333703, 0.3333333333333333703, 0.3333333333333333703, 0.3333333333333333703, 0.3333333333333333703, 0.3333333333333333703, 0.3333333333333333703, 0.3333333333333333703, 0.3333333333333333703, 0.3333333333333333703, 0.3333333333333333703, 0.3333333333333333703, 0.3333333333333333703, 0.3333333333333333703, 0.3333333333333333703, 0.3333333333333333703, 0.3333333333333333703, 0.3333333333333333703, 0.3333333333333333703, 0.3333333333333333703, 0.3333333333333333703, 0.3333333333333333703, 0.3333333333333333703, 0.3333333333333333703, 0.3333333333333333703, 0.3333333333333333703, 0.3333333333333333703, 0.3333333333333333703, 0.3333333333333333703, 0.3333333333333333703, 0.3333333333333333703, 0.3333333333333333703, 0.3333333333333333703, 0.3333333333333333703, 0.3333333333333333703, 0.3333333333333333703, 0.3333333333333333703, 0.3333333333333333703, 0.3333333333333333703, 0.3333333333333333703, 0.3333333333333333703, 0.3333333333333333703, 0.3333333333333333703, 0.3333333333333333703, 0.3333333333333333703, 0.3333333333333333703, 0.3333333333333333703, 0.3333333333333333703, 0.3333333333333333703, 0.3333333333333333703, 0.3333333333333333703, 0.3333333333333333703, 0.3333333333333333703, 0.3333333333333333703, 0.3333333333333333703, 0.3333333333333333703, 0.3333333333333333703, 0.3333333333333333703, 0.3333333333333333703, 0.3333333333333333703, 0.3333333333333333703, 0.3333333333333333703, 0.3333333333333333703, 0.3333333333333333703, 0.3333333333333333703, 0.3333333333333333703, 0.3333333333333333703, 0.3333333333333333703, 0.3333333333333333703, 0.3333333333333333703, 0.3333333333333333703, 0.3333333333333333703, 0.3333333333333333703, 0.3333333333333333703, 0.3333333333333333703, 0.3333333333333333703, 0.3333333333333333703, 0.3333333333333333703, 0.3333333333333333703, 0.3333333333333333703, 0.3333333333333333703, 0.3333333333333333703, 0.3333333333333333703, 0.3333333333333333703, 0.3333333333333333703, 0.3333333333333333703, 0.3333333333333333703, 0.3333333333333333703, 0.3333333333333333703, 0.3333333333333333703, 0.3333333333333333703, 0.3333333333333333703, 0.3333333333333333703, 0.3333333333333333703, 0.3333333333333333703, 0.3333333333333333703, 0.3333333333333333703, 0.3333333333333333703, 0.3333333333333333703, 0.3333333333333333703, 0.3333333333333333703, 0.3333333333333333703, 0.3333333333333333703, 0.3333333333333333703, 0.3333333333333333703, 0.3333333333333333703, 0.3333333333333333703, 0.3333333333333333703, 0.3333333333333333703, 0.3333333333333333703, 0.3333333333333333703, 0.3333333333333333703, 0.3333333333333333703, 0.3333333333333333703, 0.3333333333333333703, 0.3333333333333333703, 0.3333333333333333703, 0.3333333333333333703, 0.3333333333333333703, 0.3333333333333333703, 0.3333333333333333703, 0.3333333333333333703, 0.3333333333333333703, 0.3333333333333333703, 0.3333333333333333703, 0.3333333333333333703, 0.3333333333333333703, 0.3333333333333333703, 0.3333333333333333703, 0.3333333333333333703, 0.3333333333333333703, 0.3333333333333333703, 0.3333333333333333703, 0.3333333333333333703, 0.3333333333333333703, 0.3333333333333333703, 0.3333333333333333703, 0.3333333333333333703, 0.3333333333333333703, 0.3333333333333333703, 0.3333333333333333703),
 ( 0.3333333333333333703, 0.3333333333333333703, 0.3333333333333333703, 0.3333333333333333703, 0.3333333333333333703, 0.3333333333333333703, 0.3333333333333333703, 0.3333333333333333703, 0.3333333333333333703, 0.3333333333333333703, 0.3333333333333333703, 0.3333333333333333703, 0.3333333333333333703, 0.3333333333333333703, 0.3333333333333333703, 0.3333333333333333703, 0.3333333333333333703, 0.3333333333333333703, 0.3333333333333333703, 0.3333333333333333703, 0.3333333333333333703, 0.3333333333333333703, 0.3333333333333333703, 0.3333333333333333703, 0.3333333333333333703, 0.3333333333333333703, 0.3333333333333333703, 0.3333333333333333703, 0.3333333333333333703, 0.3333333333333333703, 0.3333333333333333703, 0.3333333333333333703, 0.3333333333333333703, 0.3333333333333333703, 0.3333333333333333703, 0.3333333333333333703, 0.3333333333333333703, 0.3333333333333333703, 0.3333333333333333703, 0.3333333333333333703, 0.3333333333333333703, 0.3333333333333333703, 0.3333333333333333703, 0.3333333333333333703, 0.3333333333333333703, 0.3333333333333333703, 0.3333333333333333703, 0.3333333333333333703, 0.3333333333333333703, 0.3333333333333333703, 0.3333333333333333703, 0.3333333333333333703, 0.3333333333333333703, 0.3333333333333333703, 0.3333333333333333703, 0.3333333333333333703, 0.3333333333333333703, 0.3333333333333333703, 0.3333333333333333703, 0.3333333333333333703, 0.3333333333333333703, 0.3333333333333333703, 0.3333333333333333703, 0.3333333333333333703, 0.3333333333333333703, 0.3333333333333333703, 0.3333333333333333703, 0.3333333333333333703, 0.3333333333333333703, 0.3333333333333333703, 0.3333333333333333703, 0.3333333333333333703, 0.3333333333333333703, 0.3333333333333333703, 0.3333333333333333703, 0.3333333333333333703, 0.3333333333333333703, 0.3333333333333333703, 0.3333333333333333703, 0.3333333333333333703, 0.3333333333333333703, 0.3333333333333333703, 0.3333333333333333703, 0.3333333333333333703, 0.3333333333333333703, 0.3333333333333333703, 0.3333333333333333703, 0.3333333333333333703, 0.3333333333333333703, 0.3333333333333333703, 0.3333333333333333703, 0.3333333333333333703, 0.3333333333333333703, 0.3333333333333333703, 0.3333333333333333703, 0.3333333333333333703, 0.3333333333333333703, 0.3333333333333333703, 0.3333333333333333703, 0.3333333333333333703, 0.3333333333333333703, 0.3333333333333333703, 0.3333333333333333703, 0.3333333333333333703, 0.3333333333333333703, 0.3333333333333333703, 0.3333333333333333703, 0.3333333333333333703, 0.3333333333333333703, 0.3333333333333333703, 0.3333333333333333703, 0.3333333333333333703, 0.3333333333333333703, 0.3333333333333333703, 0.3333333333333333703, 0.3333333333333333703, 0.3333333333333333703, 0.3333333333333333703, 0.3333333333333333703, 0.3333333333333333703, 0.3333333333333333703, 0.3333333333333333703, 0.3333333333333333703, 0.3333333333333333703, 0.3333333333333333703, 0.3333333333333333703, 0.3333333333333333703, 0.3333333333333333703, 0.3333333333333333703, 0.3333333333333333703, 0.3333333333333333703, 0.3333333333333333703, 0.3333333333333333703, 0.3333333333333333703, 0.3333333333333333703, 0.3333333333333333703, 0.3333333333333333703, 0.3333333333333333703, 0.3333333333333333703, 0.3333333333333333703, 0.3333333333333333703, 0.3333333333333333703, 0.3333333333333333703, 0.3333333333333333703, 0.3333333333333333703, 0.3333333333333333703, 0.3333333333333333703, 0.3333333333333333703, 0.3333333333333333703, 0.3333333333333333703, 0.3333333333333333703, 0.3333333333333333703, 0.3333333333333333703, 0.3333333333333333703, 0.3333333333333333703, 0.3333333333333333703, 0.3333333333333333703, 0.3333333333333333703, 0.3333333333333333703, 0.3333333333333333703, 0.3333333333333333703, 0.3333333333333333703, 0.3333333333333333703, 0.3333333333333333703, 0.3333333333333333703, 0.3333333333333333703, 0.3333333333333333703, 0.3333333333333333703, 0.3333333333333333703, 0.3333333333333333703, 0.3333333333333333703, 0.3333333333333333703, 0.3333333333333333703, 0.3333333333333333703, 0.3333333333333333703, 0.3333333333333333703, 0.3333333333333333703, 0.3333333333333333703, 0.3333333333333333703, 0.3333333333333333703, 0.3333333333333333703, 0.3333333333333333703, 0.3333333333333333703, 0.3333333333333333703, 0.3333333333333333703, 0.3333333333333333703, 0.3333333333333333703, 0.3333333333333333703, 0.3333333333333333703, 0.3333333333333333703, 0.3333333333333333703, 0.3333333333333333703, 0.3333333333333333703, 0.3333333333333333703, 0.3333333333333333703, 0.3333333333333333703, 0.3333333333333333703, 0.3333333333333333703, 0.3333333333333333703, 0.3333333333333333703, 0.3333333333333333703, 0.3333333333333333703, 0.3333333333333333703, 0.3333333333333333703, 0.3333333333333333703, 0.3333333333333333703, 0.3333333333333333703, 0.3333333333333333703, 0.3333333333333333703, 0.3333333333333333703, 0.3333333333333333703, 0.3333333333333333703, 0.3333333333333333703, 0.3333333333333333703, 0.3333333333333333703, 0.3333333333333333703, 0.3333333333333333703, 0.3333333333333333703, 0.3333333333333333703, 0.3333333333333333703, 0.3333333333333333703, 0.3333333333333333703, 0.3333333333333333703, 0.3333333333333333703, 0.3333333333333333703, 0.3333333333333333703, 0.3333333333333333703, 0.3333333333333333703, 0.3333333333333333703, 0.3333333333333333703, 0.3333333333333333703, 0.3333333333333333703, 0.3333333333333333703, 0.3333333333333333703, 0.3333333333333333703, 0.3333333333333333703, 0.3333333333333333703, 0.3333333333333333703, 0.3333333333333333703, 0.3333333333333333703, 0.3333333333333333703, 0.3333333333333333703, 0.3333333333333333703, 0.3333333333333333703, 0.3333333333333333703, 0.3333333333333333703, 0.3333333333333333703, 0.3333333333333333703, 0.3333333333333333703, 0.3333333333333333703, 0.3333333333333333703, 0.3333333333333333703, 0.3333333333333333703, 0.3333333333333333703, 0.3333333333333333703, 0.3333333333333333703, 0.3333333333333333703, 0.3333333333333333703, 0.3333333333333333703, 0.3333333333333333703, 0.3333333333333333703, 0.3333333333333333703, 0.3333333333333333703, 0.3333333333333333703, 0.3333333333333333703, 0.3333333333333333703, 0.3333333333333333703, 0.3333333333333333703, 0.3333333333333333703, 0.3333333333333333703, 0.3333333333333333703, 0.3333333333333333703, 0.3333333333333333703, 0.3333333333333333703, 0.3333333333333333703, 0.3333333333333333703, 0.3333333333333333703, 0.3333333333333333703, 0.3333333333333333703, 0.3333333333333333703, 0.3333333333333333703, 0.3333333333333333703, 0.3333333333333333703, 0.3333333333333333703, 0.3333333333333333703, 0.3333333333333333703, 0.3333333333333333703, 0.3333333333333333703, 0.3333333333333333703, 0.3333333333333333703, 0.3333333333333333703, 0.3333333333333333703, 0.3333333333333333703, 0.3333333333333333703, 0.3333333333333333703, 0.3333333333333333703, 0.3333333333333333703, 0.3333333333333333703, 0.3333333333333333703, 0.3333333333333333703, 0.3333333333333333703, 0.3333333333333333703, 0.3333333333333333703, 0.3333333333333333703, 0.3333333333333333703, 0.3333333333333333703, 0.3333333333333333703, 0.3333333333333333703, 0.3333333333333333703, 0.3333333333333333703, 0.3333333333333333703, 0.3333333333333333703, 0.3333333333333333703, 0.3333333333333333703, 0.3333333333333333703, 0.3333333333333333703, 0.3333333333333333703, 0.3333333333333333703, 0.3333333333333333703, 0.3333333333333333703, 0.3333333333333333703, 0.3333333333333333703, 0.3333333333333333703, 0.3333333333333333703, 0.3333333333333333703, 0.3333333333333333703, 0.3333333333333333703, 0.3333333333333333703, 0.3333333333333333703, 0.3333333333333333703, 0.3333333333333333703, 0.3333333333333333703, 0.3333333333333333703, 0.3333333333333333703, 0.3333333333333333703, 0.3333333333333333703),
 ( 1.000000000000000000, 1.000000000000000000, 1.000000000000000000, 1.000000000000000000, 1.000000000000000000, 1.000000000000000000, 1.000000000000000000, 1.000000000000000000, 1.000000000000000000, 1.000000000000000000, 1.000000000000000000, 1.000000000000000000, 1.000000000000000000, 1.000000000000000000, 1.000000000000000000, 1.000000000000000000, 1.000000000000000000, 1.000000000000000000, 1.000000000000000000, 1.000000000000000000, 1.000000000000000000, 1.000000000000000000, 1.000000000000000000, 1.000000000000000000, 1.000000000000000000, 1.000000000000000000, 1.000000000000000000, 1.000000000000000000, 1.000000000000000000, 1.000000000000000000, 1.000000000000000000, 1.000000000000000000, 1.000000000000000000, 1.000000000000000000, 1.000000000000000000, 1.000000000000000000, 1.000000000000000000, 1.000000000000000000, 1.000000000000000000, 1.000000000000000000, 1.000000000000000000, 1.000000000000000000, 1.000000000000000000, 1.000000000000000000, 1.000000000000000000, 1.000000000000000000, 1.000000000000000000, 1.000000000000000000, 1.000000000000000000, 1.000000000000000000, 1.000000000000000000, 1.000000000000000000, 1.000000000000000000, 1.000000000000000000, 1.000000000000000000, 1.000000000000000000, 1.000000000000000000, 1.000000000000000000, 1.000000000000000000, 1.000000000000000000, 1.000000000000000000, 1.000000000000000000, 1.000000000000000000, 1.000000000000000000, 1.000000000000000000, 1.000000000000000000, 1.000000000000000000, 1.000000000000000000, 1.000000000000000000, 1.000000000000000000, 1.000000000000000000, 1.000000000000000000, 1.000000000000000000, 1.000000000000000000, 1.000000000000000000, 1.000000000000000000, 1.000000000000000000, 1.000000000000000000, 1.000000000000000000, 1.000000000000000000, 1.000000000000000000, 1.000000000000000000, 1.000000000000000000, 1.000000000000000000, 1.000000000000000000, 1.000000000000000000, 1.000000000000000000, 1.000000000000000000, 1.000000000000000000, 1.000000000000000000, 1.000000000000000000, 1.000000000000000000, 1.000000000000000000, 1.000000000000000000, 1.000000000000000000, 1.000000000000000000, 1.000000000000000000, 1.000000000000000000, 1.000000000000000000, 1.000000000000000000, 1.000000000000000000, 1.000000000000000000, 1.000000000000000000, 1.000000000000000000, 1.000000000000000000, 1.000000000000000000, 1.000000000000000000, 1.000000000000000000, 1.000000000000000000, 1.000000000000000000, 1.000000000000000000, 1.000000000000000000, 1.000000000000000000, 1.000000000000000000, 1.000000000000000000, 1.000000000000000000, 1.000000000000000000, 1.000000000000000000, 1.000000000000000000, 1.000000000000000000, 1.000000000000000000, 1.000000000000000000, 1.000000000000000000, 1.000000000000000000, 1.000000000000000000, 1.000000000000000000, 1.000000000000000000, 1.000000000000000000, 1.000000000000000000, 1.000000000000000000, 1.000000000000000000, 1.000000000000000000, 1.000000000000000000, 1.000000000000000000, 1.000000000000000000, 1.000000000000000000, 1.000000000000000000, 1.000000000000000000, 1.000000000000000000, 1.000000000000000000, 1.000000000000000000, 1.000000000000000000, 1.000000000000000000, 1.000000000000000000, 1.000000000000000000, 1.000000000000000000, 1.000000000000000000, 1.000000000000000000, 1.000000000000000000, 1.000000000000000000, 1.000000000000000000, 1.000000000000000000, 1.000000000000000000, 1.000000000000000000, 1.000000000000000000, 1.000000000000000000, 1.000000000000000000, 1.000000000000000000, 1.000000000000000000, 1.000000000000000000, 1.000000000000000000, 1.000000000000000000, 1.000000000000000000, 1.000000000000000000, 1.000000000000000000, 1.000000000000000000, 1.000000000000000000, 1.000000000000000000, 1.000000000000000000, 1.000000000000000000, 1.000000000000000000, 1.000000000000000000, 1.000000000000000000, 1.000000000000000000, 1.000000000000000000, 1.000000000000000000, 1.000000000000000000, 1.000000000000000000, 1.000000000000000000, 1.000000000000000000, 1.000000000000000000, 1.000000000000000000, 1.000000000000000000, 1.000000000000000000, 1.000000000000000000, 1.000000000000000000, 1.000000000000000000, 1.000000000000000000, 1.000000000000000000, 1.000000000000000000, 1.000000000000000000, 1.000000000000000000, 1.000000000000000000, 1.000000000000000000, 1.000000000000000000, 1.000000000000000000, 1.000000000000000000, 1.000000000000000000, 1.000000000000000000, 1.000000000000000000, 1.000000000000000000, 1.000000000000000000, 1.000000000000000000, 1.000000000000000000, 1.000000000000000000, 1.000000000000000000, 1.000000000000000000, 1.000000000000000000, 1.000000000000000000, 1.000000000000000000, 1.000000000000000000, 1.000000000000000000, 1.000000000000000000, 1.000000000000000000, 1.000000000000000000, 1.000000000000000000, 1.000000000000000000, 1.000000000000000000, 1.000000000000000000, 1.000000000000000000, 1.000000000000000000, 1.000000000000000000, 1.000000000000000000, 1.000000000000000000, 1.000000000000000000, 1.000000000000000000, 1.000000000000000000, 1.000000000000000000, 1.000000000000000000, 1.000000000000000000, 1.000000000000000000, 1.000000000000000000, 1.000000000000000000, 1.000000000000000000, 1.000000000000000000, 1.000000000000000000, 1.000000000000000000, 1.000000000000000000, 1.000000000000000000, 1.000000000000000000, 1.000000000000000000, 1.000000000000000000, 1.000000000000000000, 1.000000000000000000, 1.000000000000000000, 1.000000000000000000, 1.000000000000000000, 1.000000000000000000, 1.000000000000000000, 1.000000000000000000, 1.000000000000000000, 1.000000000000000000, 1.000000000000000000, 1.000000000000000000, 1.000000000000000000, 1.000000000000000000, 1.000000000000000000, 1.000000000000000000, 1.000000000000000000, 1.000000000000000000, 1.000000000000000000, 1.000000000000000000, 1.000000000000000000, 1.000000000000000000, 1.000000000000000000, 1.000000000000000000, 1.000000000000000000, 1.000000000000000000, 1.000000000000000000, 1.000000000000000000, 1.000000000000000000, 1.000000000000000000, 1.000000000000000000, 1.000000000000000000, 1.000000000000000000, 1.000000000000000000, 1.000000000000000000, 1.000000000000000000, 1.000000000000000000, 1.000000000000000000, 1.000000000000000000, 1.000000000000000000, 1.000000000000000000, 1.000000000000000000, 1.000000000000000000, 1.000000000000000000, 1.000000000000000000, 1.000000000000000000, 1.000000000000000000, 1.000000000000000000, 1.000000000000000000, 1.000000000000000000, 1.000000000000000000, 1.000000000000000000, 1.000000000000000000, 1.000000000000000000, 1.000000000000000000, 1.000000000000000000, 1.000000000000000000, 1.000000000000000000, 1.000000000000000000, 1.000000000000000000, 1.000000000000000000, 1.000000000000000000, 1.000000000000000000, 1.000000000000000000, 1.000000000000000000, 1.000000000000000000, 1.000000000000000000, 1.000000000000000000, 1.000000000000000000, 1.000000000000000000, 1.000000000000000000, 1.000000000000000000, 1.000000000000000000, 1.000000000000000000, 1.000000000000000000, 1.000000000000000000, 1.000000000000000000, 1.000000000000000000, 1.000000000000000000, 1.000000000000000000, 1.000000000000000000, 1.000000000000000000, 1.000000000000000000, 1.000000000000000000, 1.000000000000000000, 1.000000000000000000, 1.000000000000000000, 1.000000000000000000, 1.000000000000000000, 1.000000000000000000, 1.000000000000000000, 1.000000000000000000, 1.000000000000000000, 1.000000000000000000) ) ) 
 REPRESENTATION_ITEM ( '' )  SURFACE ( )  );
#5403=CARTESIAN_POINT ( 'NONE',  ( -31.58308234758948174, -0.5371106682196264970, -221.7519263543700845 ) ) ;
#5405=CARTESIAN_POINT ( 'NONE',  ( -13.68337831708448782, -3.656824064325736590, -221.3737413816871538 ) ) ;
#5407=CARTESIAN_POINT ( 'NONE',  ( -11.19105919052231179, 21.17456633634251872, -216.2128528132037957 ) ) ;
#5408=CARTESIAN_POINT ( 'NONE',  ( -7.349743644505656093, -15.31718010764164539, -232.4470764718129772 ) ) ;
#5409=CARTESIAN_POINT ( 'NONE',  ( 4.340445191644851874, 29.86837761166362881, -227.4879512554873315 ) ) ;
#5410=CARTESIAN_POINT ( 'NONE',  ( 4.449544252370068342, -12.87211356511098082, -219.5022864574935113 ) ) ;
#5411=CARTESIAN_POINT ( 'NONE',  ( -26.22594988380878789, -0.1068133454905619700, -219.1167922977186322 ) ) ;
#5413=CARTESIAN_POINT ( 'NONE',  ( -26.02492405343843984, 6.940268742526972900, -218.8798307745116460 ) ) ;
#5415=CARTESIAN_POINT ( 'NONE',  ( -2.693916085894628942, 18.86613858709357672, -230.4911878356387263 ) ) ;
#5416=CARTESIAN_POINT ( 'NONE',  ( -21.43408368508570305, 3.680162304907783621, -233.1134812316964542 ) ) ;
#5417=CARTESIAN_POINT ( 'NONE',  ( 14.22574309452842733, 4.476723532073429546, -225.5862451792618231 ) ) ;
#5418=CARTESIAN_POINT ( 'NONE',  ( 26.39436175479395885, 14.32821500273865034, -221.6819523832376149 ) ) ;
#5419=CARTESIAN_POINT ( 'NONE',  ( 4.210909054564462295, -12.48022235161367988, -220.2789660014272215 ) ) ;
#5421=CARTESIAN_POINT ( 'NONE',  ( 11.38520239593705163, 18.87760105923376486, -235.3435298574111130 ) ) ;
#5423=CARTESIAN_POINT ( 'NONE',  ( -1.366762408920091598, -18.58806247050231875, -233.7525452272278699 ) ) ;
#5424=CARTESIAN_POINT ( 'NONE',  ( -4.073886805163430935, 14.35067061637828623, -226.4733297826468572 ) ) ;
#5425=CARTESIAN_POINT ( 'NONE',  ( 7.018811797190238622, 13.93862807232938472, -230.2855929063610176 ) ) ;
#5426=CARTESIAN_POINT ( 'NONE',  ( -20.85586116824185510, -1.996934699305910499, -232.3804859832740135 ) ) ;
#5427=CARTESIAN_POINT ( 'NONE',  ( -15.47996233766743934, 8.203483081506188768, -221.0931279926996353 ) ) ;
#5428=CARTESIAN_POINT ( 'NONE',  ( -0.6224962293416278492, 14.12372964796689701, -218.2103911528446645 ) ) ;
#5429=CARTESIAN_POINT ( 'NONE',  ( 21.18605525173251891, 3.426801613781890854, -232.1183243183448894 ) ) ;
#5431=CARTESIAN_POINT ( 'NONE',  ( 7.487558183825500535, -19.68056729374139380, -230.9679144533258466 ) ) ;
#5433=CARTESIAN_POINT ( 'NONE',  ( 5.920964624126254350, -19.79845160325395526, -232.2234910544682123 ) ) ;
#5434=CARTESIAN_POINT ( 'NONE',  ( -6.407569900110946293, 14.82357759665407215, -221.6203916094852957 ) ) ;
#5438=CARTESIAN_POINT ( 'NONE',  ( 17.68508104102419409, 23.41266195669770767, -227.5327139115408954 ) ) ;
#5439=CARTESIAN_POINT ( 'NONE',  ( 28.36095019830170472, -8.296631283839911220, -225.2861439608085448 ) ) ;
#5440=CARTESIAN_POINT ( 'NONE',  ( -9.606889355748592152, -11.26588727105406385, -229.9123324032181586 ) ) ;
#5441=CARTESIAN_POINT ( 'NONE',  ( -0.6367083786117293531, -29.73461014436635708, -220.1383336929387724 ) ) ;
#5442=CARTESIAN_POINT ( 'NONE',  ( -4.285397168228398890, 18.56782363833054106, -219.4990091916804715 ) ) ;
#5444=CARTESIAN_POINT ( 'NONE',  ( 17.51175949430614409, 14.31829016556564937, -218.8195841045835550 ) ) ;
#5445=CARTESIAN_POINT ( 'NONE',  ( -12.74846050492543625, 19.93509882904884734, -216.0172840992881049 ) ) ;
#5446=CARTESIAN_POINT ( 'NONE',  ( -9.175187729848801155, 26.50888816229029743, -227.9285554593684253 ) ) ;
#5449=CARTESIAN_POINT ( 'NONE',  ( 9.880827190695510964, 24.82036951119805579, -218.1633337467656020 ) ) ;
#5450=CARTESIAN_POINT ( 'NONE',  ( -20.92673740658815973, 5.672885432599523270, -219.1433548642331459 ) ) ;
#5451=CARTESIAN_POINT ( 'NONE',  ( 25.30941179858102430, 8.661697827793627624, -216.7530520919057722 ) ) ;
#5452=CARTESIAN_POINT ( 'NONE',  ( 13.60960062514055657, -26.18013421850907108, -225.9721930653775246 ) ) ;
#5455=CARTESIAN_POINT ( 'NONE',  ( -3.643097910890548796, 22.16888955197135047, -233.9701981029593298 ) ) ;
#5456=CARTESIAN_POINT ( 'NONE',  ( 15.68576712525985251, -3.705577278900763716, -224.6781181500375908 ) ) ;
#5457=CARTESIAN_POINT ( 'NONE',  ( 15.24934971233792957, -1.903332227395571508, -221.9416920766431076 ) ) ;
#5459=CARTESIAN_POINT ( 'NONE',  ( 27.40550551777678123, 5.967061366481472895, -228.7463788799179554 ) ) ;
#5460=CARTESIAN_POINT ( 'NONE',  ( -18.71530386740073126, -0.6857509888707814527, -217.6195632122020527 ) ) ;
#5461=CARTESIAN_POINT ( 'NONE',  ( 5.982950994121768673, -14.58086824529316594, -231.1438280359330975 ) ) ;
#5463=CARTESIAN_POINT ( 'NONE',  ( -24.24202834850560606, 19.05981756344202438, -226.6980666352953335 ) ) ;
#5464=CARTESIAN_POINT ( 'NONE',  ( -13.25293905438448405, 17.39325876214774524, -215.6628841494472510 ) ) ;
#5466=CARTESIAN_POINT ( 'NONE',  ( -14.68037037322036475, 3.441677802729143920, -220.1396515630443389 ) ) ;
#5467=CARTESIAN_POINT ( 'NONE',  ( -12.60959727102843786, -12.64039607560028600, -218.2377899390859284 ) ) ;
#5469=CARTESIAN_POINT ( 'NONE',  ( 19.20300624114736721, 0.6066039755357417462, -231.5046416827383950 ) ) ;
#5470=CARTESIAN_POINT ( 'NONE',  ( -12.44873260470819787, 7.411970124596155785, -229.4214091473984070 ) ) ;
#5471=CARTESIAN_POINT ( 'NONE',  ( 1.780865994697476307, -30.77012162006053941, -222.8552464324424705 ) ) ;
#5475=CARTESIAN_POINT ( 'NONE',  ( 23.44063276014420794, 13.61134749381700182, -229.1061940987080732 ) ) ;
#5476=CARTESIAN_POINT ( 'NONE',  ( -14.12265793148702464, 24.49085167151569919, -218.3312790639385241 ) ) ;
#5478=CARTESIAN_POINT ( 'NONE',  ( 15.70200226922815290, 22.14006925444000018, -227.8255507828836244 ) ) ;
#5479=CARTESIAN_POINT ( 'NONE',  ( -3.968800477764047319, -14.91200208314756104, -226.8245746385127575 ) ) ;
#5481=CARTESIAN_POINT ( 'NONE',  ( -8.317278876689359279, 23.15034512777772235, -218.2935523245793092 ) ) ;
#5482=CARTESIAN_POINT ( 'NONE',  ( -16.56270003954679382, 4.935922114544952777, -221.6503923146493378 ) ) ;
#5483=CARTESIAN_POINT ( 'NONE',  ( -12.79639481117843935, 1.974037863663017589, -229.6094308443170746 ) ) ;
#5485=CARTESIAN_POINT ( 'NONE',  ( -18.48279503042009964, -19.02624011246567548, -221.2510238762918107 ) ) ;
#5488=CARTESIAN_POINT ( 'NONE',  ( 25.85597688020959239, 3.954559836939000039, -230.6766427064781624 ) ) ;
#5489=CARTESIAN_POINT ( 'NONE',  ( 4.834917880317126659, -18.50358955815650219, -219.1181532354089256 ) ) ;
#5490=CARTESIAN_POINT ( 'NONE',  ( 11.57669841200422134, 10.63052136557218574, -228.9489978335593889 ) ) ;
#5491=CARTESIAN_POINT ( 'NONE',  ( -17.17400284685640344, 24.63223427531467280, -220.6313524368512162 ) ) ;
#5495=CARTESIAN_POINT ( 'NONE',  ( 13.40064012097826307, 2.532414129335418096, -221.5952957478750989 ) ) ;
#5497=CARTESIAN_POINT ( 'NONE',  ( 7.762960416026701616, 12.60702317161859121, -221.9096828323375235 ) ) ;
#5499=CARTESIAN_POINT ( 'NONE',  ( -5.420780812268581883, -12.08122409751860360, -226.5143039284326392 ) ) ;
#5500=CARTESIAN_POINT ( 'NONE',  ( 10.99893791904045415, -12.61823049403341201, -218.3266956685045841 ) ) ;
#5503=CARTESIAN_POINT ( 'NONE',  ( -13.55637112341987383, 4.614880311503475774, -231.8130385267184010 ) ) ;
#5504=CARTESIAN_POINT ( 'NONE',  ( -17.58891219272264905, -6.833323493373833379, -229.9407564095759540 ) ) ;
#5506=AXIS2_PLACEMENT_3D ( 'NONE', #13365, #9767, #16416 ) ;
#5507=CARTESIAN_POINT ( 'NONE',  ( 24.52160379727246209, 5.049198597839295033, -215.7868787176665535 ) ) ;
#5508=CARTESIAN_POINT ( 'NONE',  ( 2.535512286608554433, 13.86868953312499109, -224.9313928733152181 ) ) ;
#5509=CARTESIAN_POINT ( 'NONE',  ( 2.601379523478754674, 17.36677895276155681, -230.4357129074444117 ) ) ;
#5510=ORIENTED_EDGE ( 'NONE', *, *, #13136, .T. ) ;
#5511=CARTESIAN_POINT ( 'NONE',  ( 20.22673842361927399, -24.21895433676095877, -222.6595898022596316 ) ) ;
#5513=CARTESIAN_POINT ( 'NONE',  ( 12.85408565574548412, 7.821283853063205171, -223.1248833997948111 ) ) ;
#5514=CARTESIAN_POINT ( 'NONE',  ( -17.15943377049709184, 17.77880916606822836, -233.2929083076029144 ) ) ;
#5515=CARTESIAN_POINT ( 'NONE',  ( -21.01482965301294925, 6.368220028842532798, -231.7530032521518990 ) ) ;
#5516=CARTESIAN_POINT ( 'NONE',  ( -14.76610802599379291, -3.249507257478274180, -230.1617063156812719 ) ) ;
#5517=CARTESIAN_POINT ( 'NONE',  ( -23.49379658590067876, 11.46840048879614393, -217.2519070826072323 ) ) ;
#5522=CARTESIAN_POINT ( 'NONE',  ( -12.80756961294691010, 26.82110654133967387, -223.7464923486294026 ) ) ;
#5523=CARTESIAN_POINT ( 'NONE',  ( 22.92330650806121639, 19.11387742755395180, -231.6463539987045976 ) ) ;
#5524=CARTESIAN_POINT ( 'NONE',  ( 18.69835413980967687, -1.262199651413310031, -230.6153330080101966 ) ) ;
#5525=CARTESIAN_POINT ( 'NONE',  ( -15.10499565381530118, -6.968761303117489980, -233.6783966751926869 ) ) ;
#5526=CARTESIAN_POINT ( 'NONE',  ( -23.63383474287343589, -9.908731599815467916, -232.6396219513094081 ) ) ;
#5527=CARTESIAN_POINT ( 'NONE',  ( -12.22073052649759184, 14.03927388329973525, -215.9097966823721606 ) ) ;
#5528=CARTESIAN_POINT ( 'NONE',  ( -6.052919920376759855, -15.38051382379660836, -218.0337201863237624 ) ) ;
#5529=CARTESIAN_POINT ( 'NONE',  ( 7.639528166734322667, 11.92751229241157596, -224.6077814063189635 ) ) ;
#5530=CARTESIAN_POINT ( 'NONE',  ( 4.433847066018189231, -14.70588125837090487, -232.6468564462760469 ) ) ;
#5533=CARTESIAN_POINT ( 'NONE',  ( -15.36327147092456791, 5.453733681707060299, -220.0043800961136355 ) ) ;
#5534=FILL_AREA_STYLE ('',( #14221 ) ) ;
#5535=CARTESIAN_POINT ( 'NONE',  ( -8.752190949579933488, 24.25633523490762755, -230.6624101830059885 ) ) ;
#5536=CARTESIAN_POINT ( 'NONE',  ( -27.92885697401080591, 6.962042978589167319, -220.9552227796709190 ) ) ;
#5537=CARTESIAN_POINT ( 'NONE',  ( 18.04365516558436866, 6.721233635139160612, -218.4376093631473168 ) ) ;
#5538=CARTESIAN_POINT ( 'NONE',  ( 24.49559427486850893, 14.86117239466233642, -230.3058416388274736 ) ) ;
#5539=CARTESIAN_POINT ( 'NONE',  ( -7.879270980303660465, -15.58863178937888350, -218.8267223810934752 ) ) ;
#5540=CARTESIAN_POINT ( 'NONE',  ( 18.99256614858759207, 26.22894869843687715, -224.5811130452664202 ) ) ;
#5543=CARTESIAN_POINT ( 'NONE',  ( -11.08668407991722304, -24.47826551258279082, -233.9784602105897875 ) ) ;
#5544=CARTESIAN_POINT ( 'NONE',  ( -14.87932799058895128, 18.71706570923887369, -231.8731726670167745 ) ) ;
#5546=CARTESIAN_POINT ( 'NONE',  ( 11.98894270675143225, 20.38243841428667835, -233.2283128908360084 ) ) ;
#5547=CARTESIAN_POINT ( 'NONE',  ( -18.67270963783218463, 15.11229250701181925, -218.9067109956068578 ) ) ;
#5548=CARTESIAN_POINT ( 'NONE',  ( 2.660414182604129429, 28.99288898680367055, -232.5781547115647072 ) ) ;
#5549=CARTESIAN_POINT ( 'NONE',  ( 25.40954707198727647, 2.077273811637330159, -219.3610170479527426 ) ) ;
#5551=CARTESIAN_POINT ( 'NONE',  ( 12.31709745011784740, -23.08055702692190891, -220.7960250479738136 ) ) ;
#5553=CARTESIAN_POINT ( 'NONE',  ( 7.739744183733028748, -12.54214339878522999, -227.5419174737939159 ) ) ;
#5554=CARTESIAN_POINT ( 'NONE',  ( -1.796846813493219619, 26.08418332695505271, -220.7262848173578504 ) ) ;
#5558=CARTESIAN_POINT ( 'NONE',  ( 18.76922974182421555, 13.12635134380198210, -217.8010375391909008 ) ) ;
#5559=CARTESIAN_POINT ( 'NONE',  ( 17.00614511541963836, -1.958782916976874233, -219.4638360731791806 ) ) ;
#5560=CARTESIAN_POINT ( 'NONE',  ( -16.05483997570105714, -7.226811045751038165, -218.5819178105544438 ) ) ;
#5561=CARTESIAN_POINT ( 'NONE',  ( 2.967317674205219191, -16.40215926535219282, -217.6245344443522924 ) ) ;
#5563=CARTESIAN_POINT ( 'NONE',  ( -8.467651734177735534, 23.23776955534497546, -231.2693664226804913 ) ) ;
#5565=CARTESIAN_POINT ( 'NONE',  ( 21.91535456744164279, 7.573568724377624406, -232.0371228855588868 ) ) ;
#5566=CARTESIAN_POINT ( 'NONE',  ( -9.250876228778270871, 9.538614635316015722, -227.1332118982684563 ) ) ;
#5567=CARTESIAN_POINT ( 'NONE',  ( -7.058999618647554541, 24.62458660126260312, -219.6630466582859356 ) ) ;
#5569=CARTESIAN_POINT ( 'NONE',  ( 3.219568897812384645, 28.82511222849302257, -221.5626884747494216 ) ) ;
#5570=CARTESIAN_POINT ( 'NONE',  ( -17.99155049254074612, 5.190958499132906745, -220.1449419322306937 ) ) ;
#5571=CARTESIAN_POINT ( 'NONE',  ( 22.66015888791822519, 10.43487984001084534, -234.3950629709119937 ) ) ;
#5572=CARTESIAN_POINT ( 'NONE',  ( 11.75796858304313375, -24.75965012883946414, -219.8219186532837455 ) ) ;
#5575=CARTESIAN_POINT ( 'NONE',  ( 12.18657022793382794, 26.76558097653315471, -221.8882195427397335 ) ) ;
#5576=CARTESIAN_POINT ( 'NONE',  ( 23.43833711860394686, -7.060024820847174531, -230.3984000052215606 ) ) ;
#5578=CARTESIAN_POINT ( 'NONE',  ( 15.05360126642391450, 1.481754003466396963, -222.9454997252120734 ) ) ;
#5581=CARTESIAN_POINT ( 'NONE',  ( 1.541778504653760429, -23.48174737203985529, -233.9922866444541967 ) ) ;
#5583=CARTESIAN_POINT ( 'NONE',  ( -9.740348021262962064, 16.12529029871877384, -216.4361617420699702 ) ) ;
#5584=CARTESIAN_POINT ( 'NONE',  ( -13.41298582792616934, 27.85383138489214616, -228.6457525465575884 ) ) ;
#5586=CARTESIAN_POINT ( 'NONE',  ( -28.59157645096996347, 5.137867505054540374, -220.4667042235044505 ) ) ;
#5587=CARTESIAN_POINT ( 'NONE',  ( -13.08346052978740914, -7.620079078745922274, -220.3923444982454498 ) ) ;
#5590=CARTESIAN_POINT ( 'NONE',  ( -26.74045434827795020, 12.41518252455047744, -220.4617428697642652 ) ) ;
#5591=CARTESIAN_POINT ( 'NONE',  ( 7.717439423011566824, -15.08909893080012132, -230.2794769249191518 ) ) ;
#5593=CARTESIAN_POINT ( 'NONE',  ( 28.52435124311170966, 7.611291969169514005, -224.8315247833735384 ) ) ;
#5594=CARTESIAN_POINT ( 'NONE',  ( -7.099035520468861549, 19.73710792467281649, -233.8745459908100770 ) ) ;
#5596=CARTESIAN_POINT ( 'NONE',  ( 12.16813927252146144, 18.27141895336136912, -230.9123895730235745 ) ) ;
#5597=CARTESIAN_POINT ( 'NONE',  ( 3.610394173775429039, -14.27701378914486874, -220.9234757326916281 ) ) ;
#5599=CARTESIAN_POINT ( 'NONE',  ( 2.464084843620814702, 29.35663482419208492, -227.0015060686748143 ) ) ;
#5600=CARTESIAN_POINT ( 'NONE',  ( -9.222253059793434460, 13.27185325399938165, -229.0864811363590547 ) ) ;
#5601=CARTESIAN_POINT ( 'NONE',  ( -18.16160515720599022, 12.42447964075808997, -216.1086293678848449 ) ) ;
#5602=CARTESIAN_POINT ( 'NONE',  ( -18.79436262126649027, -19.56097393442729526, -222.1480387859219547 ) ) ;
#5605=CARTESIAN_POINT ( 'NONE',  ( 22.05207439088920651, 1.190718621721708947, -218.4927357815377604 ) ) ;
#5606=CARTESIAN_POINT ( 'NONE',  ( 8.467778565514151978, -25.57602835425881338, -228.7153423394380525 ) ) ;
#5607=CARTESIAN_POINT ( 'NONE',  ( 15.89706143421296147, 10.57416387607782227, -218.3862415393350318 ) ) ;
#5609=CARTESIAN_POINT ( 'NONE',  ( -21.02719846458807851, 18.12262440796364871, -218.0220709499931502 ) ) ;
#5611=CARTESIAN_POINT ( 'NONE',  ( 29.21307215008108216, 4.139194015751272104, -229.9658791484231699 ) ) ;
#5613=CARTESIAN_POINT ( 'NONE',  ( 0.9046320824004248085, 13.39785254849979701, -226.4815711199935890 ) ) ;
#5614=CARTESIAN_POINT ( 'NONE',  ( 15.34286276367735979, 1.557318373440422565, -222.4358706187587416 ) ) ;
#5615=CARTESIAN_POINT ( 'NONE',  ( -20.76924187596804217, -21.50248317380421170, -228.3679492147379335 ) ) ;
#5616=CARTESIAN_POINT ( 'NONE',  ( 13.49882595795384255, -9.201056071450322449, -219.2439763087855908 ) ) ;
#5619=CARTESIAN_POINT ( 'NONE',  ( -7.903959818038710061, 11.02445096303677552, -229.5951168968472871 ) ) ;
#5620=CARTESIAN_POINT ( 'NONE',  ( -14.79915263310685347, -6.493660518011266092, -224.0818296219458716 ) ) ;
#5621=CARTESIAN_POINT ( 'NONE',  ( -16.28025842329327944, 6.985656672962045732, -231.4191468057695715 ) ) ;
#5622=CARTESIAN_POINT ( 'NONE',  ( 23.21336156720804667, 12.57464006230432574, -232.9346648124233070 ) ) ;
#5623=CARTESIAN_POINT ( 'NONE',  ( 5.549682179574114471, 15.11687613544382280, -226.9959476502473308 ) ) ;
#5625=CARTESIAN_POINT ( 'NONE',  ( 10.56552815906878529, -5.142824638143381755, -223.3550139360156663 ) ) ;
#5627=CARTESIAN_POINT ( 'NONE',  ( 27.04607490430786854, 4.607450003618843049, -220.3758934308003461 ) ) ;
#5628=CARTESIAN_POINT ( 'NONE',  ( -22.70558257617108922, 14.65737936663030538, -230.9775454010380997 ) ) ;
#5630=CARTESIAN_POINT ( 'NONE',  ( -8.995433708001568718, 13.44373928221519243, -231.9251680978426577 ) ) ;
#5631=CARTESIAN_POINT ( 'NONE',  ( -26.47652094774193188, -8.527600130219385122, -218.5932275281782324 ) ) ;
#5632=CARTESIAN_POINT ( 'NONE',  ( -25.61997837663875188, 10.01664178086244483, -231.6711741719404074 ) ) ;
#5634=CARTESIAN_POINT ( 'NONE',  ( 12.23284375931666013, 4.108221165122169616, -224.0993108960438462 ) ) ;
#5635=CARTESIAN_POINT ( 'NONE',  ( -12.66290653391502907, 23.44312233264792411, -230.9359094203250606 ) ) ;
#5636=CARTESIAN_POINT ( 'NONE',  ( 5.434119414999338815, 11.18343085245738777, -221.0450680983404936 ) ) ;
#5637=CARTESIAN_POINT ( 'NONE',  ( 22.05207439088920651, 1.190718621721708947, -218.4927357815377604 ) ) ;
#5638=CARTESIAN_POINT ( 'NONE',  ( -24.78729321827560739, -16.46449136890227294, -222.3867555963062443 ) ) ;
#5639=CARTESIAN_POINT ( 'NONE',  ( 3.755480357635514022, 24.23367984900377436, -231.4105847235276201 ) ) ;
#5640=CARTESIAN_POINT ( 'NONE',  ( 0.5120693878963755719, -30.63998626839889639, -227.9504769009175220 ) ) ;
#5641=CARTESIAN_POINT ( 'NONE',  ( 17.60676319847677007, 21.31475060840986302, -219.8266339603936785 ) ) ;
#5642=CARTESIAN_POINT ( 'NONE',  ( 21.11934605992122727, -20.14300392389669270, -232.3867613253685249 ) ) ;
#5644=CARTESIAN_POINT ( 'NONE',  ( -22.38347148959098121, 12.58966534755613687, -218.4978713241202399 ) ) ;
#5646=CARTESIAN_POINT ( 'NONE',  ( 27.54201077264015396, -3.286392687948289648, -218.1575117614944190 ) ) ;
#5647=CARTESIAN_POINT ( 'NONE',  ( 11.39755372583812587, 20.40856199875060639, -231.2895618162029621 ) ) ;
#5648=CARTESIAN_POINT ( 'NONE',  ( 22.16327814861754675, 7.634676377199016706, -234.0520676664821735 ) ) ;
#5649=CARTESIAN_POINT ( 'NONE',  ( 16.07305932912010960, 0.9253679043337685872, -229.0409936706996064 ) ) ;
#5650=CARTESIAN_POINT ( 'NONE',  ( -7.475691298859681311, -12.42146568352542779, -226.9176918848390017 ) ) ;
#5652=CARTESIAN_POINT ( 'NONE',  ( 1.984991703947643904, 14.51738422979996912, -218.4500278854917781 ) ) ;
#5654=CARTESIAN_POINT ( 'NONE',  ( -7.108809775916832940, -10.55228017211132929, -220.3225562754048212 ) ) ;
#5655=CARTESIAN_POINT ( 'NONE',  ( -11.08731210905863840, 25.61052584666692766, -228.9953606804266997 ) ) ;
#5656=CARTESIAN_POINT ( 'NONE',  ( 14.60728983664449387, 19.38727400458104455, -216.6381802409380555 ) ) ;
#5658=CARTESIAN_POINT ( 'NONE',  ( -15.82760502346409304, 5.624826830110399634, -227.5369622385896946 ) ) ;
#5659=CARTESIAN_POINT ( 'NONE',  ( 4.065638640983322283, 32.08830473489500434, -226.0249194102539150 ) ) ;
#5660=CARTESIAN_POINT ( 'NONE',  ( 22.37138132874926910, 6.723028048925958622, -217.7073806909121743 ) ) ;
#5661=CARTESIAN_POINT ( 'NONE',  ( 10.17740660404977149, -19.92573511251913132, -219.0500883963018737 ) ) ;
#5662=CARTESIAN_POINT ( 'NONE',  ( 13.38323588254664642, -24.59169381177348157, -229.6955247737395780 ) ) ;
#5663=CARTESIAN_POINT ( 'NONE',  ( 0.1979841192334154676, 16.22068729745496540, -223.9539336445596973 ) ) ;
#5665=CARTESIAN_POINT ( 'NONE',  ( 15.01439307471096463, 1.118969480519667048, -226.7488225241675366 ) ) ;
#5666=CARTESIAN_POINT ( 'NONE',  ( 20.89700225552940793, -4.547446057044195911, -232.3806459760843666 ) ) ;
#5667=CARTESIAN_POINT ( 'NONE',  ( -18.44715843167851688, -19.86029123650958184, -231.9563062773970046 ) ) ;
#5668=CARTESIAN_POINT ( 'NONE',  ( -8.257247207528708444, -26.39349301559143512, -217.9383130379005138 ) ) ;
#5669=CARTESIAN_POINT ( 'NONE',  ( -2.806347010929339802, 19.90767250424812573, -230.9206976900916004 ) ) ;
#5671=CARTESIAN_POINT ( 'NONE',  ( 20.90058474538433231, 18.60939544422136294, -225.8027644507526475 ) ) ;
#5672=CARTESIAN_POINT ( 'NONE',  ( -9.517741096562200909, 20.63709896626785678, -234.1036702156204967 ) ) ;
#5673=CARTESIAN_POINT ( 'NONE',  ( -8.548213857283494477, 12.07277636836182211, -222.5354997492170241 ) ) ;
#5675=CARTESIAN_POINT ( 'NONE',  ( 3.846342036506673612, 16.55327908958690131, -231.1358846258000597 ) ) ;
#5676=CARTESIAN_POINT ( 'NONE',  ( 15.51129552754472307, 0.2180314803830030457, -231.3815478022924879 ) ) ;
#5677=CARTESIAN_POINT ( 'NONE',  ( 18.59615491886314231, -0.2392802120807639710, -217.5848846836084078 ) ) ;
#5678=CARTESIAN_POINT ( 'NONE',  ( 19.78534257568999166, -22.00365353819481840, -227.2618024355658974 ) ) ;
#5681=CARTESIAN_POINT ( 'NONE',  ( 7.762960416026701616, 12.60702317161859121, -221.9096828323375235 ) ) ;
#5682=CARTESIAN_POINT ( 'NONE',  ( 23.48259192634075632, -8.786327662478353062, -220.0176983167915807 ) ) ;
#5685=CARTESIAN_POINT ( 'NONE',  ( 7.088126259304779353, -19.25156530781288566, -233.7785425911077937 ) ) ;
#5687=CARTESIAN_POINT ( 'NONE',  ( -6.282398543089500187, 12.01615879894893801, -228.5121145169883903 ) ) ;
#5688=CARTESIAN_POINT ( 'NONE',  ( -17.15943377049709184, 17.77880916606822836, -233.2929083076029144 ) ) ;
#5689=CARTESIAN_POINT ( 'NONE',  ( -24.02434186778878455, 18.57431834865475651, -228.2662945587547370 ) ) ;
#5690=CARTESIAN_POINT ( 'NONE',  ( -12.65123680455331190, -6.798726433138870817, -228.2089845657881710 ) ) ;
#5693=CARTESIAN_POINT ( 'NONE',  ( -17.88126539071149779, 5.766250685202066961, -232.9050303536861293 ) ) ;
#5694=CARTESIAN_POINT ( 'NONE',  ( 7.470327549107519616, -12.61959153319410909, -223.5186783388273568 ) ) ;
#5696=CARTESIAN_POINT ( 'NONE',  ( -10.51143808951550085, 11.41308718311005066, -231.3573069600382439 ) ) ;
#5697=CARTESIAN_POINT ( 'NONE',  ( 27.94758519801750296, 7.894658480667867018, -227.3974864124137127 ) ) ;
#5699=CARTESIAN_POINT ( 'NONE',  ( -10.49339404011726984, 12.66576824096800991, -217.2681947942554643 ) ) ;
#5702=CARTESIAN_POINT ( 'NONE',  ( 16.49020573214642837, 22.44566021525517741, -224.7841662740084701 ) ) ;
#5703=CARTESIAN_POINT ( 'NONE',  ( -2.820113134979321590, -27.38213018110698727, -220.3670599055385821 ) ) ;
#5706=CARTESIAN_POINT ( 'NONE',  ( 3.192353461299334061, 22.13718518159985393, -217.1103300728619843 ) ) ;
#5707=CARTESIAN_POINT ( 'NONE',  ( -11.79656379827575918, 10.43402410864828589, -226.0519616335988076 ) ) ;
#5708=CARTESIAN_POINT ( 'NONE',  ( -20.80338291456855870, 18.97067006663518995, -230.9007617602332516 ) ) ;
#5709=CARTESIAN_POINT ( 'NONE',  ( -13.11077419447928349, -11.05578789306379406, -228.2719546787038212 ) ) ;
#5712=CARTESIAN_POINT ( 'NONE',  ( -14.68037037322036475, 3.441677802729143920, -220.1396515630443389 ) ) ;
#5713=CARTESIAN_POINT ( 'NONE',  ( 0.3833872033527188639, -14.95856321834011915, -223.3240416624371107 ) ) ;
#5714=CARTESIAN_POINT ( 'NONE',  ( 17.99029889091409018, 9.613712288440757092, -232.0298403238024036 ) ) ;
#5715=CARTESIAN_POINT ( 'NONE',  ( 2.837900457371055563, 25.11342719071438978, -232.9871906064174709 ) ) ;
#5716=CARTESIAN_POINT ( 'NONE',  ( -27.56397725925346975, 4.259055856374357241, -222.4951663284069241 ) ) ;
#5717=CARTESIAN_POINT ( 'NONE',  ( 4.340445191644851874, 29.86837761166362881, -227.4879512554873315 ) ) ;
#5719=CARTESIAN_POINT ( 'NONE',  ( -9.294226473174397540, -12.00440878504259601, -219.6990993854437875 ) ) ;
#5720=CARTESIAN_POINT ( 'NONE',  ( 15.11994912051959972, -12.48385213956034079, -232.8079920308188377 ) ) ;
#5723=CARTESIAN_POINT ( 'NONE',  ( -28.88770769694534479, 14.24820799418726480, -223.2044777450442155 ) ) ;
#5724=CARTESIAN_POINT ( 'NONE',  ( -14.98971194994906853, -6.742389346827670771, -223.0360336987919823 ) ) ;
#5725=CARTESIAN_POINT ( 'NONE',  ( -16.07193224038526580, 12.24477688577882439, -232.1409653212175499 ) ) ;
#5726=CARTESIAN_POINT ( 'NONE',  ( 26.59731715018858011, 13.56210517473685329, -229.5787264587298466 ) ) ;
#5727=CARTESIAN_POINT ( 'NONE',  ( -1.837924626891132229, 29.27703531260187475, -227.2344808100871774 ) ) ;
#5729=CARTESIAN_POINT ( 'NONE',  ( 9.478576170506354259, -9.424747406754709900, -230.1309108789951949 ) ) ;
#5730=CARTESIAN_POINT ( 'NONE',  ( 14.63113973005795643, 4.926264598692385199, -222.4866305912601945 ) ) ;
#5731=CARTESIAN_POINT ( 'NONE',  ( -0.3984245442872364484, 11.77931270252508789, -223.1826369159892920 ) ) ;
#5732=CIRCLE ( 'NONE', #21176, 1.000000000000000888 ) ;
#5733=CARTESIAN_POINT ( 'NONE',  ( -5.191169535941942748, 31.49570301054888688, -227.4714364261087098 ) ) ;
#5734=CARTESIAN_POINT ( 'NONE',  ( -25.32486352395475393, -3.505876693931964549, -233.0869506614649822 ) ) ;
#5735=CARTESIAN_POINT ( 'NONE',  ( -17.88126539071149779, 5.766250685202066961, -232.9050303536861293 ) ) ;
#5737=CARTESIAN_POINT ( 'NONE',  ( 23.36729170583618398, -5.500043712341283531, -232.1593072787115375 ) ) ;
#5739=CARTESIAN_POINT ( 'NONE',  ( -0.9851030586975465519, 19.34066537597387381, -233.8273485600932418 ) ) ;
#5740=CARTESIAN_POINT ( 'NONE',  ( 29.08100487150598212, 12.14819438347179670, -226.9621620069135020 ) ) ;
#5741=CARTESIAN_POINT ( 'NONE',  ( -25.29098058636142810, 5.014641116111857144, -217.4658967307323110 ) ) ;
#5742=CARTESIAN_POINT ( 'NONE',  ( 15.85665641241444668, 18.24713744004561988, -217.7195292979064902 ) ) ;
#5743=CARTESIAN_POINT ( 'NONE',  ( -28.57583275380518018, -9.842401781236429059, -222.4643230566485386 ) ) ;
#5744=CARTESIAN_POINT ( 'NONE',  ( -2.665457046508036942, 16.94988614842223029, -218.7621057649994896 ) ) ;
#5745=CARTESIAN_POINT ( 'NONE',  ( -5.420780812268581883, -12.08122409751860360, -226.5143039284326392 ) ) ;
#5746=CARTESIAN_POINT ( 'NONE',  ( 9.586902571418640662, 24.43292817174309661, -231.9968623198229807 ) ) ;
#5747=CARTESIAN_POINT ( 'NONE',  ( 3.784839621866231241, -12.46827349529254469, -229.8854786719440426 ) ) ;
#5749=CARTESIAN_POINT ( 'NONE',  ( -23.20103936322198024, 10.64725167743880085, -231.7714206262400864 ) ) ;
#5751=CARTESIAN_POINT ( 'NONE',  ( -27.94976817795961210, -4.610981384744690104, -229.1808304932418139 ) ) ;
#5752=CARTESIAN_POINT ( 'NONE',  ( 3.433394806375676733, 19.92272173529517332, -219.3341428536850799 ) ) ;
#5753=CARTESIAN_POINT ( 'NONE',  ( -16.74094048923576494, 16.03040267675914521, -217.9177456399057178 ) ) ;
#5754=CARTESIAN_POINT ( 'NONE',  ( 28.51464931495100785, 5.422321182929326966, -223.8116416110474347 ) ) ;
#5755=CARTESIAN_POINT ( 'NONE',  ( -12.44262610342426711, -20.67338498558408588, -232.3867413080560027 ) ) ;
#5756=CARTESIAN_POINT ( 'NONE',  ( 24.19672885113291727, 10.99915907690374439, -233.6834417629405891 ) ) ;
#5758=CARTESIAN_POINT ( 'NONE',  ( -11.83854910565153062, -9.589341273415847411, -217.2594489226254098 ) ) ;
#5759=CARTESIAN_POINT ( 'NONE',  ( 2.508382434586714282, 15.09451298870656011, -220.9010239894319625 ) ) ;
#5760=CARTESIAN_POINT ( 'NONE',  ( 5.833753951408669813, 12.47745132051510453, -226.2508980627489450 ) ) ;
#5762=CARTESIAN_POINT ( 'NONE',  ( -13.01542355754912172, 26.77630951171455820, -225.1545229496516356 ) ) ;
#5763=CARTESIAN_POINT ( 'NONE',  ( -0.2269548806647709305, 12.31484924552052718, -228.6688778050056783 ) ) ;
#5764=CARTESIAN_POINT ( 'NONE',  ( 23.64727379217503866, 9.907944788639682088, -232.0643337313508709 ) ) ;
#5765=CARTESIAN_POINT ( 'NONE',  ( 7.956221944547102964, -16.14435353399512252, -220.6073666753051441 ) ) ;
#5766=CARTESIAN_POINT ( 'NONE',  ( 6.260833139380572732, -16.02228513277848876, -219.5457089733663736 ) ) ;
#5767=CARTESIAN_POINT ( 'NONE',  ( -6.564517230509238743, 23.65597541655194647, -219.1225629381441991 ) ) ;
#5770=CARTESIAN_POINT ( 'NONE',  ( 14.22574309452842733, 4.476723532073429546, -225.5862451792618231 ) ) ;
#5771=CARTESIAN_POINT ( 'NONE',  ( 14.90979066288448429, -1.927202206923867234, -222.7790985701595616 ) ) ;
#5772=CARTESIAN_POINT ( 'NONE',  ( -14.78079095050690661, -5.416970230978240153, -229.7193632018645246 ) ) ;
#5773=CARTESIAN_POINT ( 'NONE',  ( 1.780803752597676537, -13.83832444325970101, -229.2250779460899537 ) ) ;
#5774=CARTESIAN_POINT ( 'NONE',  ( 6.608541902967795423, 16.43938546752961116, -220.2982508316308952 ) ) ;
#5776=CARTESIAN_POINT ( 'NONE',  ( -11.78887577478644566, 1.715692547334320084, -224.3106172711415525 ) ) ;
#5777=CARTESIAN_POINT ( 'NONE',  ( -14.73016414256368911, 22.23431809695627237, -217.1425123644553707 ) ) ;
#5778=CARTESIAN_POINT ( 'NONE',  ( 3.281983756374524663, 15.83593597903271721, -223.8697822987047346 ) ) ;
#5779=CARTESIAN_POINT ( 'NONE',  ( 29.76850351104168979, -8.061840962539296385, -221.9850081079297581 ) ) ;
#5783=CARTESIAN_POINT ( 'NONE',  ( 13.20340559785743828, 9.575208899273587093, -218.1210831379648312 ) ) ;
#5784=CARTESIAN_POINT ( 'NONE',  ( -14.47418542577149836, 8.806675964858893479, -228.0010566307936699 ) ) ;
#5785=CARTESIAN_POINT ( 'NONE',  ( 13.70635042947887428, -1.390919209824193592, -225.3477037409554953 ) ) ;
#5786=CARTESIAN_POINT ( 'NONE',  ( -1.432270239486107766, -17.91381153981195951, -219.1344183636291802 ) ) ;
#5789=CARTESIAN_POINT ( 'NONE',  ( 4.389496648589924277, 14.47660514356954131, -220.6151178996808540 ) ) ;
#5790=CARTESIAN_POINT ( 'NONE',  ( 25.46431111394153390, -2.048831322092446783, -230.3135391428295975 ) ) ;
#5792=CARTESIAN_POINT ( 'NONE',  ( -0.8413160509385254615, -28.71376977722865931, -218.8117683208458288 ) ) ;
#5794=CARTESIAN_POINT ( 'NONE',  ( -13.83274569775339202, 16.20364235096346661, -234.0851861771356539 ) ) ;
#5795=CARTESIAN_POINT ( 'NONE',  ( -5.543543819386913540, 14.51457927969963713, -217.3847528063896846 ) ) ;
#5796=CARTESIAN_POINT ( 'NONE',  ( -13.55591840520136770, 8.363404288414606924, -231.2690188357804857 ) ) ;
#5797=CARTESIAN_POINT ( 'NONE',  ( -19.65071121466273496, -22.30814805266854606, -225.1308016072272267 ) ) ;
#5800=CARTESIAN_POINT ( 'NONE',  ( -5.807479211365208727, 19.77444019604324410, -216.0778658752277863 ) ) ;
#5801=CARTESIAN_POINT ( 'NONE',  ( 3.085658278449291192, -27.83354332032029888, -231.5475985764057043 ) ) ;
#5803=CARTESIAN_POINT ( 'NONE',  ( -15.82069055112642353, 8.315535108674763976, -217.2800172218543935 ) ) ;
#5805=CARTESIAN_POINT ( 'NONE',  ( -18.09994298044773942, 1.383435435878707320, -215.7801353739235708 ) ) ;
#5806=CARTESIAN_POINT ( 'NONE',  ( -1.707778556226592581, 19.51307486516442680, -232.5708079709245055 ) ) ;
#5807=CARTESIAN_POINT ( 'NONE',  ( 13.55929460187270053, 0.3562519042583365270, -227.9787723277739246 ) ) ;
#5808=CARTESIAN_POINT ( 'NONE',  ( 20.59763700141659015, 7.383112456150029423, -232.0722244125682039 ) ) ;
#5809=CARTESIAN_POINT ( 'NONE',  ( -11.76273268715550913, -21.77324546118368787, -230.3967548854103313 ) ) ;
#5810=EDGE_CURVE ( 'NONE', #7856, #13407, #365, .T. ) ;
#5812=CARTESIAN_POINT ( 'NONE',  ( -4.855966894080006035, 26.75753167227873064, -230.1547293463117114 ) ) ;
#5813=CARTESIAN_POINT ( 'NONE',  ( -9.007976471255481954, 12.60968992764439633, -227.9367755778692981 ) ) ;
#5814=CARTESIAN_POINT ( 'NONE',  ( -20.04070223234628756, 18.12164545743767263, -231.9292141396248610 ) ) ;
#5817=CARTESIAN_POINT ( 'NONE',  ( -12.84507615163359873, -10.94093879717347129, -227.8208865714805142 ) ) ;
#5820=CARTESIAN_POINT ( 'NONE',  ( -26.02440924314744919, 2.824604386891162111, -232.0644005296583430 ) ) ;
#5821=CARTESIAN_POINT ( 'NONE',  ( 2.864019721262919926, -25.46936398327173379, -230.7696170053991978 ) ) ;
#5822=CARTESIAN_POINT ( 'NONE',  ( 15.33737796850231305, 13.57479350230705428, -232.3313557812109025 ) ) ;
#5823=CARTESIAN_POINT ( 'NONE',  ( 0.9046320824004248085, 13.39785254849979701, -226.4815711199935890 ) ) ;
#5826=CARTESIAN_POINT ( 'NONE',  ( -25.19195624009214640, 10.50676406307063182, -220.0954552869889937 ) ) ;
#5827=CARTESIAN_POINT ( 'NONE',  ( 15.88965480228581839, 12.37830464553330678, -233.8570207506254235 ) ) ;
#5829=CARTESIAN_POINT ( 'NONE',  ( 14.54149994592679107, 8.070685273005897997, -229.7292930672863349 ) ) ;
#5831=CARTESIAN_POINT ( 'NONE',  ( -12.14186164972853810, -9.217338937739926408, -220.4665480714278374 ) ) ;
#5832=CARTESIAN_POINT ( 'NONE',  ( 1.836136847161299990, -12.84546502099244591, -226.1727064218434293 ) ) ;
#5835=CARTESIAN_POINT ( 'NONE',  ( -4.450022810944913587, 12.45400981846350597, -225.2098051417536340 ) ) ;
#5836=CARTESIAN_POINT ( 'NONE',  ( 22.41656803062015157, -8.700679067278056067, -214.8043567724421337 ) ) ;
#5837=CARTESIAN_POINT ( 'NONE',  ( 10.12956299421491302, 11.38773431477224385, -230.3175791991728829 ) ) ;
#5838=CARTESIAN_POINT ( 'NONE',  ( 8.856360819293511710, 14.24139612884802553, -227.7731680686805475 ) ) ;
#5840=CARTESIAN_POINT ( 'NONE',  ( 10.41909793732091494, -5.130961835214151279, -225.2553394319931783 ) ) ;
#5841=CARTESIAN_POINT ( 'NONE',  ( 20.23125423326388628, 7.836699765464857137, -217.8891354894872450 ) ) ;
#5843=CARTESIAN_POINT ( 'NONE',  ( -5.568057711815838751, 28.69723585065299076, -232.1518503103610271 ) ) ;
#5844=CARTESIAN_POINT ( 'NONE',  ( -7.812160407601123069, 10.19183344000749081, -223.8148904943605828 ) ) ;
#5845=CARTESIAN_POINT ( 'NONE',  ( -16.30907414568449454, -3.310091733494833655, -231.8954501777161283 ) ) ;
#5846=CARTESIAN_POINT ( 'NONE',  ( -18.09776816382430908, 23.50806826204562583, -229.9568677523880638 ) ) ;
#5848=CARTESIAN_POINT ( 'NONE',  ( 27.36047156164216787, -8.591464759722228450, -221.3690063136810977 ) ) ;
#5849=CARTESIAN_POINT ( 'NONE',  ( -6.496078068315311427, 23.46891392553531119, -233.1042179568201220 ) ) ;
#5850=CARTESIAN_POINT ( 'NONE',  ( 29.33969601628096768, 11.98971187598327504, -225.2039690377576733 ) ) ;
#5851=CARTESIAN_POINT ( 'NONE',  ( -12.44873260470819787, 7.411970124596155785, -229.4214091473984070 ) ) ;
#5852=CARTESIAN_POINT ( 'NONE',  ( 11.82943521288609823, 27.58963564415041247, -226.1180395413371400 ) ) ;
#5856=CARTESIAN_POINT ( 'NONE',  ( -1.316322971969275502, 14.13179993441458215, -224.9782367179667233 ) ) ;
#5857=CARTESIAN_POINT ( 'NONE',  ( -13.67406442719345883, -9.319000780081536206, -231.1492214949047934 ) ) ;
#5858=CARTESIAN_POINT ( 'NONE',  ( 8.689059922489732912, 15.18271246186214363, -218.7354841152034908 ) ) ;
#5859=CARTESIAN_POINT ( 'NONE',  ( 6.910796951316678260, -9.495606915386650471, -226.6778026831113380 ) ) ;
#5861=CARTESIAN_POINT ( 'NONE',  ( -18.94992041651601156, 14.87246523864368974, -232.0280096192260828 ) ) ;
#5862=CARTESIAN_POINT ( 'NONE',  ( 24.57161139520042781, -7.530326316930160857, -232.9949629211864419 ) ) ;
#5863=CARTESIAN_POINT ( 'NONE',  ( 7.508136856874425114, 24.19512352541684663, -230.0608033085341617 ) ) ;
#5864=CARTESIAN_POINT ( 'NONE',  ( -15.11329978779464689, 11.41628732213579411, -231.7124318929555500 ) ) ;
#5865=CARTESIAN_POINT ( 'NONE',  ( -15.57331739480619248, 4.297375044201914740, -216.4079605712025511 ) ) ;
#5866=CARTESIAN_POINT ( 'NONE',  ( -20.91998163778511355, -19.58520498255836628, -224.2692832511962990 ) ) ;
#5867=CARTESIAN_POINT ( 'NONE',  ( 17.65694480011521250, 15.62497337860048674, -235.2008064134603273 ) ) ;
#5871=CARTESIAN_POINT ( 'NONE',  ( -15.80613518906033121, -10.93105391054944597, -234.9065563738643903 ) ) ;
#5872=CARTESIAN_POINT ( 'NONE',  ( -4.224287562409271501, 29.03635716824519264, -224.1823526280761882 ) ) ;
#5874=CARTESIAN_POINT ( 'NONE',  ( 13.30790133003807441, 0.6370684082013071681, -222.3495379725305270 ) ) ;
#5875=CARTESIAN_POINT ( 'NONE',  ( -8.985448925281199095, 11.82743561134668475, -224.1067108988273162 ) ) ;
#5877=CARTESIAN_POINT ( 'NONE',  ( -4.619644865335168049, 14.75104250038670450, -232.3086264397671812 ) ) ;
#5878=CARTESIAN_POINT ( 'NONE',  ( -15.23434562258889891, -0.4010941804143903222, -220.4743703065900036 ) ) ;
#5880=CARTESIAN_POINT ( 'NONE',  ( -4.241635020808209866, -19.61639137582426429, -216.9458228475819226 ) ) ;
#5882=CARTESIAN_POINT ( 'NONE',  ( 11.12240951639491549, -23.90857633046665853, -218.9373339142375130 ) ) ;
#5884=CARTESIAN_POINT ( 'NONE',  ( 22.66390650824515873, 11.48342577402021725, -231.3155567808436217 ) ) ;
#5885=CARTESIAN_POINT ( 'NONE',  ( 29.12543877365354916, -1.475122899492763873, -224.0746120762670444 ) ) ;
#5886=CARTESIAN_POINT ( 'NONE',  ( -8.491902988188710921, -10.37035003683405066, -223.9502466269643435 ) ) ;
#5887=CARTESIAN_POINT ( 'NONE',  ( -18.64257584594551531, -16.66392856591270899, -217.1407738418131999 ) ) ;
#5888=CARTESIAN_POINT ( 'NONE',  ( 4.152856881432678726, 16.71326706899027670, -228.3712188091315909 ) ) ;
#5890=CARTESIAN_POINT ( 'NONE',  ( -15.00242079508237936, 7.335218745534954898, -232.9526071471669013 ) ) ;
#5892=CARTESIAN_POINT ( 'NONE',  ( -11.33137429837660193, 27.25022425932026238, -230.1650924901870212 ) ) ;
#5893=CARTESIAN_POINT ( 'NONE',  ( -2.993956627714193353, 22.04778837082692178, -231.1741803919495339 ) ) ;
#5894=CARTESIAN_POINT ( 'NONE',  ( 27.04962740251871978, -7.854494666110665158, -217.8595067830158882 ) ) ;
#5895=ORIENTED_EDGE ( 'NONE', *, *, #18322, .T. ) ;
#5896=CARTESIAN_POINT ( 'NONE',  ( 10.88376588832297287, 7.577514201227793400, -222.7215714477710833 ) ) ;
#5898=CARTESIAN_POINT ( 'NONE',  ( -15.77374768176864173, 20.07639682234129097, -218.6858893794192795 ) ) ;
#5899=CARTESIAN_POINT ( 'NONE',  ( 11.17228388010293649, 5.622653638471959425, -222.3672781564363845 ) ) ;
#5900=CARTESIAN_POINT ( 'NONE',  ( 0.2799207934783670693, -28.72270877262613453, -227.3216717588132667 ) ) ;
#5903=CARTESIAN_POINT ( 'NONE',  ( 7.639528166734322667, 11.92751229241157596, -224.6077814063189635 ) ) ;
#5904=CARTESIAN_POINT ( 'NONE',  ( 17.50516624540364319, -11.67908417450482794, -218.9956384138364740 ) ) ;
#5906=CARTESIAN_POINT ( 'NONE',  ( -15.46269062504165781, -26.67469327287815517, -225.2085449711190677 ) ) ;
#5908=CARTESIAN_POINT ( 'NONE',  ( 5.248230734842167955, 23.54336384919183445, -216.8914391693808739 ) ) ;
#5910=CARTESIAN_POINT ( 'NONE',  ( 4.213939275857851108, 16.79797086795582928, -215.8378124706958943 ) ) ;
#5912=CARTESIAN_POINT ( 'NONE',  ( -12.74846050492543625, 19.93509882904884734, -216.0172840992881049 ) ) ;
#5913=CARTESIAN_POINT ( 'NONE',  ( -14.01584329375060456, -3.774282517739922405, -220.6818330080343173 ) ) ;
#5916=CARTESIAN_POINT ( 'NONE',  ( -15.66530208164916260, 23.23467148471576849, -218.1250122661128046 ) ) ;
#5917=CARTESIAN_POINT ( 'NONE',  ( 3.671249956548685578, -18.86103685443826805, -233.0640024924723548 ) ) ;
#5919=CARTESIAN_POINT ( 'NONE',  ( -22.04257564474043818, 18.72061943465525857, -219.1781831295219263 ) ) ;
#5920=CARTESIAN_POINT ( 'NONE',  ( 22.24262848503957812, 2.205713500382371794, -232.7243927205662430 ) ) ;
#5921=CARTESIAN_POINT ( 'NONE',  ( 5.720314275582434327, 25.17872937134267630, -219.7530083620574430 ) ) ;
#5923=CARTESIAN_POINT ( 'NONE',  ( 14.04819512851487673, 6.831178966487911453, -222.6676118107292552 ) ) ;
#5924=CARTESIAN_POINT ( 'NONE',  ( -9.501265986711061373, -18.16888683615402300, -230.9326763462221948 ) ) ;
#5926=CARTESIAN_POINT ( 'NONE',  ( 17.31940731551425827, 24.90170669671083914, -222.9868986272316533 ) ) ;
#5927=CARTESIAN_POINT ( 'NONE',  ( -6.255852670334142829, 13.96671599789818252, -220.4426911866496823 ) ) ;
#5928=CARTESIAN_POINT ( 'NONE',  ( -11.05707385098054729, 9.265475627845670914, -220.9763772784480693 ) ) ;
#5929=CARTESIAN_POINT ( 'NONE',  ( 29.82766783012230505, -1.714217446056379934, -229.3564438616236316 ) ) ;
#5932=ORIENTED_EDGE ( 'NONE', *, *, #5810, .T. ) ;
#5933=CARTESIAN_POINT ( 'NONE',  ( 15.57986488780344736, -0.6155558446892130942, -225.2777919203616932 ) ) ;
#5934=CARTESIAN_POINT ( 'NONE',  ( -7.509561119170069077, -14.53281319394193538, -217.7574163112487042 ) ) ;
#5935=CARTESIAN_POINT ( 'NONE',  ( 14.38487221378403014, 1.734196266254829588, -227.4481254949095330 ) ) ;
#5936=CARTESIAN_POINT ( 'NONE',  ( 2.008896548638861024, 20.64812324442097591, -233.5818019448501843 ) ) ;
#5938=CARTESIAN_POINT ( 'NONE',  ( -24.05551141223569545, 2.266836731622281498, -230.7594878221277384 ) ) ;
#5940=CARTESIAN_POINT ( 'NONE',  ( 7.739849882373770917, 11.59357455229016409, -219.5521933286238720 ) ) ;
#5941=CARTESIAN_POINT ( 'NONE',  ( 26.29894631880581812, 12.29609390142961090, -226.3100047295820332 ) ) ;
#5943=CARTESIAN_POINT ( 'NONE',  ( -24.53655852862112496, -9.573911656693818273, -234.4221496410225143 ) ) ;
#5945=CARTESIAN_POINT ( 'NONE',  ( -12.04756914620937636, -13.80987496524771885, -232.8991007102355582 ) ) ;
#5946=CARTESIAN_POINT ( 'NONE',  ( 1.127544764349826867, -27.89617517048659323, -231.9509945439240823 ) ) ;
#5949=CARTESIAN_POINT ( 'NONE',  ( -1.336753021691559962, 16.04398320409420720, -230.2310715620304507 ) ) ;
#5950=CARTESIAN_POINT ( 'NONE',  ( 11.84677440217253341, -6.023754617643652054, -230.4469913264703962 ) ) ;
#5951=CARTESIAN_POINT ( 'NONE',  ( 14.31589812732703670, -5.349901619299376243, -221.2752230612865105 ) ) ;
#5952=CARTESIAN_POINT ( 'NONE',  ( -18.04772061096520375, 5.916925414182395038, -217.8829197293425750 ) ) ;
#5953=CARTESIAN_POINT ( 'NONE',  ( 11.64932556965463561, 7.668732705389711413, -229.0406978839571366 ) ) ;
#5954=CARTESIAN_POINT ( 'NONE',  ( 10.48640380280471618, 25.27581435651469022, -227.8976696013017715 ) ) ;
#5956=CARTESIAN_POINT ( 'NONE',  ( 4.565444334214069144, -15.90021673156186388, -218.4840512714275462 ) ) ;
#5958=CARTESIAN_POINT ( 'NONE',  ( -5.582510911615395699, 27.25430150734737111, -233.3200100877314469 ) ) ;
#5959=CARTESIAN_POINT ( 'NONE',  ( -17.20794623181132721, 21.97849129791581291, -217.9187454682870850 ) ) ;
#5960=CARTESIAN_POINT ( 'NONE',  ( -23.63383474287343589, -9.908731599815467916, -232.6396219513094081 ) ) ;
#5961=CARTESIAN_POINT ( 'NONE',  ( -3.060450601941519189, 13.29454208326677289, -222.0135664617158682 ) ) ;
#5962=CARTESIAN_POINT ( 'NONE',  ( -21.89065952084848021, -0.9940043559354364566, -216.9999999999999716 ) ) ;
#5965=CARTESIAN_POINT ( 'NONE',  ( 15.50779141722566656, -5.694711448414747856, -219.6385356284298211 ) ) ;
#5966=CARTESIAN_POINT ( 'NONE',  ( -5.590964611773372894, 13.92546790642523113, -228.7941110425196882 ) ) ;
#5967=CARTESIAN_POINT ( 'NONE',  ( 29.64577750251057608, 2.839131411071813549, -220.9704389295326905 ) ) ;
#5968=CARTESIAN_POINT ( 'NONE',  ( -21.93900267957129557, 7.862893636934532360, -233.4951761057262161 ) ) ;
#5969=CARTESIAN_POINT ( 'NONE',  ( 14.68783945462866924, 9.535285537539673228, -219.4694094309942045 ) ) ;
#5971=CARTESIAN_POINT ( 'NONE',  ( -6.702936938788568888, 25.88675107068059944, -218.1129661040884287 ) ) ;
#5972=CARTESIAN_POINT ( 'NONE',  ( -21.63546480557098306, -21.44004028177477750, -223.8762611443524122 ) ) ;
#5973=CARTESIAN_POINT ( 'NONE',  ( 17.43816562714825125, 15.15720016074785903, -232.3748236813696906 ) ) ;
#5974=CARTESIAN_POINT ( 'NONE',  ( -7.475691298859681311, -12.42146568352542779, -226.9176918848390017 ) ) ;
#5977=CARTESIAN_POINT ( 'NONE',  ( -13.37045227479810094, 5.250293981428504786, -224.2914120185227205 ) ) ;
#5978=CARTESIAN_POINT ( 'NONE',  ( 11.81564506561547390, -6.597897255275705142, -225.1493936678799628 ) ) ;
#5980=CARTESIAN_POINT ( 'NONE',  ( 3.198229568054530070, 16.42319727383711481, -222.3960047798183552 ) ) ;
#5981=CARTESIAN_POINT ( 'NONE',  ( -15.82622499106666325, 9.895986579907866343, -218.5115209877527604 ) ) ;
#5982=CARTESIAN_POINT ( 'NONE',  ( -31.04415783139704388, 5.868882651865275690, -221.1472518903637194 ) ) ;
#5983=CARTESIAN_POINT ( 'NONE',  ( -7.384981288797311194, -12.33405319921006615, -226.2189290763054998 ) ) ;
#5985=CARTESIAN_POINT ( 'NONE',  ( 18.03440114592047649, 4.755211820135348155, -216.3599228381250157 ) ) ;
#5987=CARTESIAN_POINT ( 'NONE',  ( -25.41475252190474521, -13.58614899836300260, -217.5872217295323310 ) ) ;
#5988=CARTESIAN_POINT ( 'NONE',  ( 3.192353461299334061, 22.13718518159985393, -217.1103300728619843 ) ) ;
#5989=CARTESIAN_POINT ( 'NONE',  ( 18.40125535140034430, 0.01434342441762339639, -233.2485400239426099 ) ) ;
#5990=CARTESIAN_POINT ( 'NONE',  ( -5.562203253303141359, 12.75725363875033302, -225.3078268727488478 ) ) ;
#5991=CARTESIAN_POINT ( 'NONE',  ( 14.28815361401014172, 13.86049093364188778, -216.0585456615740156 ) ) ;
#5992=CARTESIAN_POINT ( 'NONE',  ( -1.243024450407066439, -19.42038079238686876, -231.9048276842376595 ) ) ;
#5994=CARTESIAN_POINT ( 'NONE',  ( -7.084830653876206696, -25.45310193036084456, -219.3007580301989492 ) ) ;
#5995=CARTESIAN_POINT ( 'NONE',  ( 24.03642272140365677, 3.646960756862087205, -218.2320643939070806 ) ) ;
#5996=CARTESIAN_POINT ( 'NONE',  ( 19.88636028791461641, -20.85574262981397453, -219.9907771812986823 ) ) ;
#5997=CARTESIAN_POINT ( 'NONE',  ( -22.53818779203657741, -7.663114047788936567, -232.6164956747681458 ) ) ;
#5998=CARTESIAN_POINT ( 'NONE',  ( -11.40116373163465369, -15.95513543764466213, -216.7841692646331353 ) ) ;
#5999=CARTESIAN_POINT ( 'NONE',  ( 11.39755372583812587, 20.40856199875060639, -231.2895618162029621 ) ) ;
#6001=CARTESIAN_POINT ( 'NONE',  ( -12.10179538005628963, 1.685214252672075030, -222.4835512146784424 ) ) ;
#6002=CARTESIAN_POINT ( 'NONE',  ( 3.763426558366607111, 28.60172112197566818, -230.1816715025297526 ) ) ;
#6003=CARTESIAN_POINT ( 'NONE',  ( 3.635089269978064141, 27.05650967970794341, -222.4639105745756638 ) ) ;
#6004=CARTESIAN_POINT ( 'NONE',  ( 23.46500920064399409, -11.67104692860896620, -233.8722294412333724 ) ) ;
#6006=CARTESIAN_POINT ( 'NONE',  ( 14.69853173970351179, 23.44775873627089524, -231.2711109634281001 ) ) ;
#6007=CARTESIAN_POINT ( 'NONE',  ( -12.15411956849120756, 11.21601165624538687, -228.1895064089065670 ) ) ;
#6008=CARTESIAN_POINT ( 'NONE',  ( -17.91550223652134122, 4.809113705933536487, -230.6324822114035555 ) ) ;
#6009=CARTESIAN_POINT ( 'NONE',  ( -4.902442737337177725, -13.94343087703807704, -224.3742458082145959 ) ) ;
#6012=CARTESIAN_POINT ( 'NONE',  ( 5.017623471397871349, 29.83561274492976878, -222.9769172135417250 ) ) ;
#6013=CARTESIAN_POINT ( 'NONE',  ( 13.82101996411362244, -10.82539765916244789, -229.0162845096555770 ) ) ;
#6015=CARTESIAN_POINT ( 'NONE',  ( -11.28700884291539630, -21.85791790461604478, -233.5354093188319951 ) ) ;
#6017=CARTESIAN_POINT ( 'NONE',  ( 5.017623471397871349, 29.83561274492976878, -222.9769172135417250 ) ) ;
#6018=PRODUCT_DEFINITION ( 'UNKNOWN', '', #3461, #1320 ) ;
#6019=CARTESIAN_POINT ( 'NONE',  ( -0.2269548806647709305, 12.31484924552052718, -228.6688778050056783 ) ) ;
#6021=CARTESIAN_POINT ( 'NONE',  ( -11.98736441306973077, 11.45674391201457176, -217.8252237716743025 ) ) ;
#6022=CARTESIAN_POINT ( 'NONE',  ( -26.76734473129764069, -3.453818734898710829, -232.3222361544058003 ) ) ;
#6025=CARTESIAN_POINT ( 'NONE',  ( -7.913358619554302642, 16.16796202616373890, -233.0981776325470491 ) ) ;
#6026=CARTESIAN_POINT ( 'NONE',  ( -14.99584720478923572, -27.01727836854440312, -219.7524089968786996 ) ) ;
#6027=CARTESIAN_POINT ( 'NONE',  ( 13.28406271702445274, -5.237238614233280742, -225.2640488721434622 ) ) ;
#6028=CARTESIAN_POINT ( 'NONE',  ( -16.65698539163286540, 11.03290537638306112, -233.6474915129378758 ) ) ;
#6029=CARTESIAN_POINT ( 'NONE',  ( -25.59521542166570640, 7.637420400166985424, -216.4190921938142935 ) ) ;
#6030=CARTESIAN_POINT ( 'NONE',  ( 0.07890756785233743464, 25.14108539708653822, -218.4152285319504756 ) ) ;
#6032=CARTESIAN_POINT ( 'NONE',  ( 14.18323607655884722, 3.286047475533308226, -222.8710065128477140 ) ) ;
#6033=CARTESIAN_POINT ( 'NONE',  ( -12.46707500365009480, -15.03319212650626824, -230.3369784839848933 ) ) ;
#6035=CARTESIAN_POINT ( 'NONE',  ( 5.833753951408669813, 12.47745132051510453, -226.2508980627489450 ) ) ;
#6036=CARTESIAN_POINT ( 'NONE',  ( -12.70465517376339193, 12.03139199664008530, -229.6235454691090752 ) ) ;
#6037=CARTESIAN_POINT ( 'NONE',  ( -21.72273972318264867, 21.08396222359856864, -224.0477214759881690 ) ) ;
#6038=CARTESIAN_POINT ( 'NONE',  ( 30.39189047201120175, -1.943849802383817993, -228.0804048816970919 ) ) ;
#6041=CARTESIAN_POINT ( 'NONE',  ( -24.68906941503829700, 2.445024713909649705, -232.6803430500543755 ) ) ;
#6042=CARTESIAN_POINT ( 'NONE',  ( -6.657868545208735611, -13.01156946085308874, -219.4730114480542227 ) ) ;
#6043=CARTESIAN_POINT ( 'NONE',  ( 13.84082998555989974, 1.588769853554271361, -227.5469802220412134 ) ) ;
#6044=CARTESIAN_POINT ( 'NONE',  ( 0.6364901924797052857, 13.89978473517355617, -221.8840706290426397 ) ) ;
#6046=CARTESIAN_POINT ( 'NONE',  ( -20.67624351032310059, -0.8683020119106035217, -219.0957770725675005 ) ) ;
#6047=CARTESIAN_POINT ( 'NONE',  ( 10.39636392256998221, 18.46527700675686035, -215.1860221565626148 ) ) ;
#6049=CARTESIAN_POINT ( 'NONE',  ( 14.05129436669267662, 0.2182301052511314010, -222.0076932542802695 ) ) ;
#6050=CARTESIAN_POINT ( 'NONE',  ( 26.48990917286906921, 12.16675355942207659, -225.0153622588060216 ) ) ;
#6053=CARTESIAN_POINT ( 'NONE',  ( 16.72004689093256857, -4.507886829375356008, -228.6412576449023959 ) ) ;
#6054=CARTESIAN_POINT ( 'NONE',  ( -23.54665576872953636, -14.78900941482413067, -230.7594827126482073 ) ) ;
#6057=CARTESIAN_POINT ( 'NONE',  ( -1.248802714212398968, 14.93471382136348602, -228.4293827518713158 ) ) ;
#6058=CARTESIAN_POINT ( 'NONE',  ( 13.95860357795928941, -2.197645239214564672, -231.3209047126647988 ) ) ;
#6059=CARTESIAN_POINT ( 'NONE',  ( 13.62757736989142465, -5.584028114184929947, -227.2616851496390211 ) ) ;
#6060=CARTESIAN_POINT ( 'NONE',  ( -14.58575946311604277, 2.190332613129932327, -228.6717927865686590 ) ) ;
#6061=CARTESIAN_POINT ( 'NONE',  ( 16.69977105456987232, 16.51652889326612694, -233.6667933521891030 ) ) ;
#6062=CARTESIAN_POINT ( 'NONE',  ( 14.66646255503707152, 18.43809875292740230, -219.3480462970252063 ) ) ;
#6064=CARTESIAN_POINT ( 'NONE',  ( 5.447232503735224718, -25.66160541809718865, -232.3984543420957323 ) ) ;
#6068=CARTESIAN_POINT ( 'NONE',  ( -13.31245686955614005, 26.96290519511623174, -230.1796856776773836 ) ) ;
#6069=CARTESIAN_POINT ( 'NONE',  ( -9.747505956077446854, 15.39125695327449783, -233.2799778227147840 ) ) ;
#6070=CARTESIAN_POINT ( 'NONE',  ( 24.55456120837795808, -10.86188008310946351, -220.0712554825904590 ) ) ;
#6071=CARTESIAN_POINT ( 'NONE',  ( -6.474151797443945533, 21.29193859232740138, -215.9573456447696458 ) ) ;
#6073=CARTESIAN_POINT ( 'NONE',  ( -0.1452471002967452851, 24.29564289358754081, -234.0861481044164805 ) ) ;
#6074=CARTESIAN_POINT ( 'NONE',  ( 15.06072304412464291, 3.291435955319735651, -218.8606307204261725 ) ) ;
#6075=CARTESIAN_POINT ( 'NONE',  ( -11.67631226053870996, 6.737291529340801333, -227.3110382950315227 ) ) ;
#6076=CARTESIAN_POINT ( 'NONE',  ( 15.61962121506769385, 4.525360868525488911, -229.0684696061408090 ) ) ;
#6078=CARTESIAN_POINT ( 'NONE',  ( 1.847452069095833593, 15.11597492720254543, -223.6261404253179421 ) ) ;
#6079=CARTESIAN_POINT ( 'NONE',  ( -22.51170993270524789, -14.32174306031543054, -231.7292175355062795 ) ) ;
#6080=CARTESIAN_POINT ( 'NONE',  ( 10.55627441269396094, 10.31758739525044888, -223.1990319438957613 ) ) ;
#6081=CARTESIAN_POINT ( 'NONE',  ( -3.630465294598614889, -13.73165509241056093, -221.1424077787270619 ) ) ;
#6083=CARTESIAN_POINT ( 'NONE',  ( -14.35594238341465889, 9.236863657925704629, -219.6542735655305307 ) ) ;
#6084=CARTESIAN_POINT ( 'NONE',  ( 17.47229821656412341, -21.26691171910925249, -219.4940788861217413 ) ) ;
#6085=CARTESIAN_POINT ( 'NONE',  ( 3.281983756374524663, 15.83593597903271721, -223.8697822987047346 ) ) ;
#6086=CARTESIAN_POINT ( 'NONE',  ( -9.954421844142357756, 11.21484508112568079, -226.0177122452137439 ) ) ;
#6087=CARTESIAN_POINT ( 'NONE',  ( -13.63292518690856170, 3.968236334994402981, -218.3158317831635316 ) ) ;
#6088=CARTESIAN_POINT ( 'NONE',  ( -20.58881354142085485, -10.73024182470851606, -219.1570184730780397 ) ) ;
#6090=CARTESIAN_POINT ( 'NONE',  ( 13.21888801141564151, 2.135177519634172238, -228.0426311217386797 ) ) ;
#6092=CARTESIAN_POINT ( 'NONE',  ( -9.690988788510356500, -7.266623515821958534, -222.7221403394456445 ) ) ;
#6093=CARTESIAN_POINT ( 'NONE',  ( -1.975202609796049336, 20.81351768191813889, -217.5779402428482001 ) ) ;
#6094=CARTESIAN_POINT ( 'NONE',  ( 24.19635128940818447, 10.31396593861802380, -216.9479509989864425 ) ) ;
#6095=CARTESIAN_POINT ( 'NONE',  ( -14.46024998630872282, 14.54669730493860946, -231.4156670963686508 ) ) ;
#6097=CARTESIAN_POINT ( 'NONE',  ( 12.92410717862594893, 29.37236178718849189, -224.5435071569520744 ) ) ;
#6099=CARTESIAN_POINT ( 'NONE',  ( 0.8935217740153370558, -25.09083646304939919, -218.5222943608621335 ) ) ;
#6101=CARTESIAN_POINT ( 'NONE',  ( -1.827935560680505445, -14.81092009092713369, -225.7372845858837707 ) ) ;
#6102=CARTESIAN_POINT ( 'NONE',  ( 23.49048926389013658, 9.645778135078892035, -218.7307869890797463 ) ) ;
#6103=CARTESIAN_POINT ( 'NONE',  ( 13.62757736989142465, -5.584028114184929947, -227.2616851496390211 ) ) ;
#6105=CARTESIAN_POINT ( 'NONE',  ( 24.67321061357916889, 1.914345543126667826, -232.4367140101115581 ) ) ;
#6106=CARTESIAN_POINT ( 'NONE',  ( -15.46269062504165781, -26.67469327287815517, -225.2085449711190677 ) ) ;
#6107=CARTESIAN_POINT ( 'NONE',  ( 10.64798096806036121, 19.48085866535796740, -231.3996658690317361 ) ) ;
#6109=CARTESIAN_POINT ( 'NONE',  ( 15.80790828609669951, 3.698719088746416972, -219.8106174092292804 ) ) ;
#6110=CARTESIAN_POINT ( 'NONE',  ( 5.069241901512100412, 14.34986542013820632, -229.6420000777802954 ) ) ;
#6111=CARTESIAN_POINT ( 'NONE',  ( 9.382249691333727881, 26.55946126407900820, -224.4468135941759215 ) ) ;
#6112=CARTESIAN_POINT ( 'NONE',  ( 14.87770435525805013, -9.987123395515542512, -215.8225415630120665 ) ) ;
#6113=CARTESIAN_POINT ( 'NONE',  ( 22.20554449732931346, 18.01468431515759860, -218.9348803756412849 ) ) ;
#6114=CARTESIAN_POINT ( 'NONE',  ( -15.19607346356906952, 9.485739149828241068, -229.2407115334993080 ) ) ;
#6115=CARTESIAN_POINT ( 'NONE',  ( -15.54392142943450317, 6.670312097614393920, -219.6934017696036676 ) ) ;
#6116=CARTESIAN_POINT ( 'NONE',  ( -5.429593058350183910, -25.95961553913046416, -230.5291520159703111 ) ) ;
#6118=CARTESIAN_POINT ( 'NONE',  ( 16.38151749656409351, 8.902090001712490874, -231.2955017965201989 ) ) ;
#6119=CARTESIAN_POINT ( 'NONE',  ( 20.36520141328406552, -18.94542628267938156, -227.6082859645964902 ) ) ;
#6122=CARTESIAN_POINT ( 'NONE',  ( -5.804961988600464196, -12.67915086496026511, -228.7923277404792088 ) ) ;
#6124=CARTESIAN_POINT ( 'NONE',  ( 5.069241901512100412, 14.34986542013820632, -229.6420000777802954 ) ) ;
#6125=CARTESIAN_POINT ( 'NONE',  ( -4.155456637169709921, 11.30291311430030987, -225.2606024264729001 ) ) ;
#6127=CARTESIAN_POINT ( 'NONE',  ( -19.00318367631585659, 13.14621133775862916, -233.8403879275295765 ) ) ;
#6128=CARTESIAN_POINT ( 'NONE',  ( 24.22993967103762714, -2.502297861120115208, -232.9814837474525007 ) ) ;
#6129=CARTESIAN_POINT ( 'NONE',  ( 21.96352831578809273, -0.3315607655629317918, -233.9427286327412503 ) ) ;
#6131=CARTESIAN_POINT ( 'NONE',  ( -6.855867220396999251, 12.17758473459128332, -220.6375607554995213 ) ) ;
#6132=CARTESIAN_POINT ( 'NONE',  ( -9.794218246645117532, -15.26311849320921255, -215.4893187949746505 ) ) ;
#6133=CARTESIAN_POINT ( 'NONE',  ( 14.02668320743028119, -5.282748560960272677, -221.9001732195871739 ) ) ;
#6135=CARTESIAN_POINT ( 'NONE',  ( -23.52999999174766543, 19.39566142560855866, -221.9446938626390704 ) ) ;
#6136=CARTESIAN_POINT ( 'NONE',  ( -20.49711526797010208, 7.006997077916217620, -215.3369776077118445 ) ) ;
#6138=CARTESIAN_POINT ( 'NONE',  ( -1.837924626891132229, 29.27703531260187475, -227.2344808100871774 ) ) ;
#6140=CARTESIAN_POINT ( 'NONE',  ( -14.37318171526297483, 2.227741863946853140, -231.7654527934561202 ) ) ;
#6141=CARTESIAN_POINT ( 'NONE',  ( -12.44689724543316522, -19.26441470091720731, -219.1960634559673622 ) ) ;
#6143=CARTESIAN_POINT ( 'NONE',  ( -17.78731991475362406, 16.78509880370027929, -218.2387321183659310 ) ) ;
#6144=CARTESIAN_POINT ( 'NONE',  ( 10.12956299421491302, 11.38773431477224385, -230.3175791991728829 ) ) ;
#6145=CARTESIAN_POINT ( 'NONE',  ( 3.711349367426693746, 16.84755988915346236, -233.7359972593521888 ) ) ;
#6146=CARTESIAN_POINT ( 'NONE',  ( -14.26213125333782727, -4.747741064748048245, -225.2154851558723294 ) ) ;
#6149=CARTESIAN_POINT ( 'NONE',  ( -11.49049084071896409, 11.06834963248926940, -218.3354249205727058 ) ) ;
#6150=CARTESIAN_POINT ( 'NONE',  ( -8.875208054371373834, -23.27682998066124398, -233.1222812539844540 ) ) ;
#6151=CARTESIAN_POINT ( 'NONE',  ( 25.18785298611088308, 3.974282393449815931, -218.7636041058819956 ) ) ;
#6152=CARTESIAN_POINT ( 'NONE',  ( -3.003186468682855104, 15.63968344752823469, -231.5301608670590667 ) ) ;
#6154=CARTESIAN_POINT ( 'NONE',  ( -18.04102731735134313, 0.8647102676311391178, -229.4625228093430849 ) ) ;
#6155=CARTESIAN_POINT ( 'NONE',  ( 11.00045714400293306, 20.20239058357963913, -215.1666500215986275 ) ) ;
#6157=CARTESIAN_POINT ( 'NONE',  ( 23.49048926389013658, 9.645778135078892035, -218.7307869890797463 ) ) ;
#6159=CARTESIAN_POINT ( 'NONE',  ( 27.03411061974195562, -3.460823241630351710, -221.7771387205989413 ) ) ;
#6160=CARTESIAN_POINT ( 'NONE',  ( -14.78079095050690661, -5.416970230978240153, -229.7193632018645246 ) ) ;
#6164=CARTESIAN_POINT ( 'NONE',  ( -14.84124724799726991, 21.42277200659090042, -233.6300684249849553 ) ) ;
#6165=CARTESIAN_POINT ( 'NONE',  ( 19.66172111867919270, -11.21951684559458506, -235.3531537740016972 ) ) ;
#6166=CARTESIAN_POINT ( 'NONE',  ( 25.83609367470520723, -15.13481494965009411, -225.4685613576401124 ) ) ;
#6167=CARTESIAN_POINT ( 'NONE',  ( -15.30295614572244922, 9.661125001905515930, -218.8475896279880146 ) ) ;
#6168=CARTESIAN_POINT ( 'NONE',  ( 30.52813181070726856, 5.438803974502569361, -223.5441926215666513 ) ) ;
#6169=CARTESIAN_POINT ( 'NONE',  ( 8.312165662451315384, 13.84431584962456974, -225.8109542921768025 ) ) ;
#6170=VERTEX_POINT ( 'NONE', #19736 ) ;
#6171=CARTESIAN_POINT ( 'NONE',  ( 3.520698644836853131, -14.14291361662535884, -221.2714412251625618 ) ) ;
#6173=CARTESIAN_POINT ( 'NONE',  ( -16.85225081326727903, 6.237400186851330020, -234.5847093771173206 ) ) ;
#6175=CARTESIAN_POINT ( 'NONE',  ( -4.296082356836364191, 12.57880442405704002, -229.5247240216588125 ) ) ;
#6176=CARTESIAN_POINT ( 'NONE',  ( 3.490829917597003895, 11.40812925993816229, -222.8973702487053004 ) ) ;
#6177=CARTESIAN_POINT ( 'NONE',  ( 15.40548389857710987, -8.435137368586953954, -220.3367290259554920 ) ) ;
#6178=CARTESIAN_POINT ( 'NONE',  ( -9.740348021262962064, 16.12529029871877384, -216.4361617420699702 ) ) ;
#6182=CARTESIAN_POINT ( 'NONE',  ( -2.328291070394212792, 14.80737693666302945, -219.0291440940735868 ) ) ;
#6183=CARTESIAN_POINT ( 'NONE',  ( 30.57915561709945251, 3.468229287067555067, -223.8876084027091906 ) ) ;
#6184=CARTESIAN_POINT ( 'NONE',  ( -24.02434186778878455, 18.57431834865475651, -228.2662945587547370 ) ) ;
#6185=CARTESIAN_POINT ( 'NONE',  ( 15.76910524310159900, 5.601482066865847820, -220.3440822020379528 ) ) ;
#6186=CARTESIAN_POINT ( 'NONE',  ( 6.608541902967795423, 16.43938546752961116, -220.2982508316308952 ) ) ;
#6188=CARTESIAN_POINT ( 'NONE',  ( 9.132190541728901323, 17.73033835127231939, -219.5524510795130766 ) ) ;
#6189=CARTESIAN_POINT ( 'NONE',  ( -18.89430729770302975, -12.42271633246521212, -233.2230176520695295 ) ) ;
#6190=CARTESIAN_POINT ( 'NONE',  ( 22.84140515590350518, 18.29101041979067332, -226.2334522600520472 ) ) ;
#6191=CARTESIAN_POINT ( 'NONE',  ( -1.232290808404003624, -30.06229647885771428, -229.8325228448912583 ) ) ;
#6195=CARTESIAN_POINT ( 'NONE',  ( -11.08731210905863840, 25.61052584666692766, -228.9953606804266997 ) ) ;
#6197=CARTESIAN_POINT ( 'NONE',  ( 12.90505172109588194, -11.18139282378177768, -218.7382941517081747 ) ) ;
#6198=CARTESIAN_POINT ( 'NONE',  ( 26.39436175479395885, 14.32821500273865034, -221.6819523832376149 ) ) ;
#6199=CARTESIAN_POINT ( 'NONE',  ( -20.97727766418175932, 9.381545086430262970, -232.5968905491617420 ) ) ;
#6200=CARTESIAN_POINT ( 'NONE',  ( -12.38801939673351704, 9.361418580567464787, -232.8075769614211765 ) ) ;
#6201=CARTESIAN_POINT ( 'NONE',  ( -16.42300678490213883, -6.478264502461970054, -228.9348778629521064 ) ) ;
#6202=CARTESIAN_POINT ( 'NONE',  ( 10.93653298376230687, 10.42959444671468106, -232.5920418140667039 ) ) ;
#6204=CARTESIAN_POINT ( 'NONE',  ( -14.71809293534535534, -5.923356948231951691, -217.5005292165803041 ) ) ;
#6205=CARTESIAN_POINT ( 'NONE',  ( 7.213476267053916757, 16.78447451494783138, -217.5857052077849687 ) ) ;
#6207=CARTESIAN_POINT ( 'NONE',  ( -20.86570240061152148, 1.122719768445835875, -219.0984131021933763 ) ) ;
#6209=CARTESIAN_POINT ( 'NONE',  ( -18.02718827071834085, 20.33515877052379395, -229.5060669840136143 ) ) ;
#6210=CARTESIAN_POINT ( 'NONE',  ( 10.81638188557560731, 14.98959006186633403, -234.2424515599453514 ) ) ;
#6213=CARTESIAN_POINT ( 'NONE',  ( 3.499756879752360827, -15.16424639601953039, -225.9472731234413061 ) ) ;
#6214=CARTESIAN_POINT ( 'NONE',  ( 1.967796959512672306, -15.42100964229427085, -222.1538042820122314 ) ) ;
#6215=CARTESIAN_POINT ( 'NONE',  ( -24.77996431573922820, 10.49354383977773786, -234.1655613096203581 ) ) ;
#6216=CARTESIAN_POINT ( 'NONE',  ( 14.02668320743028119, -5.282748560960272677, -221.9001732195871739 ) ) ;
#6217=CARTESIAN_POINT ( 'NONE',  ( -18.11268275035277853, -3.459088653808292335, -218.4233329573673359 ) ) ;
#6218=CARTESIAN_POINT ( 'NONE',  ( -21.52428768452188734, -21.65989873160339840, -225.4304055049964006 ) ) ;
#6219=CARTESIAN_POINT ( 'NONE',  ( 3.689800395305025127, 23.07294874520714956, -219.2515233573129478 ) ) ;
#6221=CARTESIAN_POINT ( 'NONE',  ( -17.17981675979428147, 1.478343374046288128, -216.2419730925687418 ) ) ;
#6222=CARTESIAN_POINT ( 'NONE',  ( 4.340445191644851874, 29.86837761166362881, -227.4879512554873315 ) ) ;
#6223=CARTESIAN_POINT ( 'NONE',  ( 13.41709597927210496, 19.57823531746157997, -218.2666972400567147 ) ) ;
#6224=CARTESIAN_POINT ( 'NONE',  ( 15.50373320885645079, -27.90820408561472732, -228.0623419774833280 ) ) ;
#6227=CARTESIAN_POINT ( 'NONE',  ( 16.10596270516584028, 24.75152718569329835, -228.9330127594856492 ) ) ;
#6228=CARTESIAN_POINT ( 'NONE',  ( -21.01242583983345469, 16.60754347445175227, -220.8286358486543293 ) ) ;
#6229=CARTESIAN_POINT ( 'NONE',  ( -24.49083850720273148, 4.222094140707651100, -219.1543001448025905 ) ) ;
#6231=CARTESIAN_POINT ( 'NONE',  ( 5.920190106170357680, -27.41802839654005197, -221.0732524667164114 ) ) ;
#6234=CARTESIAN_POINT ( 'NONE',  ( 20.41153371889344825, 17.18812948447019551, -230.7531656956970778 ) ) ;
#6235=CARTESIAN_POINT ( 'NONE',  ( 14.94445598564424493, -12.06760924077967090, -230.4366326412025785 ) ) ;
#6236=CARTESIAN_POINT ( 'NONE',  ( -28.61025869263052712, 6.891613135096296361, -222.2489362813765013 ) ) ;
#6237=CARTESIAN_POINT ( 'NONE',  ( -7.531388159411753769, -21.98719092781708540, -216.0713624712111312 ) ) ;
#6239=CARTESIAN_POINT ( 'NONE',  ( 4.543450689403089271, 15.91052110650461771, -218.9437823786444426 ) ) ;
#6241=CARTESIAN_POINT ( 'NONE',  ( 0.9169988354999972779, 20.59043933275470550, -235.2854195559275752 ) ) ;
#6243=CARTESIAN_POINT ( 'NONE',  ( -3.643097910890548796, 22.16888955197135047, -233.9701981029593298 ) ) ;
#6244=CARTESIAN_POINT ( 'NONE',  ( -13.36955836198420577, -3.222265253903016990, -227.4060678739157026 ) ) ;
#6247=CARTESIAN_POINT ( 'NONE',  ( -17.39699619235753048, 15.64332637722790054, -216.0406373264262641 ) ) ;
#6248=CARTESIAN_POINT ( 'NONE',  ( -9.037518995728490268, -13.81466884781966620, -216.3195389756191673 ) ) ;
#6249=CARTESIAN_POINT ( 'NONE',  ( 25.83609367470520723, -15.13481494965009411, -225.4685613576401124 ) ) ;
#6250=CARTESIAN_POINT ( 'NONE',  ( -2.958555384449997661, 13.07587799061801093, -222.7767538261418565 ) ) ;
#6251=CARTESIAN_POINT ( 'NONE',  ( -27.05172747931452903, 14.36075930490012276, -228.5082213655825853 ) ) ;
#6252=CARTESIAN_POINT ( 'NONE',  ( -9.290933312444883185, 29.15551353946876745, -225.8551562993724247 ) ) ;
#6253=CARTESIAN_POINT ( 'NONE',  ( -14.87984907657228639, 0.2138881189739126887, -228.7773920408832282 ) ) ;
#6254=CARTESIAN_POINT ( 'NONE',  ( 15.70179827786738969, 6.572001003133339125, -229.5476218741844434 ) ) ;
#6255=CARTESIAN_POINT ( 'NONE',  ( -8.783466540727490113, -25.47690852953548557, -220.9562114332719318 ) ) ;
#6257=CARTESIAN_POINT ( 'NONE',  ( -9.988594796049140356, 11.34066464990972811, -226.6453149279956563 ) ) ;
#6258=CARTESIAN_POINT ( 'NONE',  ( 17.97920459523930958, 17.43922474653955490, -233.2737719749805763 ) ) ;
#6259=CARTESIAN_POINT ( 'NONE',  ( 1.220475224794998370, 29.83033731899746144, -230.4224274340063801 ) ) ;
#6261=CARTESIAN_POINT ( 'NONE',  ( 13.66858788651615164, -3.112492835348085407, -221.5154270223497690 ) ) ;
#6264=CARTESIAN_POINT ( 'NONE',  ( -9.250876228778270871, 9.538614635316015722, -227.1332118982684563 ) ) ;
#6265=CARTESIAN_POINT ( 'NONE',  ( -6.443428446094314310, -19.32516562084312994, -233.2789765400915201 ) ) ;
#6266=CARTESIAN_POINT ( 'NONE',  ( 14.98418162551161714, 4.450317369940187895, -227.9894155827521161 ) ) ;
#6268=CARTESIAN_POINT ( 'NONE',  ( 12.53674998645855787, 17.96979015029927851, -232.8843215672231679 ) ) ;
#6270=CARTESIAN_POINT ( 'NONE',  ( -11.10182655035041144, 8.778638955377752850, -227.1050196202568827 ) ) ;
#6271=CARTESIAN_POINT ( 'NONE',  ( 17.10545320562996352, 22.53742678899184781, -232.4605876935045785 ) ) ;
#6274=CARTESIAN_POINT ( 'NONE',  ( 17.19674704922021391, 23.07334190050143974, -228.8256488842130238 ) ) ;
#6276=CARTESIAN_POINT ( 'NONE',  ( 15.57890332219703389, -7.739300371747003027, -228.5080386124398899 ) ) ;
#6277=CARTESIAN_POINT ( 'NONE',  ( -25.82802808205240552, -14.78441951539553401, -222.6940535085979604 ) ) ;
#6281=CARTESIAN_POINT ( 'NONE',  ( -0.4548635697939061306, 27.30478022265488036, -219.8474162243132071 ) ) ;
#6282=CARTESIAN_POINT ( 'NONE',  ( 30.72375212156453372, -9.269427080566114086, -227.3728682798597731 ) ) ;
#6283=CARTESIAN_POINT ( 'NONE',  ( 18.55298002304457228, -12.22359628793950570, -216.9137843736221782 ) ) ;
#6284=CARTESIAN_POINT ( 'NONE',  ( -23.20103936322198024, 10.64725167743880085, -231.7714206262400864 ) ) ;
#6285=CARTESIAN_POINT ( 'NONE',  ( -20.86570240061152148, 1.122719768445835875, -219.0984131021933763 ) ) ;
#6286=CARTESIAN_POINT ( 'NONE',  ( 11.87550186346493497, 14.27797038184677270, -220.2068243228838185 ) ) ;
#6288=CARTESIAN_POINT ( 'NONE',  ( -0.6326494355537284342, -15.87741594504987219, -229.6822519216137266 ) ) ;
#6290=CARTESIAN_POINT ( 'NONE',  ( -30.17036082276531772, 5.959165309317525860, -219.4883053239162791 ) ) ;
#6291=CARTESIAN_POINT ( 'NONE',  ( 18.69149182921226782, 24.00661454656289706, -229.8257469855424517 ) ) ;
#6292=CARTESIAN_POINT ( 'NONE',  ( 4.401501667365108617, 18.53594119471695123, -215.1186850315663150 ) ) ;
#6293=CARTESIAN_POINT ( 'NONE',  ( 13.21219219391003818, -8.064832675337259005, -225.0434479037668041 ) ) ;
#6294=CARTESIAN_POINT ( 'NONE',  ( -6.571166997218196748, 12.74865329367398736, -229.9840124400968762 ) ) ;
#6295=CARTESIAN_POINT ( 'NONE',  ( -14.10849459794400751, -0.2436790717799666162, -223.1085195285415921 ) ) ;
#6297=CARTESIAN_POINT ( 'NONE',  ( 12.58033168766476528, 20.35631482982274676, -235.1670639654690547 ) ) ;
#6299=CARTESIAN_POINT ( 'NONE',  ( -27.11599398522282911, 10.60460483532474996, -224.7310548435675912 ) ) ;
#6300=CARTESIAN_POINT ( 'NONE',  ( -23.49379658590067876, 11.46840048879614393, -217.2519070826072323 ) ) ;
#6301=CARTESIAN_POINT ( 'NONE',  ( 17.43816562714825125, 15.15720016074785903, -232.3748236813696906 ) ) ;
#6302=CARTESIAN_POINT ( 'NONE',  ( 9.425340689562565544, 25.38932416188112384, -221.3391712389563963 ) ) ;
#6305=CARTESIAN_POINT ( 'NONE',  ( 15.70200226922815290, 22.14006925444000018, -227.8255507828836244 ) ) ;
#6306=CARTESIAN_POINT ( 'NONE',  ( -11.88525712185471050, -8.925198460467992589, -221.0951487055306472 ) ) ;
#6307=CARTESIAN_POINT ( 'NONE',  ( 15.33737796850231305, 13.57479350230705428, -232.3313557812109025 ) ) ;
#6308=CARTESIAN_POINT ( 'NONE',  ( -9.979217823323752512, -26.65442139683551659, -219.8174849573283325 ) ) ;
#6310=CARTESIAN_POINT ( 'NONE',  ( -4.386767007475907754, 14.39570986262862107, -223.2690175027443615 ) ) ;
#6311=EDGE_CURVE ( 'NONE', #11616, #9103, #2482, .T. ) ;
#6312=CARTESIAN_POINT ( 'NONE',  ( 24.05238142633148968, -17.07083877791421500, -221.4615098029387070 ) ) ;
#6313=CARTESIAN_POINT ( 'NONE',  ( 17.98704291748025952, 16.14142602298251461, -217.3684083235702644 ) ) ;
#6314=CARTESIAN_POINT ( 'NONE',  ( -5.365396334125453137, 16.47374957271378904, -219.4721119688156534 ) ) ;
#6315=CARTESIAN_POINT ( 'NONE',  ( -20.73319232323294514, 5.144688277016327582, -214.6391322078443977 ) ) ;
#6316=CARTESIAN_POINT ( 'NONE',  ( -17.33275459786259276, -4.423804729537573088, -220.8440611986277418 ) ) ;
#6317=CARTESIAN_POINT ( 'NONE',  ( -27.32994399549947673, 3.379920396491164603, -227.9326384921875217 ) ) ;
#6319=CARTESIAN_POINT ( 'NONE',  ( -29.62561404221338890, 0.9211338879504321620, -221.2478075149841743 ) ) ;
#6320=CARTESIAN_POINT ( 'NONE',  ( 19.40629804599390340, 15.10110417999774057, -216.3942729496570223 ) ) ;
#6321=CARTESIAN_POINT ( 'NONE',  ( 29.11492790716816614, 6.132849117128307270, -229.8316941169402412 ) ) ;
#6322=CARTESIAN_POINT ( 'NONE',  ( -4.651113456395510326, 27.58151660986499110, -218.3072938287727141 ) ) ;
#6323=CARTESIAN_POINT ( 'NONE',  ( 8.730612144237051453, 13.93563980088501886, -217.1627566045470132 ) ) ;
#6326=CARTESIAN_POINT ( 'NONE',  ( 8.343784211782431015, -26.96289276196324636, -225.6651636531778422 ) ) ;
#6328=CARTESIAN_POINT ( 'NONE',  ( 2.179383121900682951, -16.00498718933496889, -221.0566978482307832 ) ) ;
#6329=CARTESIAN_POINT ( 'NONE',  ( -12.02603758797190459, 8.152912069735307909, -218.2257190893353709 ) ) ;
#6330=CARTESIAN_POINT ( 'NONE',  ( 8.785770181087007913, -10.38731345016515917, -223.4272116603623317 ) ) ;
#6331=CARTESIAN_POINT ( 'NONE',  ( -23.84209965496292227, -7.976777114481962805, -232.1458837748831456 ) ) ;
#6332=CARTESIAN_POINT ( 'NONE',  ( -14.24095617957673632, -25.86326826095433162, -229.7068514753157160 ) ) ;
#6333=CARTESIAN_POINT ( 'NONE',  ( 12.89118769162836031, 6.140251663080722899, -228.8792332048833771 ) ) ;
#6335=CARTESIAN_POINT ( 'NONE',  ( -18.17591565587962776, 16.23604867791855355, -233.2845329962925121 ) ) ;
#6336=CARTESIAN_POINT ( 'NONE',  ( 14.91731358302415877, 13.33846450914490056, -217.2468882285060658 ) ) ;
#6337=CARTESIAN_POINT ( 'NONE',  ( 4.301648988406530094, 13.23079486486395240, -223.2766268961034655 ) ) ;
#6338=CARTESIAN_POINT ( 'NONE',  ( 7.017641603801325623, 14.96204511409594673, -228.1064041248110073 ) ) ;
#6339=CARTESIAN_POINT ( 'NONE',  ( 8.134488596945347538, -11.59059696487595481, -231.6292735970982335 ) ) ;
#6340=CARTESIAN_POINT ( 'NONE',  ( 27.13894094332088969, 12.30518789341946295, -220.2765066586875093 ) ) ;
#6341=CARTESIAN_POINT ( 'NONE',  ( -12.80756961294691010, 26.82110654133967387, -223.7464923486294026 ) ) ;
#6342=CARTESIAN_POINT ( 'NONE',  ( -9.776740361816679936, -16.43846667899986258, -218.0739489017842061 ) ) ;
#6343=CARTESIAN_POINT ( 'NONE',  ( -20.26851768784797869, -0.8260594303982465858, -217.1279713726092098 ) ) ;
#6346=CARTESIAN_POINT ( 'NONE',  ( 18.50911814746675788, 15.92944434255054453, -232.0449215596906072 ) ) ;
#6347=CARTESIAN_POINT ( 'NONE',  ( 18.87161431088011199, -9.942086275362749248, -230.8324498438813350 ) ) ;
#6348=CARTESIAN_POINT ( 'NONE',  ( -12.62195384480319582, 9.244619650382723819, -228.6283004876635516 ) ) ;
#6349=CARTESIAN_POINT ( 'NONE',  ( -8.376153411442972541, -27.59911039556260448, -219.0729038785590888 ) ) ;
#6350=CARTESIAN_POINT ( 'NONE',  ( -0.3969026096611234511, 20.89748314411456676, -216.3289738411752978 ) ) ;
#6351=CARTESIAN_POINT ( 'NONE',  ( 3.044038000507106378, 30.22621415828681180, -231.1553244844465382 ) ) ;
#6353=CARTESIAN_POINT ( 'NONE',  ( 2.837900457371055563, 25.11342719071438978, -232.9871906064174709 ) ) ;
#6354=CARTESIAN_POINT ( 'NONE',  ( 29.78177645116457128, -4.041743286679309044, -225.6339783681140432 ) ) ;
#6355=CARTESIAN_POINT ( 'NONE',  ( 24.68983475587330645, -0.6584631617853404784, -233.6195837498767958 ) ) ;
#6357=CARTESIAN_POINT ( 'NONE',  ( 4.343013938751969505, 13.02036404005131587, -224.7825435359082178 ) ) ;
#6358=CARTESIAN_POINT ( 'NONE',  ( -12.24325066776002657, -20.13554689852184509, -214.7483342848939856 ) ) ;
#6359=CARTESIAN_POINT ( 'NONE',  ( 10.40291689048662782, -13.87512507945592333, -231.9656913702303029 ) ) ;
#6360=CARTESIAN_POINT ( 'NONE',  ( 14.98777556431132219, -10.10815648641214004, -217.9795565018743844 ) ) ;
#6361=CARTESIAN_POINT ( 'NONE',  ( -20.04070223234628756, 18.12164545743767263, -231.9292141396248610 ) ) ;
#6362=CARTESIAN_POINT ( 'NONE',  ( 5.909674498212842408, 15.76475534640655773, -228.4922217450045139 ) ) ;
#6363=CARTESIAN_POINT ( 'NONE',  ( -28.17543631911187063, 3.557555778861649642, -230.1980773687482156 ) ) ;
#6364=CARTESIAN_POINT ( 'NONE',  ( -16.65220264499505376, 11.77543314451157563, -216.3149620944649030 ) ) ;
#6365=CARTESIAN_POINT ( 'NONE',  ( -26.50758677328550306, -10.71756779952945671, -226.4207925882492987 ) ) ;
#6367=CARTESIAN_POINT ( 'NONE',  ( -22.07068341299880743, 18.38202870573248049, -227.7785760498121306 ) ) ;
#6368=CARTESIAN_POINT ( 'NONE',  ( 9.336393807558161839, 27.79372469574263960, -228.5913636680961361 ) ) ;
#6369=CARTESIAN_POINT ( 'NONE',  ( -6.496078068315311427, 23.46891392553531119, -233.1042179568201220 ) ) ;
#6370=CARTESIAN_POINT ( 'NONE',  ( 23.33467929415965614, -0.4823873731835089940, -233.9427286327415629 ) ) ;
#6373=CARTESIAN_POINT ( 'NONE',  ( -9.443239614166923701, 9.388015667058336788, -222.3195230688234290 ) ) ;
#6374=CARTESIAN_POINT ( 'NONE',  ( -3.917974041549708630, -18.23196399112299559, -217.4080104222929606 ) ) ;
#6375=CARTESIAN_POINT ( 'NONE',  ( 27.40550551777678123, 5.967061366481472895, -228.7463788799179554 ) ) ;
#6376=CARTESIAN_POINT ( 'NONE',  ( 12.99034161053428349, 11.71468708507361889, -230.9043293568357740 ) ) ;
#6378=CARTESIAN_POINT ( 'NONE',  ( 14.31589812732703670, -5.349901619299376243, -221.2752230612865105 ) ) ;
#6379=CARTESIAN_POINT ( 'NONE',  ( -21.66801938871533650, 16.28801167444048659, -218.5240035253498547 ) ) ;
#6380=CARTESIAN_POINT ( 'NONE',  ( 27.84414217501293010, 2.965433895642837214, -221.8999927093654492 ) ) ;
#6385=CARTESIAN_POINT ( 'NONE',  ( 26.08609146265030176, -9.082777145696592669, -223.3125241607380360 ) ) ;
#6386=CARTESIAN_POINT ( 'NONE',  ( -12.44777057840899559, -8.577008958641105352, -229.4809580173677830 ) ) ;
#6390=CARTESIAN_POINT ( 'NONE',  ( 6.332229114051408203, 16.75791367489523154, -229.7702805136205200 ) ) ;
#6392=CARTESIAN_POINT ( 'NONE',  ( 13.50228739682142454, -27.74890714798514679, -227.9743917065363519 ) ) ;
#6393=CARTESIAN_POINT ( 'NONE',  ( 27.32546652195855685, -7.354568365469916991, -229.0866163655393279 ) ) ;
#6394=CARTESIAN_POINT ( 'NONE',  ( -12.33203608746942237, 8.428128317385924717, -222.9277009507565026 ) ) ;
#6395=CARTESIAN_POINT ( 'NONE',  ( 29.11492790716816614, 6.132849117128307270, -229.8316941169402412 ) ) ;
#6396=CARTESIAN_POINT ( 'NONE',  ( 23.44063276014420794, 13.61134749381700182, -229.1061940987080732 ) ) ;
#6398=CARTESIAN_POINT ( 'NONE',  ( 4.286954182150454429, -15.41507397180808425, -219.0323159710399352 ) ) ;
#6400=CARTESIAN_POINT ( 'NONE',  ( -18.67456582549428390, 11.07053394491094345, -214.7114755712704550 ) ) ;
#6402=CARTESIAN_POINT ( 'NONE',  ( 7.739849882373770917, 11.59357455229016409, -219.5521933286238720 ) ) ;
#6403=CARTESIAN_POINT ( 'NONE',  ( -2.218529449563984901, 24.06491599887877442, -214.8915873797660652 ) ) ;
#6404=CARTESIAN_POINT ( 'NONE',  ( 22.90686649137879627, -15.60507238429272192, -227.8443525802422585 ) ) ;
#6405=CARTESIAN_POINT ( 'NONE',  ( 0.7245137624042983227, 13.44764381486384330, -223.4043886706536455 ) ) ;
#6406=CARTESIAN_POINT ( 'NONE',  ( -16.20072894238734307, 0.5024448614660336210, -230.4554067149722130 ) ) ;
#6408=CARTESIAN_POINT ( 'NONE',  ( 11.13671218404335761, 30.21738803452449673, -224.2405745632392211 ) ) ;
#6409=CARTESIAN_POINT ( 'NONE',  ( -15.61959985466312872, 8.133362592386543355, -230.7826037412100106 ) ) ;
#6410=CARTESIAN_POINT ( 'NONE',  ( -2.958555384449997661, 13.07587799061801093, -222.7767538261418565 ) ) ;
#6411=CARTESIAN_POINT ( 'NONE',  ( 19.72515656911863147, 14.02277373989196541, -218.0718040828188009 ) ) ;
#6412=CARTESIAN_POINT ( 'NONE',  ( 15.03112630398312177, 24.11065413595933293, -226.8236212149936080 ) ) ;
#6415=CARTESIAN_POINT ( 'NONE',  ( -15.51091956967506391, -1.782849713491490018, -228.8089183834494520 ) ) ;
#6416=CARTESIAN_POINT ( 'NONE',  ( 12.85408565574548412, 7.821283853063205171, -223.1248833997948111 ) ) ;
#6417=CARTESIAN_POINT ( 'NONE',  ( 0.4137397183702169468, -14.31347623323147289, -219.6167997211809393 ) ) ;
#6419=CARTESIAN_POINT ( 'NONE',  ( -8.435479365662203577, 14.12888021429238528, -220.5365774424437859 ) ) ;
#6420=CARTESIAN_POINT ( 'NONE',  ( 9.009845654114897684, -15.13764346805314354, -231.2790349225496129 ) ) ;
#6421=CARTESIAN_POINT ( 'NONE',  ( 13.64836464229338198, 15.83060743948028737, -232.0893758582176929 ) ) ;
#6422=CARTESIAN_POINT ( 'NONE',  ( -10.32994309255856535, 16.55762392127841665, -218.3313395458419279 ) ) ;
#6423=CARTESIAN_POINT ( 'NONE',  ( -5.383332542724544645, 15.12651309054520432, -231.5699995578976313 ) ) ;
#6426=CARTESIAN_POINT ( 'NONE',  ( -14.92584319327083442, -9.764953932613968490, -229.6443584147421006 ) ) ;
#6427=CARTESIAN_POINT ( 'NONE',  ( 22.17049319811867036, 0.5483778423327810847, -216.5715983009590673 ) ) ;
#6430=CARTESIAN_POINT ( 'NONE',  ( -17.75199675706278413, -2.086992369311378326, -216.9839424855219931 ) ) ;
#6431=CARTESIAN_POINT ( 'NONE',  ( 12.95792863868717149, 16.83236386576623644, -216.3406066345214356 ) ) ;
#6432=CARTESIAN_POINT ( 'NONE',  ( -19.33106196848021341, 9.919700385716687663, -219.0532654734256255 ) ) ;
#6433=CARTESIAN_POINT ( 'NONE',  ( -2.047892494109819328, 12.88402507277750786, -223.5104301352110951 ) ) ;
#6434=CARTESIAN_POINT ( 'NONE',  ( 16.20788843645364352, 6.828976201867700269, -231.6689701909764665 ) ) ;
#6435=CARTESIAN_POINT ( 'NONE',  ( -20.34211109426514597, -24.21145056749966074, -225.0780941718357724 ) ) ;
#6437=CARTESIAN_POINT ( 'NONE',  ( -13.66944713747931139, -25.56883467164384527, -222.3908458502962731 ) ) ;
#6438=CARTESIAN_POINT ( 'NONE',  ( -13.09048442463468120, -0.002406630494250819839, -229.7150300986316438 ) ) ;
#6439=CARTESIAN_POINT ( 'NONE',  ( 12.02378739738799140, -16.98783239109716092, -233.4545636224233931 ) ) ;
#6440=CARTESIAN_POINT ( 'NONE',  ( -16.64477864544768337, -2.947896226079009807, -219.6737919733007516 ) ) ;
#6441=CARTESIAN_POINT ( 'NONE',  ( -22.23616899077527975, -11.51447210886970751, -217.5950109096934568 ) ) ;
#6442=CARTESIAN_POINT ( 'NONE',  ( 19.13999328532042910, 9.776920959053244431, -216.1190985676915375 ) ) ;
#6444=CARTESIAN_POINT ( 'NONE',  ( -13.71158422780231056, 12.21432067443984693, -232.9166272955793033 ) ) ;
#6445=CARTESIAN_POINT ( 'NONE',  ( 11.35656094503625901, 14.01405796444069018, -230.6944611846958537 ) ) ;
#6446=CARTESIAN_POINT ( 'NONE',  ( 4.603870848087811218, 30.13529352683433515, -225.9623629403671430 ) ) ;
#6447=CARTESIAN_POINT ( 'NONE',  ( 12.14863411169100971, 10.95505907656739097, -219.3725293661985063 ) ) ;
#6448=CARTESIAN_POINT ( 'NONE',  ( 12.92161125358352791, -8.797851723037126703, -217.2061419145261425 ) ) ;
#6449=CARTESIAN_POINT ( 'NONE',  ( -10.10782416658048710, 9.083762506436128703, -227.1045422723873344 ) ) ;
#6450=CARTESIAN_POINT ( 'NONE',  ( -0.7286890422672397394, 21.00519367000705273, -234.2149015821977969 ) ) ;
#6451=CARTESIAN_POINT ( 'NONE',  ( -12.50828242918857036, -25.45147276965577277, -228.7626325223041022 ) ) ;
#6452=CARTESIAN_POINT ( 'NONE',  ( -13.92046207272054303, -0.1600067567908077248, -224.5811699126800818 ) ) ;
#6455=CARTESIAN_POINT ( 'NONE',  ( 14.85123888640019452, 5.067529763532427012, -221.9058491819374979 ) ) ;
#6456=CARTESIAN_POINT ( 'NONE',  ( 15.55571562362403704, -22.93410568583619025, -228.9591035895856805 ) ) ;
#6457=CARTESIAN_POINT ( 'NONE',  ( -13.97943781666340790, 5.798109546139844639, -228.2992319913466019 ) ) ;
#6458=CARTESIAN_POINT ( 'NONE',  ( 5.359747511823000465, 20.14556701535824601, -232.9094821222151381 ) ) ;
#6459=CARTESIAN_POINT ( 'NONE',  ( -12.14186164972853810, -9.217338937739926408, -220.4665480714278374 ) ) ;
#6461=CARTESIAN_POINT ( 'NONE',  ( 13.93840998928060415, 0.7705246578886114639, -220.8158265847476116 ) ) ;
#6462=CARTESIAN_POINT ( 'NONE',  ( 14.28815361401014172, 13.86049093364188778, -216.0585456615740156 ) ) ;
#6464=CARTESIAN_POINT ( 'NONE',  ( -5.807479211365208727, 19.77444019604324410, -216.0778658752277863 ) ) ;
#6465=CARTESIAN_POINT ( 'NONE',  ( 17.73959705210031146, -11.46016327460725748, -231.4839417819510459 ) ) ;
#6468=CARTESIAN_POINT ( 'NONE',  ( 4.883314309504700468, 19.06839645569368358, -217.0171359871271193 ) ) ;
#6469=CARTESIAN_POINT ( 'NONE',  ( -14.97068153222459408, -28.62142063984003215, -225.0224449979507142 ) ) ;
#6470=CARTESIAN_POINT ( 'NONE',  ( 10.10435529162921853, -13.32996982371095918, -231.5224098423250894 ) ) ;
#6472=CARTESIAN_POINT ( 'NONE',  ( -20.80338291456855870, 18.97067006663518995, -230.9007617602332516 ) ) ;
#6473=CARTESIAN_POINT ( 'NONE',  ( 10.48640380280471618, 25.27581435651469022, -227.8976696013017715 ) ) ;
#6475=CARTESIAN_POINT ( 'NONE',  ( -19.94037810645588138, 20.40093185429846656, -220.0593903119159620 ) ) ;
#6476=CARTESIAN_POINT ( 'NONE',  ( -18.52912398332900068, -6.554396152115366192, -218.2980051671528088 ) ) ;
#6478=CARTESIAN_POINT ( 'NONE',  ( -10.84440549681320221, 27.00404139634608214, -224.0969657459751261 ) ) ;
#6479=CARTESIAN_POINT ( 'NONE',  ( 22.73582563804385970, 20.20868311426415431, -227.8513184012435886 ) ) ;
#6480=CARTESIAN_POINT ( 'NONE',  ( 1.984991703947643904, 14.51738422979996912, -218.4500278854917781 ) ) ;
#6481=CARTESIAN_POINT ( 'NONE',  ( 16.07480884343054939, -7.767425703123992164, -217.5935768756353923 ) ) ;
#6483=CARTESIAN_POINT ( 'NONE',  ( -14.00380962569832199, 8.747390586476997854, -231.7950903513155936 ) ) ;
#6484=CARTESIAN_POINT ( 'NONE',  ( -24.53655852862112496, -9.573911656693818273, -234.4221496410225143 ) ) ;
#6486=CARTESIAN_POINT ( 'NONE',  ( 12.04687593227112430, 27.54339840196571743, -224.6466266724203820 ) ) ;
#6490=CARTESIAN_POINT ( 'NONE',  ( -14.87984907657228639, 0.2138881189739126887, -228.7773920408832282 ) ) ;
#6491=CARTESIAN_POINT ( 'NONE',  ( -16.48591407464216729, 7.092323989942422635, -218.8909951703408012 ) ) ;
#6492=CARTESIAN_POINT ( 'NONE',  ( 13.15438416660314225, 5.520603777723624539, -227.0878346348094681 ) ) ;
#6493=( NAMED_UNIT ( * ) PLANE_ANGLE_UNIT ( ) SI_UNIT ( $, .RADIAN. ) );
#6495=CARTESIAN_POINT ( 'NONE',  ( 14.98418162551161714, 4.450317369940187895, -227.9894155827521161 ) ) ;
#6497=CARTESIAN_POINT ( 'NONE',  ( 23.75342044390781027, -1.773323855525749781, -231.1605140052801630 ) ) ;
#6498=CARTESIAN_POINT ( 'NONE',  ( -16.39524763169126942, -10.97410814576847926, -232.9630882351523837 ) ) ;
#6502=CARTESIAN_POINT ( 'NONE',  ( 5.142103055192286831, 28.18228231877369439, -225.8998064704803994 ) ) ;
#6503=CARTESIAN_POINT ( 'NONE',  ( 19.43707201973751708, -21.22621598813149646, -232.3303264720597667 ) ) ;
#6504=CARTESIAN_POINT ( 'NONE',  ( 10.99893791904045415, -12.61823049403341201, -218.3266956685045841 ) ) ;
#6506=CARTESIAN_POINT ( 'NONE',  ( -12.78923236353123727, 15.53885160143439315, -231.8946633672937878 ) ) ;
#6507=CARTESIAN_POINT ( 'NONE',  ( 12.23284375931666013, 4.108221165122169616, -224.0993108960438462 ) ) ;
#6508=CARTESIAN_POINT ( 'NONE',  ( 16.23850682336481199, 8.051046992137072422, -219.2473483181185827 ) ) ;
#6510=CARTESIAN_POINT ( 'NONE',  ( -6.954422770286640798, -15.70181985945210634, -221.3390676453758488 ) ) ;
#6512=CARTESIAN_POINT ( 'NONE',  ( -15.39319649241581800, 0.3563955590804028795, -232.4397289486159082 ) ) ;
#6513=CARTESIAN_POINT ( 'NONE',  ( 9.100443535964535258, 24.01370002727352215, -234.5397711707082635 ) ) ;
#6514=CARTESIAN_POINT ( 'NONE',  ( 27.02504508796729255, -10.76203424748690907, -225.6681254905965943 ) ) ;
#6516=CARTESIAN_POINT ( 'NONE',  ( 4.340445191644851874, 29.86837761166362881, -227.4879512554873315 ) ) ;
#6517=CARTESIAN_POINT ( 'NONE',  ( -17.88126539071149779, 5.766250685202066961, -232.9050303536861293 ) ) ;
#6518=B_SPLINE_CURVE_WITH_KNOTS ( 'NONE', 3,
 ( #16864, #3338, #22251, #13712, #18985, #15180, #1439, #10109, #12020, #10442, #8429, #8312, #13830, #10220, #13486, #20326, #20440, #87, #8541, #15405, #5138, #18878, #3454, #11799, #4923, #20666, #18666, #3226, #16974, #1553, #10333, #1772, #8646, #12130, #15507, #6958, #3564, #17302, #8761, #15621, #2429, #21110, #9312, #743, #10670, #17422, #17867, #17640 ),
 .UNSPECIFIED., .F., .F.,
 ( 4, 2, 2, 2, 2, 2, 2, 2, 2, 2, 2, 2, 2, 2, 2, 2, 2, 2, 2, 2, 2, 2, 2, 4 ),
 ( 0.004817815020603932220, 0.005107125076144584247, 0.005396435131685235406, 0.005685745187225887433, 0.005975055242766539459, 0.006553675353847844380, 0.006842985409388494672, 0.007132295464929145831, 0.007710915576010501926, 0.008289535687091858021, 0.008868155798173214116, 0.009446775909254571946, 0.01002539602033592978, 0.01060401613141728414, 0.01118263624249864197, 0.01176125635357999979, 0.01205056640912068044, 0.01233987646466135762, 0.01262918652020203827, 0.01291849657574271892, 0.01320780663128339610, 0.01349711668682407675, 0.01378642674236475740, 0.01407573679790543458 ),
 .UNSPECIFIED. ) ;
#6519=CARTESIAN_POINT ( 'NONE',  ( 8.036750260989780514, 26.29729070384984624, -233.5018314387838529 ) ) ;
#6520=CARTESIAN_POINT ( 'NONE',  ( -27.01279207917464475, 4.316569700791554887, -221.4451031230926219 ) ) ;
#6521=CARTESIAN_POINT ( 'NONE',  ( -3.501680520304516264, 14.31538576447642264, -219.8967178229432307 ) ) ;
#6523=CARTESIAN_POINT ( 'NONE',  ( 14.96080648943632241, 22.28365808184747721, -220.1237743409445216 ) ) ;
#6527=CARTESIAN_POINT ( 'NONE',  ( 27.04607490430786854, 4.607450003618843049, -220.3758934308003461 ) ) ;
#6528=CARTESIAN_POINT ( 'NONE',  ( -13.13160344394316503, -9.470348871083606568, -223.0142826039989075 ) ) ;
#6531=CARTESIAN_POINT ( 'NONE',  ( -9.661739055621840322, 20.41227307912577871, -232.0920144483423257 ) ) ;
#6533=CARTESIAN_POINT ( 'NONE',  ( 3.619268272960482591, -21.10655420957111517, -217.8630709410095108 ) ) ;
#6534=CARTESIAN_POINT ( 'NONE',  ( 14.91731358302415877, 13.33846450914490056, -217.2468882285060658 ) ) ;
#6535=CARTESIAN_POINT ( 'NONE',  ( -4.466732464217805898, 19.42663028452474450, -231.9485309169485561 ) ) ;
#6536=CARTESIAN_POINT ( 'NONE',  ( -5.298027976154672025, 13.43376398981453157, -220.6333279128949982 ) ) ;
#6537=CARTESIAN_POINT ( 'NONE',  ( -24.13163560393529394, -13.84165259829251227, -223.2936513752361805 ) ) ;
#6539=CARTESIAN_POINT ( 'NONE',  ( 8.812073984913094904, 13.12649198322903210, -229.9172071780580495 ) ) ;
#6540=CARTESIAN_POINT ( 'NONE',  ( -28.00010259152825398, 3.831607968041374157, -225.8381323513402208 ) ) ;
#6543=CARTESIAN_POINT ( 'NONE',  ( -14.73876579896802141, -0.4225899574144328374, -230.2531052195884342 ) ) ;
#6544=CARTESIAN_POINT ( 'NONE',  ( 13.20340559785743828, 9.575208899273587093, -218.1210831379648312 ) ) ;
#6545=CARTESIAN_POINT ( 'NONE',  ( -22.90687623753526125, 9.466200233939549236, -230.1557007022273638 ) ) ;
#6546=CARTESIAN_POINT ( 'NONE',  ( 8.546572992885776543, 19.06776382077057974, -214.7173484156796519 ) ) ;
#6547=CARTESIAN_POINT ( 'NONE',  ( 23.83082175545800752, 15.77842900014857896, -219.5351905769044834 ) ) ;
#6549=CARTESIAN_POINT ( 'NONE',  ( -8.875208054371373834, -23.27682998066124398, -233.1222812539844540 ) ) ;
#6551=ORIENTED_EDGE ( 'NONE', *, *, #18200, .T. ) ;
#6552=CARTESIAN_POINT ( 'NONE',  ( -10.03082531488024109, -22.09229706162428286, -231.9736132431984572 ) ) ;
#6553=CARTESIAN_POINT ( 'NONE',  ( -21.85741505224184777, 1.741064654082184582, -235.1654459941842390 ) ) ;
#6554=CARTESIAN_POINT ( 'NONE',  ( 13.47054497134856277, -24.75371201277411615, -218.7687119198782000 ) ) ;
#6555=CARTESIAN_POINT ( 'NONE',  ( 11.88751558872989378, -3.770303194171726435, -225.3699946362665969 ) ) ;
#6556=CARTESIAN_POINT ( 'NONE',  ( -20.85586116824185510, -1.996934699305910499, -232.3804859832740135 ) ) ;
#6557=CARTESIAN_POINT ( 'NONE',  ( 25.40172858355122898, 15.07073195964820833, -229.0276483847865450 ) ) ;
#6559=CARTESIAN_POINT ( 'NONE',  ( -15.57505478537380306, 24.84242291948262249, -225.5907943047649837 ) ) ;
#6560=CARTESIAN_POINT ( 'NONE',  ( 12.49127101283658803, 6.474961340449192804, -221.2149164507559078 ) ) ;
#6561=CARTESIAN_POINT ( 'NONE',  ( 15.33737796850231305, 13.57479350230705428, -232.3313557812109025 ) ) ;
#6562=CARTESIAN_POINT ( 'NONE',  ( 8.778334628954494789, 12.71782457734010841, -222.1923057070808909 ) ) ;
#6563=CARTESIAN_POINT ( 'NONE',  ( 22.36312131198404174, -23.32398317548372546, -224.0789201928890861 ) ) ;
#6564=CARTESIAN_POINT ( 'NONE',  ( -2.917590128672695293, 18.81591489065672818, -216.3635620530855022 ) ) ;
#6565=ADVANCED_FACE ( 'NONE', ( #2995 ), #14510, .F. ) ;
#6570=CARTESIAN_POINT ( 'NONE',  ( 10.83706092800007781, 10.12544885278926543, -227.1716144446442343 ) ) ;
#6571=CARTESIAN_POINT ( 'NONE',  ( 3.737871636182809265, -14.23896033977216113, -229.0757302894822942 ) ) ;
#6572=CARTESIAN_POINT ( 'NONE',  ( -26.38808873681881906, 13.30696350521622939, -225.1492950792419663 ) ) ;
#6573=CARTESIAN_POINT ( 'NONE',  ( 3.160467108836292116, 14.95099014189016629, -228.9242958482614370 ) ) ;
#6574=CARTESIAN_POINT ( 'NONE',  ( -13.67406442719345883, -9.319000780081536206, -231.1492214949047934 ) ) ;
#6576=CARTESIAN_POINT ( 'NONE',  ( -23.52458685063474420, 4.195399146287285497, -230.7490123595086970 ) ) ;
#6577=CARTESIAN_POINT ( 'NONE',  ( 20.05374812456133782, 24.17492691056345677, -223.1494843338164458 ) ) ;
#6578=EDGE_LOOP ( 'NONE', ( #14497, #16847 ) ) ;
#6579=CARTESIAN_POINT ( 'NONE',  ( -0.1571923090946999446, 19.34188126963334398, -216.6893131123363787 ) ) ;
#6580=CARTESIAN_POINT ( 'NONE',  ( 13.61677703237491777, -11.64725695657166682, -220.6715806775949034 ) ) ;
#6581=CARTESIAN_POINT ( 'NONE',  ( 24.14841045621385263, -15.62485098017456586, -229.9279278555176518 ) ) ;
#6583=CARTESIAN_POINT ( 'NONE',  ( 6.093530912645064745, 16.79941505724243811, -232.1766444656230419 ) ) ;
#6584=CARTESIAN_POINT ( 'NONE',  ( -12.06899374386015644, -4.263779665926158202, -221.6855044605631520 ) ) ;
#6585=CARTESIAN_POINT ( 'NONE',  ( 5.609436632608550966, -13.11664087352601094, -229.3324225951633650 ) ) ;
#6587=CARTESIAN_POINT ( 'NONE',  ( 14.99336262864975211, -23.54026314425397004, -231.3018640253376361 ) ) ;
#6589=CARTESIAN_POINT ( 'NONE',  ( -25.00745438246740804, 14.90779342625281778, -219.2410538611701156 ) ) ;
#6590=CARTESIAN_POINT ( 'NONE',  ( 14.78510113471881304, 14.77128235908076803, -230.8056908117964383 ) ) ;
#6591=CARTESIAN_POINT ( 'NONE',  ( -17.88126539071149779, 5.766250685202066961, -232.9050303536861293 ) ) ;
#6592=CARTESIAN_POINT ( 'NONE',  ( -14.83806045519817829, 13.18806197935771074, -233.4179411789645542 ) ) ;
#6593=CARTESIAN_POINT ( 'NONE',  ( -14.04666385475200485, -11.54975518965215286, -229.4392169170632201 ) ) ;
#6595=CARTESIAN_POINT ( 'NONE',  ( -8.857704405076667342, 24.20848540845601704, -218.8859504303524091 ) ) ;
#6597=CARTESIAN_POINT ( 'NONE',  ( 11.63337745479824292, 8.229076005436313679, -220.5472098800687206 ) ) ;
#6598=CARTESIAN_POINT ( 'NONE',  ( 2.165130313308041288, 31.55305250914585002, -225.6791154433767304 ) ) ;
#6599=CARTESIAN_POINT ( 'NONE',  ( 25.09678678204237201, -16.96620885351193309, -225.7902784465786965 ) ) ;
#6602=CARTESIAN_POINT ( 'NONE',  ( -14.73016414256368911, 22.23431809695627237, -217.1425123644553707 ) ) ;
#6603=CARTESIAN_POINT ( 'NONE',  ( -8.622882141441040815, -8.945706011589379614, -222.9266619361505377 ) ) ;
#6605=CARTESIAN_POINT ( 'NONE',  ( 18.50911814746675788, 15.92944434255054453, -232.0449215596906072 ) ) ;
#6608=CARTESIAN_POINT ( 'NONE',  ( 13.28406271702445274, -5.237238614233280742, -225.2640488721434622 ) ) ;
#6609=CARTESIAN_POINT ( 'NONE',  ( -28.59157645096996347, 5.137867505054540374, -220.4667042235044505 ) ) ;
#6610=CARTESIAN_POINT ( 'NONE',  ( -12.99458409358603284, 11.56864380452031504, -232.0274663316965018 ) ) ;
#6611=CARTESIAN_POINT ( 'NONE',  ( 16.31458447723494132, 2.619382102851042671, -229.5862799001085364 ) ) ;
#6612=CARTESIAN_POINT ( 'NONE',  ( -7.972347216402701164, -18.74702622849856937, -232.1058264431568148 ) ) ;
#6616=CARTESIAN_POINT ( 'NONE',  ( 19.27468327664662695, -19.23223527390535637, -221.0469535581208618 ) ) ;
#6620=CARTESIAN_POINT ( 'NONE',  ( 10.63406535173453271, 22.16595115341124256, -219.6461356279925781 ) ) ;
#6621=CARTESIAN_POINT ( 'NONE',  ( 17.90345650676399814, -22.75668921074696982, -218.1849408917474022 ) ) ;
#6622=CARTESIAN_POINT ( 'NONE',  ( 12.70477135646371281, -9.814387909761604689, -230.3443492180780652 ) ) ;
#6623=EDGE_LOOP ( 'NONE', ( #14938, #18806 ) ) ;
#6624=CARTESIAN_POINT ( 'NONE',  ( -17.78731991475362406, 16.78509880370027929, -218.2387321183659310 ) ) ;
#6625=CARTESIAN_POINT ( 'NONE',  ( -17.29038495093124084, 2.707785585324113065, -229.0475017805649998 ) ) ;
#6626=CARTESIAN_POINT ( 'NONE',  ( 14.37653162493774239, 9.985418694807894013, -229.1686718965858063 ) ) ;
#6629=CARTESIAN_POINT ( 'NONE',  ( -8.783466540727490113, -25.47690852953548557, -220.9562114332719318 ) ) ;
#6631=CARTESIAN_POINT ( 'NONE',  ( -28.12586305337175219, 12.75764838638491305, -230.3810511299127768 ) ) ;
#6632=CARTESIAN_POINT ( 'NONE',  ( 13.06625079052675531, 10.14096931681969238, -232.1435240729728093 ) ) ;
#6633=CARTESIAN_POINT ( 'NONE',  ( 9.790069677392189362, -14.58761328102826837, -228.7245293813585647 ) ) ;
#6634=CARTESIAN_POINT ( 'NONE',  ( 11.82943521288609823, 27.58963564415041247, -226.1180395413371400 ) ) ;
#6635=CARTESIAN_POINT ( 'NONE',  ( -29.88125065636863198, 4.504452993877526623, -226.2048141718237275 ) ) ;
#6637=CARTESIAN_POINT ( 'NONE',  ( 10.66732316618037402, 25.78610527446713263, -216.5597036843431624 ) ) ;
#6638=CARTESIAN_POINT ( 'NONE',  ( -13.66744685701839046, 5.938820276054873837, -223.0954633396572149 ) ) ;
#6639=CARTESIAN_POINT ( 'NONE',  ( -6.101488798441174310, 11.33371047077072369, -225.3616985956418546 ) ) ;
#6641=CARTESIAN_POINT ( 'NONE',  ( 18.06016678184731461, 2.257982981100609354, -218.9983079406065940 ) ) ;
#6642=CARTESIAN_POINT ( 'NONE',  ( 3.689800395305025127, 23.07294874520714956, -219.2515233573129478 ) ) ;
#6643=CARTESIAN_POINT ( 'NONE',  ( 28.33476664927451338, -0.7768526459456059907, -228.3750448408243869 ) ) ;
#6645=CARTESIAN_POINT ( 'NONE',  ( -22.20848920810297855, -2.028924892417935055, -232.4401719831211039 ) ) ;
#6646=CARTESIAN_POINT ( 'NONE',  ( 17.07668571305246985, 2.037405138410691485, -219.7626854147787867 ) ) ;
#6647=CARTESIAN_POINT ( 'NONE',  ( -12.96306772261163154, -8.963621967909368493, -225.1938837381851215 ) ) ;
#6649=CARTESIAN_POINT ( 'NONE',  ( -8.030397104878142400, 15.90963402996711373, -230.6518438502475590 ) ) ;
#6651=CARTESIAN_POINT ( 'NONE',  ( 1.632321987819951969, -14.78074153629778387, -224.5834756332612301 ) ) ;
#6652=CARTESIAN_POINT ( 'NONE',  ( 26.51393280883522863, 15.12455065102723495, -226.1955201378414415 ) ) ;
#6653=CARTESIAN_POINT ( 'NONE',  ( -10.84440549681320221, 27.00404139634608214, -224.0969657459751261 ) ) ;
#6654=CARTESIAN_POINT ( 'NONE',  ( -16.96626096607909417, 26.06638125783293347, -227.3272535207661349 ) ) ;
#6656=CARTESIAN_POINT ( 'NONE',  ( 29.48160760559006732, -8.328447718542550504, -230.7159994440206390 ) ) ;
#6658=CARTESIAN_POINT ( 'NONE',  ( 14.31308345469695453, 12.76656023072872159, -231.9445021321040770 ) ) ;
#6659=CARTESIAN_POINT ( 'NONE',  ( -26.88784739727922357, 10.07520213145270915, -227.1866063047054922 ) ) ;
#6660=CARTESIAN_POINT ( 'NONE',  ( -16.29666348338687953, 2.994680995215331709, -221.2421885839926006 ) ) ;
#6663=CARTESIAN_POINT ( 'NONE',  ( -13.18205254385204661, -0.5588607053421433823, -223.2849229087554761 ) ) ;
#6664=CARTESIAN_POINT ( 'NONE',  ( 8.554868430186942874, 10.42313681336814568, -223.0114508542762621 ) ) ;
#6665=CARTESIAN_POINT ( 'NONE',  ( -26.35007260221545877, 6.140745174321167177, -221.9336216792591188 ) ) ;
#6666=CARTESIAN_POINT ( 'NONE',  ( 7.651502705057454889, 16.60422307457919544, -215.4679461133464144 ) ) ;
#6667=CARTESIAN_POINT ( 'NONE',  ( 18.39533937270110187, 14.26564464607222504, -233.9088367426310242 ) ) ;
#6668=CARTESIAN_POINT ( 'NONE',  ( -8.622882141441040815, -8.945706011589379614, -222.9266619361505377 ) ) ;
#6670=CARTESIAN_POINT ( 'NONE',  ( -5.139154528335864391, -14.05392405596956529, -226.2842807754188641 ) ) ;
#6672=CARTESIAN_POINT ( 'NONE',  ( -16.95112677453439431, 10.32962960657076934, -214.9445123409346650 ) ) ;
#6673=CARTESIAN_POINT ( 'NONE',  ( 5.609436632608550966, -13.11664087352601094, -229.3324225951633650 ) ) ;
#6674=CARTESIAN_POINT ( 'NONE',  ( -3.003186468682855104, 15.63968344752823469, -231.5301608670590667 ) ) ;
#6675=CARTESIAN_POINT ( 'NONE',  ( 29.76850351104168979, -8.061840962539296385, -221.9850081079297581 ) ) ;
#6676=CARTESIAN_POINT ( 'NONE',  ( -19.88402822078561627, -6.951120502836210413, -232.7962440186676361 ) ) ;
#6677=AXIS2_PLACEMENT_3D ( 'NONE', #18028, #16226, #2707 ) ;
#6678=CARTESIAN_POINT ( 'NONE',  ( 12.49127101283658803, 6.474961340449192804, -221.2149164507559078 ) ) ;
#6680=CARTESIAN_POINT ( 'NONE',  ( -12.67136363292824086, 22.56975222910433843, -219.0840033572168011 ) ) ;
#6681=CARTESIAN_POINT ( 'NONE',  ( 25.40172858355122898, 15.07073195964820833, -229.0276483847865450 ) ) ;
#6682=CARTESIAN_POINT ( 'NONE',  ( 11.57669841200422134, 10.63052136557218574, -228.9489978335593889 ) ) ;
#6683=CARTESIAN_POINT ( 'NONE',  ( 7.249842700832647147, 18.24319783868832801, -219.1110502051974720 ) ) ;
#6684=CARTESIAN_POINT ( 'NONE',  ( 3.531840179394873491, -11.29480931768500618, -224.5922842895475355 ) ) ;
#6685=CARTESIAN_POINT ( 'NONE',  ( -5.854583994961135573, 13.10358817970001866, -222.4168379437668648 ) ) ;
#6686=CARTESIAN_POINT ( 'NONE',  ( -13.69675006931110417, 3.702342960760605539, -228.0723273272095355 ) ) ;
#6688=CARTESIAN_POINT ( 'NONE',  ( 8.072455080350884771, -13.51419333260225741, -221.0758372092125228 ) ) ;
#6689=CARTESIAN_POINT ( 'NONE',  ( -16.81936022032888545, 5.700806722825413786, -218.5726178058217215 ) ) ;
#6691=CARTESIAN_POINT ( 'NONE',  ( -4.784012432433236484, 23.31984772163034947, -232.0554186943449508 ) ) ;
#6693=CARTESIAN_POINT ( 'NONE',  ( -14.40111287326894640, -6.123720356435734757, -220.5571602876142094 ) ) ;
#6694=CARTESIAN_POINT ( 'NONE',  ( 29.11492790716816614, 6.132849117128307270, -229.8316941169402412 ) ) ;
#6695=CARTESIAN_POINT ( 'NONE',  ( 19.29971334243027314, 24.42889259816135095, -228.2141526116784291 ) ) ;
#6697=CARTESIAN_POINT ( 'NONE',  ( -10.45786516112131892, 23.61456281964591852, -233.2869923610001592 ) ) ;
#6698=CARTESIAN_POINT ( 'NONE',  ( 18.69377297094946755, -6.763382089143314957, -232.1160126380615338 ) ) ;
#6699=CARTESIAN_POINT ( 'NONE',  ( 15.56514059923893178, -9.210181625211102840, -232.5361143517874325 ) ) ;
#6700=CARTESIAN_POINT ( 'NONE',  ( -11.33137429837660193, 27.25022425932026238, -230.1650924901870212 ) ) ;
#6702=CARTESIAN_POINT ( 'NONE',  ( 10.66614775643814994, 26.29080367171353672, -230.0818785118670178 ) ) ;
#6703=CARTESIAN_POINT ( 'NONE',  ( -18.15502857810558268, -5.877683472035677426, -234.3930847616834683 ) ) ;
#6704=CARTESIAN_POINT ( 'NONE',  ( -11.40116373163465369, -15.95513543764466213, -216.7841692646331353 ) ) ;
#6705=CARTESIAN_POINT ( 'NONE',  ( 7.958080982411646076, -16.12895853103474408, -217.0903302464454612 ) ) ;
#6706=CARTESIAN_POINT ( 'NONE',  ( -9.403561938624596550, 12.70246821120386471, -220.7484614495429582 ) ) ;
#6707=CARTESIAN_POINT ( 'NONE',  ( 16.29563576379945999, 21.41235115595959826, -221.8114656550040991 ) ) ;
#6708=CARTESIAN_POINT ( 'NONE',  ( -22.04257564474043818, 18.72061943465525857, -219.1781831295219263 ) ) ;
#6709=CARTESIAN_POINT ( 'NONE',  ( -27.17783334270200157, 15.20409188923851751, -223.6555185980277258 ) ) ;
#6710=CARTESIAN_POINT ( 'NONE',  ( -14.97948828349161232, -4.621108923465524931, -227.6270126398174796 ) ) ;
#6713=CARTESIAN_POINT ( 'NONE',  ( -4.866400999161825780, 25.69921167300892861, -231.0100031340613782 ) ) ;
#6714=CARTESIAN_POINT ( 'NONE',  ( 10.70175380652492336, 7.370128018021000038, -224.3479584370086286 ) ) ;
#6715=CARTESIAN_POINT ( 'NONE',  ( 8.865150807857233417, 8.939496441981303221, -220.7647208555746090 ) ) ;
#6716=CARTESIAN_POINT ( 'NONE',  ( 10.52067862919218832, -10.34113464825721351, -228.4460540958991714 ) ) ;
#6719=CARTESIAN_POINT ( 'NONE',  ( -3.205260335674071648, 17.52234722004434531, -232.9754319808710363 ) ) ;
#6720=CARTESIAN_POINT ( 'NONE',  ( -19.24125987773642166, -8.201885216777814236, -235.2928755229699789 ) ) ;
#6721=EDGE_CURVE ( 'NONE', #6170, #13407, #6518, .T. ) ;
#6723=CARTESIAN_POINT ( 'NONE',  ( 14.22574309452842733, 4.476723532073429546, -225.5862451792618231 ) ) ;
#6725=CARTESIAN_POINT ( 'NONE',  ( 11.39114332821395692, -8.257479203742953189, -226.5648397932267528 ) ) ;
#6727=CARTESIAN_POINT ( 'NONE',  ( -24.48580119005125866, 9.312492396273500006, -232.5498413856076070 ) ) ;
#6729=CARTESIAN_POINT ( 'NONE',  ( 18.69835413980967687, -1.262199651413310031, -230.6153330080101966 ) ) ;
#6730=CARTESIAN_POINT ( 'NONE',  ( -13.55429797312971374, -24.97278848321653300, -221.1627755146857908 ) ) ;
#6734=CARTESIAN_POINT ( 'NONE',  ( 20.29112488791128399, -13.23242053965672049, -219.3899762660180102 ) ) ;
#6737=CARTESIAN_POINT ( 'NONE',  ( 9.322595869360968734, 23.38184458253662967, -230.2763482547081821 ) ) ;
#6738=CARTESIAN_POINT ( 'NONE',  ( 2.482746429915354547, 16.41797261123590346, -229.5599230346982154 ) ) ;
#6739=CARTESIAN_POINT ( 'NONE',  ( 6.889583945421565048, -13.03635046449108081, -231.0237689561592731 ) ) ;
#6740=CARTESIAN_POINT ( 'NONE',  ( 13.99926435381047618, -21.11851526759364006, -232.9234173943665951 ) ) ;
#6742=CARTESIAN_POINT ( 'NONE',  ( -7.240690404266621805, 13.01623002570985044, -225.3000933658701967 ) ) ;
#6743=CARTESIAN_POINT ( 'NONE',  ( -21.18474081038989354, 8.486062504918864491, -230.7949373529753530 ) ) ;
#6744=CARTESIAN_POINT ( 'NONE',  ( 23.24653631066306048, 11.83805845626388020, -219.6020901153134162 ) ) ;
#6746=CARTESIAN_POINT ( 'NONE',  ( -8.081326109241135924, -15.70152450856234871, -229.3783721713404304 ) ) ;
#6749=CARTESIAN_POINT ( 'NONE',  ( 3.672031556878595282, 11.54613252248376831, -227.4694100414545801 ) ) ;
#6750=CARTESIAN_POINT ( 'NONE',  ( 17.97642781552999836, -18.85565020944788373, -229.3765379620127760 ) ) ;
#6751=CARTESIAN_POINT ( 'NONE',  ( 12.53674998645855787, 17.96979015029927851, -232.8843215672231679 ) ) ;
#6752=CARTESIAN_POINT ( 'NONE',  ( -14.87984907657228639, 0.2138881189739126887, -228.7773920408832282 ) ) ;
#6753=CARTESIAN_POINT ( 'NONE',  ( 5.784594921161807513, 11.98867617302893329, -219.3746160931291058 ) ) ;
#6754=CARTESIAN_POINT ( 'NONE',  ( -14.30096418567650041, 6.974026439069829664, -228.7941652905285537 ) ) ;
#6755=CARTESIAN_POINT ( 'NONE',  ( -7.429838964355703901, 14.87322129099639234, -232.2632863647814077 ) ) ;
#6757=CARTESIAN_POINT ( 'NONE',  ( 4.682724365302521896, -22.35092628325669750, -215.9543778044225348 ) ) ;
#6760=CARTESIAN_POINT ( 'NONE',  ( -27.09167109716269550, -0.2825935922571593539, -219.8389404328913486 ) ) ;
#6761=CARTESIAN_POINT ( 'NONE',  ( 17.34727976380017722, 4.822939981779328811, -230.8836217450937909 ) ) ;
#6762=CARTESIAN_POINT ( 'NONE',  ( -12.44262610342426711, -20.67338498558408588, -232.3867413080560027 ) ) ;
#6765=CARTESIAN_POINT ( 'NONE',  ( 5.133806223762193532, -16.42362916962670383, -230.4968203642818310 ) ) ;
#6766=CARTESIAN_POINT ( 'NONE',  ( 25.30228294196351868, 7.987863777258004561, -233.0744943826964573 ) ) ;
#6767=CARTESIAN_POINT ( 'NONE',  ( -17.08384421609436643, 23.56421365837046622, -225.2902702884460666 ) ) ;
#6768=CARTESIAN_POINT ( 'NONE',  ( -11.23881320317003407, 15.84151802331611236, -234.2799649731619809 ) ) ;
#6770=CARTESIAN_POINT ( 'NONE',  ( -26.10238271615538252, -1.908654064438627174, -220.4792571320490708 ) ) ;
#6771=ORIENTED_EDGE ( 'NONE', *, *, #6721, .F. ) ;
#6772=CARTESIAN_POINT ( 'NONE',  ( 7.743212835174657194, 11.90778931056080481, -226.0491028376908105 ) ) ;
#6773=CARTESIAN_POINT ( 'NONE',  ( -15.60078324628501356, 3.527872497691606934, -227.4630248446626695 ) ) ;
#6774=CARTESIAN_POINT ( 'NONE',  ( 29.64577750251057608, 2.839131411071813549, -220.9704389295326905 ) ) ;
#6776=CARTESIAN_POINT ( 'NONE',  ( 14.60728983664449387, 19.38727400458104455, -216.6381802409380555 ) ) ;
#6777=CARTESIAN_POINT ( 'NONE',  ( -15.65611835717891687, 5.486779671999271635, -227.0554626315911264 ) ) ;
#6778=CARTESIAN_POINT ( 'NONE',  ( -0.9851030586975465519, 19.34066537597387381, -233.8273485600932418 ) ) ;
#6779=CARTESIAN_POINT ( 'NONE',  ( 17.66865342763861690, 2.849170916951684784, -230.9175656266857004 ) ) ;
#6780=CARTESIAN_POINT ( 'NONE',  ( -13.37406041957185110, -11.77244451953823834, -233.9958171493936732 ) ) ;
#6782=CARTESIAN_POINT ( 'NONE',  ( -12.50828242918857036, -25.45147276965577277, -228.7626325223041022 ) ) ;
#6784=CARTESIAN_POINT ( 'NONE',  ( -15.42311360645077301, 11.97619046995196079, -234.9244673706848801 ) ) ;
#6785=CARTESIAN_POINT ( 'NONE',  ( 1.780803752597676537, -13.83832444325970101, -229.2250779460899537 ) ) ;
#6786=CARTESIAN_POINT ( 'NONE',  ( 0.4042326456706432647, 15.50845657815858303, -219.2680337625893401 ) ) ;
#6787=CARTESIAN_POINT ( 'NONE',  ( 26.45187990207246997, -15.96729416691344383, -220.4105496189887674 ) ) ;
#6788=CARTESIAN_POINT ( 'NONE',  ( -15.51091956967506391, -1.782849713491490018, -228.8089183834494520 ) ) ;
#6790=CARTESIAN_POINT ( 'NONE',  ( 13.88312867625433711, 12.44451767566605760, -217.7066242262208391 ) ) ;
#6792=CARTESIAN_POINT ( 'NONE',  ( -11.11821474075380678, 16.53100589793018926, -232.3736596382188395 ) ) ;
#6793=CARTESIAN_POINT ( 'NONE',  ( 24.20411255886326529, 12.66254860825103634, -218.0144359054998802 ) ) ;
#6794=CARTESIAN_POINT ( 'NONE',  ( 13.43730899468209294, 8.427513769504761498, -221.4030804848920297 ) ) ;
#6795=CARTESIAN_POINT ( 'NONE',  ( 12.23475091788960434, 6.342242864926500800, -221.9572581868331156 ) ) ;
#6796=CARTESIAN_POINT ( 'NONE',  ( 4.433847066018189231, -14.70588125837090487, -232.6468564462760469 ) ) ;
#6797=CARTESIAN_POINT ( 'NONE',  ( -1.884624261322229266, 13.00421381464247084, -226.7648460381863345 ) ) ;
#6799=CARTESIAN_POINT ( 'NONE',  ( 28.51464931495100785, 5.422321182929326966, -223.8116416110474347 ) ) ;
#6800=CARTESIAN_POINT ( 'NONE',  ( 3.568716337251232051, -21.91366830329386772, -233.6537821856145172 ) ) ;
#6801=CARTESIAN_POINT ( 'NONE',  ( -11.35482716595652875, 11.86850131893102223, -220.6599844941370350 ) ) ;
#6803=CARTESIAN_POINT ( 'NONE',  ( 2.471164685565028662, 14.01327037412690935, -223.4905256513065410 ) ) ;
#6804=CARTESIAN_POINT ( 'NONE',  ( -25.10035252441274167, -15.33546242866430198, -228.3913311683031964 ) ) ;
#6805=CARTESIAN_POINT ( 'NONE',  ( 12.93042813863272755, 0.4488092930645843914, -225.5263188864764174 ) ) ;
#6807=CARTESIAN_POINT ( 'NONE',  ( 21.14441169763230732, 12.98245189690719315, -217.0976687089155064 ) ) ;
#6809=CARTESIAN_POINT ( 'NONE',  ( 12.04687593227112430, 27.54339840196571743, -224.6466266724203820 ) ) ;
#6810=CARTESIAN_POINT ( 'NONE',  ( 13.37416304104233333, -8.359606308866407431, -226.7674924273047452 ) ) ;
#6811=CARTESIAN_POINT ( 'NONE',  ( 12.74640035234706659, -6.767230903810586895, -221.4971111014800726 ) ) ;
#6813=CARTESIAN_POINT ( 'NONE',  ( 1.773982976645536835, 19.12448993322812285, -233.2315972735944172 ) ) ;
#6814=CARTESIAN_POINT ( 'NONE',  ( -12.42228566111607968, -8.873047627549107474, -232.6540845750675999 ) ) ;
#6815=CARTESIAN_POINT ( 'NONE',  ( -15.46269062504165781, -26.67469327287815517, -225.2085449711190677 ) ) ;
#6816=CARTESIAN_POINT ( 'NONE',  ( 6.053458391837899910, -12.85229775019162268, -220.9645494416007523 ) ) ;
#6817=CARTESIAN_POINT ( 'NONE',  ( -13.40354389326479456, 23.35336998323175450, -219.8517474526506987 ) ) ;
#6818=CARTESIAN_POINT ( 'NONE',  ( 10.89019654021101857, 23.08162452736882031, -220.1893104909416934 ) ) ;
#6819=CARTESIAN_POINT ( 'NONE',  ( -14.07917727715460821, 7.534853284453274291, -218.6337090155677458 ) ) ;
#6820=CARTESIAN_POINT ( 'NONE',  ( -13.33011381921379090, 5.829915729572584304, -219.4453182727427816 ) ) ;
#6821=CARTESIAN_POINT ( 'NONE',  ( -19.48378335617362112, -12.36282430725977655, -218.8185104403611945 ) ) ;
#6823=CARTESIAN_POINT ( 'NONE',  ( -4.691002462566371101, 21.98518063340150164, -232.2516024630330094 ) ) ;
#6824=CARTESIAN_POINT ( 'NONE',  ( 23.44028133050380802, 19.87677100428751231, -223.1503774981096342 ) ) ;
#6825=CARTESIAN_POINT ( 'NONE',  ( 15.79748369401691122, 19.19631269170049137, -215.0096632418193963 ) ) ;
#6826=CARTESIAN_POINT ( 'NONE',  ( 11.63416633096549369, -11.60453582225250990, -230.7583135875248104 ) ) ;
#6830=CARTESIAN_POINT ( 'NONE',  ( -11.26857159993117996, 28.96895336474501192, -225.6039696848669678 ) ) ;
#6831=CARTESIAN_POINT ( 'NONE',  ( -11.10256751292636324, -5.696117445562730808, -228.9287437256430451 ) ) ;
#6833=CARTESIAN_POINT ( 'NONE',  ( 19.19288224840068935, 10.13059690604263174, -232.1906135022504998 ) ) ;
#6834=CARTESIAN_POINT ( 'NONE',  ( -29.30406754532526037, 5.063969254119831120, -221.8212091093853076 ) ) ;
#6835=CARTESIAN_POINT ( 'NONE',  ( 13.49882595795384255, -9.201056071450322449, -219.2439763087855908 ) ) ;
#6836=CARTESIAN_POINT ( 'NONE',  ( -11.46843428684449151, 6.508406145394057596, -225.7212143570321814 ) ) ;
#6838=CARTESIAN_POINT ( 'NONE',  ( -21.89482327431018760, 1.733733432562314158, -233.1353281693111796 ) ) ;
#6839=CARTESIAN_POINT ( 'NONE',  ( -3.515149843921121509, -20.22121776728782550, -231.9652171757311123 ) ) ;
#6843=CARTESIAN_POINT ( 'NONE',  ( 13.30832375548903990, -9.333840824262514602, -222.9696809959601183 ) ) ;
#6844=CARTESIAN_POINT ( 'NONE',  ( -27.09167109716269550, -0.2825935922571593539, -219.8389404328913486 ) ) ;
#6846=CARTESIAN_POINT ( 'NONE',  ( 14.78510113471881304, 14.77128235908076803, -230.8056908117964383 ) ) ;
#6847=CARTESIAN_POINT ( 'NONE',  ( 10.12648780932046755, 24.76571117977573522, -228.8499436907259792 ) ) ;
#6848=CARTESIAN_POINT ( 'NONE',  ( 7.445043070300236820, -12.68569377707410339, -219.2962123921901991 ) ) ;
#6849=CARTESIAN_POINT ( 'NONE',  ( 5.953549895739506326, -12.70069413479034104, -221.3143591192976203 ) ) ;
#6851=APPLICATION_CONTEXT ( 'automotive_design' ) ;
#6852=CARTESIAN_POINT ( 'NONE',  ( -7.284474494690100776, 13.60812129561547046, -227.7414351104868331 ) ) ;
#6853=CARTESIAN_POINT ( 'NONE',  ( -16.54465188417290022, 6.134005835925411709, -228.8256222654843270 ) ) ;
#6854=CARTESIAN_POINT ( 'NONE',  ( 27.94758519801750296, 7.894658480667867018, -227.3974864124137127 ) ) ;
#6855=CARTESIAN_POINT ( 'NONE',  ( -3.424870747449708652, -17.07003249573819659, -220.0803597572327135 ) ) ;
#6858=CARTESIAN_POINT ( 'NONE',  ( 21.18605525173251891, 3.426801613781890854, -232.1183243183448894 ) ) ;
#6859=CARTESIAN_POINT ( 'NONE',  ( 12.31709745011784740, -23.08055702692190891, -220.7960250479738136 ) ) ;
#6860=CARTESIAN_POINT ( 'NONE',  ( 4.883314309504700468, 19.06839645569368358, -217.0171359871271193 ) ) ;
#6861=CARTESIAN_POINT ( 'NONE',  ( -15.48255455842386219, 10.01793346089237069, -233.1197357361336913 ) ) ;
#6863=CARTESIAN_POINT ( 'NONE',  ( 30.65249971456167799, 3.724008896938769464, -225.4815109119605552 ) ) ;
#6864=CARTESIAN_POINT ( 'NONE',  ( -10.84997096467605182, 25.01800101807719301, -232.4518260228253155 ) ) ;
#6866=CARTESIAN_POINT ( 'NONE',  ( -2.270280637033633475, -14.48864307936496765, -230.4581659391201072 ) ) ;
#6869=CARTESIAN_POINT ( 'NONE',  ( -28.42127686227592420, -0.6461176296494712812, -221.6028628238154567 ) ) ;
#6870=CARTESIAN_POINT ( 'NONE',  ( -26.09112266552012471, 5.807188091516064077, -215.7774933166620883 ) ) ;
#6871=CARTESIAN_POINT ( 'NONE',  ( -14.39178795515995724, -23.41959061255243313, -230.2514514786898019 ) ) ;
#6872=( BOUNDED_SURFACE ( )  B_SPLINE_SURFACE ( 3, 3, ( 
 ( #12046, #13513, #17114, #20575, #17002, #6643, #8565, #10025, #20351, #16778, #1462, #13628, #4946, #15429, #2036, #16887, #18903, #11822, #5163, #18688, #9797, #1581, #16663, #8118, #1244, #9915, #20464, #8456, #14983, #15324, #22170, #21823, #1354, #13283, #4713, #20239, #11592, #18466, #18797, #3028, #3366, #8226, #4833, #7099, #15649, #10799, #10577, #114, #341, #8668, #17664, #7320, #6982, #15531, #13855, #12599, #17448, #20695, #446, #21028, #3478, #15979, #10356, #3922, #2017, #8897, #2235, #15763, #14075, #9115, #556, #3587, #17219, #1792, #5616, #9004, #5272, #15868, #20802, #7432, #10694, #7209, #21133, #14300, #5720, #14190, #12153, #12494, #19010, #17558, #10464, #20913, #17327, #12263, #19341, #1904, #2127, #8787, #3811, #229, #5500, #12380, #13963, #19231, #5380, #19116, #3693, #14519, #19557, #6470, #6359, #15150, #4664, #9858, #15040, #19666, #11652, #21770, #17781, #2455, #21992, #1187, #20181, #8281, #13231, #2562, #18523, #12823, #8066, #4145, #11131, #16723, #14931, #3089, #4775, #4253, #6585, #17999, #9972, #20077, #16831, #11537, #1409, #2347, #19444, #11024, #8174, #18410, #4031, #9744, #2972, #9232, #17892, #10907, #16092, #9337, #663, #7539, #1300, #14408, #16606, #21240, #5832, #769, #16197, #21881, #13339, #12710, #7648, #21352, #5946, #15591, #18957, #3197, #3533, #8514, #17388, #20636, #3424, #8842, #3639, #15708, #10413, #285, #17274, #11771, #5221, #15267, #11988, #5329, #22224, #1848, #10520, #12102, #8726, #13795, #1964, #5107, #8619, #11876, #20517, #20411, #5000, #53, #15377, #13575, #172, #6926, #13456, #7041, #13913, #20748, #13681, #12211, #15479, #18635, #18740, #20296, #17167, #19064, #4891, #10080, #18849, #16945, #6815, #1745, #3307, #10304, #1521, #8399, #22117, #6704, #10190, #17060, #1637, #21290, #2289, #5886, #10849, #11076, #5440, #12762, #7264, #17835, #9175, #4197, #5667, #610, #12322, #14134, #19612, #17943, #12438, #2507, #3753, #7485, #14457, #21080, #9385, #16247, #10746, #19289, #14354, #12545, #7379, #12653, #393, #7154, #17612, #3866, #14020, #14247, #10638, #3975, #19176, #20856, #10964, #17505, #2072, #8952, #15816, #19392, #20972, #4087, #2400, #5560, #2178, #9059, #7588, #17723, #16038, #15925, #21186, #5772, #503, #19499, #9282, #16142, #714, #5997, #6331, #21513, #936, #12976, #3055, #7814, #16577, #4526, #11510, #18273, #16690, #21407, #6217, #6440, #21739, #14570, #16358, #2834, #13204, #21851, #4744, #12870, #20151, #9716, #1158, #1270, #21625, #19824, #13092, #2727, #14900, #4409, #9945, #11291, #7920, #20049, #18162, #8034, #14784, #14679 ),
 ( #16470, #11404, #6105, #19938, #4636, #18378, #13309, #8146, #1047, #822, #2942, #15011, #9829, #11623, #18495, #7701, #19719, #4299, #9608, #11181, #18048, #2617, #9498, #10278, #21962, #16918, #15562, #8696, #22085, #20720, #13427, #17144, #1818, #8487, #142, #3614, #20382, #6675, #1720, #15351, #17034, #28, #10055, #13882, #4976, #13547, #7010, #1609, #20268, #13656, #6555, #5301, #20607, #4864, #11741, #18609, #16805, #22199, #3171, #13768, #12075, #1380, #12183, #8256, #17247, #6787, #20491, #19037, #5082, #11963, #15123, #1492, #8370, #15240, #11851, #18932, #6898, #18824, #18716, #3396, #5193, #8595, #3280, #10165, #15456, #3507, #10386, #2375, #5642, #9258, #14217, #14433, #8815, #16117, #10607, #21159, #12518, #7565, #9033, #3949, #15678, #17476, #690, #21266, #15791, #5859, #7126, #10825, #17810, #2153, #12740, #19585, #14106, #370, #17695, #15897, #10721, #16008, #3725, #10492, #20943, #7237, #17358, #17587, #13993, #7351, #258, #1935, #14327, #20829, #5410, #12293, #19146, #477, #2047, #7459, #5747, #8925, #5530, #12409, #10937, #21052, #19368, #19260, #2264, #9147, #12627, #584, #19473, #4062, #3840, #4613, #21490, #9364, #9692, #2592, #4279, #16335, #6417, #11159, #19914, #7900, #14875, #21600, #20026, #2483, #9587, #9802, #2813, #17918, #19693, #6191, #16553, #2917, #8122, #16223, #1248, #13070, #4503, #11488, #2704, #911, #16450, #6081, #18251, #7791, #13287, #14657, #11269, #1131, #12956, #11382, #18138, #18025, #8007, #21716, #21828, #4384, #19800, #6308, #14548, #13183, #21384, #18355, #16667, #1023, #4174, #14760, #14987, #11052, #798, #7678, #5974, #9475, #12851, #5058, #15535, #20356, #15212, #6762, #8231, #6871, #15101, #5168, #20467, #10139, #3032, #1796, #118, #18584, #18907, #8342, #3483, #4837, #11596, #18692, #3370, #1585, #6987, #18470, #20129, #10360, #8672, #13743, #13632, #11935, #4717, #9919, #16783, #18800, #1358, #22058, #3255, #17006, #3, #20579, #10252, #12050, #21937, #17223, #11713, #6528, #17118, #6647, #13397, #20243, #1466, #1697, #13517, #4950, #11826, #3146, #8569, #10029, #8460, #15328, #16892, #22174, #15433, #17786, #9119, #10802, #19235, #16096, #19120, #13967, #3697, #10911, #19448, #5724, #5620, #20699, #3815, #2131, #17668, #21032, #5504, #9008, #2351, #14304, #8901, #19014, #19345, #12267, #20806, #10582, #667, #5383, #7325, #17562, #2238, #15872, #7436, #12157, #10698, #4035, #12498, #5276, #7103, #450, #3927, #12604, #9236, #3591, #13859, #14195, #15983, #21137, #12385, #17452, #560, #15767, #10468, #17331, #1908, #8792, #2021, #15653, #233, #345 ),
 ( #7213, #14079, #20917, #16641, #11135, #19670, #14737, #21466, #7764, #13042, #772, #4587, #18003, #4257, #14847, #14634, #4149, #4359, #12714, #21690, #11357, #11029, #19562, #17896, #7542, #6058, #2459, #4477, #2786, #14412, #20002, #21244, #7982, #12932, #19778, #6282, #18332, #2893, #11242, #9342, #7652, #5836, #16201, #9669, #19888, #14523, #18226, #2567, #11463, #21577, #18113, #9776, #21358, #5950, #16528, #12827, #1107, #9451, #6165, #16311, #2681, #13156, #887, #9563, #16425, #1000, #7875, #1558, #13716, #15186, #18669, #21914, #8316, #8206, #15078, #10114, #18559, #1334, #10225, #16979, #18883, #8433, #13607, #18776, #1445, #15410, #3230, #21804, #6503, #3458, #4926, #1671, #12024, #15300, #6621, #22255, #16868, #11802, #13374, #22030, #20444, #22150, #6848, #8546, #13490, #10337, #20330, #20556, #6739, #5143, #5033, #11910, #8097, #3342, #17093, #1222, #14964, #6392, #13263, #20107, #4695, #3125, #11570, #18444, #20216, #4811, #11687, #3007, #10005, #9890, #16756, #5597, #12362, #10779, #15511, #322, #535, #15851, #8650, #10447, #19212, #427, #15962, #21116, #6964, #14282, #3793, #17541, #17647, #15743, #13946, #7190, #19097, #8988, #7077, #4010, #20781, #1998, #7302, #5362, #10677, #8879, #1883, #2108, #14172, #12581, #17428, #12246, #21007, #5255, #3904, #12135, #2213, #12478, #14056, #93, #5703, #19424, #15627, #7412, #3674, #17201, #8766, #13835, #20892, #19324, #5479, #1776, #20671, #18991, #3570, #17307, #9095, #207, #10558, #13130, #17762, #19975, #2655, #6255, #21330, #16286, #860, #13015, #11329, #9536, #4447, #10886, #18198, #2435, #1081, #7849, #12801, #16503, #2326, #14495, #16396, #5924, #19647, #4232, #5809, #4334, #2761, #7738, #11112, #12690, #14608, #17980, #14820, #6141, #14715, #21443, #9211, #16179, #11005, #750, #7955, #21665, #9642, #16074, #7626, #644, #6033, #7521, #14389, #11218, #12907, #21222, #2543, #19754, #17873, #9422, #21550, #18086, #19537, #4124, #975, #9319, #19861, #18746, #21998, #3313, #8287, #8520, #2866, #10198, #4670, #15273, #6593, #1643, #3095, #20302, #9750, #11543, #17066, #15383, #9864, #22230, #1195, #4897, #11883, #18529, #6821, #13687, #8181, #16729, #11777, #9978, #4783, #10086, #20083, #4562, #15046, #1306, #11438, #11658, #8072, #1415, #16613, #18307, #8406, #14937, #21777, #6365, #13237, #16839, #18417, #1527, #22123, #2980, #21887, #6476, #5006, #15156, #13462, #13345, #20187, #18641, #3204, #16951, #6710, #13581, #20417, #694, #4066, #10310, #10941, #15600, #2487, #5751, #10828, #16227, #11055, #803, #17814, #7682, #2379, #18855, #12631, #59 ),
 ( #589, #21164, #21271, #19372, #17281, #17699, #480, #19477, #10420, #20524, #1855, #5646, #9263, #8733, #7462, #12523, #5228, #3541, #20643, #7355, #17923, #4179, #12743, #16120, #5113, #3953, #9150, #7570, #14436, #2266, #16012, #9367, #5862, #14222, #3430, #19589, #18964, #12109, #21058, #11995, #14330, #17174, #1751, #8625, #15486, #6933, #13804, #19918, #20132, #13186, #5978, #7796, #9696, #20030, #13291, #18473, #4283, #11602, #16557, #14878, #14992, #13074, #11273, #4505, #16454, #6312, #4388, #1361, #18142, #21605, #4617, #2708, #1136, #6197, #21494, #8014, #21719, #9922, #14764, #9591, #11492, #2598, #1251, #9479, #21831, #18359, #11386, #19696, #3036, #16786, #12960, #4721, #1026, #14551, #6084, #12854, #18254, #2921, #2817, #21387, #11162, #18029, #16339, #915, #8126, #9808, #16671, #14660, #19804, #7903, #6420, #8673, #13519, #1588, #8463, #5, #20583, #3372, #13746, #8235, #5169, #8346, #10361, #1698, #11828, #3484, #15104, #20360, #8570, #18695, #3258, #10142, #10033, #18802, #18908, #15330, #17011, #16895, #6765, #22176, #1797, #6874, #15435, #13634, #21941, #5061, #12051, #20246, #20469, #17224, #15537, #4841, #15217, #11938, #6533, #13402, #11717, #1470, #18587, #3149, #22061, #6651, #4952, #10253, #17119, #18873, #3332, #10328, #81, #7066, #3448, #1767, #6952, #11900, #3559, #13707, #9996, #16968, #13935, #15400, #12125, #196, #5131, #17084, #10437, #5024, #22247, #18661, #10215, #8641, #6839, #17297, #18980, #18763, #20770, #1661, #1872, #20544, #8755, #12015, #15616, #16858, #11678, #11794, #13824, #17190, #18549, #8536, #15502, #1434, #3221, #3116, #8307, #1547, #15174, #22020, #20661, #6612, #5243, #13481, #20320, #15291, #8424, #4918, #10104, #22140, #6730, #13598, #20435, #8976, #17529, #12678, #12467, #1987, #2202, #10547, #19526, #9199, #8867, #17417, #15732, #14482, #19313, #309, #2314, #634, #5352, #17861, #12235, #5797, #3891, #10769, #4113, #16168, #738, #17635, #7180, #5467, #19086, #3662, #7510, #10874, #14045, #17750, #416, #9307, #12569, #9083, #7614, #2424, #20881, #16064, #12350, #19414, #19202, #15840, #15950, #525, #14377, #10992, #3998, #21211, #3782, #10664, #2096, #7290, #14161, #20997, #5587, #7403, #14273, #21105, #5690, #16384, #963, #16273, #14808, #13226, #4435, #14703, #848, #18187, #21537, #2967, #16601, #18296, #11317, #1295, #4323, #21432, #11206, #18405, #4659, #20072, #13118, #5913, #2750, #9631, #2855, #6244, #13002, #16493, #9853, #21765, #7837, #4220, #4551, #19743, #6022, #18072, #8169, #12895, #21651, #1070, #9739, #7944, #14925, #19636, #19964, #11532 ),
 ( #11427, #2644, #6128, #9524, #19848, #1182, #8060, #6354, #16718, #21316, #12790, #11100, #17968, #2532, #9409, #7726, #14597, #13334, #20291, #17268, #18735, #15475, #3527, #8509, #20406, #13790, #8394, #3301, #21987, #6698, #11983, #10185, #20628, #48, #15262, #1840, #22111, #6921, #17054, #5214, #1631, #18951, #20176, #12096, #15145, #3419, #15372, #10406, #13570, #22219, #4770, #6810, #8614, #11646, #4995, #15035, #13676, #6465, #8276, #20513, #5103, #21876, #18517, #3084, #9967, #18844, #10299, #16826, #11871, #11766, #17163, #1404, #18630, #1740, #6580, #3192, #13450, #4886, #10075, #16940, #1516, #15700, #17604, #15918, #4081, #8945, #3745, #2172, #19058, #17717, #3634, #16029, #9050, #20963, #13906, #12647, #10957, #7147, #7477, #19169, #14347, #277, #163, #7255, #14238, #12430, #17830, #7033, #8718, #21180, #19494, #2282, #496, #7370, #15585, #20741, #5322, #21073, #12203, #10629, #14127, #5551, #10842, #9166, #5661, #603, #10514, #5765, #14012, #17380, #12538, #17498, #1955, #8833, #12315, #19385, #2065, #15810, #387, #20849, #3968, #5431, #19281, #3858, #10739, #21508, #2612, #6326, #19933, #21620, #7809, #4631, #7696, #2501, #14566, #21734, #8029, #16571, #16466, #9276, #14674, #12972, #6213, #9604, #16354, #19819, #13198, #2830, #19712, #7583, #7915, #818, #9380, #21401, #11505, #16240, #18156, #6099, #13088, #4405, #1042, #1153, #20043, #14450, #2393, #11286, #2723, #9711, #931, #5992, #14779, #16136, #12866, #4520, #11399, #4295, #9493, #18267, #11176, #14895, #708, #18043, #21285, #5880, #12757, #19606, #4192, #11069, #17938, #5076, #13304, #3390, #18710, #8363, #1265, #22, #20600, #16800, #17138, #6549, #1713, #3050, #9824, #16911, #1603, #22079, #5187, #16685, #18373, #8589, #6891, #11955, #11845, #3273, #2935, #8141, #15006, #10158, #13761, #13422, #1486, #15234, #20485, #18818, #17028, #10272, #21844, #15451, #9940, #6435, #15344, #20262, #20146, #4739, #21957, #8481, #4859, #11736, #18604, #11617, #22193, #18490, #6668, #3165, #1374, #13541, #10049, #8250, #13650, #6780, #20376, #15118, #4969, #12177, #17352, #9445, #17997, #4251, #3835, #18926, #17471, #364, #9028, #19255, #3720, #7232, #881, #12821, #7120, #17241, #17582, #10485, #19031, #1929, #14629, #3608, #5525, #15786, #470, #14099, #5943, #10378, #2042, #2560, #10716, #3501, #5296, #19664, #12404, #2148, #21461, #1812, #12069, #15891, #7757, #252, #8920, #20938, #14517, #11129, #7646, #16306, #8690, #15556, #8809, #136, #21349, #13986, #7004, #13877, #15672, #20715, #20824, #5403, #12287, #19139, #10602, #20211, #11458, #21685 ),
 ( #18553, #12927, #6497, #13150, #19996, #4806, #16863, #1438, #4582, #11237, #6159, #19773, #4352, #8201, #11564, #18107, #18439, #1101, #10000, #13258, #18327, #8311, #3120, #15179, #3002, #6053, #9885, #2675, #20101, #7870, #2887, #11682, #14842, #16749, #9557, #4690, #1329, #6385, #16419, #9770, #1217, #4470, #16636, #13036, #19883, #14958, #15071, #8092, #21909, #13368, #995, #14733, #21572, #11351, #6276, #18221, #21799, #2780, #9664, #16523, #7976, #201, #10552, #15506, #5137, #20774, #15404, #10332, #6734, #13711, #18984, #17194, #5356, #7070, #22250, #8872, #6843, #13939, #1771, #12239, #3452, #3666, #20324, #19090, #22143, #10441, #20549, #5247, #8645, #1990, #13485, #22025, #17421, #6616, #15620, #86, #6957, #4922, #11798, #18665, #13829, #3225, #10219, #12019, #18877, #1876, #10108, #20665, #16973, #1552, #8428, #13602, #15295, #3563, #1665, #20439, #5028, #3337, #12129, #17088, #8540, #17301, #11904, #8760, #18769, #21109, #9086, #17534, #12574, #15955, #19640, #10996, #12682, #5694, #17972, #21001, #15844, #5591, #12794, #21322, #7618, #7514, #313, #19418, #4002, #19531, #638, #7407, #10877, #4225, #16172, #10773, #20885, #21215, #14166, #420, #12471, #2536, #7294, #9204, #17755, #4117, #2318, #9311, #14049, #16067, #5917, #14381, #7184, #8980, #5801, #17866, #14486, #11104, #5471, #15736, #2428, #742, #12355, #14277, #19317, #19205, #3786, #3896, #10668, #2100, #17639, #529, #2206, #21542, #11431, #1074, #16388, #18300, #16605, #4774, #9635, #4439, #2859, #19747, #18409, #4327, #16722, #9743, #21656, #14601, #13338, #11651, #7841, #8173, #19852, #15039, #967, #853, #4555, #2971, #7730, #14812, #21880, #8065, #21436, #2648, #1186, #14930, #6469, #20180, #6026, #18522, #21769, #6358, #9857, #7948, #6132, #6248, #9413, #13006, #13230, #20076, #11322, #16497, #4663, #18191, #11536, #13122, #14707, #1299, #16277, #12900, #19968, #2754, #11210, #18076, #9529, #20295, #10412, #3423, #15376, #8280, #7040, #5328, #1520, #1847, #13574, #8725, #10079, #16830, #1636, #8618, #6814, #12210, #1408, #3088, #15590, #13912, #18956, #18848, #10303, #9971, #15149, #21991, #17166, #20747, #20410, #8513, #22223, #5220, #3532, #1744, #17273, #6584, #171, #16944, #13455, #52, #4999, #4890, #11770, #6703, #15478, #11875, #18739, #3306, #18634, #6925, #3196, #13680, #10189, #8398, #20516, #17059, #15266, #20635, #13794, #5106, #22116, #11987, #12101, #2071, #16141, #2398, #10963, #10848, #3638, #2177, #7378, #16037, #3974, #10745, #14246, #7587, #19498, #14133, #1963, #2288, #17504, #19175, #8951, #21289, #3752, #12544 ),
 ( #8841, #9174, #20971, #713, #17722, #9058, #14456, #9281, #5885, #609, #19063, #7484, #17387, #14353, #20855, #17611, #17834, #5559, #21185, #10519, #5771, #12652, #19391, #15707, #15924, #21079, #15815, #3865, #10637, #392, #5666, #4086, #502, #284, #7153, #14019, #5439, #12321, #7263, #19288, #12437, #14782, #11074, #18047, #15010, #16469, #13203, #1269, #6216, #18161, #11509, #6103, #1046, #19717, #4408, #9715, #7919, #18377, #20048, #12975, #21850, #19823, #4635, #21624, #2941, #13091, #16689, #17942, #9828, #12869, #1157, #19937, #8145, #11290, #4525, #2506, #4298, #12761, #19611, #2616, #4196, #9384, #11403, #16246, #2726, #821, #7700, #16357, #9497, #18272, #9607, #2833, #16576, #5996, #14569, #935, #7813, #21406, #8033, #11180, #14899, #14678, #21512, #21738, #6330, #11622, #9944, #15560, #20380, #18494, #3394, #1718, #6439, #18930, #13308, #6896, #13545, #4974, #20605, #17245, #3054, #6554, #5191, #12073, #11740, #10384, #16804, #22197, #13766, #11849, #3505, #20150, #10053, #18608, #13654, #18714, #6673, #11961, #21961, #1816, #16916, #3170, #8694, #3278, #1379, #10163, #8255, #4743, #10276, #15122, #13426, #20267, #4863, #17032, #1490, #17142, #8593, #8368, #15238, #22083, #1607, #8485, #15349, #6785, #20489, #5080, #18822, #15454, #26, #7008, #20718, #2262, #5640, #12181, #12516, #17474, #4060, #7349, #12407, #17808, #12625, #2373, #19366, #9256, #3947, #5299, #14215, #1933, #20941, #14325, #8923, #10823, #19471, #21050, #17693, #475, #10935, #14104, #17585, #20827, #7235, #7124, #13991, #9031, #9145, #5528, #16006, #582, #140, #7457, #21157, #5745, #368, #13880, #2151, #19035, #5408, #3612, #3838, #10490, #17356, #15895, #19258, #8813, #15789, #10719, #12291, #15676, #256, #19143, #3723, #10605, #2045, #2915, #9473, #8005, #11267, #14873, #19798, #20024, #14431, #21714, #16221, #4501, #18136, #13181, #14655, #9585, #14546, #796, #5972, #18353, #7676, #16448, #4382, #11380, #2702, #9690, #21264, #21488, #6306, #14758, #7563, #9362, #1021, #21598, #4611, #11486, #5857, #16115, #7898, #6189, #16551, #6079, #12849, #12954, #688, #19691, #13068, #19912, #4277, #909, #18249, #11157, #2811, #7789, #21382, #1129, #12738, #19583, #16333, #18023, #4172, #11050, #17916, #2480, #2590, #10137, #22056, #14985, #13740, #12048, #8229, #8567, #20241, #15431, #16781, #1246, #8340, #15326, #13515, #18905, #8120, #9799, #1, #20577, #3368, #3253, #17004, #16665, #21826, #6415, #1583, #5166, #4835, #15210, #6645, #11933, #10250, #8458, #17116, #13285, #1695, #1356, #6869, #6760, #11711, #20127, #4715, #13395 ) ),
 .UNSPECIFIED., .T., .F., .F. ) 
 B_SPLINE_SURFACE_WITH_KNOTS ( ( 4, 3, 4 ),
 ( 4, 2, 2, 2, 2, 2, 2, 2, 2, 2, 2, 2, 2, 2, 2, 2, 2, 2, 2, 2, 2, 2, 2, 2, 2, 2, 2, 2, 2, 2, 2, 2, 2, 2, 2, 2, 2, 2, 2, 2, 2, 2, 2, 2, 2, 2, 2, 2, 2, 2, 2, 2, 2, 2, 2, 2, 2, 2, 2, 2, 2, 2, 2, 2, 2, 2, 2, 2, 2, 2, 2, 2, 2, 2, 2, 2, 2, 2, 2, 2, 2, 2, 2, 2, 2, 2, 2, 2, 2, 2, 2, 2, 2, 2, 2, 2, 2, 2, 2, 2, 2, 2, 2, 2, 2, 2, 2, 2, 2, 2, 2, 2, 2, 2, 2, 2, 2, 2, 2, 2, 2, 2, 2, 2, 2, 2, 2, 2, 2, 2, 2, 2, 2, 2, 2, 2, 2, 2, 2, 2, 2, 2, 2, 2, 2, 2, 2, 2, 2, 2, 2, 2, 2, 2, 2, 2, 2, 2, 2, 2, 2, 2, 2, 2, 2, 2, 2, 2, 2, 4 ),
 ( 0.000000000000000000, 0.5000000000000000000, 1.000000000000000000 ),
 ( 0.4999446919652688059, 0.5028747035357847839, 0.5058047151063008728, 0.5087347266768169618, 0.5116647382473329397, 0.5145947498178489177, 0.5175247613883648956, 0.5204547729588808735, 0.5233847845293969625, 0.5268031313616656774, 0.5285123047777999794, 0.5302214781939342814, 0.5336398250262029963, 0.5353489984423374093, 0.5370581718584717112, 0.5404765186907403152, 0.5438948655230090301, 0.5473132123552777450, 0.5507315591875463490, 0.5541499060198149529, 0.5575682528520836678, 0.5609865996843523828, 0.5644049465166209867, 0.5661141199327552886, 0.5678232933488895906, 0.5712416401811581945, 0.5729508135972924965, 0.5746599870134267984, 0.5780783338456955134, 0.5814966806779642283, 0.5849150275102328322, 0.5883333743425015472, 0.5917517211747702621, 0.5951700680070388660, 0.5985884148393075810, 0.6020067616715762959, 0.6037159350877105979, 0.6054251085038448998, 0.6088434553361135038, 0.6122618021683822187, 0.6139709755845166317, 0.6156801490006509336, 0.6190984958329195376, 0.6225168426651882525, 0.6259351894974569674, 0.6293535363297255714, 0.6327718831619942863, 0.6361902299942630012, 0.6396085768265316052, 0.6430269236588003201, 0.6447360970749347331, 0.6464452704910690350, 0.6498636173233376390, 0.6532819641556063539, 0.6549911375717407669, 0.6567003109878750688, 0.6601186578201436728, 0.6635370046524122767, 0.6669553514846809916, 0.6703736983169497066, 0.6737920451492183105, 0.6772103919814870254, 0.6806287388137557404, 0.6840470856460243443, 0.6857562590621586462, 0.6866108457702257972, 0.6874654324782930592, 0.6908837793105617742, 0.6943021261428303781, 0.6960112995589646800, 0.6977204729750989820, 0.7011388198073676969, 0.7045571666396364119, 0.7079755134719050158, 0.7113938603041736197, 0.7148122071364423347, 0.7182305539687110496, 0.7216489008009796535, 0.7250672476332483685, 0.7267764210493827814, 0.7284855944655170834, 0.7319039412977856873, 0.7353222881300544023, 0.7387406349623231172, 0.7421589817945917211, 0.7455773286268603250, 0.7489956754591290400, 0.7524140222913977549, 0.7558323691236663588, 0.7592507159559350738, 0.7626690627882037887, 0.7660874096204723926, 0.7695057564527411076, 0.7729241032850098225, 0.7763424501172784264, 0.7797607969495471414, 0.7831791437818158563, 0.7865974906140844602, 0.7900158374463531752, 0.7934341842786218901, 0.7968525311108904940, 0.8002708779431590980, 0.8036892247754278129, 0.8053983981915622259, 0.8071075716076965278, 0.8105259184399651318, 0.8122350918560994337, 0.8139442652722337357, 0.8173626121045024506, 0.8207809589367711656, 0.8241993057690397695, 0.8276176526013083734, 0.8310359994335770883, 0.8344543462658458033, 0.8378726930981144072, 0.8412910399303831221, 0.8430002133465175351, 0.8447093867626518371, 0.8481277335949204410, 0.8515460804271891559, 0.8549644272594578709, 0.8583827740917264748, 0.8618011209239951897, 0.8652194677562639047, 0.8686378145885325086, 0.8720561614208012235, 0.8754745082530699385, 0.8788928550853385424, 0.8823112019176071463, 0.8857295487498758613, 0.8874387221660102743, 0.8891478955821445762, 0.8925662424144131801, 0.8942754158305474821, 0.8959845892466818951, 0.8994029360789506100, 0.9028212829112192139, 0.9062396297434879289, 0.9096579765757566438, 0.9130763234080252477, 0.9164946702402939627, 0.9199130170725626776, 0.9233313639048312815, 0.9250405373209655835, 0.9267497107370999965, 0.9301680575693687114, 0.9335864044016373153, 0.9352955778177716173, 0.9370047512339059192, 0.9404230980661746342, 0.9438414448984433491, 0.9472597917307119531, 0.9506781385629806680, 0.9540964853952493829, 0.9575148322275179869, 0.9609331790597867018, 0.9643515258920554167, 0.9660606993081897187, 0.9677698727243240207, 0.9711882195565927356, 0.9728973929727271486, 0.9746065663888614505, 0.9780249132211300545, 0.9814432600533987694, 0.9848616068856674843, 0.9882799537179360883, 0.9912099652884520662, 0.9941399768589680441, 0.9970699884294840221, 1.000000000000000000 ),
 .UNSPECIFIED. ) 
 GEOMETRIC_REPRESENTATION_ITEM ( )  RATIONAL_B_SPLINE_SURFACE ( (
 ( 1.000000000000000000, 1.000000000000000000, 1.000000000000000000, 1.000000000000000000, 1.000000000000000000, 1.000000000000000000, 1.000000000000000000, 1.000000000000000000, 1.000000000000000000, 1.000000000000000000, 1.000000000000000000, 1.000000000000000000, 1.000000000000000000, 1.000000000000000000, 1.000000000000000000, 1.000000000000000000, 1.000000000000000000, 1.000000000000000000, 1.000000000000000000, 1.000000000000000000, 1.000000000000000000, 1.000000000000000000, 1.000000000000000000, 1.000000000000000000, 1.000000000000000000, 1.000000000000000000, 1.000000000000000000, 1.000000000000000000, 1.000000000000000000, 1.000000000000000000, 1.000000000000000000, 1.000000000000000000, 1.000000000000000000, 1.000000000000000000, 1.000000000000000000, 1.000000000000000000, 1.000000000000000000, 1.000000000000000000, 1.000000000000000000, 1.000000000000000000, 1.000000000000000000, 1.000000000000000000, 1.000000000000000000, 1.000000000000000000, 1.000000000000000000, 1.000000000000000000, 1.000000000000000000, 1.000000000000000000, 1.000000000000000000, 1.000000000000000000, 1.000000000000000000, 1.000000000000000000, 1.000000000000000000, 1.000000000000000000, 1.000000000000000000, 1.000000000000000000, 1.000000000000000000, 1.000000000000000000, 1.000000000000000000, 1.000000000000000000, 1.000000000000000000, 1.000000000000000000, 1.000000000000000000, 1.000000000000000000, 1.000000000000000000, 1.000000000000000000, 1.000000000000000000, 1.000000000000000000, 1.000000000000000000, 1.000000000000000000, 1.000000000000000000, 1.000000000000000000, 1.000000000000000000, 1.000000000000000000, 1.000000000000000000, 1.000000000000000000, 1.000000000000000000, 1.000000000000000000, 1.000000000000000000, 1.000000000000000000, 1.000000000000000000, 1.000000000000000000, 1.000000000000000000, 1.000000000000000000, 1.000000000000000000, 1.000000000000000000, 1.000000000000000000, 1.000000000000000000, 1.000000000000000000, 1.000000000000000000, 1.000000000000000000, 1.000000000000000000, 1.000000000000000000, 1.000000000000000000, 1.000000000000000000, 1.000000000000000000, 1.000000000000000000, 1.000000000000000000, 1.000000000000000000, 1.000000000000000000, 1.000000000000000000, 1.000000000000000000, 1.000000000000000000, 1.000000000000000000, 1.000000000000000000, 1.000000000000000000, 1.000000000000000000, 1.000000000000000000, 1.000000000000000000, 1.000000000000000000, 1.000000000000000000, 1.000000000000000000, 1.000000000000000000, 1.000000000000000000, 1.000000000000000000, 1.000000000000000000, 1.000000000000000000, 1.000000000000000000, 1.000000000000000000, 1.000000000000000000, 1.000000000000000000, 1.000000000000000000, 1.000000000000000000, 1.000000000000000000, 1.000000000000000000, 1.000000000000000000, 1.000000000000000000, 1.000000000000000000, 1.000000000000000000, 1.000000000000000000, 1.000000000000000000, 1.000000000000000000, 1.000000000000000000, 1.000000000000000000, 1.000000000000000000, 1.000000000000000000, 1.000000000000000000, 1.000000000000000000, 1.000000000000000000, 1.000000000000000000, 1.000000000000000000, 1.000000000000000000, 1.000000000000000000, 1.000000000000000000, 1.000000000000000000, 1.000000000000000000, 1.000000000000000000, 1.000000000000000000, 1.000000000000000000, 1.000000000000000000, 1.000000000000000000, 1.000000000000000000, 1.000000000000000000, 1.000000000000000000, 1.000000000000000000, 1.000000000000000000, 1.000000000000000000, 1.000000000000000000, 1.000000000000000000, 1.000000000000000000, 1.000000000000000000, 1.000000000000000000, 1.000000000000000000, 1.000000000000000000, 1.000000000000000000, 1.000000000000000000, 1.000000000000000000, 1.000000000000000000, 1.000000000000000000, 1.000000000000000000, 1.000000000000000000, 1.000000000000000000, 1.000000000000000000, 1.000000000000000000, 1.000000000000000000, 1.000000000000000000, 1.000000000000000000, 1.000000000000000000, 1.000000000000000000, 1.000000000000000000, 1.000000000000000000, 1.000000000000000000, 1.000000000000000000, 1.000000000000000000, 1.000000000000000000, 1.000000000000000000, 1.000000000000000000, 1.000000000000000000, 1.000000000000000000, 1.000000000000000000, 1.000000000000000000, 1.000000000000000000, 1.000000000000000000, 1.000000000000000000, 1.000000000000000000, 1.000000000000000000, 1.000000000000000000, 1.000000000000000000, 1.000000000000000000, 1.000000000000000000, 1.000000000000000000, 1.000000000000000000, 1.000000000000000000, 1.000000000000000000, 1.000000000000000000, 1.000000000000000000, 1.000000000000000000, 1.000000000000000000, 1.000000000000000000, 1.000000000000000000, 1.000000000000000000, 1.000000000000000000, 1.000000000000000000, 1.000000000000000000, 1.000000000000000000, 1.000000000000000000, 1.000000000000000000, 1.000000000000000000, 1.000000000000000000, 1.000000000000000000, 1.000000000000000000, 1.000000000000000000, 1.000000000000000000, 1.000000000000000000, 1.000000000000000000, 1.000000000000000000, 1.000000000000000000, 1.000000000000000000, 1.000000000000000000, 1.000000000000000000, 1.000000000000000000, 1.000000000000000000, 1.000000000000000000, 1.000000000000000000, 1.000000000000000000, 1.000000000000000000, 1.000000000000000000, 1.000000000000000000, 1.000000000000000000, 1.000000000000000000, 1.000000000000000000, 1.000000000000000000, 1.000000000000000000, 1.000000000000000000, 1.000000000000000000, 1.000000000000000000, 1.000000000000000000, 1.000000000000000000, 1.000000000000000000, 1.000000000000000000, 1.000000000000000000, 1.000000000000000000, 1.000000000000000000, 1.000000000000000000, 1.000000000000000000, 1.000000000000000000, 1.000000000000000000, 1.000000000000000000, 1.000000000000000000, 1.000000000000000000, 1.000000000000000000, 1.000000000000000000, 1.000000000000000000, 1.000000000000000000, 1.000000000000000000, 1.000000000000000000, 1.000000000000000000, 1.000000000000000000, 1.000000000000000000, 1.000000000000000000, 1.000000000000000000, 1.000000000000000000, 1.000000000000000000, 1.000000000000000000, 1.000000000000000000, 1.000000000000000000, 1.000000000000000000, 1.000000000000000000, 1.000000000000000000, 1.000000000000000000, 1.000000000000000000, 1.000000000000000000, 1.000000000000000000, 1.000000000000000000, 1.000000000000000000, 1.000000000000000000, 1.000000000000000000, 1.000000000000000000, 1.000000000000000000, 1.000000000000000000, 1.000000000000000000, 1.000000000000000000, 1.000000000000000000, 1.000000000000000000, 1.000000000000000000, 1.000000000000000000, 1.000000000000000000, 1.000000000000000000, 1.000000000000000000, 1.000000000000000000, 1.000000000000000000, 1.000000000000000000, 1.000000000000000000, 1.000000000000000000, 1.000000000000000000, 1.000000000000000000, 1.000000000000000000, 1.000000000000000000, 1.000000000000000000, 1.000000000000000000, 1.000000000000000000, 1.000000000000000000, 1.000000000000000000, 1.000000000000000000, 1.000000000000000000, 1.000000000000000000, 1.000000000000000000, 1.000000000000000000, 1.000000000000000000, 1.000000000000000000, 1.000000000000000000, 1.000000000000000000, 1.000000000000000000, 1.000000000000000000, 1.000000000000000000, 1.000000000000000000, 1.000000000000000000, 1.000000000000000000, 1.000000000000000000, 1.000000000000000000, 1.000000000000000000, 1.000000000000000000, 1.000000000000000000, 1.000000000000000000, 1.000000000000000000, 1.000000000000000000, 1.000000000000000000, 1.000000000000000000, 1.000000000000000000, 1.000000000000000000),
 ( 0.3333333333333333703, 0.3333333333333333703, 0.3333333333333333703, 0.3333333333333333703, 0.3333333333333333703, 0.3333333333333333703, 0.3333333333333333703, 0.3333333333333333703, 0.3333333333333333703, 0.3333333333333333703, 0.3333333333333333703, 0.3333333333333333703, 0.3333333333333333703, 0.3333333333333333703, 0.3333333333333333703, 0.3333333333333333703, 0.3333333333333333703, 0.3333333333333333703, 0.3333333333333333703, 0.3333333333333333703, 0.3333333333333333703, 0.3333333333333333703, 0.3333333333333333703, 0.3333333333333333703, 0.3333333333333333703, 0.3333333333333333703, 0.3333333333333333703, 0.3333333333333333703, 0.3333333333333333703, 0.3333333333333333703, 0.3333333333333333703, 0.3333333333333333703, 0.3333333333333333703, 0.3333333333333333703, 0.3333333333333333703, 0.3333333333333333703, 0.3333333333333333703, 0.3333333333333333703, 0.3333333333333333703, 0.3333333333333333703, 0.3333333333333333703, 0.3333333333333333703, 0.3333333333333333703, 0.3333333333333333703, 0.3333333333333333703, 0.3333333333333333703, 0.3333333333333333703, 0.3333333333333333703, 0.3333333333333333703, 0.3333333333333333703, 0.3333333333333333703, 0.3333333333333333703, 0.3333333333333333703, 0.3333333333333333703, 0.3333333333333333703, 0.3333333333333333703, 0.3333333333333333703, 0.3333333333333333703, 0.3333333333333333703, 0.3333333333333333703, 0.3333333333333333703, 0.3333333333333333703, 0.3333333333333333703, 0.3333333333333333703, 0.3333333333333333703, 0.3333333333333333703, 0.3333333333333333703, 0.3333333333333333703, 0.3333333333333333703, 0.3333333333333333703, 0.3333333333333333703, 0.3333333333333333703, 0.3333333333333333703, 0.3333333333333333703, 0.3333333333333333703, 0.3333333333333333703, 0.3333333333333333703, 0.3333333333333333703, 0.3333333333333333703, 0.3333333333333333703, 0.3333333333333333703, 0.3333333333333333703, 0.3333333333333333703, 0.3333333333333333703, 0.3333333333333333703, 0.3333333333333333703, 0.3333333333333333703, 0.3333333333333333703, 0.3333333333333333703, 0.3333333333333333703, 0.3333333333333333703, 0.3333333333333333703, 0.3333333333333333703, 0.3333333333333333703, 0.3333333333333333703, 0.3333333333333333703, 0.3333333333333333703, 0.3333333333333333703, 0.3333333333333333703, 0.3333333333333333703, 0.3333333333333333703, 0.3333333333333333703, 0.3333333333333333703, 0.3333333333333333703, 0.3333333333333333703, 0.3333333333333333703, 0.3333333333333333703, 0.3333333333333333703, 0.3333333333333333703, 0.3333333333333333703, 0.3333333333333333703, 0.3333333333333333703, 0.3333333333333333703, 0.3333333333333333703, 0.3333333333333333703, 0.3333333333333333703, 0.3333333333333333703, 0.3333333333333333703, 0.3333333333333333703, 0.3333333333333333703, 0.3333333333333333703, 0.3333333333333333703, 0.3333333333333333703, 0.3333333333333333703, 0.3333333333333333703, 0.3333333333333333703, 0.3333333333333333703, 0.3333333333333333703, 0.3333333333333333703, 0.3333333333333333703, 0.3333333333333333703, 0.3333333333333333703, 0.3333333333333333703, 0.3333333333333333703, 0.3333333333333333703, 0.3333333333333333703, 0.3333333333333333703, 0.3333333333333333703, 0.3333333333333333703, 0.3333333333333333703, 0.3333333333333333703, 0.3333333333333333703, 0.3333333333333333703, 0.3333333333333333703, 0.3333333333333333703, 0.3333333333333333703, 0.3333333333333333703, 0.3333333333333333703, 0.3333333333333333703, 0.3333333333333333703, 0.3333333333333333703, 0.3333333333333333703, 0.3333333333333333703, 0.3333333333333333703, 0.3333333333333333703, 0.3333333333333333703, 0.3333333333333333703, 0.3333333333333333703, 0.3333333333333333703, 0.3333333333333333703, 0.3333333333333333703, 0.3333333333333333703, 0.3333333333333333703, 0.3333333333333333703, 0.3333333333333333703, 0.3333333333333333703, 0.3333333333333333703, 0.3333333333333333703, 0.3333333333333333703, 0.3333333333333333703, 0.3333333333333333703, 0.3333333333333333703, 0.3333333333333333703, 0.3333333333333333703, 0.3333333333333333703, 0.3333333333333333703, 0.3333333333333333703, 0.3333333333333333703, 0.3333333333333333703, 0.3333333333333333703, 0.3333333333333333703, 0.3333333333333333703, 0.3333333333333333703, 0.3333333333333333703, 0.3333333333333333703, 0.3333333333333333703, 0.3333333333333333703, 0.3333333333333333703, 0.3333333333333333703, 0.3333333333333333703, 0.3333333333333333703, 0.3333333333333333703, 0.3333333333333333703, 0.3333333333333333703, 0.3333333333333333703, 0.3333333333333333703, 0.3333333333333333703, 0.3333333333333333703, 0.3333333333333333703, 0.3333333333333333703, 0.3333333333333333703, 0.3333333333333333703, 0.3333333333333333703, 0.3333333333333333703, 0.3333333333333333703, 0.3333333333333333703, 0.3333333333333333703, 0.3333333333333333703, 0.3333333333333333703, 0.3333333333333333703, 0.3333333333333333703, 0.3333333333333333703, 0.3333333333333333703, 0.3333333333333333703, 0.3333333333333333703, 0.3333333333333333703, 0.3333333333333333703, 0.3333333333333333703, 0.3333333333333333703, 0.3333333333333333703, 0.3333333333333333703, 0.3333333333333333703, 0.3333333333333333703, 0.3333333333333333703, 0.3333333333333333703, 0.3333333333333333703, 0.3333333333333333703, 0.3333333333333333703, 0.3333333333333333703, 0.3333333333333333703, 0.3333333333333333703, 0.3333333333333333703, 0.3333333333333333703, 0.3333333333333333703, 0.3333333333333333703, 0.3333333333333333703, 0.3333333333333333703, 0.3333333333333333703, 0.3333333333333333703, 0.3333333333333333703, 0.3333333333333333703, 0.3333333333333333703, 0.3333333333333333703, 0.3333333333333333703, 0.3333333333333333703, 0.3333333333333333703, 0.3333333333333333703, 0.3333333333333333703, 0.3333333333333333703, 0.3333333333333333703, 0.3333333333333333703, 0.3333333333333333703, 0.3333333333333333703, 0.3333333333333333703, 0.3333333333333333703, 0.3333333333333333703, 0.3333333333333333703, 0.3333333333333333703, 0.3333333333333333703, 0.3333333333333333703, 0.3333333333333333703, 0.3333333333333333703, 0.3333333333333333703, 0.3333333333333333703, 0.3333333333333333703, 0.3333333333333333703, 0.3333333333333333703, 0.3333333333333333703, 0.3333333333333333703, 0.3333333333333333703, 0.3333333333333333703, 0.3333333333333333703, 0.3333333333333333703, 0.3333333333333333703, 0.3333333333333333703, 0.3333333333333333703, 0.3333333333333333703, 0.3333333333333333703, 0.3333333333333333703, 0.3333333333333333703, 0.3333333333333333703, 0.3333333333333333703, 0.3333333333333333703, 0.3333333333333333703, 0.3333333333333333703, 0.3333333333333333703, 0.3333333333333333703, 0.3333333333333333703, 0.3333333333333333703, 0.3333333333333333703, 0.3333333333333333703, 0.3333333333333333703, 0.3333333333333333703, 0.3333333333333333703, 0.3333333333333333703, 0.3333333333333333703, 0.3333333333333333703, 0.3333333333333333703, 0.3333333333333333703, 0.3333333333333333703, 0.3333333333333333703, 0.3333333333333333703, 0.3333333333333333703, 0.3333333333333333703, 0.3333333333333333703, 0.3333333333333333703, 0.3333333333333333703, 0.3333333333333333703, 0.3333333333333333703, 0.3333333333333333703, 0.3333333333333333703, 0.3333333333333333703, 0.3333333333333333703, 0.3333333333333333703, 0.3333333333333333703, 0.3333333333333333703, 0.3333333333333333703, 0.3333333333333333703, 0.3333333333333333703, 0.3333333333333333703, 0.3333333333333333703, 0.3333333333333333703, 0.3333333333333333703, 0.3333333333333333703, 0.3333333333333333703, 0.3333333333333333703, 0.3333333333333333703, 0.3333333333333333703, 0.3333333333333333703, 0.3333333333333333703, 0.3333333333333333703, 0.3333333333333333703, 0.3333333333333333703, 0.3333333333333333703, 0.3333333333333333703, 0.3333333333333333703, 0.3333333333333333703, 0.3333333333333333703, 0.3333333333333333703, 0.3333333333333333703),
 ( 0.3333333333333333703, 0.3333333333333333703, 0.3333333333333333703, 0.3333333333333333703, 0.3333333333333333703, 0.3333333333333333703, 0.3333333333333333703, 0.3333333333333333703, 0.3333333333333333703, 0.3333333333333333703, 0.3333333333333333703, 0.3333333333333333703, 0.3333333333333333703, 0.3333333333333333703, 0.3333333333333333703, 0.3333333333333333703, 0.3333333333333333703, 0.3333333333333333703, 0.3333333333333333703, 0.3333333333333333703, 0.3333333333333333703, 0.3333333333333333703, 0.3333333333333333703, 0.3333333333333333703, 0.3333333333333333703, 0.3333333333333333703, 0.3333333333333333703, 0.3333333333333333703, 0.3333333333333333703, 0.3333333333333333703, 0.3333333333333333703, 0.3333333333333333703, 0.3333333333333333703, 0.3333333333333333703, 0.3333333333333333703, 0.3333333333333333703, 0.3333333333333333703, 0.3333333333333333703, 0.3333333333333333703, 0.3333333333333333703, 0.3333333333333333703, 0.3333333333333333703, 0.3333333333333333703, 0.3333333333333333703, 0.3333333333333333703, 0.3333333333333333703, 0.3333333333333333703, 0.3333333333333333703, 0.3333333333333333703, 0.3333333333333333703, 0.3333333333333333703, 0.3333333333333333703, 0.3333333333333333703, 0.3333333333333333703, 0.3333333333333333703, 0.3333333333333333703, 0.3333333333333333703, 0.3333333333333333703, 0.3333333333333333703, 0.3333333333333333703, 0.3333333333333333703, 0.3333333333333333703, 0.3333333333333333703, 0.3333333333333333703, 0.3333333333333333703, 0.3333333333333333703, 0.3333333333333333703, 0.3333333333333333703, 0.3333333333333333703, 0.3333333333333333703, 0.3333333333333333703, 0.3333333333333333703, 0.3333333333333333703, 0.3333333333333333703, 0.3333333333333333703, 0.3333333333333333703, 0.3333333333333333703, 0.3333333333333333703, 0.3333333333333333703, 0.3333333333333333703, 0.3333333333333333703, 0.3333333333333333703, 0.3333333333333333703, 0.3333333333333333703, 0.3333333333333333703, 0.3333333333333333703, 0.3333333333333333703, 0.3333333333333333703, 0.3333333333333333703, 0.3333333333333333703, 0.3333333333333333703, 0.3333333333333333703, 0.3333333333333333703, 0.3333333333333333703, 0.3333333333333333703, 0.3333333333333333703, 0.3333333333333333703, 0.3333333333333333703, 0.3333333333333333703, 0.3333333333333333703, 0.3333333333333333703, 0.3333333333333333703, 0.3333333333333333703, 0.3333333333333333703, 0.3333333333333333703, 0.3333333333333333703, 0.3333333333333333703, 0.3333333333333333703, 0.3333333333333333703, 0.3333333333333333703, 0.3333333333333333703, 0.3333333333333333703, 0.3333333333333333703, 0.3333333333333333703, 0.3333333333333333703, 0.3333333333333333703, 0.3333333333333333703, 0.3333333333333333703, 0.3333333333333333703, 0.3333333333333333703, 0.3333333333333333703, 0.3333333333333333703, 0.3333333333333333703, 0.3333333333333333703, 0.3333333333333333703, 0.3333333333333333703, 0.3333333333333333703, 0.3333333333333333703, 0.3333333333333333703, 0.3333333333333333703, 0.3333333333333333703, 0.3333333333333333703, 0.3333333333333333703, 0.3333333333333333703, 0.3333333333333333703, 0.3333333333333333703, 0.3333333333333333703, 0.3333333333333333703, 0.3333333333333333703, 0.3333333333333333703, 0.3333333333333333703, 0.3333333333333333703, 0.3333333333333333703, 0.3333333333333333703, 0.3333333333333333703, 0.3333333333333333703, 0.3333333333333333703, 0.3333333333333333703, 0.3333333333333333703, 0.3333333333333333703, 0.3333333333333333703, 0.3333333333333333703, 0.3333333333333333703, 0.3333333333333333703, 0.3333333333333333703, 0.3333333333333333703, 0.3333333333333333703, 0.3333333333333333703, 0.3333333333333333703, 0.3333333333333333703, 0.3333333333333333703, 0.3333333333333333703, 0.3333333333333333703, 0.3333333333333333703, 0.3333333333333333703, 0.3333333333333333703, 0.3333333333333333703, 0.3333333333333333703, 0.3333333333333333703, 0.3333333333333333703, 0.3333333333333333703, 0.3333333333333333703, 0.3333333333333333703, 0.3333333333333333703, 0.3333333333333333703, 0.3333333333333333703, 0.3333333333333333703, 0.3333333333333333703, 0.3333333333333333703, 0.3333333333333333703, 0.3333333333333333703, 0.3333333333333333703, 0.3333333333333333703, 0.3333333333333333703, 0.3333333333333333703, 0.3333333333333333703, 0.3333333333333333703, 0.3333333333333333703, 0.3333333333333333703, 0.3333333333333333703, 0.3333333333333333703, 0.3333333333333333703, 0.3333333333333333703, 0.3333333333333333703, 0.3333333333333333703, 0.3333333333333333703, 0.3333333333333333703, 0.3333333333333333703, 0.3333333333333333703, 0.3333333333333333703, 0.3333333333333333703, 0.3333333333333333703, 0.3333333333333333703, 0.3333333333333333703, 0.3333333333333333703, 0.3333333333333333703, 0.3333333333333333703, 0.3333333333333333703, 0.3333333333333333703, 0.3333333333333333703, 0.3333333333333333703, 0.3333333333333333703, 0.3333333333333333703, 0.3333333333333333703, 0.3333333333333333703, 0.3333333333333333703, 0.3333333333333333703, 0.3333333333333333703, 0.3333333333333333703, 0.3333333333333333703, 0.3333333333333333703, 0.3333333333333333703, 0.3333333333333333703, 0.3333333333333333703, 0.3333333333333333703, 0.3333333333333333703, 0.3333333333333333703, 0.3333333333333333703, 0.3333333333333333703, 0.3333333333333333703, 0.3333333333333333703, 0.3333333333333333703, 0.3333333333333333703, 0.3333333333333333703, 0.3333333333333333703, 0.3333333333333333703, 0.3333333333333333703, 0.3333333333333333703, 0.3333333333333333703, 0.3333333333333333703, 0.3333333333333333703, 0.3333333333333333703, 0.3333333333333333703, 0.3333333333333333703, 0.3333333333333333703, 0.3333333333333333703, 0.3333333333333333703, 0.3333333333333333703, 0.3333333333333333703, 0.3333333333333333703, 0.3333333333333333703, 0.3333333333333333703, 0.3333333333333333703, 0.3333333333333333703, 0.3333333333333333703, 0.3333333333333333703, 0.3333333333333333703, 0.3333333333333333703, 0.3333333333333333703, 0.3333333333333333703, 0.3333333333333333703, 0.3333333333333333703, 0.3333333333333333703, 0.3333333333333333703, 0.3333333333333333703, 0.3333333333333333703, 0.3333333333333333703, 0.3333333333333333703, 0.3333333333333333703, 0.3333333333333333703, 0.3333333333333333703, 0.3333333333333333703, 0.3333333333333333703, 0.3333333333333333703, 0.3333333333333333703, 0.3333333333333333703, 0.3333333333333333703, 0.3333333333333333703, 0.3333333333333333703, 0.3333333333333333703, 0.3333333333333333703, 0.3333333333333333703, 0.3333333333333333703, 0.3333333333333333703, 0.3333333333333333703, 0.3333333333333333703, 0.3333333333333333703, 0.3333333333333333703, 0.3333333333333333703, 0.3333333333333333703, 0.3333333333333333703, 0.3333333333333333703, 0.3333333333333333703, 0.3333333333333333703, 0.3333333333333333703, 0.3333333333333333703, 0.3333333333333333703, 0.3333333333333333703, 0.3333333333333333703, 0.3333333333333333703, 0.3333333333333333703, 0.3333333333333333703, 0.3333333333333333703, 0.3333333333333333703, 0.3333333333333333703, 0.3333333333333333703, 0.3333333333333333703, 0.3333333333333333703, 0.3333333333333333703, 0.3333333333333333703, 0.3333333333333333703, 0.3333333333333333703, 0.3333333333333333703, 0.3333333333333333703, 0.3333333333333333703, 0.3333333333333333703, 0.3333333333333333703, 0.3333333333333333703, 0.3333333333333333703, 0.3333333333333333703, 0.3333333333333333703, 0.3333333333333333703, 0.3333333333333333703, 0.3333333333333333703, 0.3333333333333333703, 0.3333333333333333703, 0.3333333333333333703, 0.3333333333333333703, 0.3333333333333333703, 0.3333333333333333703, 0.3333333333333333703, 0.3333333333333333703, 0.3333333333333333703, 0.3333333333333333703, 0.3333333333333333703, 0.3333333333333333703, 0.3333333333333333703, 0.3333333333333333703, 0.3333333333333333703, 0.3333333333333333703),
 ( 1.000000000000000000, 1.000000000000000000, 1.000000000000000000, 1.000000000000000000, 1.000000000000000000, 1.000000000000000000, 1.000000000000000000, 1.000000000000000000, 1.000000000000000000, 1.000000000000000000, 1.000000000000000000, 1.000000000000000000, 1.000000000000000000, 1.000000000000000000, 1.000000000000000000, 1.000000000000000000, 1.000000000000000000, 1.000000000000000000, 1.000000000000000000, 1.000000000000000000, 1.000000000000000000, 1.000000000000000000, 1.000000000000000000, 1.000000000000000000, 1.000000000000000000, 1.000000000000000000, 1.000000000000000000, 1.000000000000000000, 1.000000000000000000, 1.000000000000000000, 1.000000000000000000, 1.000000000000000000, 1.000000000000000000, 1.000000000000000000, 1.000000000000000000, 1.000000000000000000, 1.000000000000000000, 1.000000000000000000, 1.000000000000000000, 1.000000000000000000, 1.000000000000000000, 1.000000000000000000, 1.000000000000000000, 1.000000000000000000, 1.000000000000000000, 1.000000000000000000, 1.000000000000000000, 1.000000000000000000, 1.000000000000000000, 1.000000000000000000, 1.000000000000000000, 1.000000000000000000, 1.000000000000000000, 1.000000000000000000, 1.000000000000000000, 1.000000000000000000, 1.000000000000000000, 1.000000000000000000, 1.000000000000000000, 1.000000000000000000, 1.000000000000000000, 1.000000000000000000, 1.000000000000000000, 1.000000000000000000, 1.000000000000000000, 1.000000000000000000, 1.000000000000000000, 1.000000000000000000, 1.000000000000000000, 1.000000000000000000, 1.000000000000000000, 1.000000000000000000, 1.000000000000000000, 1.000000000000000000, 1.000000000000000000, 1.000000000000000000, 1.000000000000000000, 1.000000000000000000, 1.000000000000000000, 1.000000000000000000, 1.000000000000000000, 1.000000000000000000, 1.000000000000000000, 1.000000000000000000, 1.000000000000000000, 1.000000000000000000, 1.000000000000000000, 1.000000000000000000, 1.000000000000000000, 1.000000000000000000, 1.000000000000000000, 1.000000000000000000, 1.000000000000000000, 1.000000000000000000, 1.000000000000000000, 1.000000000000000000, 1.000000000000000000, 1.000000000000000000, 1.000000000000000000, 1.000000000000000000, 1.000000000000000000, 1.000000000000000000, 1.000000000000000000, 1.000000000000000000, 1.000000000000000000, 1.000000000000000000, 1.000000000000000000, 1.000000000000000000, 1.000000000000000000, 1.000000000000000000, 1.000000000000000000, 1.000000000000000000, 1.000000000000000000, 1.000000000000000000, 1.000000000000000000, 1.000000000000000000, 1.000000000000000000, 1.000000000000000000, 1.000000000000000000, 1.000000000000000000, 1.000000000000000000, 1.000000000000000000, 1.000000000000000000, 1.000000000000000000, 1.000000000000000000, 1.000000000000000000, 1.000000000000000000, 1.000000000000000000, 1.000000000000000000, 1.000000000000000000, 1.000000000000000000, 1.000000000000000000, 1.000000000000000000, 1.000000000000000000, 1.000000000000000000, 1.000000000000000000, 1.000000000000000000, 1.000000000000000000, 1.000000000000000000, 1.000000000000000000, 1.000000000000000000, 1.000000000000000000, 1.000000000000000000, 1.000000000000000000, 1.000000000000000000, 1.000000000000000000, 1.000000000000000000, 1.000000000000000000, 1.000000000000000000, 1.000000000000000000, 1.000000000000000000, 1.000000000000000000, 1.000000000000000000, 1.000000000000000000, 1.000000000000000000, 1.000000000000000000, 1.000000000000000000, 1.000000000000000000, 1.000000000000000000, 1.000000000000000000, 1.000000000000000000, 1.000000000000000000, 1.000000000000000000, 1.000000000000000000, 1.000000000000000000, 1.000000000000000000, 1.000000000000000000, 1.000000000000000000, 1.000000000000000000, 1.000000000000000000, 1.000000000000000000, 1.000000000000000000, 1.000000000000000000, 1.000000000000000000, 1.000000000000000000, 1.000000000000000000, 1.000000000000000000, 1.000000000000000000, 1.000000000000000000, 1.000000000000000000, 1.000000000000000000, 1.000000000000000000, 1.000000000000000000, 1.000000000000000000, 1.000000000000000000, 1.000000000000000000, 1.000000000000000000, 1.000000000000000000, 1.000000000000000000, 1.000000000000000000, 1.000000000000000000, 1.000000000000000000, 1.000000000000000000, 1.000000000000000000, 1.000000000000000000, 1.000000000000000000, 1.000000000000000000, 1.000000000000000000, 1.000000000000000000, 1.000000000000000000, 1.000000000000000000, 1.000000000000000000, 1.000000000000000000, 1.000000000000000000, 1.000000000000000000, 1.000000000000000000, 1.000000000000000000, 1.000000000000000000, 1.000000000000000000, 1.000000000000000000, 1.000000000000000000, 1.000000000000000000, 1.000000000000000000, 1.000000000000000000, 1.000000000000000000, 1.000000000000000000, 1.000000000000000000, 1.000000000000000000, 1.000000000000000000, 1.000000000000000000, 1.000000000000000000, 1.000000000000000000, 1.000000000000000000, 1.000000000000000000, 1.000000000000000000, 1.000000000000000000, 1.000000000000000000, 1.000000000000000000, 1.000000000000000000, 1.000000000000000000, 1.000000000000000000, 1.000000000000000000, 1.000000000000000000, 1.000000000000000000, 1.000000000000000000, 1.000000000000000000, 1.000000000000000000, 1.000000000000000000, 1.000000000000000000, 1.000000000000000000, 1.000000000000000000, 1.000000000000000000, 1.000000000000000000, 1.000000000000000000, 1.000000000000000000, 1.000000000000000000, 1.000000000000000000, 1.000000000000000000, 1.000000000000000000, 1.000000000000000000, 1.000000000000000000, 1.000000000000000000, 1.000000000000000000, 1.000000000000000000, 1.000000000000000000, 1.000000000000000000, 1.000000000000000000, 1.000000000000000000, 1.000000000000000000, 1.000000000000000000, 1.000000000000000000, 1.000000000000000000, 1.000000000000000000, 1.000000000000000000, 1.000000000000000000, 1.000000000000000000, 1.000000000000000000, 1.000000000000000000, 1.000000000000000000, 1.000000000000000000, 1.000000000000000000, 1.000000000000000000, 1.000000000000000000, 1.000000000000000000, 1.000000000000000000, 1.000000000000000000, 1.000000000000000000, 1.000000000000000000, 1.000000000000000000, 1.000000000000000000, 1.000000000000000000, 1.000000000000000000, 1.000000000000000000, 1.000000000000000000, 1.000000000000000000, 1.000000000000000000, 1.000000000000000000, 1.000000000000000000, 1.000000000000000000, 1.000000000000000000, 1.000000000000000000, 1.000000000000000000, 1.000000000000000000, 1.000000000000000000, 1.000000000000000000, 1.000000000000000000, 1.000000000000000000, 1.000000000000000000, 1.000000000000000000, 1.000000000000000000, 1.000000000000000000, 1.000000000000000000, 1.000000000000000000, 1.000000000000000000, 1.000000000000000000, 1.000000000000000000, 1.000000000000000000, 1.000000000000000000, 1.000000000000000000, 1.000000000000000000, 1.000000000000000000, 1.000000000000000000, 1.000000000000000000, 1.000000000000000000, 1.000000000000000000, 1.000000000000000000, 1.000000000000000000, 1.000000000000000000, 1.000000000000000000, 1.000000000000000000, 1.000000000000000000, 1.000000000000000000, 1.000000000000000000, 1.000000000000000000, 1.000000000000000000, 1.000000000000000000, 1.000000000000000000, 1.000000000000000000, 1.000000000000000000, 1.000000000000000000, 1.000000000000000000, 1.000000000000000000, 1.000000000000000000, 1.000000000000000000, 1.000000000000000000, 1.000000000000000000, 1.000000000000000000, 1.000000000000000000, 1.000000000000000000, 1.000000000000000000),
 ( 0.3333333333333333703, 0.3333333333333333703, 0.3333333333333333703, 0.3333333333333333703, 0.3333333333333333703, 0.3333333333333333703, 0.3333333333333333703, 0.3333333333333333703, 0.3333333333333333703, 0.3333333333333333703, 0.3333333333333333703, 0.3333333333333333703, 0.3333333333333333703, 0.3333333333333333703, 0.3333333333333333703, 0.3333333333333333703, 0.3333333333333333703, 0.3333333333333333703, 0.3333333333333333703, 0.3333333333333333703, 0.3333333333333333703, 0.3333333333333333703, 0.3333333333333333703, 0.3333333333333333703, 0.3333333333333333703, 0.3333333333333333703, 0.3333333333333333703, 0.3333333333333333703, 0.3333333333333333703, 0.3333333333333333703, 0.3333333333333333703, 0.3333333333333333703, 0.3333333333333333703, 0.3333333333333333703, 0.3333333333333333703, 0.3333333333333333703, 0.3333333333333333703, 0.3333333333333333703, 0.3333333333333333703, 0.3333333333333333703, 0.3333333333333333703, 0.3333333333333333703, 0.3333333333333333703, 0.3333333333333333703, 0.3333333333333333703, 0.3333333333333333703, 0.3333333333333333703, 0.3333333333333333703, 0.3333333333333333703, 0.3333333333333333703, 0.3333333333333333703, 0.3333333333333333703, 0.3333333333333333703, 0.3333333333333333703, 0.3333333333333333703, 0.3333333333333333703, 0.3333333333333333703, 0.3333333333333333703, 0.3333333333333333703, 0.3333333333333333703, 0.3333333333333333703, 0.3333333333333333703, 0.3333333333333333703, 0.3333333333333333703, 0.3333333333333333703, 0.3333333333333333703, 0.3333333333333333703, 0.3333333333333333703, 0.3333333333333333703, 0.3333333333333333703, 0.3333333333333333703, 0.3333333333333333703, 0.3333333333333333703, 0.3333333333333333703, 0.3333333333333333703, 0.3333333333333333703, 0.3333333333333333703, 0.3333333333333333703, 0.3333333333333333703, 0.3333333333333333703, 0.3333333333333333703, 0.3333333333333333703, 0.3333333333333333703, 0.3333333333333333703, 0.3333333333333333703, 0.3333333333333333703, 0.3333333333333333703, 0.3333333333333333703, 0.3333333333333333703, 0.3333333333333333703, 0.3333333333333333703, 0.3333333333333333703, 0.3333333333333333703, 0.3333333333333333703, 0.3333333333333333703, 0.3333333333333333703, 0.3333333333333333703, 0.3333333333333333703, 0.3333333333333333703, 0.3333333333333333703, 0.3333333333333333703, 0.3333333333333333703, 0.3333333333333333703, 0.3333333333333333703, 0.3333333333333333703, 0.3333333333333333703, 0.3333333333333333703, 0.3333333333333333703, 0.3333333333333333703, 0.3333333333333333703, 0.3333333333333333703, 0.3333333333333333703, 0.3333333333333333703, 0.3333333333333333703, 0.3333333333333333703, 0.3333333333333333703, 0.3333333333333333703, 0.3333333333333333703, 0.3333333333333333703, 0.3333333333333333703, 0.3333333333333333703, 0.3333333333333333703, 0.3333333333333333703, 0.3333333333333333703, 0.3333333333333333703, 0.3333333333333333703, 0.3333333333333333703, 0.3333333333333333703, 0.3333333333333333703, 0.3333333333333333703, 0.3333333333333333703, 0.3333333333333333703, 0.3333333333333333703, 0.3333333333333333703, 0.3333333333333333703, 0.3333333333333333703, 0.3333333333333333703, 0.3333333333333333703, 0.3333333333333333703, 0.3333333333333333703, 0.3333333333333333703, 0.3333333333333333703, 0.3333333333333333703, 0.3333333333333333703, 0.3333333333333333703, 0.3333333333333333703, 0.3333333333333333703, 0.3333333333333333703, 0.3333333333333333703, 0.3333333333333333703, 0.3333333333333333703, 0.3333333333333333703, 0.3333333333333333703, 0.3333333333333333703, 0.3333333333333333703, 0.3333333333333333703, 0.3333333333333333703, 0.3333333333333333703, 0.3333333333333333703, 0.3333333333333333703, 0.3333333333333333703, 0.3333333333333333703, 0.3333333333333333703, 0.3333333333333333703, 0.3333333333333333703, 0.3333333333333333703, 0.3333333333333333703, 0.3333333333333333703, 0.3333333333333333703, 0.3333333333333333703, 0.3333333333333333703, 0.3333333333333333703, 0.3333333333333333703, 0.3333333333333333703, 0.3333333333333333703, 0.3333333333333333703, 0.3333333333333333703, 0.3333333333333333703, 0.3333333333333333703, 0.3333333333333333703, 0.3333333333333333703, 0.3333333333333333703, 0.3333333333333333703, 0.3333333333333333703, 0.3333333333333333703, 0.3333333333333333703, 0.3333333333333333703, 0.3333333333333333703, 0.3333333333333333703, 0.3333333333333333703, 0.3333333333333333703, 0.3333333333333333703, 0.3333333333333333703, 0.3333333333333333703, 0.3333333333333333703, 0.3333333333333333703, 0.3333333333333333703, 0.3333333333333333703, 0.3333333333333333703, 0.3333333333333333703, 0.3333333333333333703, 0.3333333333333333703, 0.3333333333333333703, 0.3333333333333333703, 0.3333333333333333703, 0.3333333333333333703, 0.3333333333333333703, 0.3333333333333333703, 0.3333333333333333703, 0.3333333333333333703, 0.3333333333333333703, 0.3333333333333333703, 0.3333333333333333703, 0.3333333333333333703, 0.3333333333333333703, 0.3333333333333333703, 0.3333333333333333703, 0.3333333333333333703, 0.3333333333333333703, 0.3333333333333333703, 0.3333333333333333703, 0.3333333333333333703, 0.3333333333333333703, 0.3333333333333333703, 0.3333333333333333703, 0.3333333333333333703, 0.3333333333333333703, 0.3333333333333333703, 0.3333333333333333703, 0.3333333333333333703, 0.3333333333333333703, 0.3333333333333333703, 0.3333333333333333703, 0.3333333333333333703, 0.3333333333333333703, 0.3333333333333333703, 0.3333333333333333703, 0.3333333333333333703, 0.3333333333333333703, 0.3333333333333333703, 0.3333333333333333703, 0.3333333333333333703, 0.3333333333333333703, 0.3333333333333333703, 0.3333333333333333703, 0.3333333333333333703, 0.3333333333333333703, 0.3333333333333333703, 0.3333333333333333703, 0.3333333333333333703, 0.3333333333333333703, 0.3333333333333333703, 0.3333333333333333703, 0.3333333333333333703, 0.3333333333333333703, 0.3333333333333333703, 0.3333333333333333703, 0.3333333333333333703, 0.3333333333333333703, 0.3333333333333333703, 0.3333333333333333703, 0.3333333333333333703, 0.3333333333333333703, 0.3333333333333333703, 0.3333333333333333703, 0.3333333333333333703, 0.3333333333333333703, 0.3333333333333333703, 0.3333333333333333703, 0.3333333333333333703, 0.3333333333333333703, 0.3333333333333333703, 0.3333333333333333703, 0.3333333333333333703, 0.3333333333333333703, 0.3333333333333333703, 0.3333333333333333703, 0.3333333333333333703, 0.3333333333333333703, 0.3333333333333333703, 0.3333333333333333703, 0.3333333333333333703, 0.3333333333333333703, 0.3333333333333333703, 0.3333333333333333703, 0.3333333333333333703, 0.3333333333333333703, 0.3333333333333333703, 0.3333333333333333703, 0.3333333333333333703, 0.3333333333333333703, 0.3333333333333333703, 0.3333333333333333703, 0.3333333333333333703, 0.3333333333333333703, 0.3333333333333333703, 0.3333333333333333703, 0.3333333333333333703, 0.3333333333333333703, 0.3333333333333333703, 0.3333333333333333703, 0.3333333333333333703, 0.3333333333333333703, 0.3333333333333333703, 0.3333333333333333703, 0.3333333333333333703, 0.3333333333333333703, 0.3333333333333333703, 0.3333333333333333703, 0.3333333333333333703, 0.3333333333333333703, 0.3333333333333333703, 0.3333333333333333703, 0.3333333333333333703, 0.3333333333333333703, 0.3333333333333333703, 0.3333333333333333703, 0.3333333333333333703, 0.3333333333333333703, 0.3333333333333333703, 0.3333333333333333703, 0.3333333333333333703, 0.3333333333333333703, 0.3333333333333333703, 0.3333333333333333703, 0.3333333333333333703, 0.3333333333333333703, 0.3333333333333333703, 0.3333333333333333703, 0.3333333333333333703, 0.3333333333333333703, 0.3333333333333333703, 0.3333333333333333703, 0.3333333333333333703, 0.3333333333333333703, 0.3333333333333333703, 0.3333333333333333703, 0.3333333333333333703, 0.3333333333333333703, 0.3333333333333333703),
 ( 0.3333333333333333703, 0.3333333333333333703, 0.3333333333333333703, 0.3333333333333333703, 0.3333333333333333703, 0.3333333333333333703, 0.3333333333333333703, 0.3333333333333333703, 0.3333333333333333703, 0.3333333333333333703, 0.3333333333333333703, 0.3333333333333333703, 0.3333333333333333703, 0.3333333333333333703, 0.3333333333333333703, 0.3333333333333333703, 0.3333333333333333703, 0.3333333333333333703, 0.3333333333333333703, 0.3333333333333333703, 0.3333333333333333703, 0.3333333333333333703, 0.3333333333333333703, 0.3333333333333333703, 0.3333333333333333703, 0.3333333333333333703, 0.3333333333333333703, 0.3333333333333333703, 0.3333333333333333703, 0.3333333333333333703, 0.3333333333333333703, 0.3333333333333333703, 0.3333333333333333703, 0.3333333333333333703, 0.3333333333333333703, 0.3333333333333333703, 0.3333333333333333703, 0.3333333333333333703, 0.3333333333333333703, 0.3333333333333333703, 0.3333333333333333703, 0.3333333333333333703, 0.3333333333333333703, 0.3333333333333333703, 0.3333333333333333703, 0.3333333333333333703, 0.3333333333333333703, 0.3333333333333333703, 0.3333333333333333703, 0.3333333333333333703, 0.3333333333333333703, 0.3333333333333333703, 0.3333333333333333703, 0.3333333333333333703, 0.3333333333333333703, 0.3333333333333333703, 0.3333333333333333703, 0.3333333333333333703, 0.3333333333333333703, 0.3333333333333333703, 0.3333333333333333703, 0.3333333333333333703, 0.3333333333333333703, 0.3333333333333333703, 0.3333333333333333703, 0.3333333333333333703, 0.3333333333333333703, 0.3333333333333333703, 0.3333333333333333703, 0.3333333333333333703, 0.3333333333333333703, 0.3333333333333333703, 0.3333333333333333703, 0.3333333333333333703, 0.3333333333333333703, 0.3333333333333333703, 0.3333333333333333703, 0.3333333333333333703, 0.3333333333333333703, 0.3333333333333333703, 0.3333333333333333703, 0.3333333333333333703, 0.3333333333333333703, 0.3333333333333333703, 0.3333333333333333703, 0.3333333333333333703, 0.3333333333333333703, 0.3333333333333333703, 0.3333333333333333703, 0.3333333333333333703, 0.3333333333333333703, 0.3333333333333333703, 0.3333333333333333703, 0.3333333333333333703, 0.3333333333333333703, 0.3333333333333333703, 0.3333333333333333703, 0.3333333333333333703, 0.3333333333333333703, 0.3333333333333333703, 0.3333333333333333703, 0.3333333333333333703, 0.3333333333333333703, 0.3333333333333333703, 0.3333333333333333703, 0.3333333333333333703, 0.3333333333333333703, 0.3333333333333333703, 0.3333333333333333703, 0.3333333333333333703, 0.3333333333333333703, 0.3333333333333333703, 0.3333333333333333703, 0.3333333333333333703, 0.3333333333333333703, 0.3333333333333333703, 0.3333333333333333703, 0.3333333333333333703, 0.3333333333333333703, 0.3333333333333333703, 0.3333333333333333703, 0.3333333333333333703, 0.3333333333333333703, 0.3333333333333333703, 0.3333333333333333703, 0.3333333333333333703, 0.3333333333333333703, 0.3333333333333333703, 0.3333333333333333703, 0.3333333333333333703, 0.3333333333333333703, 0.3333333333333333703, 0.3333333333333333703, 0.3333333333333333703, 0.3333333333333333703, 0.3333333333333333703, 0.3333333333333333703, 0.3333333333333333703, 0.3333333333333333703, 0.3333333333333333703, 0.3333333333333333703, 0.3333333333333333703, 0.3333333333333333703, 0.3333333333333333703, 0.3333333333333333703, 0.3333333333333333703, 0.3333333333333333703, 0.3333333333333333703, 0.3333333333333333703, 0.3333333333333333703, 0.3333333333333333703, 0.3333333333333333703, 0.3333333333333333703, 0.3333333333333333703, 0.3333333333333333703, 0.3333333333333333703, 0.3333333333333333703, 0.3333333333333333703, 0.3333333333333333703, 0.3333333333333333703, 0.3333333333333333703, 0.3333333333333333703, 0.3333333333333333703, 0.3333333333333333703, 0.3333333333333333703, 0.3333333333333333703, 0.3333333333333333703, 0.3333333333333333703, 0.3333333333333333703, 0.3333333333333333703, 0.3333333333333333703, 0.3333333333333333703, 0.3333333333333333703, 0.3333333333333333703, 0.3333333333333333703, 0.3333333333333333703, 0.3333333333333333703, 0.3333333333333333703, 0.3333333333333333703, 0.3333333333333333703, 0.3333333333333333703, 0.3333333333333333703, 0.3333333333333333703, 0.3333333333333333703, 0.3333333333333333703, 0.3333333333333333703, 0.3333333333333333703, 0.3333333333333333703, 0.3333333333333333703, 0.3333333333333333703, 0.3333333333333333703, 0.3333333333333333703, 0.3333333333333333703, 0.3333333333333333703, 0.3333333333333333703, 0.3333333333333333703, 0.3333333333333333703, 0.3333333333333333703, 0.3333333333333333703, 0.3333333333333333703, 0.3333333333333333703, 0.3333333333333333703, 0.3333333333333333703, 0.3333333333333333703, 0.3333333333333333703, 0.3333333333333333703, 0.3333333333333333703, 0.3333333333333333703, 0.3333333333333333703, 0.3333333333333333703, 0.3333333333333333703, 0.3333333333333333703, 0.3333333333333333703, 0.3333333333333333703, 0.3333333333333333703, 0.3333333333333333703, 0.3333333333333333703, 0.3333333333333333703, 0.3333333333333333703, 0.3333333333333333703, 0.3333333333333333703, 0.3333333333333333703, 0.3333333333333333703, 0.3333333333333333703, 0.3333333333333333703, 0.3333333333333333703, 0.3333333333333333703, 0.3333333333333333703, 0.3333333333333333703, 0.3333333333333333703, 0.3333333333333333703, 0.3333333333333333703, 0.3333333333333333703, 0.3333333333333333703, 0.3333333333333333703, 0.3333333333333333703, 0.3333333333333333703, 0.3333333333333333703, 0.3333333333333333703, 0.3333333333333333703, 0.3333333333333333703, 0.3333333333333333703, 0.3333333333333333703, 0.3333333333333333703, 0.3333333333333333703, 0.3333333333333333703, 0.3333333333333333703, 0.3333333333333333703, 0.3333333333333333703, 0.3333333333333333703, 0.3333333333333333703, 0.3333333333333333703, 0.3333333333333333703, 0.3333333333333333703, 0.3333333333333333703, 0.3333333333333333703, 0.3333333333333333703, 0.3333333333333333703, 0.3333333333333333703, 0.3333333333333333703, 0.3333333333333333703, 0.3333333333333333703, 0.3333333333333333703, 0.3333333333333333703, 0.3333333333333333703, 0.3333333333333333703, 0.3333333333333333703, 0.3333333333333333703, 0.3333333333333333703, 0.3333333333333333703, 0.3333333333333333703, 0.3333333333333333703, 0.3333333333333333703, 0.3333333333333333703, 0.3333333333333333703, 0.3333333333333333703, 0.3333333333333333703, 0.3333333333333333703, 0.3333333333333333703, 0.3333333333333333703, 0.3333333333333333703, 0.3333333333333333703, 0.3333333333333333703, 0.3333333333333333703, 0.3333333333333333703, 0.3333333333333333703, 0.3333333333333333703, 0.3333333333333333703, 0.3333333333333333703, 0.3333333333333333703, 0.3333333333333333703, 0.3333333333333333703, 0.3333333333333333703, 0.3333333333333333703, 0.3333333333333333703, 0.3333333333333333703, 0.3333333333333333703, 0.3333333333333333703, 0.3333333333333333703, 0.3333333333333333703, 0.3333333333333333703, 0.3333333333333333703, 0.3333333333333333703, 0.3333333333333333703, 0.3333333333333333703, 0.3333333333333333703, 0.3333333333333333703, 0.3333333333333333703, 0.3333333333333333703, 0.3333333333333333703, 0.3333333333333333703, 0.3333333333333333703, 0.3333333333333333703, 0.3333333333333333703, 0.3333333333333333703, 0.3333333333333333703, 0.3333333333333333703, 0.3333333333333333703, 0.3333333333333333703, 0.3333333333333333703, 0.3333333333333333703, 0.3333333333333333703, 0.3333333333333333703, 0.3333333333333333703, 0.3333333333333333703, 0.3333333333333333703, 0.3333333333333333703, 0.3333333333333333703, 0.3333333333333333703, 0.3333333333333333703, 0.3333333333333333703, 0.3333333333333333703, 0.3333333333333333703, 0.3333333333333333703, 0.3333333333333333703, 0.3333333333333333703, 0.3333333333333333703, 0.3333333333333333703, 0.3333333333333333703, 0.3333333333333333703),
 ( 1.000000000000000000, 1.000000000000000000, 1.000000000000000000, 1.000000000000000000, 1.000000000000000000, 1.000000000000000000, 1.000000000000000000, 1.000000000000000000, 1.000000000000000000, 1.000000000000000000, 1.000000000000000000, 1.000000000000000000, 1.000000000000000000, 1.000000000000000000, 1.000000000000000000, 1.000000000000000000, 1.000000000000000000, 1.000000000000000000, 1.000000000000000000, 1.000000000000000000, 1.000000000000000000, 1.000000000000000000, 1.000000000000000000, 1.000000000000000000, 1.000000000000000000, 1.000000000000000000, 1.000000000000000000, 1.000000000000000000, 1.000000000000000000, 1.000000000000000000, 1.000000000000000000, 1.000000000000000000, 1.000000000000000000, 1.000000000000000000, 1.000000000000000000, 1.000000000000000000, 1.000000000000000000, 1.000000000000000000, 1.000000000000000000, 1.000000000000000000, 1.000000000000000000, 1.000000000000000000, 1.000000000000000000, 1.000000000000000000, 1.000000000000000000, 1.000000000000000000, 1.000000000000000000, 1.000000000000000000, 1.000000000000000000, 1.000000000000000000, 1.000000000000000000, 1.000000000000000000, 1.000000000000000000, 1.000000000000000000, 1.000000000000000000, 1.000000000000000000, 1.000000000000000000, 1.000000000000000000, 1.000000000000000000, 1.000000000000000000, 1.000000000000000000, 1.000000000000000000, 1.000000000000000000, 1.000000000000000000, 1.000000000000000000, 1.000000000000000000, 1.000000000000000000, 1.000000000000000000, 1.000000000000000000, 1.000000000000000000, 1.000000000000000000, 1.000000000000000000, 1.000000000000000000, 1.000000000000000000, 1.000000000000000000, 1.000000000000000000, 1.000000000000000000, 1.000000000000000000, 1.000000000000000000, 1.000000000000000000, 1.000000000000000000, 1.000000000000000000, 1.000000000000000000, 1.000000000000000000, 1.000000000000000000, 1.000000000000000000, 1.000000000000000000, 1.000000000000000000, 1.000000000000000000, 1.000000000000000000, 1.000000000000000000, 1.000000000000000000, 1.000000000000000000, 1.000000000000000000, 1.000000000000000000, 1.000000000000000000, 1.000000000000000000, 1.000000000000000000, 1.000000000000000000, 1.000000000000000000, 1.000000000000000000, 1.000000000000000000, 1.000000000000000000, 1.000000000000000000, 1.000000000000000000, 1.000000000000000000, 1.000000000000000000, 1.000000000000000000, 1.000000000000000000, 1.000000000000000000, 1.000000000000000000, 1.000000000000000000, 1.000000000000000000, 1.000000000000000000, 1.000000000000000000, 1.000000000000000000, 1.000000000000000000, 1.000000000000000000, 1.000000000000000000, 1.000000000000000000, 1.000000000000000000, 1.000000000000000000, 1.000000000000000000, 1.000000000000000000, 1.000000000000000000, 1.000000000000000000, 1.000000000000000000, 1.000000000000000000, 1.000000000000000000, 1.000000000000000000, 1.000000000000000000, 1.000000000000000000, 1.000000000000000000, 1.000000000000000000, 1.000000000000000000, 1.000000000000000000, 1.000000000000000000, 1.000000000000000000, 1.000000000000000000, 1.000000000000000000, 1.000000000000000000, 1.000000000000000000, 1.000000000000000000, 1.000000000000000000, 1.000000000000000000, 1.000000000000000000, 1.000000000000000000, 1.000000000000000000, 1.000000000000000000, 1.000000000000000000, 1.000000000000000000, 1.000000000000000000, 1.000000000000000000, 1.000000000000000000, 1.000000000000000000, 1.000000000000000000, 1.000000000000000000, 1.000000000000000000, 1.000000000000000000, 1.000000000000000000, 1.000000000000000000, 1.000000000000000000, 1.000000000000000000, 1.000000000000000000, 1.000000000000000000, 1.000000000000000000, 1.000000000000000000, 1.000000000000000000, 1.000000000000000000, 1.000000000000000000, 1.000000000000000000, 1.000000000000000000, 1.000000000000000000, 1.000000000000000000, 1.000000000000000000, 1.000000000000000000, 1.000000000000000000, 1.000000000000000000, 1.000000000000000000, 1.000000000000000000, 1.000000000000000000, 1.000000000000000000, 1.000000000000000000, 1.000000000000000000, 1.000000000000000000, 1.000000000000000000, 1.000000000000000000, 1.000000000000000000, 1.000000000000000000, 1.000000000000000000, 1.000000000000000000, 1.000000000000000000, 1.000000000000000000, 1.000000000000000000, 1.000000000000000000, 1.000000000000000000, 1.000000000000000000, 1.000000000000000000, 1.000000000000000000, 1.000000000000000000, 1.000000000000000000, 1.000000000000000000, 1.000000000000000000, 1.000000000000000000, 1.000000000000000000, 1.000000000000000000, 1.000000000000000000, 1.000000000000000000, 1.000000000000000000, 1.000000000000000000, 1.000000000000000000, 1.000000000000000000, 1.000000000000000000, 1.000000000000000000, 1.000000000000000000, 1.000000000000000000, 1.000000000000000000, 1.000000000000000000, 1.000000000000000000, 1.000000000000000000, 1.000000000000000000, 1.000000000000000000, 1.000000000000000000, 1.000000000000000000, 1.000000000000000000, 1.000000000000000000, 1.000000000000000000, 1.000000000000000000, 1.000000000000000000, 1.000000000000000000, 1.000000000000000000, 1.000000000000000000, 1.000000000000000000, 1.000000000000000000, 1.000000000000000000, 1.000000000000000000, 1.000000000000000000, 1.000000000000000000, 1.000000000000000000, 1.000000000000000000, 1.000000000000000000, 1.000000000000000000, 1.000000000000000000, 1.000000000000000000, 1.000000000000000000, 1.000000000000000000, 1.000000000000000000, 1.000000000000000000, 1.000000000000000000, 1.000000000000000000, 1.000000000000000000, 1.000000000000000000, 1.000000000000000000, 1.000000000000000000, 1.000000000000000000, 1.000000000000000000, 1.000000000000000000, 1.000000000000000000, 1.000000000000000000, 1.000000000000000000, 1.000000000000000000, 1.000000000000000000, 1.000000000000000000, 1.000000000000000000, 1.000000000000000000, 1.000000000000000000, 1.000000000000000000, 1.000000000000000000, 1.000000000000000000, 1.000000000000000000, 1.000000000000000000, 1.000000000000000000, 1.000000000000000000, 1.000000000000000000, 1.000000000000000000, 1.000000000000000000, 1.000000000000000000, 1.000000000000000000, 1.000000000000000000, 1.000000000000000000, 1.000000000000000000, 1.000000000000000000, 1.000000000000000000, 1.000000000000000000, 1.000000000000000000, 1.000000000000000000, 1.000000000000000000, 1.000000000000000000, 1.000000000000000000, 1.000000000000000000, 1.000000000000000000, 1.000000000000000000, 1.000000000000000000, 1.000000000000000000, 1.000000000000000000, 1.000000000000000000, 1.000000000000000000, 1.000000000000000000, 1.000000000000000000, 1.000000000000000000, 1.000000000000000000, 1.000000000000000000, 1.000000000000000000, 1.000000000000000000, 1.000000000000000000, 1.000000000000000000, 1.000000000000000000, 1.000000000000000000, 1.000000000000000000, 1.000000000000000000, 1.000000000000000000, 1.000000000000000000, 1.000000000000000000, 1.000000000000000000, 1.000000000000000000, 1.000000000000000000, 1.000000000000000000, 1.000000000000000000, 1.000000000000000000, 1.000000000000000000, 1.000000000000000000, 1.000000000000000000, 1.000000000000000000, 1.000000000000000000, 1.000000000000000000, 1.000000000000000000, 1.000000000000000000, 1.000000000000000000, 1.000000000000000000, 1.000000000000000000, 1.000000000000000000, 1.000000000000000000, 1.000000000000000000, 1.000000000000000000, 1.000000000000000000, 1.000000000000000000, 1.000000000000000000, 1.000000000000000000, 1.000000000000000000, 1.000000000000000000) ) ) 
 REPRESENTATION_ITEM ( '' )  SURFACE ( )  );
#6874=CARTESIAN_POINT ( 'NONE',  ( 5.920964624126254350, -19.79845160325395526, -232.2234910544682123 ) ) ;
#6875=CARTESIAN_POINT ( 'NONE',  ( -27.52457542293397097, 5.447957517019466067, -230.2717933641555135 ) ) ;
#6876=CARTESIAN_POINT ( 'NONE',  ( 10.31623634631035991, 26.83927646318382898, -220.2315638557092541 ) ) ;
#6877=CARTESIAN_POINT ( 'NONE',  ( -9.491065840222427497, 13.31995980477872266, -232.8537120564120073 ) ) ;
#6879=CARTESIAN_POINT ( 'NONE',  ( 24.04182214053767908, -5.779968796880146975, -234.9365023861272164 ) ) ;
#6881=CARTESIAN_POINT ( 'NONE',  ( 22.84140515590350518, 18.29101041979067332, -226.2334522600520472 ) ) ;
#6883=CARTESIAN_POINT ( 'NONE',  ( -11.94727018630768178, 9.025563988971828877, -220.6148682757971358 ) ) ;
#6884=CARTESIAN_POINT ( 'NONE',  ( -13.63002737749749826, 6.315035547785179837, -227.0490028799284516 ) ) ;
#6885=CARTESIAN_POINT ( 'NONE',  ( -12.79488508867961549, -11.10380203712096581, -230.9440799972209106 ) ) ;
#6887=CARTESIAN_POINT ( 'NONE',  ( 29.89309326230132058, 6.052383583152112223, -228.3539431708548477 ) ) ;
#6888=CARTESIAN_POINT ( 'NONE',  ( -24.92290506463145405, 6.124412323591598373, -220.3779252408000104 ) ) ;
#6889=CARTESIAN_POINT ( 'NONE',  ( 13.85207896949186335, 7.847214149978243292, -217.3457543576531066 ) ) ;
#6890=CARTESIAN_POINT ( 'NONE',  ( 21.18605525173251891, 3.426801613781890854, -232.1183243183448894 ) ) ;
#6891=CARTESIAN_POINT ( 'NONE',  ( -9.935407011182972425, -19.19496561732008999, -215.7587022423821850 ) ) ;
#6894=CARTESIAN_POINT ( 'NONE',  ( -9.776740361816679936, -16.43846667899986258, -218.0739489017842061 ) ) ;
#6895=CARTESIAN_POINT ( 'NONE',  ( -5.607934827417612844, 15.68271927908880770, -232.1026723719274969 ) ) ;
#6896=CARTESIAN_POINT ( 'NONE',  ( 14.99336262864975211, -23.54026314425397004, -231.3018640253376361 ) ) ;
#6897=CARTESIAN_POINT ( 'NONE',  ( -9.517741096562200909, 20.63709896626785678, -234.1036702156204967 ) ) ;
#6898=CARTESIAN_POINT ( 'NONE',  ( 10.25809576580632232, -7.052396458808492419, -221.5466685117269208 ) ) ;
#6899=CARTESIAN_POINT ( 'NONE',  ( -23.54665576872953636, -14.78900941482413067, -230.7594827126482073 ) ) ;
#6900=CARTESIAN_POINT ( 'NONE',  ( -20.00523085820573499, 3.356386534894876927, -232.9491364426554298 ) ) ;
#6902=CARTESIAN_POINT ( 'NONE',  ( -3.130917144532865848, 26.01013079854885390, -229.4331404728494874 ) ) ;
#6903=CARTESIAN_POINT ( 'NONE',  ( 20.18206873099720156, 1.748383523995667987, -234.4526011791959661 ) ) ;
#6905=CARTESIAN_POINT ( 'NONE',  ( 21.35706335192880445, 15.67286272432725092, -219.2578158352350783 ) ) ;
#6906=CARTESIAN_POINT ( 'NONE',  ( 25.40172858355122898, 15.07073195964820833, -229.0276483847865450 ) ) ;
#6907=CARTESIAN_POINT ( 'NONE',  ( -3.878264816061211651, -12.95777722686681344, -227.3767537598947683 ) ) ;
#6908=CARTESIAN_POINT ( 'NONE',  ( 2.770531592831002143, 22.28948935999365943, -215.1307751200139649 ) ) ;
#6909=PRODUCT ( 'Frothing Whisk', 'Frothing Whisk', '', ( #14372 ) ) ;
#6910=CARTESIAN_POINT ( 'NONE',  ( 16.00819137755116373, 4.595691552992191120, -229.5669508871464757 ) ) ;
#6911=CARTESIAN_POINT ( 'NONE',  ( 9.903783394593444811, -26.64562852513063973, -229.6560785209296682 ) ) ;
#6912=CARTESIAN_POINT ( 'NONE',  ( -10.40174557315337900, 22.75579539577861965, -231.4492192189165962 ) ) ;
#6913=CARTESIAN_POINT ( 'NONE',  ( 2.579827969572558111, 15.91317371615649101, -219.7652087782269916 ) ) ;
#6915=CARTESIAN_POINT ( 'NONE',  ( -15.58529874627549461, -6.917566422457355202, -219.0138643999995054 ) ) ;
#6916=CARTESIAN_POINT ( 'NONE',  ( -15.19607346356906952, 9.485739149828241068, -229.2407115334993080 ) ) ;
#6918=CARTESIAN_POINT ( 'NONE',  ( 11.75630001506626776, 9.075791953625659048, -230.4239556728226717 ) ) ;
#6920=CARTESIAN_POINT ( 'NONE',  ( 5.623554730548537606, 15.65270319720736225, -231.3185741195121068 ) ) ;
#6921=CARTESIAN_POINT ( 'NONE',  ( 26.62161015268053177, -11.01850213254573951, -223.2145259598937344 ) ) ;
#6922=CARTESIAN_POINT ( 'NONE',  ( 12.31594623278127720, -7.047777776961618557, -228.0736214755532956 ) ) ;
#6924=CARTESIAN_POINT ( 'NONE',  ( 22.46220731426537043, 18.23201731183003460, -227.5436199598787539 ) ) ;
#6925=CARTESIAN_POINT ( 'NONE',  ( -30.11338598929818389, -8.317867968210222784, -227.6364879822423006 ) ) ;
#6926=CARTESIAN_POINT ( 'NONE',  ( -5.636842872076440081, -13.76003991320737541, -219.7405193562604495 ) ) ;
#6927=CARTESIAN_POINT ( 'NONE',  ( 5.982950994121768673, -14.58086824529316594, -231.1438280359330975 ) ) ;
#6928=CARTESIAN_POINT ( 'NONE',  ( -5.706122936196527107, 15.14201253431006045, -228.6865785740211550 ) ) ;
#6930=CARTESIAN_POINT ( 'NONE',  ( 15.04029996350473830, 7.457450192165341107, -220.5007084872782173 ) ) ;
#6931=CARTESIAN_POINT ( 'NONE',  ( -25.29098058636142810, 5.014641116111857144, -217.4658967307323110 ) ) ;
#6932=CARTESIAN_POINT ( 'NONE',  ( -9.060146982536336324, 27.14942986116457746, -225.6568961786626062 ) ) ;
#6933=CARTESIAN_POINT ( 'NONE',  ( 14.41459438711767760, -7.262430563887544821, -219.0449948566021021 ) ) ;
#6936=CARTESIAN_POINT ( 'NONE',  ( -4.080659539198054020, 15.43130099126780408, -228.8058965243247656 ) ) ;
#6937=CARTESIAN_POINT ( 'NONE',  ( -26.35007260221545877, 6.140745174321167177, -221.9336216792591188 ) ) ;
#6938=CARTESIAN_POINT ( 'NONE',  ( 10.85325209735074559, 11.82487774067193342, -216.5214842375702062 ) ) ;
#6939=CARTESIAN_POINT ( 'NONE',  ( 12.94117841657163126, -3.283311917827119064, -226.8844617769393039 ) ) ;
#6942=CARTESIAN_POINT ( 'NONE',  ( -7.189383125363055349, 14.28512618638020548, -231.7475838278701303 ) ) ;
#6943=CARTESIAN_POINT ( 'NONE',  ( -10.57293828068126373, -5.503282544971903611, -227.1466070594375708 ) ) ;
#6945=CARTESIAN_POINT ( 'NONE',  ( 27.75679124201660741, 4.911524026080384075, -221.4430403652340829 ) ) ;
#6946=CARTESIAN_POINT ( 'NONE',  ( -13.98136146596813845, 3.850743984385103680, -228.7620665878280590 ) ) ;
#6947=CARTESIAN_POINT ( 'NONE',  ( 13.82188917133564132, -5.740199443570373816, -227.9076376976435654 ) ) ;
#6949=CARTESIAN_POINT ( 'NONE',  ( -22.11084984981285118, 10.96048252433489623, -216.6117774006995376 ) ) ;
#6951=CARTESIAN_POINT ( 'NONE',  ( -13.92046207272054303, -0.1600067567908077248, -224.5811699126800818 ) ) ;
#6952=CARTESIAN_POINT ( 'NONE',  ( 0.2799207934783670693, -28.72270877262613453, -227.3216717588132667 ) ) ;
#6956=CARTESIAN_POINT ( 'NONE',  ( -29.30406754532526037, 5.063969254119831120, -221.8212091093853076 ) ) ;
#6957=CARTESIAN_POINT ( 'NONE',  ( 16.32467020957917114, -16.75837631771952019, -218.4891864258081853 ) ) ;
#6958=CARTESIAN_POINT ( 'NONE',  ( 13.58381642412367896, -1.690444079054164161, -222.5208797957015747 ) ) ;
#6960=CARTESIAN_POINT ( 'NONE',  ( 10.63406535173453271, 22.16595115341124256, -219.6461356279925781 ) ) ;
#6962=CARTESIAN_POINT ( 'NONE',  ( -11.19105919052231179, 21.17456633634251872, -216.2128528132037957 ) ) ;
#6963=CARTESIAN_POINT ( 'NONE',  ( 15.08139719848974103, 12.15862464477973504, -219.3112749338812080 ) ) ;
#6964=CARTESIAN_POINT ( 'NONE',  ( 5.447232503735224718, -25.66160541809718865, -232.3984543420957323 ) ) ;
#6965=CARTESIAN_POINT ( 'NONE',  ( 24.23593707391374608, -4.329230177290460446, -233.5551557188744312 ) ) ;
#6966=CARTESIAN_POINT ( 'NONE',  ( -9.988594796049140356, 11.34066464990972811, -226.6453149279956563 ) ) ;
#6967=CARTESIAN_POINT ( 'NONE',  ( -15.19607346356906952, 9.485739149828241068, -229.2407115334993080 ) ) ;
#6968=CARTESIAN_POINT ( 'NONE',  ( -17.18633058961025029, 6.481319267413964802, -216.1357216783315494 ) ) ;
#6970=CARTESIAN_POINT ( 'NONE',  ( -3.332878961853828592, -21.58676603248690284, -218.0452238110532619 ) ) ;
#6974=CARTESIAN_POINT ( 'NONE',  ( 17.76485367938521875, 4.373152267827974171, -218.8623009891758215 ) ) ;
#6975=CARTESIAN_POINT ( 'NONE',  ( 14.18740332497314149, -14.20295060558812672, -230.7262566610843351 ) ) ;
#6976=CARTESIAN_POINT ( 'NONE',  ( 4.389496648589924277, 14.47660514356954131, -220.6151178996808540 ) ) ;
#6977=CARTESIAN_POINT ( 'NONE',  ( -13.83274569775339202, 16.20364235096346661, -234.0851861771356539 ) ) ;
#6978=CARTESIAN_POINT ( 'NONE',  ( 14.29548763234129538, 2.320071712424730315, -230.2610858871018422 ) ) ;
#6979=CARTESIAN_POINT ( 'NONE',  ( 5.069241901512100412, 14.34986542013820632, -229.6420000777802954 ) ) ;
#6980=CARTESIAN_POINT ( 'NONE',  ( 25.18785298611088308, 3.974282393449815931, -218.7636041058819956 ) ) ;
#6981=CARTESIAN_POINT ( 'NONE',  ( -5.178973235464019886, -24.35492185057628944, -233.6431870320687381 ) ) ;
#6982=CARTESIAN_POINT ( 'NONE',  ( 13.82188917133564132, -5.740199443570373816, -227.9076376976435654 ) ) ;
#6986=CARTESIAN_POINT ( 'NONE',  ( 28.51464931495100785, 5.422321182929326966, -223.8116416110474347 ) ) ;
#6987=CARTESIAN_POINT ( 'NONE',  ( -10.41267218490845181, -10.94250683577548244, -225.3448144993165556 ) ) ;
#6988=CARTESIAN_POINT ( 'NONE',  ( -20.71192633727912380, 6.339941255257877550, -217.2401662359725094 ) ) ;
#6989=CARTESIAN_POINT ( 'NONE',  ( 3.367418898937407867, 27.20023797116225595, -219.3349021808245709 ) ) ;
#6990=CARTESIAN_POINT ( 'NONE',  ( 2.482746429915354547, 16.41797261123590346, -229.5599230346982154 ) ) ;
#6992=CARTESIAN_POINT ( 'NONE',  ( -25.38303270991942284, -1.762464254583185452, -219.8781034644853776 ) ) ;
#6993=CARTESIAN_POINT ( 'NONE',  ( 10.07175337281514871, 14.76776740066196325, -231.7834566702614723 ) ) ;
#6994=CARTESIAN_POINT ( 'NONE',  ( -19.18087294808806931, 21.32275554655070593, -230.8558978902391061 ) ) ;
#6995=CARTESIAN_POINT ( 'NONE',  ( -16.75232826114664775, 4.232868982398014346, -229.4158550594996200 ) ) ;
#6996=CARTESIAN_POINT ( 'NONE',  ( -17.90134810484358141, -14.13951559615540710, -232.9640066987647344 ) ) ;
#6999=CARTESIAN_POINT ( 'NONE',  ( 25.62718606866737403, 13.33219119508369310, -230.9315691959737933 ) ) ;
#7001=CARTESIAN_POINT ( 'NONE',  ( -11.86888352782322897, 15.29489941890347282, -218.1379771575364259 ) ) ;
#7002=CARTESIAN_POINT ( 'NONE',  ( 17.60070748514786132, 25.68479983175475567, -229.9331108608050158 ) ) ;
#7003=CARTESIAN_POINT ( 'NONE',  ( 27.16757474806794903, 2.676291341565463888, -220.8863403533574115 ) ) ;
#7004=CARTESIAN_POINT ( 'NONE',  ( -27.54101393026537181, -2.112662437277116556, -233.6092940012385384 ) ) ;
#7006=CARTESIAN_POINT ( 'NONE',  ( -22.73457989858237127, -6.881456255901889030, -216.4806380023168799 ) ) ;
#7007=CARTESIAN_POINT ( 'NONE',  ( -10.98447002683091256, 8.146786682930290624, -230.8316952156193338 ) ) ;
#7008=CARTESIAN_POINT ( 'NONE',  ( 1.292981098121811279, -26.53499626907933262, -232.9055005154886828 ) ) ;
#7009=CARTESIAN_POINT ( 'NONE',  ( -8.501641725227710111, 25.47064987787527102, -217.3358698761548737 ) ) ;
#7010=CARTESIAN_POINT ( 'NONE',  ( 13.95236037140391261, -4.360547358326352096, -218.9684814425422132 ) ) ;
#7011=CARTESIAN_POINT ( 'NONE',  ( 15.27183824227296327, -0.1003146413681868659, -228.0000000000005969 ) ) ;
#7012=CARTESIAN_POINT ( 'NONE',  ( 20.18206873099720156, 1.748383523995667987, -234.4526011791959661 ) ) ;
#7014=CARTESIAN_POINT ( 'NONE',  ( -3.926352947695993745, 17.69140300707508473, -220.1607884481205986 ) ) ;
#7015=CARTESIAN_POINT ( 'NONE',  ( 30.47710800431509170, 7.409378661937554789, -223.2007768404241688 ) ) ;
#7016=CARTESIAN_POINT ( 'NONE',  ( 17.60676319847677007, 21.31475060840986302, -219.8266339603936785 ) ) ;
#7017=CARTESIAN_POINT ( 'NONE',  ( 17.23039831256031817, 3.331158952577910615, -216.4027685342793461 ) ) ;
#7018=CARTESIAN_POINT ( 'NONE',  ( -0.1378023845299804762, -12.51091464425689104, -226.1051157421467508 ) ) ;
#7021=CARTESIAN_POINT ( 'NONE',  ( 0.8673818989965740300, 28.69424263383094598, -231.7310846804014659 ) ) ;
#7023=CARTESIAN_POINT ( 'NONE',  ( -10.13139158240655391, -23.04245082364802499, -234.6840773296079874 ) ) ;
#7024=CARTESIAN_POINT ( 'NONE',  ( -10.84440549681320221, 27.00404139634608214, -224.0969657459751261 ) ) ;
#7025=CARTESIAN_POINT ( 'NONE',  ( 16.69977105456987232, 16.51652889326612694, -233.6667933521891030 ) ) ;
#7026=CARTESIAN_POINT ( 'NONE',  ( -14.93108815068229589, -1.792787290847115633, -227.6165763581034582 ) ) ;
#7027=CARTESIAN_POINT ( 'NONE',  ( -16.27736488614644372, 5.941157768540612949, -228.4237983497913547 ) ) ;
#7028=CARTESIAN_POINT ( 'NONE',  ( -15.54392142943450317, 6.670312097614393920, -219.6934017696036676 ) ) ;
#7030=CARTESIAN_POINT ( 'NONE',  ( 16.49791052269847569, 3.745513941566326999, -220.1874559167976884 ) ) ;
#7032=CARTESIAN_POINT ( 'NONE',  ( 12.53674998645855787, 17.96979015029927851, -232.8843215672231679 ) ) ;
#7033=CARTESIAN_POINT ( 'NONE',  ( 9.672299229151310129, -14.28303711772943529, -228.3078296064027484 ) ) ;
#7036=CARTESIAN_POINT ( 'NONE',  ( 13.66858788651615164, -3.112492835348085407, -221.5154270223497690 ) ) ;
#7037=CARTESIAN_POINT ( 'NONE',  ( -8.316066124693966444, 26.67103469786491843, -222.2304303634109885 ) ) ;
#7039=CARTESIAN_POINT ( 'NONE',  ( 10.57926812561479757, 10.00910231482511215, -225.8341706491384286 ) ) ;
#7040=CARTESIAN_POINT ( 'NONE',  ( -11.83854910565153062, -9.589341273415847411, -217.2594489226254098 ) ) ;
#7041=CARTESIAN_POINT ( 'NONE',  ( -5.279374154171231126, -12.28263746854076466, -222.5283095625445640 ) ) ;
#7042=CARTESIAN_POINT ( 'NONE',  ( 14.18709644517307922, -11.45356969546147496, -232.2178450427173004 ) ) ;
#7043=CARTESIAN_POINT ( 'NONE',  ( -0.2748333203896175525, 17.57683079704640505, -221.1444293135629948 ) ) ;
#7045=CARTESIAN_POINT ( 'NONE',  ( 12.56556766396551872, 9.776144415819011613, -223.4791766911294815 ) ) ;
#7046=CARTESIAN_POINT ( 'NONE',  ( -19.00318367631585659, 13.14621133775862916, -233.8403879275295765 ) ) ;
#7047=CARTESIAN_POINT ( 'NONE',  ( -7.770318051073092036, 21.02940971564074957, -231.8751410922876630 ) ) ;
#7048=EDGE_CURVE ( 'NONE', #6170, #4018, #22102, .T. ) ;
#7050=CARTESIAN_POINT ( 'NONE',  ( 7.163080459435270164, 24.05253566895842354, -232.4475987112033408 ) ) ;
#7051=CARTESIAN_POINT ( 'NONE',  ( 17.22423229049764970, 1.395540479540137380, -217.3898520248025363 ) ) ;
#7052=CARTESIAN_POINT ( 'NONE',  ( 12.75306435971521068, 14.56583715532477186, -214.9711136650476533 ) ) ;
#7053=CARTESIAN_POINT ( 'NONE',  ( 5.377793152941013233, -17.45375835550001753, -231.2474386379397231 ) ) ;
#7056=ORIENTED_EDGE ( 'NONE', *, *, #6311, .T. ) ;
#7057=COLOUR_RGB ( '', 0.09019608, 0.27058824, 0.51372549) ;
#7058=CARTESIAN_POINT ( 'NONE',  ( -2.698926868850080041, 12.89339462271858316, -226.7595176699009585 ) ) ;
#7059=CARTESIAN_POINT ( 'NONE',  ( 27.51601410384567359, -3.359424968747257711, -222.6356212526655725 ) ) ;
#7061=CARTESIAN_POINT ( 'NONE',  ( 12.71450444683213021, 7.595266944807587350, -224.4213778964231665 ) ) ;
#7062=CARTESIAN_POINT ( 'NONE',  ( -21.89065952084848021, -0.9940043559354364566, -216.9999999999999716 ) ) ;
#7063=CARTESIAN_POINT ( 'NONE',  ( 6.131461862964278531, -15.14974102410872625, -231.6805438559109973 ) ) ;
#7064=CARTESIAN_POINT ( 'NONE',  ( -10.65455960636934662, 10.37188583052882862, -219.5197110153079620 ) ) ;
#7065=CARTESIAN_POINT ( 'NONE',  ( -20.94800339253696109, 4.477632454355491731, -216.5423208360950298 ) ) ;
#7066=CARTESIAN_POINT ( 'NONE',  ( 0.9095753368782393267, -25.50589708844611891, -231.1945442011520697 ) ) ;
#7068=CARTESIAN_POINT ( 'NONE',  ( 21.31262902390056624, 0.4111834581965390645, -232.0572713672585792 ) ) ;
#7069=CARTESIAN_POINT ( 'NONE',  ( -13.11494368899652052, 3.355507568391938200, -225.9121440085824304 ) ) ;
#7070=CARTESIAN_POINT ( 'NONE',  ( 15.01754996320599744, -10.17932250226635738, -220.3401326760229040 ) ) ;
#7074=CARTESIAN_POINT ( 'NONE',  ( 23.24653631066306048, 11.83805845626388020, -219.6020901153134162 ) ) ;
#7075=CARTESIAN_POINT ( 'NONE',  ( -9.964021556040458805, 12.25789996591640119, -217.8262340283327774 ) ) ;
#7076=CARTESIAN_POINT ( 'NONE',  ( 23.44063276014420794, 13.61134749381700182, -229.1061940987080732 ) ) ;
#7077=CARTESIAN_POINT ( 'NONE',  ( 1.792482182455914064, -21.59191373485632681, -217.1959973011389593 ) ) ;
#7078=CARTESIAN_POINT ( 'NONE',  ( 19.73224149047082321, -2.635265996080750295, -233.5133592171236501 ) ) ;
#7081=CARTESIAN_POINT ( 'NONE',  ( -4.691002462566371101, 21.98518063340150164, -232.2516024630330094 ) ) ;
#7082=CARTESIAN_POINT ( 'NONE',  ( -22.19349712985372491, 11.03542788991621748, -219.7744882786627443 ) ) ;
#7083=CARTESIAN_POINT ( 'NONE',  ( -29.50764134580612463, 7.783340782857166573, -219.9768238800827191 ) ) ;
#7085=CARTESIAN_POINT ( 'NONE',  ( -10.27880337231260199, -13.06498408352235430, -227.3766186522184682 ) ) ;
#7088=CARTESIAN_POINT ( 'NONE',  ( 27.50364976068844669, 3.973406265104437729, -228.8805639113908228 ) ) ;
#7089=CARTESIAN_POINT ( 'NONE',  ( 16.26678737605450564, -16.61684638199339048, -230.8698708339908308 ) ) ;
#7090=CARTESIAN_POINT ( 'NONE',  ( 14.54149994592679107, 8.070685273005897997, -229.7292930672863349 ) ) ;
#7091=CARTESIAN_POINT ( 'NONE',  ( -18.39892766464214446, 25.11039525536027739, -225.3444503920457294 ) ) ;
#7092=EDGE_CURVE ( 'NONE', #3103, #4932, #4125, .T. ) ;
#7093=CARTESIAN_POINT ( 'NONE',  ( 20.96405783751201213, 6.249056650590980588, -215.6254004080763309 ) ) ;
#7095=CARTESIAN_POINT ( 'NONE',  ( 15.12287735332712835, 21.03907941686458116, -231.7894952627153202 ) ) ;
#7096=CARTESIAN_POINT ( 'NONE',  ( 13.39175109400946262, 1.184731213613737566, -222.2403203283322739 ) ) ;
#7098=CARTESIAN_POINT ( 'NONE',  ( 0.5120693878963755719, -30.63998626839889639, -227.9504769009175220 ) ) ;
#7099=CARTESIAN_POINT ( 'NONE',  ( 18.22947608839760747, -6.525328669204546905, -217.7409786913911205 ) ) ;
#7101=CYLINDRICAL_SURFACE ( 'NONE', #15201, 3.000000000000002665 ) ;
#7102=CARTESIAN_POINT ( 'NONE',  ( -23.66836017558062011, 21.44695383684080525, -223.6245772351065568 ) ) ;
#7103=CARTESIAN_POINT ( 'NONE',  ( -15.75487091793989158, -3.404709188850186585, -225.0852311470768825 ) ) ;
#7104=CARTESIAN_POINT ( 'NONE',  ( 13.06430160593375689, 2.561628050526134182, -220.6026188403641299 ) ) ;
#7105=CARTESIAN_POINT ( 'NONE',  ( 2.785859284650920031, 14.19821255961969619, -226.9946081512528906 ) ) ;
#7106=CARTESIAN_POINT ( 'NONE',  ( 0.9879969248128627202, 20.02408072508558945, -218.2055348255049410 ) ) ;
#7108=CARTESIAN_POINT ( 'NONE',  ( -16.27785121718144623, -3.187812258433146084, -227.1052622255949132 ) ) ;
#7109=CARTESIAN_POINT ( 'NONE',  ( 18.06016678184731461, 2.257982981100609354, -218.9983079406065940 ) ) ;
#7110=CARTESIAN_POINT ( 'NONE',  ( -12.30606003331388543, 10.59782772616791036, -231.0021630509705801 ) ) ;
#7111=CARTESIAN_POINT ( 'NONE',  ( -18.91027996815576628, 5.295101183552822555, -231.2253513302548527 ) ) ;
#7112=CARTESIAN_POINT ( 'NONE',  ( -13.29422863469367577, -26.11207831950312652, -226.3284374130324750 ) ) ;
#7113=CARTESIAN_POINT ( 'NONE',  ( -18.71530386740073126, -0.6857509888707814527, -217.6195632122020527 ) ) ;
#7115=CARTESIAN_POINT ( 'NONE',  ( 14.85156906897832485, -2.727936025914895701, -226.2641653400703206 ) ) ;
#7117=CARTESIAN_POINT ( 'NONE',  ( -13.92941769543345032, 11.48925904027772127, -219.8938199480626281 ) ) ;
#7118=CARTESIAN_POINT ( 'NONE',  ( 8.463901354249619757, 8.457277735286822917, -222.5555366599873821 ) ) ;
#7119=CARTESIAN_POINT ( 'NONE',  ( -20.43618815875133521, 1.403378831510147196, -232.9646741665398224 ) ) ;
#7120=CARTESIAN_POINT ( 'NONE',  ( -11.89542047990565266, -6.454581786823162304, -219.2692666839191133 ) ) ;
#7122=CARTESIAN_POINT ( 'NONE',  ( -28.09913862414779473, -9.456046895945956265, -221.0065986266286870 ) ) ;
#7123=CARTESIAN_POINT ( 'NONE',  ( -7.352050649209116884, 10.05454564170545417, -223.7370967983176229 ) ) ;
#7124=CARTESIAN_POINT ( 'NONE',  ( -7.832594822155400927, -23.57318293858060088, -216.4298491688572028 ) ) ;
#7125=CARTESIAN_POINT ( 'NONE',  ( 9.107417252317809186, 16.30291009569977234, -218.0131178633739921 ) ) ;
#7126=CARTESIAN_POINT ( 'NONE',  ( 7.144703960786618957, -9.913249271193393497, -228.5244988832443198 ) ) ;
#7128=CARTESIAN_POINT ( 'NONE',  ( 17.34461553379066601, 6.893916422670210764, -233.3442385185644525 ) ) ;
#7131=CARTESIAN_POINT ( 'NONE',  ( -2.723069588102707606, 15.58614045890443833, -225.0254611642426141 ) ) ;
#7132=CARTESIAN_POINT ( 'NONE',  ( -17.43458823433387650, 2.804998135793385750, -231.8077100320880959 ) ) ;
#7133=CARTESIAN_POINT ( 'NONE',  ( 21.39553407250273054, 8.453402029343234148, -217.9531594780983141 ) ) ;
#7134=CARTESIAN_POINT ( 'NONE',  ( 13.98152565379061052, 2.156981915107639036, -230.5667344709999611 ) ) ;
#7135=CARTESIAN_POINT ( 'NONE',  ( -3.535116539333309049, -19.81104435003528152, -216.2789031305144931 ) ) ;
#7136=CARTESIAN_POINT ( 'NONE',  ( 8.126072675580726212, 14.68573014611672534, -233.8823376361746966 ) ) ;
#7138=CARTESIAN_POINT ( 'NONE',  ( -15.15491452760745439, -27.84330619910961957, -221.4571841043341180 ) ) ;
#7139=CARTESIAN_POINT ( 'NONE',  ( -4.879985665934096772, 15.33285679834440174, -220.9402849574511833 ) ) ;
#7140=CARTESIAN_POINT ( 'NONE',  ( 11.63337745479824292, 8.229076005436313679, -220.5472098800687206 ) ) ;
#7141=CARTESIAN_POINT ( 'NONE',  ( -15.15819830826754355, -2.370657588173597841, -221.8013720140894236 ) ) ;
#7142=CARTESIAN_POINT ( 'NONE',  ( -16.88145396433676027, 5.002512658926777434, -221.2364783498041731 ) ) ;
#7144=CARTESIAN_POINT ( 'NONE',  ( -4.296082356836364191, 12.57880442405704002, -229.5247240216588125 ) ) ;
#7145=CARTESIAN_POINT ( 'NONE',  ( 18.55287065739596031, 7.869864349944380777, -232.8430408253643691 ) ) ;
#7147=CARTESIAN_POINT ( 'NONE',  ( 13.43702744235484303, -16.51261215982735209, -219.1853238157515875 ) ) ;
#7148=CARTESIAN_POINT ( 'NONE',  ( 4.804712767000853368, -14.77773536573586455, -228.5128529893618747 ) ) ;
#7150=CARTESIAN_POINT ( 'NONE',  ( -5.560972518124746244, 14.60655266358653215, -227.5460946431043681 ) ) ;
#7152=CARTESIAN_POINT ( 'NONE',  ( 21.35706335192880445, 15.67286272432725092, -219.2578158352350783 ) ) ;
#7153=CARTESIAN_POINT ( 'NONE',  ( 27.32546652195855685, -7.354568365469916991, -229.0866163655393279 ) ) ;
#7154=CARTESIAN_POINT ( 'NONE',  ( -13.21314811618155716, -9.038438575223175064, -230.6430079410957603 ) ) ;
#7155=CARTESIAN_POINT ( 'NONE',  ( -1.778254167844783851, -12.78790610364390012, -225.9413532495922254 ) ) ;
#7156=CARTESIAN_POINT ( 'NONE',  ( -2.906906946766868227, 27.66682465340607422, -226.6559963821499082 ) ) ;
#7158=CARTESIAN_POINT ( 'NONE',  ( 14.03916608299427082, 11.26328028684000415, -220.2447382113059007 ) ) ;
#7159=CARTESIAN_POINT ( 'NONE',  ( -11.69688825528096388, 18.63404371591177622, -215.8612738028812714 ) ) ;
#7160=CARTESIAN_POINT ( 'NONE',  ( -16.90193019167508126, 18.45790510038867893, -217.5707532411249758 ) ) ;
#7161=CARTESIAN_POINT ( 'NONE',  ( 4.303123380281038024, 17.66787810618728827, -231.9745698734655832 ) ) ;
#7162=CARTESIAN_POINT ( 'NONE',  ( -18.46822229429615447, 3.027586163204024405, -230.1002726880134333 ) ) ;
#7163=CARTESIAN_POINT ( 'NONE',  ( 6.812728368504421539, 14.35307019806973194, -216.7766581591129977 ) ) ;
#7165=CARTESIAN_POINT ( 'NONE',  ( 12.70013114424463296, -16.94540864491495924, -217.3462533088837745 ) ) ;
#7169=CARTESIAN_POINT ( 'NONE',  ( -8.823862513872974489, 14.92351368520778898, -217.1499513473673346 ) ) ;
#7170=CARTESIAN_POINT ( 'NONE',  ( -32.13037437807204810, -1.025156162654832670, -224.7589498746283141 ) ) ;
#7171=CARTESIAN_POINT ( 'NONE',  ( 17.00614511541963836, -1.958782916976874233, -219.4638360731791806 ) ) ;
#7172=CARTESIAN_POINT ( 'NONE',  ( 23.49048926389013658, 9.645778135078892035, -218.7307869890797463 ) ) ;
#7173=CARTESIAN_POINT ( 'NONE',  ( -15.23434562258889891, -0.4010941804143903222, -220.4743703065900036 ) ) ;
#7174=CARTESIAN_POINT ( 'NONE',  ( 14.99336262864975211, -23.54026314425397004, -231.3018640253376361 ) ) ;
#7176=CARTESIAN_POINT ( 'NONE',  ( -10.24288955603410933, 28.30762631303078791, -220.8855665231519083 ) ) ;
#7177=CARTESIAN_POINT ( 'NONE',  ( -17.20794623181132721, 21.97849129791581291, -217.9187454682870850 ) ) ;
#7179=CARTESIAN_POINT ( 'NONE',  ( -26.02440924314744919, 2.824604386891162111, -232.0644005296583430 ) ) ;
#7180=CARTESIAN_POINT ( 'NONE',  ( -14.34029329777712469, -14.57793623142476669, -217.2545494607695389 ) ) ;
#7183=CARTESIAN_POINT ( 'NONE',  ( -20.94800339253696109, 4.477632454355491731, -216.5423208360950298 ) ) ;
#7184=CARTESIAN_POINT ( 'NONE',  ( 3.489817674839083228, -23.52381883976217836, -233.5393804659674117 ) ) ;
#7186=CARTESIAN_POINT ( 'NONE',  ( 14.72648027392381387, 10.15511732729369676, -229.5776536674053716 ) ) ;
#7187=CARTESIAN_POINT ( 'NONE',  ( -16.38161496430853248, 17.22219235543852989, -215.3343469598664797 ) ) ;
#7188=CARTESIAN_POINT ( 'NONE',  ( 22.03647168421188596, 0.3315607655626346961, -232.0572713672587213 ) ) ;
#7189=CARTESIAN_POINT ( 'NONE',  ( 14.03916608299427082, 11.26328028684000415, -220.2447382113059007 ) ) ;
#7190=CARTESIAN_POINT ( 'NONE',  ( 3.550474435626596037, -26.82390172985419952, -218.7255222707324549 ) ) ;
#7191=CARTESIAN_POINT ( 'NONE',  ( 14.01369322398082851, -0.3099216430074364093, -221.6784101578248283 ) ) ;
#7193=CARTESIAN_POINT ( 'NONE',  ( -5.775873073292457249, 17.47547275616994256, -218.7209647771908578 ) ) ;
#7194=CARTESIAN_POINT ( 'NONE',  ( -21.99356461413155728, 5.827088221545293045, -219.1725956997024127 ) ) ;
#7195=CARTESIAN_POINT ( 'NONE',  ( 16.55609572527610851, 2.729108819536508967, -230.5704679660131831 ) ) ;
#7197=CARTESIAN_POINT ( 'NONE',  ( -18.43493186415240714, -20.29552032882516244, -227.2236339120829030 ) ) ;
#7200=CARTESIAN_POINT ( 'NONE',  ( 18.78616100366561881, 3.045752412654093355, -231.5393376370170699 ) ) ;
#7201=CARTESIAN_POINT ( 'NONE',  ( 8.483411394722875087, -26.22410139474833457, -227.7697325675642617 ) ) ;
#7202=CARTESIAN_POINT ( 'NONE',  ( 16.38151749656409351, 8.902090001712490874, -231.2955017965201989 ) ) ;
#7203=CARTESIAN_POINT ( 'NONE',  ( -8.823862513872974489, 14.92351368520778898, -217.1499513473673346 ) ) ;
#7204=CARTESIAN_POINT ( 'NONE',  ( 29.33969601628096768, 11.98971187598327504, -225.2039690377576733 ) ) ;
#7206=CARTESIAN_POINT ( 'NONE',  ( 9.107417252317809186, 16.30291009569977234, -218.0131178633739921 ) ) ;
#7208=CARTESIAN_POINT ( 'NONE',  ( -10.11868820210310282, -13.51996935893276053, -218.1704188629865371 ) ) ;
#7209=CARTESIAN_POINT ( 'NONE',  ( 12.70477135646371281, -9.814387909761604689, -230.3443492180780652 ) ) ;
#7212=CARTESIAN_POINT ( 'NONE',  ( -27.53108621362071773, 14.15137273650544536, -219.7961709676081625 ) ) ;
#7213=CARTESIAN_POINT ( 'NONE',  ( 22.16968511661848495, 1.542591969257128826, -234.6098499860488857 ) ) ;
#7214=EDGE_CURVE ( 'NONE', #161, #7856, #14609, .T. ) ;
#7215=CARTESIAN_POINT ( 'NONE',  ( 28.53243699394185384, 6.329221954355706004, -218.6437889135959267 ) ) ;
#7216=CARTESIAN_POINT ( 'NONE',  ( 5.702651035983461902, 12.42242820409033222, -224.7304266323218656 ) ) ;
#7217=CARTESIAN_POINT ( 'NONE',  ( 5.365126951644291431, 19.60085171667039816, -218.9155869426879519 ) ) ;
#7219=CARTESIAN_POINT ( 'NONE',  ( 9.772444363920737231, -9.146208674228628155, -219.7841758423534486 ) ) ;
#7221=CARTESIAN_POINT ( 'NONE',  ( 14.98418162551161714, 4.450317369940187895, -227.9894155827521161 ) ) ;
#7222=CARTESIAN_POINT ( 'NONE',  ( -14.95675039876920032, 11.42095949000369259, -217.2220932760075129 ) ) ;
#7223=CARTESIAN_POINT ( 'NONE',  ( -10.95054816480499760, 8.339404316518379545, -224.1596700080921778 ) ) ;
#7224=CARTESIAN_POINT ( 'NONE',  ( -14.80115690555879659, -8.758261077448048937, -218.2925738755452016 ) ) ;
#7225=CARTESIAN_POINT ( 'NONE',  ( -15.58461825850822180, 18.91734573546571951, -233.7691177939990723 ) ) ;
#7228=CARTESIAN_POINT ( 'NONE',  ( 13.19406830060760605, 4.163358546877222288, -228.8532745215267425 ) ) ;
#7229=CARTESIAN_POINT ( 'NONE',  ( -12.33583941212908108, 22.27382123621224608, -231.6290720151527296 ) ) ;
#7230=CARTESIAN_POINT ( 'NONE',  ( 19.13589083395335422, 16.69125564174534659, -234.7442498487877174 ) ) ;
#7231=CARTESIAN_POINT ( 'NONE',  ( -13.65925618638770800, 3.289586759644148817, -222.1579143493116533 ) ) ;
#7232=CARTESIAN_POINT ( 'NONE',  ( -14.04855893775563125, -7.839533416607601168, -216.6740050463540115 ) ) ;
#7233=CARTESIAN_POINT ( 'NONE',  ( -30.71739798481564421, -2.702902032605977389, -225.9472362185736642 ) ) ;
#7234=CARTESIAN_POINT ( 'NONE',  ( -17.81561310496929806, 18.25637658208611569, -215.7745954696244439 ) ) ;
#7235=CARTESIAN_POINT ( 'NONE',  ( -8.257247207528708444, -26.39349301559143512, -217.9383130379005138 ) ) ;
#7236=CARTESIAN_POINT ( 'NONE',  ( 8.329997790135040603, 12.51216704542961899, -228.7022893680961602 ) ) ;
#7237=CARTESIAN_POINT ( 'NONE',  ( 12.91141610427636621, -26.43280511468161720, -217.7946055251781274 ) ) ;
#7239=CARTESIAN_POINT ( 'NONE',  ( -20.71192633727912380, 6.339941255257877550, -217.2401662359725094 ) ) ;
#7241=CARTESIAN_POINT ( 'NONE',  ( 1.455106383990497187, 21.12056149333958999, -230.8076663600630241 ) ) ;
#7242=CARTESIAN_POINT ( 'NONE',  ( -22.10934047915427314, 0.9940043559354312386, -216.9999999999999716 ) ) ;
#7243=CARTESIAN_POINT ( 'NONE',  ( 25.33562512631297281, 12.25422971834577268, -228.6777356031426791 ) ) ;
#7244=CARTESIAN_POINT ( 'NONE',  ( 11.54460987479198053, 9.649171130674412566, -228.7280371210653698 ) ) ;
#7245=CARTESIAN_POINT ( 'NONE',  ( -9.447593206125553422, -28.82180577676834332, -226.7547558591687675 ) ) ;
#7246=CARTESIAN_POINT ( 'NONE',  ( 8.036750260989780514, 26.29729070384984624, -233.5018314387838529 ) ) ;
#7248=CARTESIAN_POINT ( 'NONE',  ( -4.912481909026474192, -29.12074637257241250, -231.0965163926508410 ) ) ;
#7249=CARTESIAN_POINT ( 'NONE',  ( -4.067324790461362305, 15.10342260507846746, -228.2464404076259257 ) ) ;
#7250=CARTESIAN_POINT ( 'NONE',  ( 16.55626903245587656, 22.80423546114836952, -218.9884947126587633 ) ) ;
#7251=CARTESIAN_POINT ( 'NONE',  ( -13.58070052954164275, 11.19572749768420650, -220.2511552028196604 ) ) ;
#7252=CARTESIAN_POINT ( 'NONE',  ( -7.403072389817287657, 18.92851032520892929, -215.2068968469505137 ) ) ;
#7253=CARTESIAN_POINT ( 'NONE',  ( 16.56146809408446430, -0.9616313295950813522, -228.5729530379900609 ) ) ;
#7255=CARTESIAN_POINT ( 'NONE',  ( 9.923626285694149729, -13.24753681723166210, -222.8613851586638361 ) ) ;
#7257=CARTESIAN_POINT ( 'NONE',  ( 9.759123193367146953, -21.89695672029116480, -217.8292787338521919 ) ) ;
#7258=CARTESIAN_POINT ( 'NONE',  ( -7.366083718505351818, 19.86648438590005838, -231.8662444779758971 ) ) ;
#7262=CARTESIAN_POINT ( 'NONE',  ( 17.43816562714825125, 15.15720016074785903, -232.3748236813696906 ) ) ;
#7263=CARTESIAN_POINT ( 'NONE',  ( 27.36047156164216787, -8.591464759722228450, -221.3690063136810977 ) ) ;
#7264=CARTESIAN_POINT ( 'NONE',  ( -12.04756914620937636, -13.80987496524771885, -232.8991007102355582 ) ) ;
#7265=CARTESIAN_POINT ( 'NONE',  ( 4.682724365302521896, -22.35092628325669750, -215.9543778044225348 ) ) ;
#7266=CARTESIAN_POINT ( 'NONE',  ( 0.6289891638115701067, 16.47510600144228832, -227.0521699048171342 ) ) ;
#7268=CARTESIAN_POINT ( 'NONE',  ( 12.51085646230496273, 9.582567546749562126, -224.6200301875240939 ) ) ;
#7270=CARTESIAN_POINT ( 'NONE',  ( -2.817219543927646175, 14.13981714106644993, -229.6779615865167443 ) ) ;
#7271=CARTESIAN_POINT ( 'NONE',  ( -13.30451247859013897, 19.85560227862636040, -232.3493821534129609 ) ) ;
#7274=CARTESIAN_POINT ( 'NONE',  ( 3.080453011304693511, 29.32691491905673331, -222.8956499783474499 ) ) ;
#7275=CARTESIAN_POINT ( 'NONE',  ( -16.04492519386327487, 1.819644280589142626, -223.4665098021627614 ) ) ;
#7276=CARTESIAN_POINT ( 'NONE',  ( 22.17049319811867036, 0.5483778423327810847, -216.5715983009590673 ) ) ;
#7277=CARTESIAN_POINT ( 'NONE',  ( 6.203932113039332563, -21.09630782756332223, -232.3325312104709894 ) ) ;
#7278=CARTESIAN_POINT ( 'NONE',  ( 17.57135037026572277, 0.09191994211922807634, -232.8447871904542410 ) ) ;
#7280=CARTESIAN_POINT ( 'NONE',  ( 4.603870848087811218, 30.13529352683433515, -225.9623629403671430 ) ) ;
#7281=CARTESIAN_POINT ( 'NONE',  ( 17.02517607141322031, -4.660589389729973497, -229.0519452290894833 ) ) ;
#7284=CARTESIAN_POINT ( 'NONE',  ( 16.64225601860865211, 1.926018578292457928, -220.2177910260893725 ) ) ;
#7285=CARTESIAN_POINT ( 'NONE',  ( 2.098184199980985376, -13.29281380427311099, -222.1652846463370281 ) ) ;
#7287=CARTESIAN_POINT ( 'NONE',  ( -22.04257564474043818, 18.72061943465525857, -219.1781831295219263 ) ) ;
#7288=CARTESIAN_POINT ( 'NONE',  ( -8.995433708001568718, 13.44373928221519243, -231.9251680978426577 ) ) ;
#7289=CARTESIAN_POINT ( 'NONE',  ( -18.71530386740073126, -0.6857509888707814527, -217.6195632122020527 ) ) ;
#7290=CARTESIAN_POINT ( 'NONE',  ( -14.80115690555879659, -8.758261077448048937, -218.2925738755452016 ) ) ;
#7293=CARTESIAN_POINT ( 'NONE',  ( -28.59157645096996347, 5.137867505054540374, -220.4667042235044505 ) ) ;
#7294=CARTESIAN_POINT ( 'NONE',  ( 4.343570314325058135, -14.31236505836544026, -220.3716640818165615 ) ) ;
#7298=CARTESIAN_POINT ( 'NONE',  ( 24.38255093784924199, 7.851200578213498815, -231.2687759850219607 ) ) ;
#7299=CARTESIAN_POINT ( 'NONE',  ( -6.331039912586185814, 17.62337457105953220, -233.2305561356360499 ) ) ;
#7301=CARTESIAN_POINT ( 'NONE',  ( 11.05872493453861161, 12.09300746323778775, -226.7727269015348952 ) ) ;
#7302=CARTESIAN_POINT ( 'NONE',  ( 0.2144678239183100965, -16.00554277676860693, -220.6792656679080267 ) ) ;
#7304=CARTESIAN_POINT ( 'NONE',  ( -0.1881941282075867139, 17.37563936270229092, -230.9177995227891813 ) ) ;
#7305=CARTESIAN_POINT ( 'NONE',  ( -9.523248388595575875, 12.31121908620753125, -221.6288572946744182 ) ) ;
#7306=CARTESIAN_POINT ( 'NONE',  ( -12.88152464663890306, 6.317716727793897924, -230.5294309895745073 ) ) ;
#7307=CARTESIAN_POINT ( 'NONE',  ( -13.72210242120180901, -11.34614737046836908, -229.0742334187831659 ) ) ;
#7310=CARTESIAN_POINT ( 'NONE',  ( 19.87150736056128864, 8.436445599727830924, -233.0166429845654932 ) ) ;
#7311=CARTESIAN_POINT ( 'NONE',  ( 6.900253619295916963, -14.54306101932516881, -223.7596260804713211 ) ) ;
#7312=CARTESIAN_POINT ( 'NONE',  ( 24.42567939027770407, 10.22651298688739097, -219.4562066833365748 ) ) ;
#7313=CARTESIAN_POINT ( 'NONE',  ( -9.749377714296398878, 10.28442384816749922, -229.3722863967025205 ) ) ;
#7316=CARTESIAN_POINT ( 'NONE',  ( 12.48419387172699579, 6.663456953110941328, -219.2717027540951165 ) ) ;
#7317=CARTESIAN_POINT ( 'NONE',  ( 4.543450689403089271, 15.91052110650461771, -218.9437823786444426 ) ) ;
#7319=CARTESIAN_POINT ( 'NONE',  ( -5.902479482706956659, -14.78727544128710214, -218.5565286504736946 ) ) ;
#7320=CARTESIAN_POINT ( 'NONE',  ( 13.62757736989142465, -5.584028114184929947, -227.2616851496390211 ) ) ;
#7324=CARTESIAN_POINT ( 'NONE',  ( -21.50655177804914686, 20.61731362457859973, -218.7935603611527426 ) ) ;
#7325=CARTESIAN_POINT ( 'NONE',  ( -24.13290183362846264, -6.995619630784887022, -220.0347092962472288 ) ) ;
#7328=CARTESIAN_POINT ( 'NONE',  ( -13.88743542672353826, 10.36310385030668613, -230.6144170796622745 ) ) ;
#7329=CARTESIAN_POINT ( 'NONE',  ( 11.09231067055629616, 7.417581979752235100, -227.5152062457793534 ) ) ;
#7330=CARTESIAN_POINT ( 'NONE',  ( -1.268862717067444024, 15.25222216985846480, -229.0661283592426116 ) ) ;
#7332=CARTESIAN_POINT ( 'NONE',  ( 11.85708236628466672, -10.49065743416967145, -217.1712987709648530 ) ) ;
#7334=CARTESIAN_POINT ( 'NONE',  ( 21.60524407607017849, 3.028118258437591415, -217.8361640396714449 ) ) ;
#7336=CARTESIAN_POINT ( 'NONE',  ( -19.58639255110637478, 14.91076398872931819, -217.1105532241463720 ) ) ;
#7337=CARTESIAN_POINT ( 'NONE',  ( -11.27928845652762213, 14.86256579634383002, -216.2427993537644966 ) ) ;
#7338=CARTESIAN_POINT ( 'NONE',  ( -24.95227886253013239, -16.82584358170602101, -223.8363818545792299 ) ) ;
#7339=CARTESIAN_POINT ( 'NONE',  ( -14.00380962569832199, 8.747390586476997854, -231.7950903513155936 ) ) ;
#7341=CARTESIAN_POINT ( 'NONE',  ( 29.11492790716816614, 6.132849117128307270, -229.8316941169402412 ) ) ;
#7343=CARTESIAN_POINT ( 'NONE',  ( -12.14452111807825041, 26.21581784948545035, -221.1455569020914140 ) ) ;
#7344=CARTESIAN_POINT ( 'NONE',  ( 23.07558131619435571, 16.33594519118144817, -217.0553921114837124 ) ) ;
#7345=CARTESIAN_POINT ( 'NONE',  ( 17.47660375112063491, 0.1533180678384444551, -220.6249646429494931 ) ) ;
#7346=B_SPLINE_CURVE_WITH_KNOTS ( 'NONE', 3,
 ( #15023, #18506, #6343, #7113, #1284, #20817, #21973, #3602, #6452, #11522, #1170, #18284, #9956, #20279, #2955, #16815, #15251, #4874, #1921, #8802, #1391, #9843, #16589, #11753, #16704, #8158, #8381, #14914, #21753, #15663, #13216, #18619, #13322, #20163, #4756, #10064, #16928, #6686, #20393, #5289, #12168, #244, #5735, #3711, #17796, #7665, #5632, #15884, #2142, #19459, #3938, #12509, #2362, #5517, #9352, #462, #9020, #19572, #19356, #3827, #10813, #7447, #17681, #14090, #9132, #2252, #4048, #15778, #7339, #9246, #14535, #17573, #12396, #14206, #16212, #17906, #4159, #10924, #21370, #17463, #15995, #2470, #19247, #19131, #10594, #14421, #16106, #2033, #678, #21042, #8912, #571, #14315, #21147, #784, #12279, #7553, #358, #12614, #7225, #21254, #12726, #5846, #11040, #20930, #10709, #4599, #4268, #1235, #13168, #1347, #6178, #1011, #11583, #16768, #3020, #2692, #13275, #6294, #18238, #11146, #2904, #1119, #18457, #20118, #21589, #15090, #13057, #4706, #899, #12838, #19902, #19682, #18014, #9905, #6071, #16654, #9789, #11255, #11476, #2580, #5961, #20013, #8218, #16437, #11369, #2799, #8109, #9463, #16323, #21477, #7995, #21816, #19788, #7777, #14975, #7886, #14646, #12943, #9574, #18343, #18125, #4371, #4490, #14748, #9681, #16540, #14860, #6405, #21703, #4824, #3135, #10016, #18681, #18788, #8446, #17212, #8780, #12146, #6516, #105, #13847, #13728, #1895, #11701, #20457, #15199, #6860, #13619, #10239, #10458, #6976, #16992, #18571, #5156, #3581, #20342, #13385, #21926, #22045, #15422, #18897, #17319, #5045, #1455, #15315, #16880, #6634, #8328, #4938, #20229, #19002, #20568, #12036, #16407, #15522, #1574, #13505, #11814, #3243, #8558, #20684, #10127, #11922, #3471, #22162, #3356, #6751, #17105, #1684, #10349, #1786, #8661, #5266, #12701, #7424, #14293, #15973, #9222, #10688, #5373, #19224, #2225, #547, #15755, #12488, #19108, #5490, #3685, #19335, #12257, #13957, #5822, #12374, #15861, #10570, #4137, #20904, #17884, #3915, #16085, #11016, #19547, #3804, #654, #21126, #5607, #20793, #2446, #15641, #14068, #14400, #17552, #21232, #334, #7090, #17658, #2119, #7202, #5714, #17440, #7532, #8998, #4021, #19436, #438, #12591, #2009, #8891, #7312, #221, #14183, #21020, #10791, #9106, #10897, #17772, #2338, #4679, #2664, #12918, #21788, #6266, #11228, #14950, #18426, #19764, #14831, #4344, #18097, #9548, #6375, #13026, #13247, #4459, #16409, #11122, #6151, #985, #16514, #12813, #19873, #7859, #4573, #9329, #20092, #16189, #9759 ),
 .UNSPECIFIED., .F., .F.,
 ( 4, 2, 2, 2, 2, 2, 2, 2, 2, 2, 2, 2, 2, 2, 2, 2, 2, 2, 2, 2, 2, 2, 2, 2, 2, 2, 2, 2, 2, 2, 2, 2, 2, 2, 2, 2, 2, 2, 2, 2, 2, 2, 2, 2, 2, 2, 2, 2, 2, 2, 2, 2, 2, 2, 2, 2, 2, 2, 2, 2, 2, 2, 2, 2, 2, 2, 2, 2, 2, 2, 2, 2, 2, 2, 2, 2, 2, 2, 2, 2, 2, 2, 2, 2, 2, 2, 2, 2, 2, 2, 2, 2, 2, 2, 2, 2, 2, 2, 2, 2, 2, 2, 2, 2, 2, 2, 2, 2, 2, 2, 2, 2, 2, 2, 2, 2, 2, 2, 2, 2, 2, 2, 2, 2, 2, 2, 2, 2, 2, 2, 2, 2, 2, 2, 2, 2, 2, 2, 2, 2, 2, 2, 2, 2, 2, 2, 2, 2, 2, 2, 2, 2, 2, 2, 2, 2, 2, 2, 2, 2, 2, 2, 2, 4 ),
 ( 0.000000000000000000, 0.001952908952989333875, 0.003905817905978667751, 0.007323408573709997045, 0.01074099924144132634, 0.01415858990917265650, 0.01586738524303832332, 0.01757618057690398666, 0.02099377124463531682, 0.02441136191236664699, 0.02782895258009797368, 0.03124654324782930384, 0.03466413391556063400, 0.03808172458329196070, 0.04149931525102329433, 0.04491690591875462102, 0.04662570125262028436, 0.04833449658648594771, 0.05175208725421727440, 0.05346088258808293775, 0.05516967792194860110, 0.05858726858967993473, 0.06200485925741126836, 0.06542244992514259505, 0.06884004059287393562, 0.07225763126060526231, 0.07567522192833658901, 0.07909281259606792958, 0.08251040326379925627, 0.08421919859766491268, 0.08592799393153058296, 0.08934558459926195129, 0.09276317526699331961, 0.09447197060085900377, 0.09618076593472468794, 0.09959835660245604239, 0.1030159472701873968, 0.1064335379379187652, 0.1098511286056501335, 0.1132687192733815018, 0.1166863099411127869, 0.1201039006088440858, 0.1235214912765753847, 0.1252302866104410273, 0.1269390819443066698, 0.1303566726120379826, 0.1320654679459036251, 0.1337742632797692399, 0.1371918539475005527, 0.1406094446152318378, 0.1440270352829631784, 0.1474446259506944912, 0.1508622166184258040, 0.1542798072861571446, 0.1576973979538884851, 0.1611149886216198257, 0.1645325792893511663, 0.1679501699570824791, 0.1713677606248137919, 0.1747853512925451325, 0.1764941466264108028, 0.1782029419602764730, 0.1816205326280078136, 0.1850381232957391542, 0.1884557139634704670, 0.1918733046312017798, 0.1952908952989331204, 0.1987084859666644887, 0.2021260766343957738, 0.2055436673021270866, 0.2072524626359927569, 0.2089612579698584272, 0.2123788486375897677, 0.2140876439714554380, 0.2157964393053211083, 0.2192140299730524489, 0.2226316206407837617, 0.2260492113085151300, 0.2294668019762464706, 0.2328843926439778111, 0.2363019833117091517, 0.2397195739794404923, 0.2431371646471718329, 0.2465547553149031734, 0.2499723459826345140, 0.2533899366503657991, 0.2568075273180971396, 0.2602251179858284802, 0.2636427086535597653, 0.2670602993212910503, 0.2704778899890223909, 0.2738954806567537315, 0.2773130713244850165, 0.2807306619922163571, 0.2841482526599476977, 0.2858570479938133402, 0.2875658433276790382, 0.2909834339954103788, 0.2926922293292760768, 0.2944010246631417194, 0.2978186153308730599, 0.3012362059986043450, 0.3046537966663356856, 0.3080713873340670261, 0.3114889780017983112, 0.3149065686695296518, 0.3183241593372609368, 0.3217417500049923329, 0.3234505453388579754, 0.3251593406727236735, 0.3285769313404549585, 0.3319945220081862991, 0.3354121126759176397, 0.3388297033436489247, 0.3422472940113802653, 0.3456648846791116059, 0.3490824753468429464, 0.3525000660145742870, 0.3559176566823056276, 0.3593352473500369682, 0.3627528380177683087, 0.3661704286854996493, 0.3695880193532309343, 0.3730056100209622749, 0.3747144053548279174, 0.3764232006886936155, 0.3798407913564249005, 0.3832583820241562411, 0.3866759726918875817, 0.3900935633596189223, 0.3935111540273502628, 0.3969287446950816034, 0.4003463353628129440, 0.4037639260305442845, 0.4054727213644099271, 0.4071815166982756251, 0.4105991073660069102, 0.4140166980337382507, 0.4157254933676038933, 0.4174342887014695913, 0.4208518793692008764, 0.4242694700369322169, 0.4276870607046635575, 0.4311046513723948981, 0.4345222420401262386, 0.4379398327078575237, 0.4413574233755888643, 0.4447750140433202048, 0.4464838093771859029, 0.4481926047110515454, 0.4516101953787828860, 0.4533189907126486395, 0.4550277860465142266, 0.4584453767142455671, 0.4618629673819769077, 0.4652805580497082483, 0.4686981487174395888, 0.4721157393851709294, 0.4755333300529022145, 0.4789509207206335550, 0.4823685113883648956, 0.4840773067222305381, 0.4857861020560962362, 0.4875580825543344710 ),
 .UNSPECIFIED. ) ;
#7347=CARTESIAN_POINT ( 'NONE',  ( -17.90134810484358141, -14.13951559615540710, -232.9640066987647344 ) ) ;
#7348=CARTESIAN_POINT ( 'NONE',  ( 1.430961520682887400, 16.89318350835024063, -220.3256763723340157 ) ) ;
#7349=CARTESIAN_POINT ( 'NONE',  ( -1.177898122437396333, -26.14463525305933445, -216.8677949074964033 ) ) ;
#7350=CARTESIAN_POINT ( 'NONE',  ( 8.979547488457603421, 23.24376652602565230, -232.6628827740196357 ) ) ;
#7351=CARTESIAN_POINT ( 'NONE',  ( 7.292867580403318506, -17.79718201325288263, -215.1213547356373397 ) ) ;
#7353=CARTESIAN_POINT ( 'NONE',  ( 30.47710800431509170, 7.409378661937554789, -223.2007768404241688 ) ) ;
#7355=CARTESIAN_POINT ( 'NONE',  ( 13.66858788651615164, -3.112492835348085407, -221.5154270223497690 ) ) ;
#7356=CARTESIAN_POINT ( 'NONE',  ( 3.325336547283623378, 18.92213121405483633, -219.7480163085221818 ) ) ;
#7357=CARTESIAN_POINT ( 'NONE',  ( 30.55431851955342282, 7.682798326916945975, -224.9061577511691610 ) ) ;
#7358=CARTESIAN_POINT ( 'NONE',  ( 16.64225601860865211, 1.926018578292457928, -220.2177910260893725 ) ) ;
#7359=CARTESIAN_POINT ( 'NONE',  ( -10.41267218490845181, -10.94250683577548244, -225.3448144993165556 ) ) ;
#7360=CARTESIAN_POINT ( 'NONE',  ( 3.137667653003819446, 15.44806861187908176, -232.6841782316817842 ) ) ;
#7363=CARTESIAN_POINT ( 'NONE',  ( -7.625346832407194242, -11.41809035428902064, -218.7189489878062716 ) ) ;
#7364=CARTESIAN_POINT ( 'NONE',  ( -15.51982305277792307, 19.76957551617798359, -231.4018974401358832 ) ) ;
#7365=CARTESIAN_POINT ( 'NONE',  ( 13.48097272627202159, 8.509510470709432894, -231.5257201610278059 ) ) ;
#7366=CARTESIAN_POINT ( 'NONE',  ( -13.92941769543345032, 11.48925904027772127, -219.8938199480626281 ) ) ;
#7368=CARTESIAN_POINT ( 'NONE',  ( -2.577721557973523314, 25.83760098923793791, -215.4660676095525389 ) ) ;
#7369=CARTESIAN_POINT ( 'NONE',  ( 25.85597688020959239, 3.954559836939000039, -230.6766427064781624 ) ) ;
#7370=CARTESIAN_POINT ( 'NONE',  ( 12.24130115618514125, -19.65891960071846967, -230.7381047918825914 ) ) ;
#7372=CARTESIAN_POINT ( 'NONE',  ( 16.43596176044053081, -17.06621466254232544, -232.8418678805942648 ) ) ;
#7374=CARTESIAN_POINT ( 'NONE',  ( -7.058999618647554541, 24.62458660126260312, -219.6630466582859356 ) ) ;
#7377=CARTESIAN_POINT ( 'NONE',  ( 11.33210854356620523, 22.81476816607802149, -217.8536224460118262 ) ) ;
#7378=CARTESIAN_POINT ( 'NONE',  ( -17.70471257751854921, -0.5540196600081067624, -232.9322037287452360 ) ) ;
#7379=CARTESIAN_POINT ( 'NONE',  ( -11.39823187951283501, -7.998194509987097689, -226.8062974464413912 ) ) ;
#7380=CARTESIAN_POINT ( 'NONE',  ( -8.258403559667634397, -29.80786866836635696, -223.3983869762195127 ) ) ;
#7381=CARTESIAN_POINT ( 'NONE',  ( -3.071946796551161984, 23.17078151772539485, -231.0066194318698933 ) ) ;
#7383=CARTESIAN_POINT ( 'NONE',  ( 18.30590144060498403, 15.06309558287673767, -219.0459394567220102 ) ) ;
#7384=CARTESIAN_POINT ( 'NONE',  ( -7.913358619554302642, 16.16796202616373890, -233.0981776325470491 ) ) ;
#7385=CARTESIAN_POINT ( 'NONE',  ( -14.60180519431160917, 24.46340507526420893, -221.8423643191928534 ) ) ;
#7387=CARTESIAN_POINT ( 'NONE',  ( 5.803912621764987456, 13.01725692290267844, -221.8367675400179166 ) ) ;
#7388=CARTESIAN_POINT ( 'NONE',  ( -15.82036597035495795, 4.920771916499852239, -223.0095317795067160 ) ) ;
#7389=CARTESIAN_POINT ( 'NONE',  ( 18.03440114592047649, 4.755211820135348155, -216.3599228381250157 ) ) ;
#7390=CARTESIAN_POINT ( 'NONE',  ( 11.72194121175188997, -15.95900783718691507, -217.6519982781775013 ) ) ;
#7393=CARTESIAN_POINT ( 'NONE',  ( 10.07175337281514871, 14.76776740066196325, -231.7834566702614723 ) ) ;
#7394=CARTESIAN_POINT ( 'NONE',  ( -13.61368873860109652, -1.873405602088730859, -231.0542245685610112 ) ) ;
#7398=CARTESIAN_POINT ( 'NONE',  ( 7.437838793555467731, -20.85539581353325289, -233.9154700400843865 ) ) ;
#7400=CARTESIAN_POINT ( 'NONE',  ( -9.443239614166923701, 9.388015667058336788, -222.3195230688234290 ) ) ;
#7401=CARTESIAN_POINT ( 'NONE',  ( -11.39536650977235510, 9.246300577217761330, -228.4898727004871546 ) ) ;
#7402=CARTESIAN_POINT ( 'NONE',  ( -10.51143808951550085, 11.41308718311005066, -231.3573069600382439 ) ) ;
#7403=CARTESIAN_POINT ( 'NONE',  ( -12.22852564478610482, -7.025360622849957437, -222.3415469712626589 ) ) ;
#7406=CARTESIAN_POINT ( 'NONE',  ( -24.68906941503829700, 2.445024713909649705, -232.6803430500543755 ) ) ;
#7407=CARTESIAN_POINT ( 'NONE',  ( 9.745394341301471641, -28.41975495766811832, -225.7559345954832963 ) ) ;
#7408=CARTESIAN_POINT ( 'NONE',  ( 14.03916608299427082, 11.26328028684000415, -220.2447382113059007 ) ) ;
#7409=CARTESIAN_POINT ( 'NONE',  ( -9.503027668167838726, 6.959046566381404730, -225.7241663910276941 ) ) ;
#7410=CARTESIAN_POINT ( 'NONE',  ( -21.89065952084848021, -0.9940043559354364566, -216.9999999999999716 ) ) ;
#7411=CARTESIAN_POINT ( 'NONE',  ( 13.72034832542693827, 10.98995328009155692, -220.6189139471235592 ) ) ;
#7412=CARTESIAN_POINT ( 'NONE',  ( -3.332878961853828592, -21.58676603248690284, -218.0452238110532619 ) ) ;
#7415=CARTESIAN_POINT ( 'NONE',  ( -4.866400999161825780, 25.69921167300892861, -231.0100031340613782 ) ) ;
#7417=CARTESIAN_POINT ( 'NONE',  ( -13.01542355754912172, 26.77630951171455820, -225.1545229496516356 ) ) ;
#7418=CARTESIAN_POINT ( 'NONE',  ( -16.40095417437164471, 2.582410108382750646, -233.5151473761628154 ) ) ;
#7419=CARTESIAN_POINT ( 'NONE',  ( -15.65248652229887405, -15.36320747609890169, -219.0899148657056230 ) ) ;
#7422=CARTESIAN_POINT ( 'NONE',  ( -22.47200958260654957, 4.697452857301940732, -216.5879371680706242 ) ) ;
#7423=CARTESIAN_POINT ( 'NONE',  ( 0.6532050297617689738, -21.40793743009686878, -217.7635283671393722 ) ) ;
#7424=CARTESIAN_POINT ( 'NONE',  ( 17.97843143658897347, 22.12221935793617078, -220.9346589834416079 ) ) ;
#7425=CARTESIAN_POINT ( 'NONE',  ( 4.603870848087811218, 30.13529352683433515, -225.9623629403671430 ) ) ;
#7428=CARTESIAN_POINT ( 'NONE',  ( -21.01482965301294925, 6.368220028842532798, -231.7530032521518990 ) ) ;
#7429=CARTESIAN_POINT ( 'NONE',  ( 2.008896548638861024, 20.64812324442097591, -233.5818019448501843 ) ) ;
#7431=CARTESIAN_POINT ( 'NONE',  ( -6.012234575298915473, -13.00555924700598709, -229.4955436083688483 ) ) ;
#7432=CARTESIAN_POINT ( 'NONE',  ( 11.90144651507291051, -8.898305237537579515, -228.5592478859710184 ) ) ;
#7435=CARTESIAN_POINT ( 'NONE',  ( -10.59650102373989533, 7.849913810122476576, -230.0486530042683171 ) ) ;
#7436=CARTESIAN_POINT ( 'NONE',  ( -18.47336874364275516, -4.831184938305232990, -219.8627234292127639 ) ) ;
#7437=CARTESIAN_POINT ( 'NONE',  ( -26.11114532382342901, 12.73400870066318902, -227.7653936945517046 ) ) ;
#7438=CARTESIAN_POINT ( 'NONE',  ( 20.26651059498356844, 18.95255124124090074, -231.7206897233655525 ) ) ;
#7439=CARTESIAN_POINT ( 'NONE',  ( 1.313727069624702981, 17.80710275190598324, -219.4197901500037062 ) ) ;
#7441=CARTESIAN_POINT ( 'NONE',  ( 17.90345650676399814, -22.75668921074696982, -218.1849408917474022 ) ) ;
#7443=CARTESIAN_POINT ( 'NONE',  ( 25.33562512631297281, 12.25422971834577268, -228.6777356031426791 ) ) ;
#7444=CARTESIAN_POINT ( 'NONE',  ( -4.424820997438546399, 11.84746159238278373, -221.7815792475208525 ) ) ;
#7445=CARTESIAN_POINT ( 'NONE',  ( -5.340143745732740754, 22.10628181454592678, -235.0476201740528097 ) ) ;
#7446=CARTESIAN_POINT ( 'NONE',  ( -21.27082149447729620, -6.316573346028001801, -216.2864220516500779 ) ) ;
#7447=CARTESIAN_POINT ( 'NONE',  ( -12.31207293045244988, 6.732038552366256923, -221.0952066824360713 ) ) ;
#7449=CARTESIAN_POINT ( 'NONE',  ( 17.43540344723615476, -3.335533435063737340, -230.8961756483947738 ) ) ;
#7450=CARTESIAN_POINT ( 'NONE',  ( -15.95412330064426065, 13.09400588185824077, -218.6613039563597169 ) ) ;
#7451=CARTESIAN_POINT ( 'NONE',  ( 18.59615491886314231, -0.2392802120807639710, -217.5848846836084078 ) ) ;
#7452=CARTESIAN_POINT ( 'NONE',  ( -18.71530386740073126, -0.6857509888707814527, -217.6195632122020527 ) ) ;
#7453=CARTESIAN_POINT ( 'NONE',  ( 11.87982377808925527, 10.85265283465803421, -229.5027252913499183 ) ) ;
#7454=CARTESIAN_POINT ( 'NONE',  ( -13.63272521699743756, -3.226083955879493814, -228.1383267723209656 ) ) ;
#7456=CARTESIAN_POINT ( 'NONE',  ( 2.208705534715813101, 15.26926593729510984, -227.3643075380122980 ) ) ;
#7457=CARTESIAN_POINT ( 'NONE',  ( -5.279374154171231126, -12.28263746854076466, -222.5283095625445640 ) ) ;
#7458=CARTESIAN_POINT ( 'NONE',  ( 15.85665641241444668, 18.24713744004561988, -217.7195292979064902 ) ) ;
#7459=CARTESIAN_POINT ( 'NONE',  ( 3.585135836405817233, -11.76492230538331896, -228.1718440842192024 ) ) ;
#7461=CARTESIAN_POINT ( 'NONE',  ( -12.82737030338386219, 8.595865151885988098, -221.6735325378515142 ) ) ;
#7462=CARTESIAN_POINT ( 'NONE',  ( 22.46263922039936745, -3.404486942579552089, -216.1438077301478415 ) ) ;
#7463=CARTESIAN_POINT ( 'NONE',  ( 2.659252340503933443, 26.58135124637517777, -228.4751214701929314 ) ) ;
#7464=CARTESIAN_POINT ( 'NONE',  ( -13.88743542672353826, 10.36310385030668613, -230.6144170796622745 ) ) ;
#7465=CARTESIAN_POINT ( 'NONE',  ( 22.03647168420945590, 0.3315607655625663064, -232.0572713672586644 ) ) ;
#7466=CARTESIAN_POINT ( 'NONE',  ( -7.913663017152074097, -13.07021161337726944, -228.8713148165744258 ) ) ;
#7467=CARTESIAN_POINT ( 'NONE',  ( 14.96462366732929716, 7.179279272144128754, -233.2042342402542374 ) ) ;
#7469=CARTESIAN_POINT ( 'NONE',  ( -5.618619326056525587, -15.54696343407853654, -233.4463397655492543 ) ) ;
#7470=CARTESIAN_POINT ( 'NONE',  ( 2.785859284650920031, 14.19821255961969619, -226.9946081512528906 ) ) ;
#7471=CARTESIAN_POINT ( 'NONE',  ( 8.903385417657583289, 10.41040586594612272, -227.6527940987422198 ) ) ;
#7472=CARTESIAN_POINT ( 'NONE',  ( -12.15411956849120756, 11.21601165624538687, -228.1895064089065670 ) ) ;
#7473=CARTESIAN_POINT ( 'NONE',  ( -0.3984245442872364484, 11.77931270252508789, -223.1826369159892920 ) ) ;
#7474=CARTESIAN_POINT ( 'NONE',  ( 18.78616100366561881, 3.045752412654093355, -231.5393376370170699 ) ) ;
#7477=CARTESIAN_POINT ( 'NONE',  ( 12.70100985296128115, -15.77027744429350165, -219.4156470604730202 ) ) ;
#7478=ORIENTED_EDGE ( 'NONE', *, *, #21324, .F. ) ;
#7479=CARTESIAN_POINT ( 'NONE',  ( 10.44758276073090109, -14.65753298717242714, -218.5965683461722904 ) ) ;
#7480=CARTESIAN_POINT ( 'NONE',  ( -7.770318051073092036, 21.02940971564074957, -231.8751410922876630 ) ) ;
#7483=CARTESIAN_POINT ( 'NONE',  ( 14.85123888640019452, 5.067529763532427012, -221.9058491819374979 ) ) ;
#7484=CARTESIAN_POINT ( 'NONE',  ( 26.48152825632016061, -2.044474411990439666, -219.3412966555575565 ) ) ;
#7485=CARTESIAN_POINT ( 'NONE',  ( -16.75313578746775889, -14.38352658620038937, -216.6304878158699978 ) ) ;
#7486=CARTESIAN_POINT ( 'NONE',  ( -2.270280637033633475, -14.48864307936496765, -230.4581659391201072 ) ) ;
#7487=CARTESIAN_POINT ( 'NONE',  ( 3.281983756374524663, 15.83593597903271721, -223.8697822987047346 ) ) ;
#7489=CARTESIAN_POINT ( 'NONE',  ( -25.59521542166570640, 7.637420400166985424, -216.4190921938142935 ) ) ;
#7490=CARTESIAN_POINT ( 'NONE',  ( -9.443239614166923701, 9.388015667058336788, -222.3195230688234290 ) ) ;
#7491=CARTESIAN_POINT ( 'NONE',  ( 4.555016420009541989, 17.65848956729471197, -229.5875910199184204 ) ) ;
#7493=CARTESIAN_POINT ( 'NONE',  ( -1.038524475621362075, 14.89017051181998141, -222.3948816610352139 ) ) ;
#7494=CARTESIAN_POINT ( 'NONE',  ( -11.79656379827575918, 10.43402410864828589, -226.0519616335988076 ) ) ;
#7495=CARTESIAN_POINT ( 'NONE',  ( 26.56239871811266440, 9.439457669498057868, -217.7226690415261885 ) ) ;
#7497=CARTESIAN_POINT ( 'NONE',  ( 19.33791609681259160, -22.44220124466257360, -223.0821732511882090 ) ) ;
#7500=CARTESIAN_POINT ( 'NONE',  ( 11.13678936984666912, 26.95732789089726111, -228.8350761760834757 ) ) ;
#7501=CARTESIAN_POINT ( 'NONE',  ( -15.42652243319914085, -1.944528292506083167, -233.0911082444762030 ) ) ;
#7504=CARTESIAN_POINT ( 'NONE',  ( 1.729916699924999746, -18.64927252049523432, -233.5000329212076906 ) ) ;
#7506=CARTESIAN_POINT ( 'NONE',  ( -9.749377714296398878, 10.28442384816749922, -229.3722863967025205 ) ) ;
#7507=CARTESIAN_POINT ( 'NONE',  ( -14.30586181932858914, 18.69563132175512266, -215.8217153853723573 ) ) ;
#7509=CARTESIAN_POINT ( 'NONE',  ( -10.65455960636934662, 10.37188583052882862, -219.5197110153079620 ) ) ;
#7510=CARTESIAN_POINT ( 'NONE',  ( -10.71823000853037655, -10.52987076429259794, -221.3501620068516331 ) ) ;
#7513=CARTESIAN_POINT ( 'NONE',  ( -17.17400284685640344, 24.63223427531467280, -220.6313524368512162 ) ) ;
#7514=CARTESIAN_POINT ( 'NONE',  ( 8.654719819004025538, -19.13368099829532909, -232.5229659899653711 ) ) ;
#7515=CARTESIAN_POINT ( 'NONE',  ( -10.65455960636934662, 10.37188583052882862, -219.5197110153079620 ) ) ;
#7516=CARTESIAN_POINT ( 'NONE',  ( 14.73597170006453361, 7.272367905564328439, -221.0092474305599239 ) ) ;
#7517=CARTESIAN_POINT ( 'NONE',  ( 2.085064686336211892, 14.99578618537741548, -226.0985834012817861 ) ) ;
#7520=CARTESIAN_POINT ( 'NONE',  ( 17.24423567610276109, 8.542587572837451404, -218.6562240232607621 ) ) ;
#7521=CARTESIAN_POINT ( 'NONE',  ( -13.89163392164661204, -16.46234366268243221, -230.8566716434345949 ) ) ;
#7522=ORIENTED_EDGE ( 'NONE', *, *, #11520, .F. ) ;
#7523=CARTESIAN_POINT ( 'NONE',  ( -3.494873682963683059, 27.70407912598904687, -220.5214894769905243 ) ) ;
#7524=CARTESIAN_POINT ( 'NONE',  ( -12.15411956849120756, 11.21601165624538687, -228.1895064089065670 ) ) ;
#7525=CARTESIAN_POINT ( 'NONE',  ( -17.07051451008491938, 15.19890664381897949, -233.6014043774825666 ) ) ;
#7527=CARTESIAN_POINT ( 'NONE',  ( -15.15256618962804858, -12.22297499669621423, -230.3735341043967821 ) ) ;
#7530=CARTESIAN_POINT ( 'NONE',  ( -20.94800339253696109, 4.477632454355491731, -216.5423208360950298 ) ) ;
#7531=CARTESIAN_POINT ( 'NONE',  ( -0.4195811904800660352, -16.41067541138124852, -229.4634529720845819 ) ) ;
#7532=CARTESIAN_POINT ( 'NONE',  ( 21.53262694368047647, 11.06794636811408594, -231.8394491640143826 ) ) ;
#7533=CARTESIAN_POINT ( 'NONE',  ( -3.643097910890548796, 22.16888955197135047, -233.9701981029593298 ) ) ;
#7534=CARTESIAN_POINT ( 'NONE',  ( -26.70018640714903668, 3.110792036746048428, -228.8761207540193823 ) ) ;
#7535=CARTESIAN_POINT ( 'NONE',  ( 11.75630001506626776, 9.075791953625659048, -230.4239556728226717 ) ) ;
#7536=CARTESIAN_POINT ( 'NONE',  ( 14.68783945462866924, 9.535285537539673228, -219.4694094309942045 ) ) ;
#7538=CARTESIAN_POINT ( 'NONE',  ( -16.75313578746775889, -14.38352658620038937, -216.6304878158699978 ) ) ;
#7539=CARTESIAN_POINT ( 'NONE',  ( 2.513843158659109456, -14.78137297724497401, -219.3443999184743518 ) ) ;
#7541=CARTESIAN_POINT ( 'NONE',  ( -12.14471622011552832, 3.716031503296523653, -220.6237729066402835 ) ) ;
#7542=CARTESIAN_POINT ( 'NONE',  ( 12.49911899277810434, -1.774523103166953497, -229.0731493570444002 ) ) ;
#7543=CARTESIAN_POINT ( 'NONE',  ( -26.38808873681881906, 13.30696350521622939, -225.1492950792419663 ) ) ;
#7544=CARTESIAN_POINT ( 'NONE',  ( 6.491278574642851851, 13.23281603069746382, -229.0355254242266767 ) ) ;
#7545=CARTESIAN_POINT ( 'NONE',  ( 9.280831573919673616, 14.67893982993557422, -228.6940810986570796 ) ) ;
#7548=CARTESIAN_POINT ( 'NONE',  ( 12.00030915192824565, -12.23229153226815313, -233.8665814532129730 ) ) ;
#7549=CARTESIAN_POINT ( 'NONE',  ( 13.69275646168278371, 8.674223198772375909, -220.8699857572541987 ) ) ;
#7550=CARTESIAN_POINT ( 'NONE',  ( -5.028549462823471039, 18.55099042571767143, -234.6264744246184648 ) ) ;
#7551=CARTESIAN_POINT ( 'NONE',  ( -4.619644865335168049, 14.75104250038670450, -232.3086264397671812 ) ) ;
#7552=CARTESIAN_POINT ( 'NONE',  ( -28.74911369566071784, -10.37195270599671737, -225.4617258471509729 ) ) ;
#7553=CARTESIAN_POINT ( 'NONE',  ( -11.24282496690421596, 12.44430180464951086, -232.4405891940542404 ) ) ;
#7555=CARTESIAN_POINT ( 'NONE',  ( 15.05575868828727515, -2.428864548505686560, -227.9368649688638584 ) ) ;
#7556=CARTESIAN_POINT ( 'NONE',  ( -5.562203253303141359, 12.75725363875033302, -225.3078268727488478 ) ) ;
#7557=CARTESIAN_POINT ( 'NONE',  ( 29.00474534066713872, 11.29707752057770698, -221.8682176444242771 ) ) ;
#7558=CARTESIAN_POINT ( 'NONE',  ( -22.17339560624464312, 16.26550580028390769, -232.0582861498566274 ) ) ;
#7559=CARTESIAN_POINT ( 'NONE',  ( 9.586902571418640662, 24.43292817174309661, -231.9968623198229807 ) ) ;
#7562=CARTESIAN_POINT ( 'NONE',  ( 4.238595127209166868, 26.19205419861516404, -230.1142052665570077 ) ) ;
#7563=CARTESIAN_POINT ( 'NONE',  ( -11.36971918743327237, -8.287084598727400220, -223.1364763414170227 ) ) ;
#7564=CARTESIAN_POINT ( 'NONE',  ( 3.449504654906655254, 27.59247159270940841, -231.3461799890608859 ) ) ;
#7565=CARTESIAN_POINT ( 'NONE',  ( 13.17462184258262070, -16.01403271225657932, -214.6792330615317610 ) ) ;
#7568=CARTESIAN_POINT ( 'NONE',  ( -11.48592899399814726, 13.65854631785387774, -230.8311022452805616 ) ) ;
#7570=CARTESIAN_POINT ( 'NONE',  ( 16.18295504345472580, -4.390854861972272261, -232.0514848646187716 ) ) ;
#7571=CARTESIAN_POINT ( 'NONE',  ( 1.820119372073704112, 23.17972341190215246, -230.7270437017659503 ) ) ;
#7572=CARTESIAN_POINT ( 'NONE',  ( -12.06153928353927540, 8.661506524875534296, -226.8425068572842349 ) ) ;
#7573=CARTESIAN_POINT ( 'NONE',  ( 14.63113973005795643, 4.926264598692385199, -222.4866305912601945 ) ) ;
#7574=CARTESIAN_POINT ( 'NONE',  ( -15.71547198132422984, -24.70787285779005060, -226.7356521228395536 ) ) ;
#7575=CARTESIAN_POINT ( 'NONE',  ( 10.00603923119254723, 9.610873433734882454, -231.2388095806506669 ) ) ;
#7577=CARTESIAN_POINT ( 'NONE',  ( -21.38010734112553024, -21.14131910627544997, -218.4623475309535365 ) ) ;
#7578=CARTESIAN_POINT ( 'NONE',  ( 8.860681144154234801, 27.11956268701432293, -229.8503778060109823 ) ) ;
#7579=CARTESIAN_POINT ( 'NONE',  ( 15.91624278015930649, 5.932232821383347954, -217.3600859879243217 ) ) ;
#7580=CARTESIAN_POINT ( 'NONE',  ( -18.36252859017411510, 21.06344830687906367, -228.5073589488702623 ) ) ;
#7581=CARTESIAN_POINT ( 'NONE',  ( -2.218529449563984901, 24.06491599887877442, -214.8915873797660652 ) ) ;
#7582=CARTESIAN_POINT ( 'NONE',  ( -21.08008464085897060, -0.9048411197481797119, -217.0000000010748522 ) ) ;
#7583=CARTESIAN_POINT ( 'NONE',  ( 2.864019721262919926, -25.46936398327173379, -230.7696170053991978 ) ) ;
#7585=CARTESIAN_POINT ( 'NONE',  ( 18.03651828442428595, -19.10816016050398147, -231.7458924702002037 ) ) ;
#7586=CARTESIAN_POINT ( 'NONE',  ( 17.99029889091409018, 9.613712288440757092, -232.0298403238024036 ) ) ;
#7587=CARTESIAN_POINT ( 'NONE',  ( -28.96081738894762125, -0.4213479615504204800, -230.3891733152809707 ) ) ;
#7588=CARTESIAN_POINT ( 'NONE',  ( -14.40111287326894640, -6.123720356435734757, -220.5571602876142094 ) ) ;
#7589=CARTESIAN_POINT ( 'NONE',  ( -9.606889355748592152, -11.26588727105406385, -229.9123324032181586 ) ) ;
#7590=CARTESIAN_POINT ( 'NONE',  ( 7.487569386194327770, 15.49107591903592862, -229.0624668269501001 ) ) ;
#7592=CARTESIAN_POINT ( 'NONE',  ( 14.02802030611117878, 3.063901161068346646, -225.6350222114233475 ) ) ;
#7593=CARTESIAN_POINT ( 'NONE',  ( -2.698926868850080041, 12.89339462271858316, -226.7595176699009585 ) ) ;
#7594=CARTESIAN_POINT ( 'NONE',  ( 3.673290835002071653, 15.92545533070904895, -226.4848186297188022 ) ) ;
#7595=CARTESIAN_POINT ( 'NONE',  ( 12.37876697492742650, -4.127359938151530905, -227.8507160500782618 ) ) ;
#7598=CARTESIAN_POINT ( 'NONE',  ( 21.26803326031697949, 19.54255073453192892, -230.5813148908474659 ) ) ;
#7599=CARTESIAN_POINT ( 'NONE',  ( -22.19349712985372491, 11.03542788991621748, -219.7744882786627443 ) ) ;
#7600=CARTESIAN_POINT ( 'NONE',  ( 20.09685469220202236, -2.033783885649083079, -233.1448060988079760 ) ) ;
#7601=CARTESIAN_POINT ( 'NONE',  ( -4.994543945659216000, -15.01629888130124435, -221.3392717856295633 ) ) ;
#7605=CARTESIAN_POINT ( 'NONE',  ( 4.484811161826725900, 15.38298568785217313, -219.4617573400562662 ) ) ;
#7606=CARTESIAN_POINT ( 'NONE',  ( 20.29112488791128399, -13.23242053965672049, -219.3899762660180102 ) ) ;
#7608=CARTESIAN_POINT ( 'NONE',  ( -8.257247207528708444, -26.39349301559143512, -217.9383130379005138 ) ) ;
#7610=CARTESIAN_POINT ( 'NONE',  ( 5.331555957413248059, 27.50712867803999728, -219.0801070358024276 ) ) ;
#7611=CARTESIAN_POINT ( 'NONE',  ( 4.914880347045685660, 14.54749271951947698, -232.8668677254037789 ) ) ;
#7613=CARTESIAN_POINT ( 'NONE',  ( -14.73016414256368911, 22.23431809695627237, -217.1425123644553707 ) ) ;
#7614=CARTESIAN_POINT ( 'NONE',  ( -12.79488508867961549, -11.10380203712096581, -230.9440799972209106 ) ) ;
#7617=CARTESIAN_POINT ( 'NONE',  ( -2.958555384449997661, 13.07587799061801093, -222.7767538261418565 ) ) ;
#7618=CARTESIAN_POINT ( 'NONE',  ( 8.222674095483935020, -17.25680718911290512, -231.8150392270642612 ) ) ;
#7620=CARTESIAN_POINT ( 'NONE',  ( -9.171998067665157350, 9.395241133357435714, -226.3428046914542051 ) ) ;
#7622=CARTESIAN_POINT ( 'NONE',  ( -20.76981451797363576, 10.27702766794165257, -234.3988437453480742 ) ) ;
#7623=CARTESIAN_POINT ( 'NONE',  ( 1.847452069095833593, 15.11597492720254543, -223.6261404253179421 ) ) ;
#7625=CARTESIAN_POINT ( 'NONE',  ( -22.10934047915441170, 0.9940043559354162506, -215.0000000000000000 ) ) ;
#7626=CARTESIAN_POINT ( 'NONE',  ( -10.71434429704389046, -13.39337408441371124, -228.3296939239235428 ) ) ;
#7628=CARTESIAN_POINT ( 'NONE',  ( 11.98894270675143225, 20.38243841428667835, -233.2283128908360084 ) ) ;
#7629=CARTESIAN_POINT ( 'NONE',  ( -15.15469129103955304, 15.56563882170958024, -231.6314069158229643 ) ) ;
#7630=CARTESIAN_POINT ( 'NONE',  ( -13.30451247859013897, 19.85560227862636040, -232.3493821534129609 ) ) ;
#7632=CARTESIAN_POINT ( 'NONE',  ( -19.35484598183500538, -9.368503549647014594, -231.4111816933332477 ) ) ;
#7635=CARTESIAN_POINT ( 'NONE',  ( -21.93900267957129557, 7.862893636934532360, -233.4951761057262161 ) ) ;
#7636=CARTESIAN_POINT ( 'NONE',  ( 5.786710755275625395, -21.74573425722988063, -218.5323380358915131 ) ) ;
#7638=CARTESIAN_POINT ( 'NONE',  ( 4.301648988406530094, 13.23079486486395240, -223.2766268961034655 ) ) ;
#7640=CARTESIAN_POINT ( 'NONE',  ( 17.72360441613731652, -1.822637811265336749, -232.2813868768326984 ) ) ;
#7641=CARTESIAN_POINT ( 'NONE',  ( 12.90536070039565963, 17.66816134723717724, -234.8562535614228750 ) ) ;
#7644=CARTESIAN_POINT ( 'NONE',  ( 22.66390650824515873, 11.48342577402021725, -231.3155567808436217 ) ) ;
#7646=CARTESIAN_POINT ( 'NONE',  ( -12.28596215050325924, -1.831058988293407852, -228.6496409048244516 ) ) ;
#7647=CARTESIAN_POINT ( 'NONE',  ( -12.11864581566431553, -23.10742878804749978, -232.9192999331436909 ) ) ;
#7648=CARTESIAN_POINT ( 'NONE',  ( 1.541778504653760429, -23.48174737203985529, -233.9922866444541967 ) ) ;
#7651=CARTESIAN_POINT ( 'NONE',  ( -1.973648319964989462, 15.33498294326524203, -220.9958390492969329 ) ) ;
#7652=CARTESIAN_POINT ( 'NONE',  ( 25.75143957690053753, -9.476334075918805055, -216.1442976756887617 ) ) ;
#7653=CARTESIAN_POINT ( 'NONE',  ( 17.01060404384151781, -6.151862203644831162, -218.3248062500343849 ) ) ;
#7654=CARTESIAN_POINT ( 'NONE',  ( -14.24491355791863612, 5.286533920242113105, -221.7104936369346433 ) ) ;
#7655=CARTESIAN_POINT ( 'NONE',  ( 10.88376588832297287, 7.577514201227793400, -222.7215714477710833 ) ) ;
#7656=CARTESIAN_POINT ( 'NONE',  ( 20.58393751692968721, 18.55948753678544705, -226.8933397075267635 ) ) ;
#7658=CARTESIAN_POINT ( 'NONE',  ( 12.44757525125794118, -27.84495572490402182, -221.5053358145852656 ) ) ;
#7662=CARTESIAN_POINT ( 'NONE',  ( -0.2269548806647709305, 12.31484924552052718, -228.6688778050056783 ) ) ;
#7663=CARTESIAN_POINT ( 'NONE',  ( -4.695076324262313250, 31.85502299853856201, -223.8918597786031341 ) ) ;
#7664=CARTESIAN_POINT ( 'NONE',  ( -21.14773328851117995, -13.15959238732831693, -217.2646803791660943 ) ) ;
#7665=CARTESIAN_POINT ( 'NONE',  ( -24.48580119005125866, 9.312492396273500006, -232.5498413856076070 ) ) ;
#7667=CARTESIAN_POINT ( 'NONE',  ( 23.12216041205843453, 0.2121350054995089496, -232.0572713672589202 ) ) ;
#7668=CARTESIAN_POINT ( 'NONE',  ( -8.316505849089994129, 18.84563905716333210, -217.0138378867507640 ) ) ;
#7669=CARTESIAN_POINT ( 'NONE',  ( 30.65249971456167799, 3.724008896938769464, -225.4815109119605552 ) ) ;
#7670=CARTESIAN_POINT ( 'NONE',  ( -20.18153419852512442, 14.25141268122526483, -233.5059133483111964 ) ) ;
#7671=CARTESIAN_POINT ( 'NONE',  ( 23.49048926389013658, 9.645778135078892035, -218.7307869890797463 ) ) ;
#7675=CARTESIAN_POINT ( 'NONE',  ( 5.711092584709906106, 26.13380667269736790, -220.5232813324456629 ) ) ;
#7676=CARTESIAN_POINT ( 'NONE',  ( -20.83683780809167629, -19.66850649927503625, -219.7460615899071570 ) ) ;
#7677=CARTESIAN_POINT ( 'NONE',  ( 12.99034161053428349, 11.71468708507361889, -230.9043293568357740 ) ) ;
#7678=CARTESIAN_POINT ( 'NONE',  ( -7.384981288797311194, -12.33405319921006615, -226.2189290763054998 ) ) ;
#7680=CARTESIAN_POINT ( 'NONE',  ( -15.11329978779464689, 11.41628732213579411, -231.7124318929555500 ) ) ;
#7682=CARTESIAN_POINT ( 'NONE',  ( -27.13703770709692265, -3.029478475984613173, -219.1636194202163779 ) ) ;
#7683=CARTESIAN_POINT ( 'NONE',  ( 7.487569386194327770, 15.49107591903592862, -229.0624668269501001 ) ) ;
#7684=CARTESIAN_POINT ( 'NONE',  ( -25.64868633208605786, 12.30364128039660798, -229.0020209687957049 ) ) ;
#7685=CARTESIAN_POINT ( 'NONE',  ( -9.924247690135956645, 7.079756654796299564, -222.1205998075789694 ) ) ;
#7686=CARTESIAN_POINT ( 'NONE',  ( -14.93311267495276518, -24.05029333330348251, -229.1587772033057888 ) ) ;
#7687=CARTESIAN_POINT ( 'NONE',  ( 29.00474534066713872, 11.29707752057770698, -221.8682176444242771 ) ) ;
#7691=CARTESIAN_POINT ( 'NONE',  ( -9.664312646807834639, -7.057764824546099547, -227.2890491868971594 ) ) ;
#7692=CARTESIAN_POINT ( 'NONE',  ( -3.494873682963683059, 27.70407912598904687, -220.5214894769905243 ) ) ;
#7693=CARTESIAN_POINT ( 'NONE',  ( 27.13894094332088969, 12.30518789341946295, -220.2765066586875093 ) ) ;
#7694=CARTESIAN_POINT ( 'NONE',  ( -11.10144104376680652, 18.49675466419975578, -232.2931259015917647 ) ) ;
#7695=CARTESIAN_POINT ( 'NONE',  ( 8.454338299486085617, 13.28844197278511530, -217.6979371188311632 ) ) ;
#7696=CARTESIAN_POINT ( 'NONE',  ( 6.477082923917054202, -23.79794467951758108, -219.1375485160026813 ) ) ;
#7698=CARTESIAN_POINT ( 'NONE',  ( -4.650330424930598561, -23.85841421069521928, -231.7493909980149454 ) ) ;
#7699=CARTESIAN_POINT ( 'NONE',  ( 28.02123297569005089, 5.903198806000402143, -227.5759114383273811 ) ) ;
#7700=CARTESIAN_POINT ( 'NONE',  ( 18.00123703865980218, -15.82960056198189491, -233.0014896689109776 ) ) ;
#7701=CARTESIAN_POINT ( 'NONE',  ( 19.91550388961935525, -0.5333217442993671842, -216.6463151812154138 ) ) ;
#7702=CARTESIAN_POINT ( 'NONE',  ( -11.06377138986482933, -15.30386857868810857, -217.0411070525910873 ) ) ;
#7703=CARTESIAN_POINT ( 'NONE',  ( 13.50603691942335693, 22.79443449215731832, -229.7689193854997995 ) ) ;
#7705=CARTESIAN_POINT ( 'NONE',  ( -14.83095329101371540, 1.580869236763225549, -217.8331819987577660 ) ) ;
#7707=CARTESIAN_POINT ( 'NONE',  ( 2.837900457371055563, 25.11342719071438978, -232.9871906064174709 ) ) ;
#7708=CARTESIAN_POINT ( 'NONE',  ( -2.906906946766868227, 27.66682465340607422, -226.6559963821499082 ) ) ;
#7709=CARTESIAN_POINT ( 'NONE',  ( 17.88855223994683286, -5.550763357372503037, -216.0002797835408614 ) ) ;
#7711=CARTESIAN_POINT ( 'NONE',  ( 16.69977105456987232, 16.51652889326612694, -233.6667933521891030 ) ) ;
#7712=CARTESIAN_POINT ( 'NONE',  ( -18.92390258637512090, 12.75887082072172163, -230.9970325548277970 ) ) ;
#7713=CARTESIAN_POINT ( 'NONE',  ( -26.91858181626453472, 10.72837452931393187, -223.4556356000267670 ) ) ;
#7714=CARTESIAN_POINT ( 'NONE',  ( -4.879290506874147226, -14.18937706998098136, -223.0759034783553147 ) ) ;
#7717=CARTESIAN_POINT ( 'NONE',  ( 5.141746912158045468, 22.01688500372448232, -216.6678693612369386 ) ) ;
#7718=CARTESIAN_POINT ( 'NONE',  ( 17.16551562789753049, -17.52877442517796780, -218.8649675774640286 ) ) ;
#7719=CARTESIAN_POINT ( 'NONE',  ( -13.81390866287826746, 1.832988708064121175, -224.4361041349432639 ) ) ;
#7720=CARTESIAN_POINT ( 'NONE',  ( -12.11864581566431553, -23.10742878804749978, -232.9192999331436909 ) ) ;
#7721=CARTESIAN_POINT ( 'NONE',  ( 0.4042326456706432647, 15.50845657815858303, -219.2680337625893401 ) ) ;
#7723=CARTESIAN_POINT ( 'NONE',  ( -5.191169535941942748, 31.49570301054888688, -227.4714364261087098 ) ) ;
#7725=CARTESIAN_POINT ( 'NONE',  ( -11.79584727357715934, 6.509288465425584036, -222.6080315736180921 ) ) ;
#7726=CARTESIAN_POINT ( 'NONE',  ( 19.99722954683925025, -4.901308424099491745, -217.6076555004800070 ) ) ;
#7729=CARTESIAN_POINT ( 'NONE',  ( -15.58461825850822180, 18.91734573546571951, -233.7691177939990723 ) ) ;
#7730=CARTESIAN_POINT ( 'NONE',  ( -5.618619326056525587, -15.54696343407853654, -233.4463397655492543 ) ) ;
#7731=CARTESIAN_POINT ( 'NONE',  ( 14.31589812732703670, -5.349901619299376243, -221.2752230612865105 ) ) ;
#7733=CARTESIAN_POINT ( 'NONE',  ( -17.75316132689678383, 25.03468689048078843, -222.1645193425721061 ) ) ;
#7734=CARTESIAN_POINT ( 'NONE',  ( -21.07387565400155438, 1.107905485989369554, -215.0000000023499069 ) ) ;
#7735=CARTESIAN_POINT ( 'NONE',  ( -1.316322971969275502, 14.13179993441458215, -224.9782367179667233 ) ) ;
#7737=CARTESIAN_POINT ( 'NONE',  ( -14.83095329101371540, 1.580869236763225549, -217.8331819987577660 ) ) ;
#7738=CARTESIAN_POINT ( 'NONE',  ( -13.83311471749147259, -24.17028674860418747, -226.2550113133487173 ) ) ;
#7740=CARTESIAN_POINT ( 'NONE',  ( 10.03842945413050458, 28.43460431997513638, -225.8374938385031214 ) ) ;
#7741=CARTESIAN_POINT ( 'NONE',  ( -13.23768812067001477, 12.78288831771969569, -230.4179793829127902 ) ) ;
#7742=CARTESIAN_POINT ( 'NONE',  ( -21.95649697515285581, 20.70968357470995258, -226.9638023349746447 ) ) ;
#7743=CARTESIAN_POINT ( 'NONE',  ( -24.66391263913385856, -10.62169550967977472, -229.5175364317193498 ) ) ;
#7748=CARTESIAN_POINT ( 'NONE',  ( -29.30406754532526037, 5.063969254119831120, -221.8212091093853076 ) ) ;
#7749=CARTESIAN_POINT ( 'NONE',  ( -7.253640667752737414, -12.78251829042625687, -230.3353663933772282 ) ) ;
#7750=CARTESIAN_POINT ( 'NONE',  ( 13.46986076300967028, 0.6273780802722437322, -227.9371333673601043 ) ) ;
#7751=CARTESIAN_POINT ( 'NONE',  ( -0.1571923090946999446, 19.34188126963334398, -216.6893131123363787 ) ) ;
#7753=CARTESIAN_POINT ( 'NONE',  ( -18.88344489807484905, 1.071113352238720617, -230.0966926586188208 ) ) ;
#7754=CARTESIAN_POINT ( 'NONE',  ( 12.92410717862594893, 29.37236178718849189, -224.5435071569520744 ) ) ;
#7755=CARTESIAN_POINT ( 'NONE',  ( 19.19288224840068935, 10.13059690604263174, -232.1906135022504998 ) ) ;
#7757=CARTESIAN_POINT ( 'NONE',  ( -14.03169683822311420, -2.573853926495621725, -218.3324423281324016 ) ) ;
#7758=CARTESIAN_POINT ( 'NONE',  ( -19.88402822078561627, -6.951120502836210413, -232.7962440186676361 ) ) ;
#7763=CARTESIAN_POINT ( 'NONE',  ( -2.125813515909480866, 15.68152656492264363, -220.3943115937447317 ) ) ;
#7764=CARTESIAN_POINT ( 'NONE',  ( 31.90367160121947876, -0.9372977198352894224, -223.6547426844143445 ) ) ;
#7765=CARTESIAN_POINT ( 'NONE',  ( 27.92729748684602598, -8.572309054117944527, -222.6487661343338686 ) ) ;
#7766=CARTESIAN_POINT ( 'NONE',  ( -28.61025869263052712, 6.891613135096296361, -222.2489362813765013 ) ) ;
#7767=CARTESIAN_POINT ( 'NONE',  ( 9.774133712851615030, 11.09751083462123766, -229.6876724410067823 ) ) ;
#7768=CARTESIAN_POINT ( 'NONE',  ( 16.29563576379945999, 21.41235115595959826, -221.8114656550040991 ) ) ;
#7770=CARTESIAN_POINT ( 'NONE',  ( 3.924989892941122438, -14.79802789183876044, -219.9433972157300445 ) ) ;
#7773=CARTESIAN_POINT ( 'NONE',  ( 4.569118550756183339, 31.72363458735121000, -222.3920438419263519 ) ) ;
#7774=CARTESIAN_POINT ( 'NONE',  ( -3.687581766460184429, 30.01855770642711718, -218.8323691868875187 ) ) ;
#7775=CARTESIAN_POINT ( 'NONE',  ( 13.96414008557630559, -4.972932825000588863, -226.4793371398648389 ) ) ;
#7777=CARTESIAN_POINT ( 'NONE',  ( -3.843007962268670585, 27.94983497691806917, -231.4302614368887703 ) ) ;
#7782=CARTESIAN_POINT ( 'NONE',  ( 1.660345614755502686, 12.19060476922103931, -223.1112690039082906 ) ) ;
#7783=CARTESIAN_POINT ( 'NONE',  ( 21.06229272850552547, 3.434461253538921621, -234.1452885155528918 ) ) ;
#7784=CARTESIAN_POINT ( 'NONE',  ( -10.51143808951550085, 11.41308718311005066, -231.3573069600382439 ) ) ;
#7785=CARTESIAN_POINT ( 'NONE',  ( 14.98418162551161714, 4.450317369940187895, -227.9894155827521161 ) ) ;
#7788=CARTESIAN_POINT ( 'NONE',  ( -0.7292515499105728383, 28.18841485102515776, -220.8637599502617093 ) ) ;
#7789=CARTESIAN_POINT ( 'NONE',  ( -16.05483997570105714, -7.226811045751038165, -218.5819178105544438 ) ) ;
#7790=CARTESIAN_POINT ( 'NONE',  ( 15.42212722119060864, 5.401662248084913465, -220.8333402320903645 ) ) ;
#7791=CARTESIAN_POINT ( 'NONE',  ( -3.771778814064143504, -12.72945944931849915, -225.7745976896340778 ) ) ;
#7794=CARTESIAN_POINT ( 'NONE',  ( -14.69827142695382527, 14.49176359921644597, -217.9600391472806109 ) ) ;
#7796=CARTESIAN_POINT ( 'NONE',  ( 12.12535264607833341, -6.902938132833007501, -227.3565233277489597 ) ) ;
#7797=CARTESIAN_POINT ( 'NONE',  ( 9.214796078729456497, 26.59493510027307650, -225.5796848805584318 ) ) ;
#7798=CARTESIAN_POINT ( 'NONE',  ( -17.78731991475362406, 16.78509880370027929, -218.2387321183659310 ) ) ;
#7799=CARTESIAN_POINT ( 'NONE',  ( -12.36382104905844592, -0.1264132474004772688, -228.0034406263598896 ) ) ;
#7800=CARTESIAN_POINT ( 'NONE',  ( -16.45250455720563210, -7.911775896682759601, -220.5271995834187067 ) ) ;
#7801=CARTESIAN_POINT ( 'NONE',  ( 14.54999166170408209, 3.068772298969228096, -219.4784171371563275 ) ) ;
#7803=CARTESIAN_POINT ( 'NONE',  ( -14.02432777873800518, -4.625777501976016559, -231.5673840409723709 ) ) ;
#7804=CARTESIAN_POINT ( 'NONE',  ( -0.5888410438786807477, 14.99789765555501475, -227.7044550383138244 ) ) ;
#7805=CARTESIAN_POINT ( 'NONE',  ( 28.65393683769942967, 4.398063292302325067, -219.1542358361629965 ) ) ;
#7806=CARTESIAN_POINT ( 'NONE',  ( -6.593106361191484410, 26.27107262772703322, -231.8730401762632596 ) ) ;
#7807=CARTESIAN_POINT ( 'NONE',  ( 5.501756899793208255, 15.97909684020861043, -233.9380718515096191 ) ) ;
#7809=CARTESIAN_POINT ( 'NONE',  ( 7.465087220526423373, -26.16405931560015219, -221.3372167714960312 ) ) ;
#7811=CARTESIAN_POINT ( 'NONE',  ( -1.380908993000753648, -20.21092959135559752, -218.0995018783601438 ) ) ;
#7812=CARTESIAN_POINT ( 'NONE',  ( 14.19800769603076240, 4.587407146151301518, -224.2928935459285071 ) ) ;
#7813=CARTESIAN_POINT ( 'NONE',  ( 16.07085865561684201, -17.65509622858733252, -216.6880805489183501 ) ) ;
#7814=CARTESIAN_POINT ( 'NONE',  ( -28.30937415889876618, -7.921132361018833556, -222.9755670691803857 ) ) ;
#7815=CARTESIAN_POINT ( 'NONE',  ( -12.14186164972853810, -9.217338937739926408, -220.4665480714278374 ) ) ;
#7816=CARTESIAN_POINT ( 'NONE',  ( 3.746955526231565248, 25.82691596581962656, -220.7780764774678062 ) ) ;
#7818=CARTESIAN_POINT ( 'NONE',  ( -21.39667546302236900, 3.687493526428279100, -235.1435990565495047 ) ) ;
#7819=CARTESIAN_POINT ( 'NONE',  ( 6.093530912645064745, 16.79941505724243811, -232.1766444656230419 ) ) ;
#7820=CARTESIAN_POINT ( 'NONE',  ( 8.321021197036545303, 25.59447019508656140, -228.6184429848799482 ) ) ;
#7821=CARTESIAN_POINT ( 'NONE',  ( 11.86117213253061387, -14.68998886196529874, -215.0859965227146802 ) ) ;
#7822=CARTESIAN_POINT ( 'NONE',  ( 26.59731715018858011, 13.56210517473685329, -229.5787264587298466 ) ) ;
#7823=CARTESIAN_POINT ( 'NONE',  ( -14.22959263369750182, 18.28478771081826793, -217.8090497856120464 ) ) ;
#7824=CARTESIAN_POINT ( 'NONE',  ( -16.40443871513620522, 4.023423476741658789, -228.9829044427089002 ) ) ;
#7825=CARTESIAN_POINT ( 'NONE',  ( -0.1049609700611137120, -29.11428177772140558, -224.8408750893923411 ) ) ;
#7828=CARTESIAN_POINT ( 'NONE',  ( 12.71450444683213021, 7.595266944807587350, -224.4213778964231665 ) ) ;
#7829=CARTESIAN_POINT ( 'NONE',  ( 23.15933523859005660, -14.47549635653155775, -222.2572217030593436 ) ) ;
#7831=CARTESIAN_POINT ( 'NONE',  ( -6.512931564893298386, -17.32529878264574563, -216.7284160531958719 ) ) ;
#7833=CARTESIAN_POINT ( 'NONE',  ( -2.735889804569492600, 12.71735652435744512, -225.1194195722198117 ) ) ;
#7834=CARTESIAN_POINT ( 'NONE',  ( -5.582510911615395699, 27.25430150734737111, -233.3200100877314469 ) ) ;
#7836=CARTESIAN_POINT ( 'NONE',  ( -8.823862513872974489, 14.92351368520778898, -217.1499513473673346 ) ) ;
#7837=CARTESIAN_POINT ( 'NONE',  ( -17.66047203424674450, -3.377913611064220056, -232.7782090104293786 ) ) ;
#7840=CARTESIAN_POINT ( 'NONE',  ( -11.98736441306973077, 11.45674391201457176, -217.8252237716743025 ) ) ;
#7841=CARTESIAN_POINT ( 'NONE',  ( -3.608027314846280031, -12.96557536209330763, -219.9492366723279702 ) ) ;
#7843=CARTESIAN_POINT ( 'NONE',  ( -11.69688825528096388, 18.63404371591177622, -215.8612738028812714 ) ) ;
#7844=CARTESIAN_POINT ( 'NONE',  ( -23.49520248890869212, 11.82830312093803649, -233.3871405502527807 ) ) ;
#7846=CARTESIAN_POINT ( 'NONE',  ( -9.439286754415764591, 28.32957437491962338, -228.7842975624562598 ) ) ;
#7847=CARTESIAN_POINT ( 'NONE',  ( -21.89065952084848021, -0.9940043559354364566, -216.9999999999999716 ) ) ;
#7848=CARTESIAN_POINT ( 'NONE',  ( -12.79639481117843935, 1.974037863663017589, -229.6094308443170746 ) ) ;
#7849=CARTESIAN_POINT ( 'NONE',  ( -7.103355004864593703, -14.30675315766165312, -225.9889059232917532 ) ) ;
#7852=CARTESIAN_POINT ( 'NONE',  ( 8.592982993077152187, 10.20906991731218838, -226.0923132092261483 ) ) ;
#7853=CARTESIAN_POINT ( 'NONE',  ( 2.987882271643250931, 28.57355997650491020, -217.8917278841813925 ) ) ;
#7854=CARTESIAN_POINT ( 'NONE',  ( -18.22136682449241363, -9.036057809225649606, -231.1742889867359736 ) ) ;
#7856=VERTEX_POINT ( 'NONE', #7188 ) ;
#7857=CARTESIAN_POINT ( 'NONE',  ( 20.54442553493903389, -1.409480604460696007, -231.2888200459364327 ) ) ;
#7858=CARTESIAN_POINT ( 'NONE',  ( -9.698809215651296611, -24.51491891025427350, -232.5150754403024962 ) ) ;
#7859=CARTESIAN_POINT ( 'NONE',  ( 18.06016678184731461, 2.257982981100609354, -218.9983079406065940 ) ) ;
#7860=CARTESIAN_POINT ( 'NONE',  ( -2.958555384449997661, 13.07587799061801093, -222.7767538261418565 ) ) ;
#7861=CARTESIAN_POINT ( 'NONE',  ( 15.01641474852163505, -2.073694611913084351, -222.8298119658091139 ) ) ;
#7863=CARTESIAN_POINT ( 'NONE',  ( -16.23590288079963173, 0.2625226423351309513, -226.8300841971807813 ) ) ;
#7864=CARTESIAN_POINT ( 'NONE',  ( 7.174260007897984792, 9.971262771497068300, -226.2872513832048469 ) ) ;
#7867=CARTESIAN_POINT ( 'NONE',  ( 12.23063869552301242, 12.84118223717021934, -218.8273164334868284 ) ) ;
#7870=CARTESIAN_POINT ( 'NONE',  ( 19.53765964318905546, -5.556987368099968627, -230.7409885362571345 ) ) ;
#7871=CARTESIAN_POINT ( 'NONE',  ( -15.58529874627549461, -6.917566422457355202, -219.0138643999995054 ) ) ;
#7874=CARTESIAN_POINT ( 'NONE',  ( -5.383332542724544645, 15.12651309054520432, -231.5699995578976313 ) ) ;
#7875=CARTESIAN_POINT ( 'NONE',  ( 24.73665505496147432, -17.48642391317526190, -218.9253764065177847 ) ) ;
#7876=CARTESIAN_POINT ( 'NONE',  ( 22.36788034568564854, -2.140002702436959225, -217.7104380410378610 ) ) ;
#7877=CARTESIAN_POINT ( 'NONE',  ( -21.28183200535960040, 1.085030287403131233, -217.0000000015322712 ) ) ;
#7878=CARTESIAN_POINT ( 'NONE',  ( 28.03290210476798094, 13.48017620089690638, -224.9212082181537937 ) ) ;
#7879=CARTESIAN_POINT ( 'NONE',  ( 8.858651440950676914, 22.47383302477780376, -230.7859943773311215 ) ) ;
#7881=CARTESIAN_POINT ( 'NONE',  ( 12.92460608403495037, -28.21656386930617089, -223.0937501850342812 ) ) ;
#7882=CARTESIAN_POINT ( 'NONE',  ( 22.03647168420945590, 0.3315607655625663064, -232.0572713672586644 ) ) ;
#7883=CARTESIAN_POINT ( 'NONE',  ( -3.687581766460184429, 30.01855770642711718, -218.8323691868875187 ) ) ;
#7884=CARTESIAN_POINT ( 'NONE',  ( 3.641537757978871248, 12.43698445400491437, -220.3805014257186485 ) ) ;
#7885=CARTESIAN_POINT ( 'NONE',  ( 14.06411491198613462, -8.094314315948059502, -222.2253600114596566 ) ) ;
#7886=CARTESIAN_POINT ( 'NONE',  ( -3.514547081416551588, 30.38636916157537016, -227.3529586180979436 ) ) ;
#7889=CARTESIAN_POINT ( 'NONE',  ( 2.291262277241625345, 17.20278591336981222, -216.2185160402476924 ) ) ;
#7890=CARTESIAN_POINT ( 'NONE',  ( 13.72784977962315267, 2.687686193488206143, -220.8507880271885995 ) ) ;
#7891=CARTESIAN_POINT ( 'NONE',  ( -20.54164754914381064, 7.122791156791981493, -233.5720402887671980 ) ) ;
#7892=CARTESIAN_POINT ( 'NONE',  ( 24.42567939027770407, 10.22651298688739097, -219.4562066833365748 ) ) ;
#7893=CARTESIAN_POINT ( 'NONE',  ( 9.094331215210646135, 23.85463374792894342, -219.7669638091879847 ) ) ;
#7897=CARTESIAN_POINT ( 'NONE',  ( 11.16964468591631920, 25.71443501674299981, -224.7497461878887464 ) ) ;
#7898=CARTESIAN_POINT ( 'NONE',  ( -16.39524763169126942, -10.97410814576847926, -232.9630882351523837 ) ) ;
#7899=CARTESIAN_POINT ( 'NONE',  ( 25.80927844399814930, 11.21489550116160316, -221.3538377621514996 ) ) ;
#7900=CARTESIAN_POINT ( 'NONE',  ( -0.07228948136920625156, -12.49432715273631445, -224.3346527204968766 ) ) ;
#7902=CARTESIAN_POINT ( 'NONE',  ( -15.82622499106666325, 9.895986579907866343, -218.5115209877527604 ) ) ;
#7903=CARTESIAN_POINT ( 'NONE',  ( 8.767697218519710844, -14.65932909790238448, -230.8495237012982386 ) ) ;
#7904=CARTESIAN_POINT ( 'NONE',  ( 9.931717191100288389, 12.93133689537362940, -228.8926047089119038 ) ) ;
#7905=CARTESIAN_POINT ( 'NONE',  ( -13.93825237094548619, 9.044872709574327985, -220.1275804576921757 ) ) ;
#7906=CARTESIAN_POINT ( 'NONE',  ( -12.02603758797190459, 8.152912069735307909, -218.2257190893353709 ) ) ;
#7907=CARTESIAN_POINT ( 'NONE',  ( -18.92071285517992507, -7.235402657652117320, -230.6453433565968680 ) ) ;
#7908=CARTESIAN_POINT ( 'NONE',  ( 8.463901354249619757, 8.457277735286822917, -222.5555366599873821 ) ) ;
#7910=CARTESIAN_POINT ( 'NONE',  ( -6.616223485457675579, -9.589312190179589024, -225.7195100648197581 ) ) ;
#7911=CARTESIAN_POINT ( 'NONE',  ( 2.703362520412529779, 29.60004130108520215, -225.6165589735000481 ) ) ;
#7912=CARTESIAN_POINT ( 'NONE',  ( 14.46993441875745390, 0.2699826811589002284, -230.0986938382904157 ) ) ;
#7913=CARTESIAN_POINT ( 'NONE',  ( -5.786930954831501772, 15.78543306641166311, -231.0475152612371517 ) ) ;
#7914=CARTESIAN_POINT ( 'NONE',  ( 3.490345297502855715, 11.17751288514984331, -224.7799703251421022 ) ) ;
#7915=CARTESIAN_POINT ( 'NONE',  ( 2.737864789122675280, -26.51934750686404385, -230.0373452194950517 ) ) ;
#7916=CARTESIAN_POINT ( 'NONE',  ( -0.8337089444836248697, -27.22572500676309559, -220.1932236949194532 ) ) ;
#7918=CARTESIAN_POINT ( 'NONE',  ( -15.57331739480619248, 4.297375044201914740, -216.4079605712025511 ) ) ;
#7919=CARTESIAN_POINT ( 'NONE',  ( 16.85953475301105442, -7.801609028127129086, -231.9437213283852941 ) ) ;
#7920=CARTESIAN_POINT ( 'NONE',  ( -28.42127686227592420, -0.6461176296494712812, -221.6028628238154567 ) ) ;
#7921=CARTESIAN_POINT ( 'NONE',  ( -12.04756914620937636, -13.80987496524771885, -232.8991007102355582 ) ) ;
#7922=CARTESIAN_POINT ( 'NONE',  ( 2.659252340503933443, 26.58135124637517777, -228.4751214701929314 ) ) ;
#7924=CARTESIAN_POINT ( 'NONE',  ( -31.12406087576577463, 7.316399946619934092, -225.0171288978685027 ) ) ;
#7925=CARTESIAN_POINT ( 'NONE',  ( -3.514547081416551588, 30.38636916157537016, -227.3529586180979436 ) ) ;
#7926=CARTESIAN_POINT ( 'NONE',  ( 2.659252340503933443, 26.58135124637517777, -228.4751214701929314 ) ) ;
#7927=CARTESIAN_POINT ( 'NONE',  ( 12.03076347463371398, -25.25364776008588308, -216.5688293904237298 ) ) ;
#7928=CARTESIAN_POINT ( 'NONE',  ( 18.23116248274160256, 13.99874872632082123, -216.0593560670294835 ) ) ;
#7929=CARTESIAN_POINT ( 'NONE',  ( -14.01525440049806193, 8.239250543314939890, -226.5804714421811070 ) ) ;
#7930=CARTESIAN_POINT ( 'NONE',  ( -16.08005950484750102, -0.1764640578214327904, -223.5999988222837942 ) ) ;
#7931=CARTESIAN_POINT ( 'NONE',  ( -5.322766963623397629, -16.65786661440869665, -219.3972027188067671 ) ) ;
#7934=CARTESIAN_POINT ( 'NONE',  ( 13.61707622192329481, 14.84143455326118932, -217.6958999636067063 ) ) ;
#7935=CARTESIAN_POINT ( 'NONE',  ( 15.35804315687698107, -7.528275283329426415, -228.0874909612831232 ) ) ;
#7936=CARTESIAN_POINT ( 'NONE',  ( -25.44919589272258520, 4.740781954932180575, -232.0725131810460766 ) ) ;
#7938=CARTESIAN_POINT ( 'NONE',  ( -6.012234575298915473, -13.00555924700598709, -229.4955436083688483 ) ) ;
#7940=CARTESIAN_POINT ( 'NONE',  ( -2.817219543927646175, 14.13981714106644993, -229.6779615865167443 ) ) ;
#7941=CARTESIAN_POINT ( 'NONE',  ( 3.672031556878595282, 11.54613252248376831, -227.4694100414545801 ) ) ;
#7943=CARTESIAN_POINT ( 'NONE',  ( -2.772442535524381579, 13.75675912271027457, -228.9770533867650215 ) ) ;
#7944=CARTESIAN_POINT ( 'NONE',  ( -28.12632608809566293, -1.403418003803144742, -218.5233027210585988 ) ) ;
#7947=CARTESIAN_POINT ( 'NONE',  ( -10.51143808951550085, 11.41308718311005066, -231.3573069600382439 ) ) ;
#7948=CARTESIAN_POINT ( 'NONE',  ( -10.19343904566850867, -16.03376756945627335, -215.1857286610140250 ) ) ;
#7949=CARTESIAN_POINT ( 'NONE',  ( 27.92729748684602598, -8.572309054117944527, -222.6487661343338686 ) ) ;
#7950=CARTESIAN_POINT ( 'NONE',  ( -9.540790481621398200, 9.981116473660406996, -228.6478862620407995 ) ) ;
#7951=CARTESIAN_POINT ( 'NONE',  ( -24.69837543585720141, 12.57569301576483589, -232.4521327773205428 ) ) ;
#7952=CARTESIAN_POINT ( 'NONE',  ( -3.130305314451475418, 18.08417128930788209, -217.9058652980469333 ) ) ;
#7953=CARTESIAN_POINT ( 'NONE',  ( -21.08008464085897060, -0.9048411197481797119, -217.0000000010748522 ) ) ;
#7954=CARTESIAN_POINT ( 'NONE',  ( 16.23850682336481199, 8.051046992137072422, -219.2473483181185827 ) ) ;
#7955=CARTESIAN_POINT ( 'NONE',  ( -9.780669591740702273, -13.62818526938769104, -222.3368934028275135 ) ) ;
#7957=CARTESIAN_POINT ( 'NONE',  ( -22.04240660558204823, 19.10355008918698871, -223.9524535985323723 ) ) ;
#7958=CARTESIAN_POINT ( 'NONE',  ( 12.98364502352995942, 13.67380631913144029, -233.1535077318696096 ) ) ;
#7959=CARTESIAN_POINT ( 'NONE',  ( -2.328291070394212792, 14.80737693666302945, -219.0291440940735868 ) ) ;
#7960=CARTESIAN_POINT ( 'NONE',  ( -14.27379873579015879, -4.865929470441826332, -223.9216412988620561 ) ) ;
#7963=CARTESIAN_POINT ( 'NONE',  ( -11.46843428684449151, 6.508406145394057596, -225.7212143570321814 ) ) ;
#7964=CARTESIAN_POINT ( 'NONE',  ( -20.46754208161335598, -23.96478097336112256, -223.3311283152840758 ) ) ;
#7966=CARTESIAN_POINT ( 'NONE',  ( 8.329997790135040603, 12.51216704542961899, -228.7022893680961602 ) ) ;
#7968=CARTESIAN_POINT ( 'NONE',  ( -15.61959985466312872, 8.133362592386543355, -230.7826037412100106 ) ) ;
#7969=CARTESIAN_POINT ( 'NONE',  ( 14.65697969206133067, 11.40587726087447606, -233.3943609825344652 ) ) ;
#7972=CARTESIAN_POINT ( 'NONE',  ( 15.54915848664191280, 0.9682401509573658194, -222.1574103577552819 ) ) ;
#7974=CARTESIAN_POINT ( 'NONE',  ( 12.58590500897257947, 11.38573988265384607, -230.4867078522624695 ) ) ;
#7976=CARTESIAN_POINT ( 'NONE',  ( 22.17529396115045870, -12.37645153867399195, -229.8268438261158906 ) ) ;
#7977=CARTESIAN_POINT ( 'NONE',  ( -14.93108815068229589, -1.792787290847115633, -227.6165763581034582 ) ) ;
#7981=CARTESIAN_POINT ( 'NONE',  ( -9.060295054034883222, 29.20313342278041802, -224.2979742714222482 ) ) ;
#7982=CARTESIAN_POINT ( 'NONE',  ( 25.69869100782391413, -6.466588899411362057, -234.2905747065633193 ) ) ;
#7983=CARTESIAN_POINT ( 'NONE',  ( 20.98776729843937972, -13.55153944770713359, -217.5092423276211946 ) ) ;
#7984=CARTESIAN_POINT ( 'NONE',  ( -29.16153046926437753, 6.356672163541281506, -226.4393515956758165 ) ) ;
#7985=CARTESIAN_POINT ( 'NONE',  ( 15.51129552754472307, 0.2180314803830030457, -231.3815478022924879 ) ) ;
#7986=CARTESIAN_POINT ( 'NONE',  ( 18.30590144060498403, 15.06309558287673767, -219.0459394567220102 ) ) ;
#7988=CARTESIAN_POINT ( 'NONE',  ( 3.722478027540565559, -17.18860102498078390, -232.3439289206262686 ) ) ;
#7990=CARTESIAN_POINT ( 'NONE',  ( -21.73153953336191790, 8.758376218440917071, -235.2971293019126051 ) ) ;
#7992=CARTESIAN_POINT ( 'NONE',  ( 9.818699534354031755, 13.69084898312510390, -233.4870046949650089 ) ) ;
#7993=CARTESIAN_POINT ( 'NONE',  ( 4.065638640983322283, 32.08830473489500434, -226.0249194102539150 ) ) ;
#7994=CARTESIAN_POINT ( 'NONE',  ( 26.42472234358771033, -2.855770380922216134, -231.8949512018254211 ) ) ;
#7995=CARTESIAN_POINT ( 'NONE',  ( -3.643097910890548796, 22.16888955197135047, -233.9701981029593298 ) ) ;
#7996=CARTESIAN_POINT ( 'NONE',  ( -13.11494368899652052, 3.355507568391938200, -225.9121440085824304 ) ) ;
#7998=CARTESIAN_POINT ( 'NONE',  ( -6.127117917506272882, 18.94558806480136681, -232.9763641438055117 ) ) ;
#7999=CARTESIAN_POINT ( 'NONE',  ( -21.16281446184100545, 3.810576631694648775, -218.4455094643457187 ) ) ;
#8000=CARTESIAN_POINT ( 'NONE',  ( -11.79584727357715934, 6.509288465425584036, -222.6080315736180921 ) ) ;
#8001=CARTESIAN_POINT ( 'NONE',  ( 25.80927844399814930, 11.21489550116160316, -221.3538377621514996 ) ) ;
#8002=CARTESIAN_POINT ( 'NONE',  ( 3.325336547283623378, 18.92213121405483633, -219.7480163085221818 ) ) ;
#8003=CARTESIAN_POINT ( 'NONE',  ( -24.65069530437947876, -0.7989515219415058711, -216.4419420286324112 ) ) ;
#8004=CARTESIAN_POINT ( 'NONE',  ( 8.856360819293511710, 14.24139612884802553, -227.7731680686805475 ) ) ;
#8005=CARTESIAN_POINT ( 'NONE',  ( -9.294226473174397540, -12.00440878504259601, -219.6990993854437875 ) ) ;
#8006=CARTESIAN_POINT ( 'NONE',  ( 12.23063869552301242, 12.84118223717021934, -218.8273164334868284 ) ) ;
#8007=CARTESIAN_POINT ( 'NONE',  ( -8.373128421490182660, -27.12459427582015792, -230.7938890564172709 ) ) ;
#8012=CARTESIAN_POINT ( 'NONE',  ( -5.775873073292457249, 17.47547275616994256, -218.7209647771908578 ) ) ;
#8014=CARTESIAN_POINT ( 'NONE',  ( 11.20610455198612598, -10.15455062626793037, -220.8168162286965526 ) ) ;
#8015=CARTESIAN_POINT ( 'NONE',  ( 15.15306935214909778, 7.771180183537883757, -217.5526096523957165 ) ) ;
#8016=CARTESIAN_POINT ( 'NONE',  ( -11.85645341316062051, 18.51497629668490674, -217.8828067666886454 ) ) ;
#8017=CARTESIAN_POINT ( 'NONE',  ( -11.10150084103673684, 3.549415896002023896, -226.0408865487038952 ) ) ;
#8018=CARTESIAN_POINT ( 'NONE',  ( -26.34963598119476913, -8.267085687785165504, -223.3493716711078889 ) ) ;
#8019=CARTESIAN_POINT ( 'NONE',  ( -19.35155980425159683, 1.157993580480985552, -230.3698774940947942 ) ) ;
#8021=CARTESIAN_POINT ( 'NONE',  ( -21.30077981517617047, -23.37245693150986270, -228.9371924788557351 ) ) ;
#8022=CARTESIAN_POINT ( 'NONE',  ( 14.69853173970351179, 23.44775873627089524, -231.2711109634281001 ) ) ;
#8024=CARTESIAN_POINT ( 'NONE',  ( 13.19406830060760605, 4.163358546877222288, -228.8532745215267425 ) ) ;
#8026=CARTESIAN_POINT ( 'NONE',  ( 3.137667653003819446, 15.44806861187908176, -232.6841782316817842 ) ) ;
#8027=CARTESIAN_POINT ( 'NONE',  ( 12.65306858828212810, 29.42930486385247590, -226.3758484992818012 ) ) ;
#8029=CARTESIAN_POINT ( 'NONE',  ( 4.568467666399979699, -17.52045581048442457, -219.7174082404806938 ) ) ;
#8031=CARTESIAN_POINT ( 'NONE',  ( -5.980659577089002532, -19.45286470896024156, -217.9322865582606710 ) ) ;
#8032=CARTESIAN_POINT ( 'NONE',  ( -22.61701582078733708, 5.416317966792455252, -214.6955127214549748 ) ) ;
#8033=CARTESIAN_POINT ( 'NONE',  ( 12.84024077373997841, -14.50125846907313054, -216.8496453050001946 ) ) ;
#8034=CARTESIAN_POINT ( 'NONE',  ( -24.25245498015852874, 0.2109992039763788352, -218.1398602137601301 ) ) ;
#8035=CARTESIAN_POINT ( 'NONE',  ( -7.349743644505656093, -15.31718010764164539, -232.4470764718129772 ) ) ;
#8036=CARTESIAN_POINT ( 'NONE',  ( 25.85827166240959940, 13.84420748389600675, -220.2831452073696425 ) ) ;
#8037=CARTESIAN_POINT ( 'NONE',  ( -10.76972226383489506, 9.682563335906554158, -229.2555443445334333 ) ) ;
#8038=CARTESIAN_POINT ( 'NONE',  ( 18.13412043358480474, 12.55378873098427128, -233.2186159706515696 ) ) ;
#8039=CARTESIAN_POINT ( 'NONE',  ( -3.755296588130283553, 23.77975947300719284, -233.7323173085780752 ) ) ;
#8040=CARTESIAN_POINT ( 'NONE',  ( 11.41090957555148222, 16.52772439454343711, -218.2458222691329013 ) ) ;
#8041=CARTESIAN_POINT ( 'NONE',  ( 22.25403255790844881, -22.02690323431350450, -229.4561893391075671 ) ) ;
#8044=CARTESIAN_POINT ( 'NONE',  ( 24.19635128940818447, 10.31396593861802380, -216.9479509989864425 ) ) ;
#8045=CARTESIAN_POINT ( 'NONE',  ( -5.974114889119001681, 17.52937113675171332, -232.3862906442651592 ) ) ;
#8046=CARTESIAN_POINT ( 'NONE',  ( -10.35216574861945560, -14.43870810227675605, -231.1876371800402126 ) ) ;
#8048=DIRECTION ( 'NONE',  ( 0.1093404791528972547, -0.9940043559354329039, 0.000000000000000000 ) ) ;
#8049=CARTESIAN_POINT ( 'NONE',  ( 12.85408565574548412, 7.821283853063205171, -223.1248833997948111 ) ) ;
#8050=CARTESIAN_POINT ( 'NONE',  ( 11.03497432892593721, -13.14185978141811972, -229.3300340223075011 ) ) ;
#8053=CARTESIAN_POINT ( 'NONE',  ( -1.308474130992312023, -24.58654860180777391, -216.2430112183533026 ) ) ;
#8055=CARTESIAN_POINT ( 'NONE',  ( -3.326157069579807946, 13.92020081821418565, -220.5733722327383930 ) ) ;
#8057=CARTESIAN_POINT ( 'NONE',  ( -4.845359737286285551, 16.85396349487340117, -233.9229833851842670 ) ) ;
#8059=CARTESIAN_POINT ( 'NONE',  ( 2.539761864897490007, 23.64215977235053501, -233.4645566207487661 ) ) ;
#8060=CARTESIAN_POINT ( 'NONE',  ( 29.34815638429084927, -3.655059647784748122, -228.0165508611016207 ) ) ;
#8061=CARTESIAN_POINT ( 'NONE',  ( 26.38334502096500245, -3.352420239867627494, -217.3603908026431384 ) ) ;
#8064=CARTESIAN_POINT ( 'NONE',  ( 5.017623471397871349, 29.83561274492976878, -222.9769172135417250 ) ) ;
#8065=CARTESIAN_POINT ( 'NONE',  ( -10.13139158240655391, -23.04245082364802499, -234.6840773296079874 ) ) ;
#8066=CARTESIAN_POINT ( 'NONE',  ( 6.741123954526870854, -14.00899218320067341, -219.0418835583997179 ) ) ;
#8067=CARTESIAN_POINT ( 'NONE',  ( 18.55298002304457228, -12.22359628793950570, -216.9137843736221782 ) ) ;
#8068=CARTESIAN_POINT ( 'NONE',  ( -17.17981675979428147, 1.478343374046288128, -216.2419730925687418 ) ) ;
#8069=CARTESIAN_POINT ( 'NONE',  ( 15.20072702475037296, 19.31591084219522614, -219.7402199933931399 ) ) ;
#8071=CARTESIAN_POINT ( 'NONE',  ( -19.26845014167239611, 9.481468541508135672, -234.4856117705182328 ) ) ;
#8072=CARTESIAN_POINT ( 'NONE',  ( -16.75383819933101748, -8.593015344009392820, -230.3978590765929084 ) ) ;
#8074=CARTESIAN_POINT ( 'NONE',  ( -12.33203608746942237, 8.428128317385924717, -222.9277009507565026 ) ) ;
#8075=CARTESIAN_POINT ( 'NONE',  ( 4.303123380281038024, 17.66787810618728827, -231.9745698734655832 ) ) ;
#8076=CARTESIAN_POINT ( 'NONE',  ( -6.581016643627174645, 27.50493254600863935, -230.8763182197739070 ) ) ;
#8077=CARTESIAN_POINT ( 'NONE',  ( -27.13703770709692265, -3.029478475984613173, -219.1636194202163779 ) ) ;
#8080=CARTESIAN_POINT ( 'NONE',  ( -12.31207293045244988, 6.732038552366256923, -221.0952066824360713 ) ) ;
#8081=CARTESIAN_POINT ( 'NONE',  ( -14.91192530170583197, -15.94630704366669782, -215.1411503333790165 ) ) ;
#8083=CARTESIAN_POINT ( 'NONE',  ( 6.093530912645064745, 16.79941505724243811, -232.1766444656230419 ) ) ;
#8086=CARTESIAN_POINT ( 'NONE',  ( 13.38839277810360429, -5.174145297632733786, -223.8523798909600941 ) ) ;
#8087=CARTESIAN_POINT ( 'NONE',  ( -20.95553895916151177, 12.88782924195037438, -232.2493899712447956 ) ) ;
#8088=CARTESIAN_POINT ( 'NONE',  ( 19.29259174080182504, 0.5828707127177102931, -219.2781652733668807 ) ) ;
#8091=FACE_OUTER_BOUND ( 'NONE', #13493, .T. ) ;
#8092=CARTESIAN_POINT ( 'NONE',  ( 15.58552416334512536, -6.625011841737234342, -222.1645676924547104 ) ) ;
#8093=CARTESIAN_POINT ( 'NONE',  ( -11.20272313682045073, -7.956653478762055087, -225.3025344850567819 ) ) ;
#8096=CARTESIAN_POINT ( 'NONE',  ( -16.89013823391154290, 26.38860451648245231, -225.6449744083545852 ) ) ;
#8097=CARTESIAN_POINT ( 'NONE',  ( 9.588041944343061118, -18.04984130968639633, -234.4334306750605776 ) ) ;
#8098=CARTESIAN_POINT ( 'NONE',  ( 16.50235023187294203, -3.000022380394500310, -230.0447763498268614 ) ) ;
#8099=CARTESIAN_POINT ( 'NONE',  ( -16.81936022032888545, 5.700806722825413786, -218.5726178058217215 ) ) ;
#8100=CARTESIAN_POINT ( 'NONE',  ( 27.13894094332088969, 12.30518789341946295, -220.2765066586875093 ) ) ;
#8101=CARTESIAN_POINT ( 'NONE',  ( 12.51085646230496273, 9.582567546749562126, -224.6200301875240939 ) ) ;
#8103=CARTESIAN_POINT ( 'NONE',  ( 6.065954396161110651, -11.55577711821250553, -228.1182208427093485 ) ) ;
#8105=CARTESIAN_POINT ( 'NONE',  ( -19.86079186537285324, -0.7838168488858909821, -215.1601656726509475 ) ) ;
#8106=CARTESIAN_POINT ( 'NONE',  ( 10.82528077991200810, 8.849546035972329250, -221.2068619981234008 ) ) ;
#8107=CARTESIAN_POINT ( 'NONE',  ( -0.2269548806647709305, 12.31484924552052718, -228.6688778050056783 ) ) ;
#8108=CARTESIAN_POINT ( 'NONE',  ( 20.48752708986941329, -13.44209471493726937, -230.9762584513030106 ) ) ;
#8109=CARTESIAN_POINT ( 'NONE',  ( -2.934221234790329369, 15.07857928364152222, -230.9558365497803720 ) ) ;
#8110=CARTESIAN_POINT ( 'NONE',  ( -26.02440924314744919, 2.824604386891162111, -232.0644005296583430 ) ) ;
#8112=CARTESIAN_POINT ( 'NONE',  ( 8.463901354249619757, 8.457277735286822917, -222.5555366599873821 ) ) ;
#8114=CARTESIAN_POINT ( 'NONE',  ( -26.88784739727922357, 10.07520213145270915, -227.1866063047054922 ) ) ;
#8115=CARTESIAN_POINT ( 'NONE',  ( -3.514547081416551588, 30.38636916157537016, -227.3529586180979436 ) ) ;
#8116=CARTESIAN_POINT ( 'NONE',  ( 22.84140515590350518, 18.29101041979067332, -226.2334522600520472 ) ) ;
#8117=CARTESIAN_POINT ( 'NONE',  ( 3.433394806375676733, 19.92272173529517332, -219.3341428536850799 ) ) ;
#8118=CARTESIAN_POINT ( 'NONE',  ( 14.64930099072384095, -2.233284345536625803, -226.6630761355773984 ) ) ;
#8120=CARTESIAN_POINT ( 'NONE',  ( -18.11268275035277853, -3.459088653808292335, -218.4233329573673359 ) ) ;
#8121=CARTESIAN_POINT ( 'NONE',  ( 13.43730899468209294, 8.427513769504761498, -221.4030804848920297 ) ) ;
#8122=CARTESIAN_POINT ( 'NONE',  ( -2.170317331930874172, -31.11073952835316803, -223.3804330553629995 ) ) ;
#8124=CARTESIAN_POINT ( 'NONE',  ( -17.14223598032838325, 23.31797360549976261, -226.5771676936548431 ) ) ;
#8126=CARTESIAN_POINT ( 'NONE',  ( 7.876378987416962296, -12.17572650474792617, -223.4643623724329018 ) ) ;
#8127=CARTESIAN_POINT ( 'NONE',  ( 14.87635807518583775, 11.13002414557121789, -232.1789382499626981 ) ) ;
#8128=CARTESIAN_POINT ( 'NONE',  ( -12.78923236353123727, 15.53885160143439315, -231.8946633672937878 ) ) ;
#8129=CARTESIAN_POINT ( 'NONE',  ( -30.66857674073067130, 4.440060741118782239, -229.9901150862898476 ) ) ;
#8130=CARTESIAN_POINT ( 'NONE',  ( -21.95460872137175201, -8.074699112730320039, -230.7190249947325071 ) ) ;
#8132=CARTESIAN_POINT ( 'NONE',  ( 21.75737151495493649, -2.205713500382455283, -233.2756072794337285 ) ) ;
#8134=CARTESIAN_POINT ( 'NONE',  ( -15.39182838237880446, -1.300641671086574469, -219.0680177603771597 ) ) ;
#8135=CARTESIAN_POINT ( 'NONE',  ( 13.48097272627202159, 8.509510470709432894, -231.5257201610278059 ) ) ;
#8136=CARTESIAN_POINT ( 'NONE',  ( -20.92673740658815973, 5.672885432599523270, -219.1433548642331459 ) ) ;
#8138=CARTESIAN_POINT ( 'NONE',  ( 8.036750260989780514, 26.29729070384984624, -233.5018314387838529 ) ) ;
#8139=CARTESIAN_POINT ( 'NONE',  ( 9.851209273476317918, 25.48401176094959553, -233.7173763849377792 ) ) ;
#8141=CARTESIAN_POINT ( 'NONE',  ( -6.657868545208735611, -13.01156946085308874, -219.4730114480542227 ) ) ;
#8143=CARTESIAN_POINT ( 'NONE',  ( 1.167080303844580058, -21.82675117811238152, -232.1335090276773485 ) ) ;
#8144=CARTESIAN_POINT ( 'NONE',  ( -11.80036766549451599, 3.629178540272184783, -221.4826559383200220 ) ) ;
#8145=CARTESIAN_POINT ( 'NONE',  ( 14.98777556431132219, -10.10815648641214004, -217.9795565018743844 ) ) ;
#8146=CARTESIAN_POINT ( 'NONE',  ( 30.27398588404266633, 0.3550328743180605762, -224.9805995843073561 ) ) ;
#8147=CARTESIAN_POINT ( 'NONE',  ( -23.84209965496292227, -7.976777114481962805, -232.1458837748831456 ) ) ;
#8148=CARTESIAN_POINT ( 'NONE',  ( 10.97349919442152810, 9.416813005082010690, -227.3764328406868742 ) ) ;
#8150=CARTESIAN_POINT ( 'NONE',  ( -11.83206531956964902, 10.60028422373495260, -231.1115289952381033 ) ) ;
#8151=CARTESIAN_POINT ( 'NONE',  ( 10.59524789654300925, 9.532374763983630928, -223.0758647391057821 ) ) ;
#8152=CARTESIAN_POINT ( 'NONE',  ( -2.808235066048971440, 30.42019778760651150, -222.6481917607299295 ) ) ;
#8153=CARTESIAN_POINT ( 'NONE',  ( 13.64836464229338198, 15.83060743948028737, -232.0893758582176929 ) ) ;
#8154=CARTESIAN_POINT ( 'NONE',  ( 20.24215890739238688, -18.92204689856563249, -233.5548650425709241 ) ) ;
#8155=CARTESIAN_POINT ( 'NONE',  ( -12.89119823113977503, 10.10140484475961564, -218.5945808114896636 ) ) ;
#8156=CARTESIAN_POINT ( 'NONE',  ( -1.406618399933933006, 16.47239985789244443, -232.2564017133012726 ) ) ;
#8157=CARTESIAN_POINT ( 'NONE',  ( -12.60959727102843786, -12.64039607560028600, -218.2377899390859284 ) ) ;
#8158=CARTESIAN_POINT ( 'NONE',  ( -26.58771759052039485, 5.114955214121561511, -218.2823714869195442 ) ) ;
#8160=CARTESIAN_POINT ( 'NONE',  ( 20.23125423326388628, 7.836699765464857137, -217.8891354894872450 ) ) ;
#8161=CARTESIAN_POINT ( 'NONE',  ( 12.89891433044458502, -16.86700836158627936, -231.6320225002741040 ) ) ;
#8162=CARTESIAN_POINT ( 'NONE',  ( -25.64868633208605786, 12.30364128039660798, -229.0020209687957049 ) ) ;
#8164=CARTESIAN_POINT ( 'NONE',  ( -24.92024473536680773, -13.74570206812420103, -220.1598944320903115 ) ) ;
#8165=CARTESIAN_POINT ( 'NONE',  ( -26.04932551096112192, 5.001193774903864409, -228.9498367494266802 ) ) ;
#8166=CARTESIAN_POINT ( 'NONE',  ( 8.730612144237051453, 13.93563980088501886, -217.1627566045470132 ) ) ;
#8168=CARTESIAN_POINT ( 'NONE',  ( 0.7245137624042983227, 13.44764381486384330, -223.4043886706536455 ) ) ;
#8169=CARTESIAN_POINT ( 'NONE',  ( -29.90835019730369737, -3.078401082523886334, -228.7630230812432046 ) ) ;
#8172=CARTESIAN_POINT ( 'NONE',  ( 1.382955251742491898, 16.46353944795171032, -231.7743150979565030 ) ) ;
#8173=CARTESIAN_POINT ( 'NONE',  ( -3.316277044624852621, -11.89182204942354382, -222.3557635030381618 ) ) ;
#8174=CARTESIAN_POINT ( 'NONE',  ( 8.532614294830283441, -28.73326933124977955, -229.1610356131385231 ) ) ;
#8175=CARTESIAN_POINT ( 'NONE',  ( 17.43540344723615476, -3.335533435063737340, -230.8961756483947738 ) ) ;
#8176=CARTESIAN_POINT ( 'NONE',  ( -27.17783334270200157, 15.20409188923851751, -223.6555185980277258 ) ) ;
#8178=CARTESIAN_POINT ( 'NONE',  ( 11.40028598017942230, 13.60807601628675023, -220.9105305289655519 ) ) ;
#8179=CARTESIAN_POINT ( 'NONE',  ( -17.96792326766206926, -0.6237852504629022299, -217.9759415197746932 ) ) ;
#8180=CARTESIAN_POINT ( 'NONE',  ( -18.17591565587962776, 16.23604867791855355, -233.2845329962925121 ) ) ;
#8181=CARTESIAN_POINT ( 'NONE',  ( -16.76407561856198214, -10.47882714055132070, -219.0733374248486598 ) ) ;
#8182=CARTESIAN_POINT ( 'NONE',  ( -16.12870690754239078, 23.19263481078822053, -221.6099859194323471 ) ) ;
#8183=CARTESIAN_POINT ( 'NONE',  ( 10.88376588832297287, 7.577514201227793400, -222.7215714477710833 ) ) ;
#8184=CARTESIAN_POINT ( 'NONE',  ( 1.867752180833619713, 31.25122076096762669, -227.4007918511463231 ) ) ;
#8185=CARTESIAN_POINT ( 'NONE',  ( 12.74640035234706659, -6.767230903810586895, -221.4971111014800726 ) ) ;
#8188=CARTESIAN_POINT ( 'NONE',  ( -18.39892766464214446, 25.11039525536027739, -225.3444503920457294 ) ) ;
#8189=CARTESIAN_POINT ( 'NONE',  ( -3.077342110593487945, -14.65776296416898816, -220.8866639047373610 ) ) ;
#8191=CARTESIAN_POINT ( 'NONE',  ( 8.689059922489732912, 15.18271246186214363, -218.7354841152034908 ) ) ;
#8193=CARTESIAN_POINT ( 'NONE',  ( 23.48720700658024896, -2.145453947144424500, -217.8824464111000054 ) ) ;
#8194=CARTESIAN_POINT ( 'NONE',  ( -12.31207293045244988, 6.732038552366256923, -221.0952066824360713 ) ) ;
#8195=CARTESIAN_POINT ( 'NONE',  ( -13.63002737749749826, 6.315035547785179837, -227.0490028799284516 ) ) ;
#8196=CARTESIAN_POINT ( 'NONE',  ( 25.40954707198727647, 2.077273811637330159, -219.3610170479527426 ) ) ;
#8199=CARTESIAN_POINT ( 'NONE',  ( 20.34032485158648029, 2.741617426884598530, -217.9827731991294968 ) ) ;
#8201=CARTESIAN_POINT ( 'NONE',  ( 23.20431681157275605, -3.694239143335118492, -219.1264243754107781 ) ) ;
#8202=CARTESIAN_POINT ( 'NONE',  ( -14.48876282330270016, -2.056064607042531911, -223.6537127325441361 ) ) ;
#8205=CARTESIAN_POINT ( 'NONE',  ( 8.132753622789847370, 14.44084924206385701, -222.7013822740049704 ) ) ;
#8206=CARTESIAN_POINT ( 'NONE',  ( 11.85708236628466672, -10.49065743416967145, -217.1712987709648530 ) ) ;
#8207=CARTESIAN_POINT ( 'NONE',  ( 6.374306683232226156, -13.38367253400339330, -219.9651431149896723 ) ) ;
#8208=CARTESIAN_POINT ( 'NONE',  ( -13.51991436508781597, 16.61129329384914755, -232.1184346153593197 ) ) ;
#8209=CARTESIAN_POINT ( 'NONE',  ( 14.50618777373884960, 4.375057440872940795, -230.8807389798650433 ) ) ;
#8210=CARTESIAN_POINT ( 'NONE',  ( 24.96615890023450035, 5.871290975262302148, -218.1661911638112201 ) ) ;
#8212=CARTESIAN_POINT ( 'NONE',  ( -7.069738587058329138, -16.45101055981254845, -220.5392980307454138 ) ) ;
#8214=CARTESIAN_POINT ( 'NONE',  ( -11.10543627608095285, 3.497967533612860613, -224.1342318769322617 ) ) ;
#8215=CARTESIAN_POINT ( 'NONE',  ( 11.78717493688862206, 28.63884142527983556, -229.7724827508652652 ) ) ;
#8216=CARTESIAN_POINT ( 'NONE',  ( 3.044038000507106378, 30.22621415828681180, -231.1553244844465382 ) ) ;
#8217=CARTESIAN_POINT ( 'NONE',  ( 28.84595539031434797, -3.450543886267656735, -229.1532420603894877 ) ) ;
#8218=CARTESIAN_POINT ( 'NONE',  ( -2.735889804569492600, 12.71735652435744512, -225.1194195722198117 ) ) ;
#8219=CARTESIAN_POINT ( 'NONE',  ( -11.79584727357715934, 6.509288465425584036, -222.6080315736180921 ) ) ;
#8221=CARTESIAN_POINT ( 'NONE',  ( 11.38520239593705163, 18.87760105923376486, -235.3435298574111130 ) ) ;
#8222=CARTESIAN_POINT ( 'NONE',  ( -26.91858181626453472, 10.72837452931393187, -223.4556356000267670 ) ) ;
#8223=CARTESIAN_POINT ( 'NONE',  ( -1.249406995060579062, 25.48934319316224162, -216.9406480707515072 ) ) ;
#8225=CARTESIAN_POINT ( 'NONE',  ( 15.50648685944955218, 24.16641006378193168, -224.4827813270165393 ) ) ;
#8226=CARTESIAN_POINT ( 'NONE',  ( 22.14341918773124362, -7.622004812940091689, -217.4502831791021720 ) ) ;
#8229=CARTESIAN_POINT ( 'NONE',  ( -26.98579662683621194, -8.531126968542736222, -229.5232528995939845 ) ) ;
#8230=CARTESIAN_POINT ( 'NONE',  ( -21.89065952084861522, -0.9940043559354512226, -215.0000000000000000 ) ) ;
#8231=CARTESIAN_POINT ( 'NONE',  ( -13.15060755141140980, -21.73659206351220519, -231.8601396556976226 ) ) ;
#8233=CARTESIAN_POINT ( 'NONE',  ( -16.57767831947938575, 23.50485984366324388, -222.7977068309636763 ) ) ;
#8235=CARTESIAN_POINT ( 'NONE',  ( 13.17817051516727922, -26.22376201054615308, -223.3126545406654486 ) ) ;
#8236=CARTESIAN_POINT ( 'NONE',  ( 16.73391517716289911, 11.95167056011791828, -233.0268722588312755 ) ) ;
#8237=CARTESIAN_POINT ( 'NONE',  ( -4.142636420702924482, 14.17169704882741321, -225.1666440184957310 ) ) ;
#8238=CARTESIAN_POINT ( 'NONE',  ( -16.13584396029534318, 23.78382729893626646, -231.6788043429177435 ) ) ;
#8241=CARTESIAN_POINT ( 'NONE',  ( -21.59231333450971135, -13.53975872187591989, -230.0942117760813517 ) ) ;
#8242=CARTESIAN_POINT ( 'NONE',  ( 8.689059922489732912, 15.18271246186214363, -218.7354841152034908 ) ) ;
#8243=CARTESIAN_POINT ( 'NONE',  ( -16.08005950484750102, -0.1764640578214327904, -223.5999988222837942 ) ) ;
#8245=CARTESIAN_POINT ( 'NONE',  ( -27.06886705769815649, 1.548837563602061262, -218.3554811309518868 ) ) ;
#8246=CARTESIAN_POINT ( 'NONE',  ( 8.821742718405863215, 10.82866050966069160, -221.4785132813277642 ) ) ;
#8247=CARTESIAN_POINT ( 'NONE',  ( -18.46822229429615447, 3.027586163204024405, -230.1002726880134333 ) ) ;
#8248=CARTESIAN_POINT ( 'NONE',  ( 2.068961274655788607, 15.13167107497539376, -217.8084559455312501 ) ) ;
#8249=CARTESIAN_POINT ( 'NONE',  ( 16.10828274231666768, 3.530956590605524692, -220.6574330336208050 ) ) ;
#8250=CARTESIAN_POINT ( 'NONE',  ( -10.99009178837907186, -10.32629327015668785, -231.8361825614163365 ) ) ;
#8252=CARTESIAN_POINT ( 'NONE',  ( -17.01799258133205228, -17.74971190556693657, -217.5843211863294755 ) ) ;
#8254=CARTESIAN_POINT ( 'NONE',  ( -25.32262741784088078, 2.623212696197013472, -234.6011982779809841 ) ) ;
#8255=CARTESIAN_POINT ( 'NONE',  ( 8.532614294830283441, -28.73326933124977955, -229.1610356131385231 ) ) ;
#8256=CARTESIAN_POINT ( 'NONE',  ( 27.71804559688024128, -15.88771542466010978, -225.5747850090131692 ) ) ;
#8257=CARTESIAN_POINT ( 'NONE',  ( -17.21167111787709914, -1.850592482912338799, -230.8442569545952665 ) ) ;
#8258=CARTESIAN_POINT ( 'NONE',  ( 11.44717363687632528, 10.34477785005100969, -220.4550508611108341 ) ) ;
#8260=CARTESIAN_POINT ( 'NONE',  ( -19.94037810645588138, 20.40093185429846656, -220.0593903119159620 ) ) ;
#8261=CARTESIAN_POINT ( 'NONE',  ( 21.27834046766391651, 19.84195992785746654, -221.8454931627593965 ) ) ;
#8262=CARTESIAN_POINT ( 'NONE',  ( 17.68508104102419409, 23.41266195669770767, -227.5327139115408954 ) ) ;
#8263=CARTESIAN_POINT ( 'NONE',  ( 11.44717363687632528, 10.34477785005100969, -220.4550508611108341 ) ) ;
#8264=CARTESIAN_POINT ( 'NONE',  ( 12.32676726801020450, -8.454629307895981327, -217.7935467833756036 ) ) ;
#8265=CARTESIAN_POINT ( 'NONE',  ( -5.629016366058284149, 14.31889596247328633, -229.4177297515988414 ) ) ;
#8268=CARTESIAN_POINT ( 'NONE',  ( 22.86997486125673618, 17.56009411325475966, -222.3578648042903296 ) ) ;
#8269=CARTESIAN_POINT ( 'NONE',  ( 4.894111852004805030, -16.26971588820515890, -218.1545738548100530 ) ) ;
#8270=CARTESIAN_POINT ( 'NONE',  ( -20.57288920227272655, 16.51351902378409520, -230.8484733908063333 ) ) ;
#8271=CARTESIAN_POINT ( 'NONE',  ( 10.40160332990717151, 27.59713857063802323, -221.5374724512453213 ) ) ;
#8272=CARTESIAN_POINT ( 'NONE',  ( -19.88402822078561627, -6.951120502836210413, -232.7962440186676361 ) ) ;
#8273=CARTESIAN_POINT ( 'NONE',  ( 21.72366288329714834, 2.385777479048636351, -215.9150265590827757 ) ) ;
#8274=CARTESIAN_POINT ( 'NONE',  ( 10.46530733675539793, 8.351728317179080818, -222.7431177495969621 ) ) ;
#8275=CARTESIAN_POINT ( 'NONE',  ( -0.3969026096611234511, 20.89748314411456676, -216.3289738411752978 ) ) ;
#8276=CARTESIAN_POINT ( 'NONE',  ( 18.71980393303116230, -12.14054210360577457, -231.5113610204687120 ) ) ;
#8277=CARTESIAN_POINT ( 'NONE',  ( 25.09678678204237201, -16.96620885351193309, -225.7902784465786965 ) ) ;
#8279=CARTESIAN_POINT ( 'NONE',  ( 0.2389779871941385414, 16.64595486589868045, -218.1658233406367629 ) ) ;
#8280=CARTESIAN_POINT ( 'NONE',  ( -12.86575055733568540, -10.70886189207742589, -216.1397835820578450 ) ) ;
#8281=CARTESIAN_POINT ( 'NONE',  ( 11.14834367153813233, -21.42845646353120870, -216.4520112529555718 ) ) ;
#8282=CARTESIAN_POINT ( 'NONE',  ( 15.65513449100897780, -26.00057195821942457, -227.4103383097017570 ) ) ;
#8283=CARTESIAN_POINT ( 'NONE',  ( -8.463283775975803280, 12.69606588598396613, -228.6351674091961286 ) ) ;
#8284=CARTESIAN_POINT ( 'NONE',  ( 12.16813927252146144, 18.27141895336136912, -230.9123895730235745 ) ) ;
#8285=CARTESIAN_POINT ( 'NONE',  ( -24.48580119005125866, 9.312492396273500006, -232.5498413856076070 ) ) ;
#8286=CARTESIAN_POINT ( 'NONE',  ( -13.34869474643618581, 6.516017165032126357, -231.2228057326931321 ) ) ;
#8287=CARTESIAN_POINT ( 'NONE',  ( -11.98034293927688765, -10.98662817740026121, -223.7553339400932373 ) ) ;
#8290=CARTESIAN_POINT ( 'NONE',  ( -9.627017372966443887, 15.60690227900018279, -218.8878023709062859 ) ) ;
#8291=CARTESIAN_POINT ( 'NONE',  ( 12.74913679152205148, 9.185760885856177893, -218.6542381594888980 ) ) ;
#8292=CARTESIAN_POINT ( 'NONE',  ( -6.415689407129693045, 29.32186846096819011, -228.3852515614991887 ) ) ;
#8294=CARTESIAN_POINT ( 'NONE',  ( 21.50885124049339936, -13.38680967545814404, -232.7305552638522954 ) ) ;
#8298=CARTESIAN_POINT ( 'NONE',  ( -19.00318367631585659, 13.14621133775862916, -233.8403879275295765 ) ) ;
#8299=CARTESIAN_POINT ( 'NONE',  ( -9.514686225151438137, -9.899715435889788751, -219.6589915062491229 ) ) ;
#8301=CARTESIAN_POINT ( 'NONE',  ( 14.31308345469695453, 12.76656023072872159, -231.9445021321040770 ) ) ;
#8303=CARTESIAN_POINT ( 'NONE',  ( 19.88636028791461641, -20.85574262981397453, -219.9907771812986823 ) ) ;
#8304=CARTESIAN_POINT ( 'NONE',  ( -28.13472254077564116, 12.33996625515159629, -224.9141344439281909 ) ) ;
#8305=CARTESIAN_POINT ( 'NONE',  ( -24.30769394037691100, 17.48612956801762053, -223.4340414801748693 ) ) ;
#8306=CARTESIAN_POINT ( 'NONE',  ( 16.77055746703809191, 7.081497542956901370, -232.0295235404293521 ) ) ;
#8307=CARTESIAN_POINT ( 'NONE',  ( -5.249799428260828904, -14.16826377401270065, -226.9124264195330056 ) ) ;
#8308=CARTESIAN_POINT ( 'NONE',  ( 15.11539441383292903, 0.3024091369739423940, -222.0146986666484565 ) ) ;
#8309=CARTESIAN_POINT ( 'NONE',  ( 28.51464931495100785, 5.422321182929326966, -223.8116416110474347 ) ) ;
#8311=CARTESIAN_POINT ( 'NONE',  ( 15.75976565806011465, -3.644771625422815298, -224.1463364774561740 ) ) ;
#8312=CARTESIAN_POINT ( 'NONE',  ( 13.35970348376145367, -2.045361282085617738, -227.1953586564414991 ) ) ;
#8315=CARTESIAN_POINT ( 'NONE',  ( 11.27486163995310164, 25.12851252939060487, -222.6718455410222930 ) ) ;
#8316=CARTESIAN_POINT ( 'NONE',  ( 13.13237050162318553, -11.26662123460813092, -216.1773046078333209 ) ) ;
#8317=CARTESIAN_POINT ( 'NONE',  ( 13.49882595795384255, -9.201056071450322449, -219.2439763087855908 ) ) ;
#8319=CARTESIAN_POINT ( 'NONE',  ( -15.51982305277792307, 19.76957551617798359, -231.4018974401358832 ) ) ;
#8320=CARTESIAN_POINT ( 'NONE',  ( -22.10934047915413814, 0.9940043559354462266, -218.9999999999999716 ) ) ;
#8321=CARTESIAN_POINT ( 'NONE',  ( 17.92683513449900445, 4.153309877386362814, -218.0960491240478234 ) ) ;
#8322=ORIENTED_EDGE ( 'NONE', *, *, #315, .F. ) ;
#8323=CARTESIAN_POINT ( 'NONE',  ( -6.842387616420496421, -14.58019248909694632, -223.2484495378617453 ) ) ;
#8325=CARTESIAN_POINT ( 'NONE',  ( -12.02603758797190459, 8.152912069735307909, -218.2257190893353709 ) ) ;
#8326=CARTESIAN_POINT ( 'NONE',  ( 11.75630001506626776, 9.075791953625659048, -230.4239556728226717 ) ) ;
#8327=CARTESIAN_POINT ( 'NONE',  ( 14.94332666820587008, -17.95933738324940165, -219.3037465242801147 ) ) ;
#8328=CARTESIAN_POINT ( 'NONE',  ( 12.04687593227112430, 27.54339840196571743, -224.6466266724203820 ) ) ;
#8329=CARTESIAN_POINT ( 'NONE',  ( -12.44873260470819787, 7.411970124596155785, -229.4214091473984070 ) ) ;
#8331=CARTESIAN_POINT ( 'NONE',  ( 22.92330650806121639, 19.11387742755395180, -231.6463539987045976 ) ) ;
#8332=CARTESIAN_POINT ( 'NONE',  ( -16.29666348338687953, 2.994680995215331709, -221.2421885839926006 ) ) ;
#8334=CARTESIAN_POINT ( 'NONE',  ( -9.716674560061926869, 27.56227806819028103, -219.4917914922789919 ) ) ;
#8336=CARTESIAN_POINT ( 'NONE',  ( 3.060417506408009469, 27.46204888741655026, -226.6022202862033623 ) ) ;
#8340=CARTESIAN_POINT ( 'NONE',  ( -25.42089018817326007, -6.263968923056941307, -218.6542964065910439 ) ) ;
#8341=CARTESIAN_POINT ( 'NONE',  ( -30.17036082276531772, 5.959165309317525860, -219.4883053239162791 ) ) ;
#8342=CARTESIAN_POINT ( 'NONE',  ( -12.60888841760081824, -15.87650330583304914, -218.3826098682522456 ) ) ;
#8345=CARTESIAN_POINT ( 'NONE',  ( -10.70754874174748039, 23.84972878377777405, -230.7991598016655246 ) ) ;
#8346=CARTESIAN_POINT ( 'NONE',  ( 11.75796858304313375, -24.75965012883946414, -219.8219186532837455 ) ) ;
#8347=CARTESIAN_POINT ( 'NONE',  ( 12.89118769162836031, 6.140251663080722899, -228.8792332048833771 ) ) ;
#8348=CARTESIAN_POINT ( 'NONE',  ( -4.490213599459100813, 14.55066867058898694, -222.6488251579668827 ) ) ;
#8349=CARTESIAN_POINT ( 'NONE',  ( -16.38161496430853248, 17.22219235543852989, -215.3343469598664797 ) ) ;
#8351=CARTESIAN_POINT ( 'NONE',  ( 18.88835481822873774, -3.841660717124094848, -234.8883833189080974 ) ) ;
#8353=CARTESIAN_POINT ( 'NONE',  ( 10.85888002857596923, 15.81835858589122878, -232.3913150909872627 ) ) ;
#8354=CARTESIAN_POINT ( 'NONE',  ( -14.08236938285573636, 6.062428076406559008, -221.7923619418395447 ) ) ;
#8355=CARTESIAN_POINT ( 'NONE',  ( -21.16281446184100545, 3.810576631694648775, -218.4455094643457187 ) ) ;
#8357=CARTESIAN_POINT ( 'NONE',  ( 14.96415947227435339, -1.927366939720012606, -222.7010313878448358 ) ) ;
#8358=CARTESIAN_POINT ( 'NONE',  ( 28.33476664927451338, -0.7768526459456059907, -228.3750448408243869 ) ) ;
#8359=CARTESIAN_POINT ( 'NONE',  ( 13.82984244654956107, 22.51831320572884820, -232.1830460045772213 ) ) ;
#8360=CARTESIAN_POINT ( 'NONE',  ( -15.50322565568834321, 9.749075856218723857, -229.6019304695566916 ) ) ;
#8361=CARTESIAN_POINT ( 'NONE',  ( -6.415689407129693045, 29.32186846096819011, -228.3852515614991887 ) ) ;
#8362=CARTESIAN_POINT ( 'NONE',  ( 14.68015846516680867, 2.651775288685355836, -224.1317433549420173 ) ) ;
#8363=CARTESIAN_POINT ( 'NONE',  ( -3.607128793317693649, -14.45447024314366402, -228.6383918289709811 ) ) ;
#8366=CARTESIAN_POINT ( 'NONE',  ( -8.983992482398329926, -13.08794618741998761, -229.3325301586503713 ) ) ;
#8367=CARTESIAN_POINT ( 'NONE',  ( -15.35982698007958724, 5.508237851081846159, -233.6994028941782631 ) ) ;
#8368=CARTESIAN_POINT ( 'NONE',  ( 2.513843158659109456, -14.78137297724497401, -219.3443999184743518 ) ) ;
#8369=CARTESIAN_POINT ( 'NONE',  ( -0.9414827276148034496, 23.96885519606619752, -216.4491898092606164 ) ) ;
#8370=CARTESIAN_POINT ( 'NONE',  ( 14.18953136290653205, -9.569333121228954298, -216.2179364387266389 ) ) ;
#8371=CARTESIAN_POINT ( 'NONE',  ( -14.40111287326894640, -6.123720356435734757, -220.5571602876142094 ) ) ;
#8372=CARTESIAN_POINT ( 'NONE',  ( 24.20411255886326529, 12.66254860825103634, -218.0144359054998802 ) ) ;
#8375=CARTESIAN_POINT ( 'NONE',  ( -13.96653539523557619, 20.94398119165846239, -231.8597527081015528 ) ) ;
#8376=CARTESIAN_POINT ( 'NONE',  ( 16.82251835652528982, 18.18719385133374544, -231.8032941011735772 ) ) ;
#8377=CARTESIAN_POINT ( 'NONE',  ( 8.329997790135040603, 12.51216704542961899, -228.7022893680961602 ) ) ;
#8378=CARTESIAN_POINT ( 'NONE',  ( 9.253909228257674258, 17.69332415812615977, -230.9900471521432621 ) ) ;
#8379=CARTESIAN_POINT ( 'NONE',  ( -0.3220389361364618397, -21.73025720764451663, -234.5721229173148856 ) ) ;
#8380=CARTESIAN_POINT ( 'NONE',  ( -12.33583941212908108, 22.27382123621224608, -231.6290720151527296 ) ) ;
#8381=CARTESIAN_POINT ( 'NONE',  ( -25.29098058636142810, 5.014641116111857144, -217.4658967307323110 ) ) ;
#8386=CARTESIAN_POINT ( 'NONE',  ( 8.168748216644726057, -13.67612414567523693, -220.8005964828080607 ) ) ;
#8387=CARTESIAN_POINT ( 'NONE',  ( -11.94782396647286049, 8.456988817430419303, -225.5094493096559063 ) ) ;
#8388=CARTESIAN_POINT ( 'NONE',  ( 2.464084843620814702, 29.35663482419208492, -227.0015060686748143 ) ) ;
#8389=CARTESIAN_POINT ( 'NONE',  ( -22.53818779203657741, -7.663114047788936567, -232.6164956747681458 ) ) ;
#8390=CARTESIAN_POINT ( 'NONE',  ( 13.30790133003807441, 0.6370684082013071681, -222.3495379725305270 ) ) ;
#8391=CARTESIAN_POINT ( 'NONE',  ( 15.88965480228581839, 12.37830464553330678, -233.8570207506254235 ) ) ;
#8393=CARTESIAN_POINT ( 'NONE',  ( 5.248230734842167955, 23.54336384919183445, -216.8914391693808739 ) ) ;
#8394=CARTESIAN_POINT ( 'NONE',  ( 15.59528062753244804, -5.679035096727840681, -230.0190217829878918 ) ) ;
#8395=CARTESIAN_POINT ( 'NONE',  ( 14.49023023880111083, -12.14520762395643061, -217.6171285705176501 ) ) ;
#8397=CARTESIAN_POINT ( 'NONE',  ( 8.979547488457603421, 23.24376652602565230, -232.6628827740196357 ) ) ;
#8398=CARTESIAN_POINT ( 'NONE',  ( -27.95235446785429545, -6.124178816625678756, -218.3296603670965226 ) ) ;
#8399=CARTESIAN_POINT ( 'NONE',  ( -13.13432812001650341, -19.42279346457301514, -216.4126494286626610 ) ) ;
#8400=CARTESIAN_POINT ( 'NONE',  ( 10.30328786010431052, -20.08430705480546408, -216.1847100135515802 ) ) ;
#8402=CARTESIAN_POINT ( 'NONE',  ( -10.10782416658048710, 9.083762506436128703, -227.1045422723873344 ) ) ;
#8403=CARTESIAN_POINT ( 'NONE',  ( 5.112468059216026539, 15.05346046978967856, -223.6558835435016590 ) ) ;
#8404=CARTESIAN_POINT ( 'NONE',  ( -13.69675006931110417, 3.702342960760605539, -228.0723273272095355 ) ) ;
#8405=CARTESIAN_POINT ( 'NONE',  ( -20.49711526797010208, 7.006997077916217620, -215.3369776077118445 ) ) ;
#8406=CARTESIAN_POINT ( 'NONE',  ( -22.73111095712577168, -10.24355154293710690, -230.8570942615963872 ) ) ;
#8408=CARTESIAN_POINT ( 'NONE',  ( -4.073886805163430935, 14.35067061637828623, -226.4733297826468572 ) ) ;
#8409=CARTESIAN_POINT ( 'NONE',  ( 23.18902850759750933, 20.27908137164207147, -226.2847847834817117 ) ) ;
#8410=CARTESIAN_POINT ( 'NONE',  ( 19.07698357483942786, 25.86742807064150895, -222.6991278896559834 ) ) ;
#8411=CARTESIAN_POINT ( 'NONE',  ( 10.62272209279942992, -9.818939940036045755, -222.1403336352628344 ) ) ;
#8414=CARTESIAN_POINT ( 'NONE',  ( -4.104500432947460808, 15.73223271406093460, -218.0734292856946297 ) ) ;
#8415=CARTESIAN_POINT ( 'NONE',  ( -19.52111408301234974, -15.33805657151784985, -234.6553009392178808 ) ) ;
#8417=CARTESIAN_POINT ( 'NONE',  ( 20.41153371889344825, 17.18812948447019551, -230.7531656956970778 ) ) ;
#8419=CARTESIAN_POINT ( 'NONE',  ( 24.96294718070021901, -13.86220829677249178, -229.4442241490162075 ) ) ;
#8421=CARTESIAN_POINT ( 'NONE',  ( -13.11494368899652052, 3.355507568391938200, -225.9121440085824304 ) ) ;
#8423=CARTESIAN_POINT ( 'NONE',  ( 15.70515172005171323, -0.7403987186381333352, -226.4590404369862995 ) ) ;
#8424=CARTESIAN_POINT ( 'NONE',  ( -12.50828242918857036, -25.45147276965577277, -228.7626325223041022 ) ) ;
#8426=CARTESIAN_POINT ( 'NONE',  ( 14.80394259695730064, 1.224172658189580432, -225.4564070658925061 ) ) ;
#8427=CARTESIAN_POINT ( 'NONE',  ( -16.20072894238734307, 0.5024448614660336210, -230.4554067149722130 ) ) ;
#8428=CARTESIAN_POINT ( 'NONE',  ( 11.61478720377483675, -14.40087791365289860, -230.4552745109343448 ) ) ;
#8429=CARTESIAN_POINT ( 'NONE',  ( 13.59365628422294137, -1.921009172773990858, -227.3069749406489564 ) ) ;
#8431=CARTESIAN_POINT ( 'NONE',  ( 10.79895562092076844, 12.01490073542734116, -225.7380208924852809 ) ) ;
#8432=CARTESIAN_POINT ( 'NONE',  ( 5.112468059216026539, 15.05346046978967856, -223.6558835435016590 ) ) ;
#8433=CARTESIAN_POINT ( 'NONE',  ( 10.18197402670511842, -10.22146582328408115, -231.5691222609812598 ) ) ;
#8434=CARTESIAN_POINT ( 'NONE',  ( 12.13827923251525220, -9.172799829723585319, -229.1860353116090891 ) ) ;
#8435=CARTESIAN_POINT ( 'NONE',  ( -16.12870690754239078, 23.19263481078822053, -221.6099859194323471 ) ) ;
#8436=CARTESIAN_POINT ( 'NONE',  ( -15.65611835717891687, 5.486779671999271635, -227.0554626315911264 ) ) ;
#8437=CARTESIAN_POINT ( 'NONE',  ( 15.80790828609669951, 3.698719088746416972, -219.8106174092292804 ) ) ;
#8440=CARTESIAN_POINT ( 'NONE',  ( -7.194605141218047173, -25.04260655977047278, -230.2952862975163271 ) ) ;
#8442=CARTESIAN_POINT ( 'NONE',  ( -13.55637112341987383, 4.614880311503475774, -231.8130385267184010 ) ) ;
#8444=CARTESIAN_POINT ( 'NONE',  ( 10.39636392256998221, 18.46527700675686035, -215.1860221565626148 ) ) ;
#8445=CARTESIAN_POINT ( 'NONE',  ( 16.48523685932656235, -13.39871719616043855, -218.9387417542926926 ) ) ;
#8446=CARTESIAN_POINT ( 'NONE',  ( 2.539761864897490007, 23.64215977235053501, -233.4645566207487661 ) ) ;
#8447=CARTESIAN_POINT ( 'NONE',  ( -28.17543631911187063, 3.557555778861649642, -230.1980773687482156 ) ) ;
#8448=CARTESIAN_POINT ( 'NONE',  ( 25.17176037151762813, 18.95054595444721102, -221.3490360113488862 ) ) ;
#8450=CARTESIAN_POINT ( 'NONE',  ( -19.84402263676350131, 8.565754689849573111, -217.6561116767911983 ) ) ;
#8451=CARTESIAN_POINT ( 'NONE',  ( -0.3969026096611234511, 20.89748314411456676, -216.3289738411752978 ) ) ;
#8454=CARTESIAN_POINT ( 'NONE',  ( 8.332496243628455090, -29.79192972398156769, -226.1452587264855367 ) ) ;
#8456=CARTESIAN_POINT ( 'NONE',  ( 17.43540344723615476, -3.335533435063737340, -230.8961756483947738 ) ) ;
#8458=CARTESIAN_POINT ( 'NONE',  ( -27.85133024402786006, -1.794102530182491773, -229.4204807338591081 ) ) ;
#8459=CARTESIAN_POINT ( 'NONE',  ( 15.52719855059926424, 1.633696074270991172, -221.7349885876216433 ) ) ;
#8460=CARTESIAN_POINT ( 'NONE',  ( -22.37826137345437871, -13.90312800710061047, -229.3506127454622572 ) ) ;
#8463=CARTESIAN_POINT ( 'NONE',  ( 12.20621255000322947, -21.57429421806300240, -232.1397031738524674 ) ) ;
#8464=EDGE_CURVE ( 'NONE', #5173, #3103, #4630, .T. ) ;
#8465=CARTESIAN_POINT ( 'NONE',  ( -15.30864812529618391, 1.596444765892653717, -220.3859421844601627 ) ) ;
#8466=CARTESIAN_POINT ( 'NONE',  ( -14.22255565734842619, 21.32307452572284134, -218.8849463683180261 ) ) ;
#8467=CARTESIAN_POINT ( 'NONE',  ( -4.591517861330576267, 12.55780501983563191, -223.5932882008353033 ) ) ;
#8468=CARTESIAN_POINT ( 'NONE',  ( -15.79547310275335725, -3.553268508742920773, -224.0225025563328813 ) ) ;
#8470=CARTESIAN_POINT ( 'NONE',  ( 9.107417252317809186, 16.30291009569977234, -218.0131178633739921 ) ) ;
#8471=CARTESIAN_POINT ( 'NONE',  ( -16.66929017373293931, 3.065794289431343689, -220.7800282905443794 ) ) ;
#8472=CARTESIAN_POINT ( 'NONE',  ( -17.65933056022148762, 0.7424667221540405260, -229.0964312085266386 ) ) ;
#8477=CARTESIAN_POINT ( 'NONE',  ( 12.98364502352995942, 13.67380631913144029, -233.1535077318696096 ) ) ;
#8478=CARTESIAN_POINT ( 'NONE',  ( -24.82235633397527508, 10.76243500821901300, -227.9886044494091948 ) ) ;
#8479=CARTESIAN_POINT ( 'NONE',  ( -0.7286890422672397394, 21.00519367000705273, -234.2149015821977969 ) ) ;
#8480=CARTESIAN_POINT ( 'NONE',  ( 21.92281339924938877, 16.67475415235398017, -231.9828670874568957 ) ) ;
#8481=CARTESIAN_POINT ( 'NONE',  ( -14.91192530170583197, -15.94630704366669782, -215.1411503333790165 ) ) ;
#8483=CARTESIAN_POINT ( 'NONE',  ( -5.534391910549205207, -14.54353160188980709, -228.1022699408985943 ) ) ;
#8484=CARTESIAN_POINT ( 'NONE',  ( -23.66836017558062011, 21.44695383684080525, -223.6245772351065568 ) ) ;
#8485=CARTESIAN_POINT ( 'NONE',  ( 1.904360901363437275, -12.77109371939166138, -224.5066922355585177 ) ) ;
#8486=CARTESIAN_POINT ( 'NONE',  ( -8.172572110426221670, 16.86653848210977813, -233.4220330256369493 ) ) ;
#8487=CARTESIAN_POINT ( 'NONE',  ( 28.08871713846552254, -6.057249427443905709, -231.1189077393881348 ) ) ;
#8489=CARTESIAN_POINT ( 'NONE',  ( -16.39524763169126942, -10.97410814576847926, -232.9630882351523837 ) ) ;
#8490=CARTESIAN_POINT ( 'NONE',  ( 10.25308675723727347, 13.16459519580956972, -229.3963488176951273 ) ) ;
#8492=CARTESIAN_POINT ( 'NONE',  ( -8.221702953833418093, 11.87876791566348800, -223.9138461338794741 ) ) ;
#8493=CARTESIAN_POINT ( 'NONE',  ( 15.74259730902452858, 17.40808440793174583, -232.1327802909178786 ) ) ;
#8494=CARTESIAN_POINT ( 'NONE',  ( 22.86997486125673618, 17.56009411325475966, -222.3578648042903296 ) ) ;
#8495=CARTESIAN_POINT ( 'NONE',  ( 14.96080648943632241, 22.28365808184747721, -220.1237743409445216 ) ) ;
#8496=CARTESIAN_POINT ( 'NONE',  ( -4.239735564391798661, -14.20018808486349116, -230.2489621771221380 ) ) ;
#8497=CARTESIAN_POINT ( 'NONE',  ( -3.162425552858488143, 20.40327580806445695, -216.0004724541873316 ) ) ;
#8498=CARTESIAN_POINT ( 'NONE',  ( 14.80394259695730064, 1.224172658189580432, -225.4564070658925061 ) ) ;
#8499=CARTESIAN_POINT ( 'NONE',  ( 8.082980660592431477, -16.66562551544545201, -231.4954396659114764 ) ) ;
#8500=CARTESIAN_POINT ( 'NONE',  ( -16.28025842329327944, 6.985656672962045732, -231.4191468057695715 ) ) ;
#8502=CARTESIAN_POINT ( 'NONE',  ( 3.378648530876271039, 26.08525450992624428, -218.4319906442508454 ) ) ;
#8504=CARTESIAN_POINT ( 'NONE',  ( -13.21314811618155716, -9.038438575223175064, -230.6430079410957603 ) ) ;
#8505=CARTESIAN_POINT ( 'NONE',  ( 21.96352831578506937, -0.3315607655626218175, -233.9427286327412787 ) ) ;
#8506=CARTESIAN_POINT ( 'NONE',  ( 7.393167209263542539, 10.77319710117329699, -221.1179833906701049 ) ) ;
#8508=CARTESIAN_POINT ( 'NONE',  ( 4.343013938751969505, 13.02036404005131587, -224.7825435359082178 ) ) ;
#8509=CARTESIAN_POINT ( 'NONE',  ( 13.96414008557630559, -4.972932825000588863, -226.4793371398648389 ) ) ;
#8510=CARTESIAN_POINT ( 'NONE',  ( 22.46263922039936745, -3.404486942579552089, -216.1438077301478415 ) ) ;
#8512=CARTESIAN_POINT ( 'NONE',  ( -3.514547081416551588, 30.38636916157537016, -227.3529586180979436 ) ) ;
#8513=CARTESIAN_POINT ( 'NONE',  ( -18.68851093906118521, -8.564152624513159395, -215.1804141040323941 ) ) ;
#8514=CARTESIAN_POINT ( 'NONE',  ( -0.6367083786117293531, -29.73461014436635708, -220.1383336929387724 ) ) ;
#8515=CARTESIAN_POINT ( 'NONE',  ( 10.99893791904045415, -12.61823049403341201, -218.3266956685045841 ) ) ;
#8516=CARTESIAN_POINT ( 'NONE',  ( -8.115738378024497379, 16.90402287339461296, -219.0833473190803034 ) ) ;
#8517=CARTESIAN_POINT ( 'NONE',  ( 10.63406535173453271, 22.16595115341124256, -219.6461356279925781 ) ) ;
#8518=CARTESIAN_POINT ( 'NONE',  ( -11.67631226053870996, 6.737291529340801333, -227.3110382950315227 ) ) ;
#8519=CARTESIAN_POINT ( 'NONE',  ( -11.83206531956964902, 10.60028422373495260, -231.1115289952381033 ) ) ;
#8520=CARTESIAN_POINT ( 'NONE',  ( -11.98587399847077783, -10.70615994290841044, -225.3229167341726225 ) ) ;
#8521=CARTESIAN_POINT ( 'NONE',  ( -11.48592899399814726, 13.65854631785387774, -230.8311022452805616 ) ) ;
#8522=CARTESIAN_POINT ( 'NONE',  ( 22.42925200799500729, 5.652256920629083581, -234.0734181799116698 ) ) ;
#8523=CARTESIAN_POINT ( 'NONE',  ( 19.13589083395335422, 16.69125564174534659, -234.7442498487877174 ) ) ;
#8524=CARTESIAN_POINT ( 'NONE',  ( 21.85730963248023428, -9.423385237436111339, -216.6089804361807580 ) ) ;
#8527=CARTESIAN_POINT ( 'NONE',  ( -11.02345917017863464, 29.02019856777526741, -223.9475008740665771 ) ) ;
#8528=CARTESIAN_POINT ( 'NONE',  ( -21.73784594492672895, -5.247588939251936146, -214.6321000900504714 ) ) ;
#8530=CARTESIAN_POINT ( 'NONE',  ( 14.63113973005795643, 4.926264598692385199, -222.4866305912601945 ) ) ;
#8531=CARTESIAN_POINT ( 'NONE',  ( -20.43618815875133521, 1.403378831510147196, -232.9646741665398224 ) ) ;
#8532=CARTESIAN_POINT ( 'NONE',  ( 13.62757736989142465, -5.584028114184929947, -227.2616851496390211 ) ) ;
#8533=CARTESIAN_POINT ( 'NONE',  ( -27.29953305526601426, 11.21644211419729054, -229.3676346105362995 ) ) ;
#8535=CARTESIAN_POINT ( 'NONE',  ( 14.64440749032966593, 2.523901497798496596, -225.4572725674553340 ) ) ;
#8536=CARTESIAN_POINT ( 'NONE',  ( -5.056986327342952947, -15.36481113542577503, -220.7955371552936583 ) ) ;
#8538=CARTESIAN_POINT ( 'NONE',  ( 15.76910524310159900, 5.601482066865847820, -220.3440822020379528 ) ) ;
#8539=CARTESIAN_POINT ( 'NONE',  ( -14.87984907657228639, 0.2138881189739126887, -228.7773920408832282 ) ) ;
#8540=CARTESIAN_POINT ( 'NONE',  ( 14.99967020447171784, -24.16696097797641940, -221.8072564961694297 ) ) ;
#8541=CARTESIAN_POINT ( 'NONE',  ( 12.80949378899885893, -2.780008750929118033, -226.1439410239644303 ) ) ;
#8544=CARTESIAN_POINT ( 'NONE',  ( 7.497537106193371770, 19.52448593130572618, -231.1338690134634248 ) ) ;
#8545=CARTESIAN_POINT ( 'NONE',  ( 8.856360819293511710, 14.24139612884802553, -227.7731680686805475 ) ) ;
#8546=CARTESIAN_POINT ( 'NONE',  ( 6.498966860804143764, -11.65341448970024274, -221.3944939044252749 ) ) ;
#8547=CARTESIAN_POINT ( 'NONE',  ( 8.709470447750865318, -17.43408031369701661, -216.5121658579468829 ) ) ;
#8549=CARTESIAN_POINT ( 'NONE',  ( -19.65084584916038324, 18.01805631773661176, -219.5040736310571106 ) ) ;
#8550=CARTESIAN_POINT ( 'NONE',  ( -20.92673740658815973, 5.672885432599523270, -219.1433548642331459 ) ) ;
#8551=CARTESIAN_POINT ( 'NONE',  ( 25.01541028746040141, 13.78427203520734423, -225.9266837950359843 ) ) ;
#8552=VERTEX_POINT ( 'NONE', #7410 ) ;
#8553=CARTESIAN_POINT ( 'NONE',  ( -7.536234698756538286, -25.83616497442384130, -229.4709156672317363 ) ) ;
#8556=CARTESIAN_POINT ( 'NONE',  ( 14.68015846516680867, 2.651775288685355836, -224.1317433549420173 ) ) ;
#8557=CARTESIAN_POINT ( 'NONE',  ( 9.672299229151310129, -14.28303711772943529, -228.3078296064027484 ) ) ;
#8558=CARTESIAN_POINT ( 'NONE',  ( 7.762960416026701616, 12.60702317161859121, -221.9096828323375235 ) ) ;
#8559=CARTESIAN_POINT ( 'NONE',  ( -18.70100282803782576, 16.58357028540773115, -216.4425743468854080 ) ) ;
#8560=CARTESIAN_POINT ( 'NONE',  ( 5.773563157792669820, 21.63217468058455140, -235.0383461317610170 ) ) ;
#8561=CARTESIAN_POINT ( 'NONE',  ( -12.98662328632235585, 28.83726371277012035, -223.5970274767108776 ) ) ;
#8562=CARTESIAN_POINT ( 'NONE',  ( -11.42613629117093765, 28.09170287990588832, -228.7150250545069241 ) ) ;
#8564=CARTESIAN_POINT ( 'NONE',  ( 5.982950994121768673, -14.58086824529316594, -231.1438280359330975 ) ) ;
#8565=CARTESIAN_POINT ( 'NONE',  ( 28.78651053433536333, -0.9604905981993369091, -227.3547688931310233 ) ) ;
#8567=CARTESIAN_POINT ( 'NONE',  ( -28.18501077041064562, -8.523171531337160545, -227.0531053546762337 ) ) ;
#8568=CARTESIAN_POINT ( 'NONE',  ( 24.03642272140365677, 3.646960756862087205, -218.2320643939070806 ) ) ;
#8569=CARTESIAN_POINT ( 'NONE',  ( -19.84632485794307399, -12.65249528142034485, -231.0223831579344278 ) ) ;
#8570=CARTESIAN_POINT ( 'NONE',  ( 6.025688374458400887, -15.61258154445926749, -220.0079782759978002 ) ) ;
#8571=CARTESIAN_POINT ( 'NONE',  ( -28.31595744342370580, 5.786754998807587924, -229.0820962600229223 ) ) ;
#8572=CARTESIAN_POINT ( 'NONE',  ( 10.03842945413050458, 28.43460431997513638, -225.8374938385031214 ) ) ;
#8573=CARTESIAN_POINT ( 'NONE',  ( -6.072587425033909803, 24.65158735603439055, -217.4249768037189767 ) ) ;
#8575=CARTESIAN_POINT ( 'NONE',  ( -17.04360437375341419, -3.174793268193519591, -228.4680687138289841 ) ) ;
#8577=CARTESIAN_POINT ( 'NONE',  ( 22.46220731426537043, 18.23201731183003460, -227.5436199598787539 ) ) ;
#8579=CARTESIAN_POINT ( 'NONE',  ( -17.89085717681497201, 10.08962028281416856, -232.3705156551908431 ) ) ;
#8580=CARTESIAN_POINT ( 'NONE',  ( -17.91550223652134122, 4.809113705933536487, -230.6324822114035555 ) ) ;
#8581=CARTESIAN_POINT ( 'NONE',  ( -10.30161254035895091, -9.966167094494833734, -223.3409979381218875 ) ) ;
#8584=CARTESIAN_POINT ( 'NONE',  ( 17.66525298603349370, 4.919957226727790456, -233.3736646485340032 ) ) ;
#8585=CARTESIAN_POINT ( 'NONE',  ( -18.42638600874552424, 7.060399206045774534, -230.3991437614443214 ) ) ;
#8586=CARTESIAN_POINT ( 'NONE',  ( 19.49137065790598555, 9.165486118354671419, -234.8706749352814995 ) ) ;
#8588=CARTESIAN_POINT ( 'NONE',  ( 15.90795275983908574, 2.546196724714939297, -229.0855319561646297 ) ) ;
#8589=CARTESIAN_POINT ( 'NONE',  ( -10.66474234094022755, -20.68992156881482813, -215.8674331684499634 ) ) ;
#8591=CARTESIAN_POINT ( 'NONE',  ( -10.06927776881013514, -17.00317020600589402, -217.8513858272130790 ) ) ;
#8592=CARTESIAN_POINT ( 'NONE',  ( -9.964021556040458805, 12.25789996591640119, -217.8262340283327774 ) ) ;
#8593=CARTESIAN_POINT ( 'NONE',  ( 2.967317674205219191, -16.40215926535219282, -217.6245344443522924 ) ) ;
#8594=CARTESIAN_POINT ( 'NONE',  ( 1.217121169770782663, 15.31158828575123110, -230.6845728599757308 ) ) ;
#8595=CARTESIAN_POINT ( 'NONE',  ( 11.58852274881379962, -8.803378160360782800, -231.6724139265004965 ) ) ;
#8596=CARTESIAN_POINT ( 'NONE',  ( -25.82802808205240552, -14.78441951539553401, -222.6940535085979604 ) ) ;
#8597=CARTESIAN_POINT ( 'NONE',  ( -13.81390866287826746, 1.832988708064121175, -224.4361041349432639 ) ) ;
#8599=CARTESIAN_POINT ( 'NONE',  ( -2.806347010929339802, 19.90767250424812573, -230.9206976900916004 ) ) ;
#8600=CARTESIAN_POINT ( 'NONE',  ( 17.41909632439413969, 2.006477695503792624, -233.4081875040758121 ) ) ;
#8601=CARTESIAN_POINT ( 'NONE',  ( 15.87442104186276381, 8.674488492264579520, -230.9702037640878416 ) ) ;
#8602=CARTESIAN_POINT ( 'NONE',  ( 16.48801037644500056, 3.165716804515234628, -216.8169430726136113 ) ) ;
#8603=CARTESIAN_POINT ( 'NONE',  ( 4.579865149819754677, -13.09122092233156387, -219.1296897471712839 ) ) ;
#8604=CARTESIAN_POINT ( 'NONE',  ( 12.58033168766476528, 20.35631482982274676, -235.1670639654690547 ) ) ;
#8605=CARTESIAN_POINT ( 'NONE',  ( 17.07668571305246985, 2.037405138410691485, -219.7626854147787867 ) ) ;
#8606=CARTESIAN_POINT ( 'NONE',  ( 12.13370821170821223, -20.35915274155448174, -217.8532457648388458 ) ) ;
#8607=CARTESIAN_POINT ( 'NONE',  ( -21.19360951076126653, 12.15251088906093457, -217.9482185194656552 ) ) ;
#8608=CARTESIAN_POINT ( 'NONE',  ( 8.175342817246784577, 19.41817470142738244, -216.6818271833384699 ) ) ;
#8609=CARTESIAN_POINT ( 'NONE',  ( -11.88525712185471050, -8.925198460467992589, -221.0951487055306472 ) ) ;
#8610=CARTESIAN_POINT ( 'NONE',  ( 24.81079154715000357, 3.171651085595392772, -216.4177249688571578 ) ) ;
#8612=CARTESIAN_POINT ( 'NONE',  ( 17.88619020626327938, 19.43517936004721847, -216.7078103882350604 ) ) ;
#8613=CARTESIAN_POINT ( 'NONE',  ( 13.61707622192329481, 14.84143455326118932, -217.6958999636067063 ) ) ;
#8614=CARTESIAN_POINT ( 'NONE',  ( 13.49585564903807722, -8.492623513249517586, -227.3331091713134811 ) ) ;
#8615=CARTESIAN_POINT ( 'NONE',  ( 25.90657540470570197, -10.31326923046670885, -218.6707845005603019 ) ) ;
#8617=CARTESIAN_POINT ( 'NONE',  ( 18.50911814746675788, 15.92944434255054453, -232.0449215596906072 ) ) ;
#8618=CARTESIAN_POINT ( 'NONE',  ( -11.84714279977019125, -8.528511525072332233, -232.0239825124074002 ) ) ;
#8619=CARTESIAN_POINT ( 'NONE',  ( -8.379125946468517938, -29.31735857037017468, -221.8060643354269814 ) ) ;
#8620=CARTESIAN_POINT ( 'NONE',  ( 5.434900225474387447, -11.93567727083262042, -224.7511004068755369 ) ) ;
#8621=CARTESIAN_POINT ( 'NONE',  ( -2.993956627714193353, 22.04778837082692178, -231.1741803919495339 ) ) ;
#8622=CARTESIAN_POINT ( 'NONE',  ( 28.52435124311170966, 7.611291969169514005, -224.8315247833735384 ) ) ;
#8623=CARTESIAN_POINT ( 'NONE',  ( -22.47200958260654957, 4.697452857301940732, -216.5879371680706242 ) ) ;
#8624=CARTESIAN_POINT ( 'NONE',  ( -8.752190949579933488, 24.25633523490762755, -230.6624101830059885 ) ) ;
#8625=CARTESIAN_POINT ( 'NONE',  ( 17.44158214791148964, -8.186237638883257617, -216.9355394212118995 ) ) ;
#8627=CARTESIAN_POINT ( 'NONE',  ( -16.57767831947938575, 23.50485984366324388, -222.7977068309636763 ) ) ;
#8628=CARTESIAN_POINT ( 'NONE',  ( 29.55842656951424985, 4.785221541509360854, -220.5134865854112718 ) ) ;
#8629=CARTESIAN_POINT ( 'NONE',  ( 18.65058977333779211, 24.40868228550881014, -219.3406275662563303 ) ) ;
#8630=CARTESIAN_POINT ( 'NONE',  ( 12.12535264607833341, -6.902938132833007501, -227.3565233277489597 ) ) ;
#8631=CARTESIAN_POINT ( 'NONE',  ( 13.55929460187270053, 0.3562519042583365270, -227.9787723277739246 ) ) ;
#8633=CARTESIAN_POINT ( 'NONE',  ( -0.1571923090946999446, 19.34188126963334398, -216.6893131123363787 ) ) ;
#8634=CARTESIAN_POINT ( 'NONE',  ( -8.763358281418030415, -9.103836352148345412, -222.0692104753270257 ) ) ;
#8636=CARTESIAN_POINT ( 'NONE',  ( 21.35706335192880445, 15.67286272432725092, -219.2578158352350783 ) ) ;
#8637=CARTESIAN_POINT ( 'NONE',  ( -14.10849459794400751, -0.2436790717799666162, -223.1085195285415921 ) ) ;
#8638=CARTESIAN_POINT ( 'NONE',  ( 15.11994912051959972, -12.48385213956034079, -232.8079920308188377 ) ) ;
#8639=CARTESIAN_POINT ( 'NONE',  ( -17.84981083811007707, 0.8485253248287054628, -231.8041300026935119 ) ) ;
#8640=CARTESIAN_POINT ( 'NONE',  ( -15.20262116893801974, 8.038155052917188570, -217.6767387945475036 ) ) ;
#8641=CARTESIAN_POINT ( 'NONE',  ( -3.176860551132370425, -19.01962362838126452, -231.5826211182368297 ) ) ;
#8644=CARTESIAN_POINT ( 'NONE',  ( -13.56774755469388616, 7.311522441667196226, -219.1912666243428021 ) ) ;
#8645=CARTESIAN_POINT ( 'NONE',  ( 19.65870185572374140, -17.77243814521307641, -229.4329728153015253 ) ) ;
#8646=CARTESIAN_POINT ( 'NONE',  ( 13.24751142555096273, -1.959735780492239288, -222.7273387214888203 ) ) ;
#8648=CARTESIAN_POINT ( 'NONE',  ( 16.53859560591101641, 22.24348416270211359, -223.7250258089275974 ) ) ;
#8649=CARTESIAN_POINT ( 'NONE',  ( 5.585286719045844173, 27.51657303716567426, -222.4190945945824751 ) ) ;
#8650=CARTESIAN_POINT ( 'NONE',  ( 3.436191426816104233, -15.97976940388950773, -231.4631329546418499 ) ) ;
#8651=CARTESIAN_POINT ( 'NONE',  ( 8.785770181087007913, -10.38731345016515917, -223.4272116603623317 ) ) ;
#8653=CARTESIAN_POINT ( 'NONE',  ( -10.30870167223346456, 11.95603877111467561, -228.4123369090513336 ) ) ;
#8654=CARTESIAN_POINT ( 'NONE',  ( -24.40185606299549192, 11.66496215664722236, -221.9473669705449765 ) ) ;
#8655=CARTESIAN_POINT ( 'NONE',  ( -12.12559971566433958, 1.856299769312002912, -227.8748781050665286 ) ) ;
#8656=CARTESIAN_POINT ( 'NONE',  ( -11.97657177269377371, -18.30092786828533846, -219.1278344157730942 ) ) ;
#8659=CARTESIAN_POINT ( 'NONE',  ( 23.64727379217503866, 9.907944788639682088, -232.0643337313508709 ) ) ;
#8660=CARTESIAN_POINT ( 'NONE',  ( 9.097575839043912538, -18.13002900832716335, -219.2719510042808224 ) ) ;
#8661=CARTESIAN_POINT ( 'NONE',  ( 17.68508104102419409, 23.41266195669770767, -227.5327139115408954 ) ) ;
#8662=CARTESIAN_POINT ( 'NONE',  ( -8.966714183099560032, 19.05224306381768073, -234.0879867025980445 ) ) ;
#8664=CARTESIAN_POINT ( 'NONE',  ( 25.30941179858102430, 8.661697827793627624, -216.7530520919057722 ) ) ;
#8665=CARTESIAN_POINT ( 'NONE',  ( 5.248230734842167955, 23.54336384919183445, -216.8914391693808739 ) ) ;
#8667=CARTESIAN_POINT ( 'NONE',  ( -1.778254167844783851, -12.78790610364390012, -225.9413532495922254 ) ) ;
#8668=CARTESIAN_POINT ( 'NONE',  ( 13.38839277810360429, -5.174145297632733786, -223.8523798909600941 ) ) ;
#8671=CARTESIAN_POINT ( 'NONE',  ( 20.58703255433590940, 0.4816031003617209372, -231.9427175861361263 ) ) ;
#8672=CARTESIAN_POINT ( 'NONE',  ( -13.33153391309230074, -13.53657406488594184, -231.3594229707590557 ) ) ;
#8673=CARTESIAN_POINT ( 'NONE',  ( 9.835929410207317147, -16.71508016877321268, -232.2716196330763694 ) ) ;
#8674=CARTESIAN_POINT ( 'NONE',  ( 26.06405806384012536, 5.488112530166501024, -216.5020692413490622 ) ) ;
#8675=CARTESIAN_POINT ( 'NONE',  ( -1.975202609796049336, 20.81351768191813889, -217.5779402428482001 ) ) ;
#8676=CARTESIAN_POINT ( 'NONE',  ( -1.386728072030569692, 16.52832439466973824, -230.7516952943509807 ) ) ;
#8678=CARTESIAN_POINT ( 'NONE',  ( 29.53814377227115884, -10.02285884041311270, -220.1614914916521286 ) ) ;
#8680=CARTESIAN_POINT ( 'NONE',  ( 8.979547488457603421, 23.24376652602565230, -232.6628827740196357 ) ) ;
#8681=CARTESIAN_POINT ( 'NONE',  ( -19.61183938075907918, 22.25855138946451106, -229.5731876748794207 ) ) ;
#8682=CARTESIAN_POINT ( 'NONE',  ( -15.82952867276381603, 3.677461268355039170, -227.9997968350711801 ) ) ;
#8683=CARTESIAN_POINT ( 'NONE',  ( -7.972347216402701164, -18.74702622849856937, -232.1058264431568148 ) ) ;
#8685=CARTESIAN_POINT ( 'NONE',  ( 14.00715608756928532, 4.299235856235253728, -230.2440235370780215 ) ) ;
#8686=CARTESIAN_POINT ( 'NONE',  ( -16.48883219358909713, 20.84100960965193394, -219.4392138569792507 ) ) ;
#8687=CARTESIAN_POINT ( 'NONE',  ( 12.08790845148079640, 6.355304031620478078, -220.0087475230167229 ) ) ;
#8688=CARTESIAN_POINT ( 'NONE',  ( 12.91815243135930480, 5.607966342865584153, -224.2227256053222959 ) ) ;
#8690=CARTESIAN_POINT ( 'NONE',  ( -13.61368873860109652, -1.873405602088730859, -231.0542245685610112 ) ) ;
#8692=CARTESIAN_POINT ( 'NONE',  ( -13.29422863469367577, -26.11207831950312652, -226.3284374130324750 ) ) ;
#8693=CARTESIAN_POINT ( 'NONE',  ( -21.50655177804914686, 20.61731362457859973, -218.7935603611527426 ) ) ;
#8694=CARTESIAN_POINT ( 'NONE',  ( 7.437838793555467731, -20.85539581353325289, -233.9154700400843865 ) ) ;
#8695=CARTESIAN_POINT ( 'NONE',  ( 2.539761864897490007, 23.64215977235053501, -233.4645566207487661 ) ) ;
#8696=CARTESIAN_POINT ( 'NONE',  ( 17.11616244378571494, -1.720737510755655064, -232.0394440302203236 ) ) ;
#8697=CARTESIAN_POINT ( 'NONE',  ( -22.05223281125454804, 0.4748437386657365367, -217.8785187290425256 ) ) ;
#8698=CARTESIAN_POINT ( 'NONE',  ( 13.06430160593375689, 2.561628050526134182, -220.6026188403641299 ) ) ;
#8699=CARTESIAN_POINT ( 'NONE',  ( -8.791002657293931932, 17.82034842365333205, -218.5247019341474584 ) ) ;
#8700=CARTESIAN_POINT ( 'NONE',  ( 17.23039831256031817, 3.331158952577910615, -216.4027685342793461 ) ) ;
#8702=CARTESIAN_POINT ( 'NONE',  ( 10.57926812561479757, 10.00910231482511215, -225.8341706491384286 ) ) ;
#8703=CARTESIAN_POINT ( 'NONE',  ( 13.17768061945195157, 6.810183613937965674, -219.8302315341053657 ) ) ;
#8704=CARTESIAN_POINT ( 'NONE',  ( -0.1874296312810625753, -16.87674362306512776, -233.1597105263269611 ) ) ;
#8705=CARTESIAN_POINT ( 'NONE',  ( 7.359401564398577733, 15.81697286067417707, -215.8326977948377987 ) ) ;
#8707=CARTESIAN_POINT ( 'NONE',  ( 22.18132842682159733, 5.591149267797686839, -232.0584733989884114 ) ) ;
#8708=CARTESIAN_POINT ( 'NONE',  ( 1.780865994697476307, -30.77012162006053941, -222.8552464324424705 ) ) ;
#8709=CARTESIAN_POINT ( 'NONE',  ( -7.873497077133136735, 15.44270125396616677, -230.2562282217168672 ) ) ;
#8710=CARTESIAN_POINT ( 'NONE',  ( 12.08198696763335178, 15.54678077493410981, -216.6084679670902631 ) ) ;
#8712=CARTESIAN_POINT ( 'NONE',  ( -15.51091956967506391, -1.782849713491490018, -228.8089183834494520 ) ) ;
#8713=CARTESIAN_POINT ( 'NONE',  ( -18.92390258637512090, 12.75887082072172163, -230.9970325548277970 ) ) ;
#8714=CARTESIAN_POINT ( 'NONE',  ( -14.08236938285573636, 6.062428076406559008, -221.7923619418395447 ) ) ;
#8715=CARTESIAN_POINT ( 'NONE',  ( 13.59483335902903178, 5.678732573479117640, -228.5032236586631313 ) ) ;
#8717=CARTESIAN_POINT ( 'NONE',  ( 10.07175337281514871, 14.76776740066196325, -231.7834566702614723 ) ) ;
#8718=CARTESIAN_POINT ( 'NONE',  ( 9.790069677392189362, -14.58761328102826837, -228.7245293813585647 ) ) ;
#8720=CARTESIAN_POINT ( 'NONE',  ( 13.20312407767240614, -7.650902547765872086, -230.0578600405493717 ) ) ;
#8721=CARTESIAN_POINT ( 'NONE',  ( -2.723069588102707606, 15.58614045890443833, -225.0254611642426141 ) ) ;
#8724=CARTESIAN_POINT ( 'NONE',  ( 12.71450444683213021, 7.595266944807587350, -224.4213778964231665 ) ) ;
#8725=CARTESIAN_POINT ( 'NONE',  ( -9.442378551029269929, -6.949684989614740793, -225.4111852319283855 ) ) ;
#8726=CARTESIAN_POINT ( 'NONE',  ( -6.642805165258356404, -28.12267032419628521, -230.9452027245340560 ) ) ;
#8727=CARTESIAN_POINT ( 'NONE',  ( 10.24538335401965661, -11.82980241027587276, -219.3753974371782363 ) ) ;
#8728=CARTESIAN_POINT ( 'NONE',  ( -2.554014161526931392, 17.56271496069470572, -229.4905841158208659 ) ) ;
#8730=CARTESIAN_POINT ( 'NONE',  ( 14.23294950300690331, 6.961167337017927892, -222.0879133937260974 ) ) ;
#8731=CARTESIAN_POINT ( 'NONE',  ( -26.74045434827795020, 12.41518252455047744, -220.4617428697642652 ) ) ;
#8732=CARTESIAN_POINT ( 'NONE',  ( -5.560972518124746244, 14.60655266358653215, -227.5460946431043681 ) ) ;
#8733=CARTESIAN_POINT ( 'NONE',  ( 23.84888352507021736, -3.411310983279423947, -216.3556234003997645 ) ) ;
#8736=CARTESIAN_POINT ( 'NONE',  ( 3.291078285693179950, 23.55624334554876498, -217.3208248278388623 ) ) ;
#8737=CARTESIAN_POINT ( 'NONE',  ( -17.29038495093124084, 2.707785585324113065, -229.0475017805649998 ) ) ;
#8738=CARTESIAN_POINT ( 'NONE',  ( 10.93653298376230687, 10.42959444671468106, -232.5920418140667039 ) ) ;
#8740=CARTESIAN_POINT ( 'NONE',  ( 5.037691872308702301, -15.96383311541683270, -230.0422288358542460 ) ) ;
#8743=CARTESIAN_POINT ( 'NONE',  ( -3.326157069579807946, 13.92020081821418565, -220.5733722327383930 ) ) ;
#8745=CARTESIAN_POINT ( 'NONE',  ( 27.74277644662361197, -2.671700443591659369, -227.2909148725441355 ) ) ;
#8747=CARTESIAN_POINT ( 'NONE',  ( 18.46552355142154411, 5.019711608606525211, -231.5099115070375433 ) ) ;
#8749=CARTESIAN_POINT ( 'NONE',  ( -13.93333636822611155, 3.327141996558931947, -221.4468162587888287 ) ) ;
#8750=CARTESIAN_POINT ( 'NONE',  ( 11.31395536621571019, -8.070181239749643964, -225.0898076798974614 ) ) ;
#8752=CARTESIAN_POINT ( 'NONE',  ( -15.58461825850822180, 18.91734573546571951, -233.7691177939990723 ) ) ;
#8754=CARTESIAN_POINT ( 'NONE',  ( -25.61997837663875188, 10.01664178086244483, -231.6711741719404074 ) ) ;
#8755=CARTESIAN_POINT ( 'NONE',  ( -7.182761810198031505, -27.78193072152378207, -222.3754761716870973 ) ) ;
#8758=CARTESIAN_POINT ( 'NONE',  ( 15.50884165284638705, 1.028647572718199843, -227.8181348745474679 ) ) ;
#8759=CARTESIAN_POINT ( 'NONE',  ( -16.65698539163286540, 11.03290537638306112, -233.6474915129378758 ) ) ;
#8760=CARTESIAN_POINT ( 'NONE',  ( 12.13370821170821223, -20.35915274155448174, -217.8532457648388458 ) ) ;
#8761=CARTESIAN_POINT ( 'NONE',  ( 13.92874801379968730, -1.549146272830121518, -222.4308591964825439 ) ) ;
#8763=CARTESIAN_POINT ( 'NONE',  ( 28.46362550855882745, 7.392895870364313282, -223.4682258299149566 ) ) ;
#8764=CARTESIAN_POINT ( 'NONE',  ( -10.59650102373989533, 7.849913810122476576, -230.0486530042683171 ) ) ;
#8765=CARTESIAN_POINT ( 'NONE',  ( 14.72648027392381387, 10.15511732729369676, -229.5776536674053716 ) ) ;
#8766=CARTESIAN_POINT ( 'NONE',  ( -3.424870747449708652, -17.07003249573819659, -220.0803597572327135 ) ) ;
#8767=CARTESIAN_POINT ( 'NONE',  ( 13.78060503451313323, -0.3076571220309521904, -222.4352540772387101 ) ) ;
#8769=CARTESIAN_POINT ( 'NONE',  ( -1.975202609796049336, 20.81351768191813889, -217.5779402428482001 ) ) ;
#8770=CARTESIAN_POINT ( 'NONE',  ( -13.91323058514953637, 8.006348396443080162, -225.5064972756604220 ) ) ;
#8771=CARTESIAN_POINT ( 'NONE',  ( -22.10934047915441170, 0.9940043559354162506, -215.0000000000000000 ) ) ;
#8773=CARTESIAN_POINT ( 'NONE',  ( -18.84435272498963343, -14.36455033211084498, -230.7675749430951555 ) ) ;
#8778=CARTESIAN_POINT ( 'NONE',  ( 24.81668481317358399, 17.11438712655213124, -222.1096362285750274 ) ) ;
#8779=CARTESIAN_POINT ( 'NONE',  ( 18.69764316139794147, -20.69319383826335823, -224.5905439953889413 ) ) ;
#8780=CARTESIAN_POINT ( 'NONE',  ( 3.449504654906655254, 27.59247159270940841, -231.3461799890608859 ) ) ;
#8781=CARTESIAN_POINT ( 'NONE',  ( -9.250876228778270871, 9.538614635316015722, -227.1332118982684563 ) ) ;
#8782=CARTESIAN_POINT ( 'NONE',  ( 11.17228388010293649, 5.622653638471959425, -222.3672781564363845 ) ) ;
#8784=CARTESIAN_POINT ( 'NONE',  ( 10.02513374692848913, 18.81568788741115128, -217.1505009242214612 ) ) ;
#8786=CARTESIAN_POINT ( 'NONE',  ( 5.451525948382545117, -12.45300865616632713, -227.8545162512558306 ) ) ;
#8787=CARTESIAN_POINT ( 'NONE',  ( 13.91151814069282722, -15.58123622716646572, -216.5183035683795367 ) ) ;
#8791=CARTESIAN_POINT ( 'NONE',  ( -14.63872435137796302, 9.306825831109410530, -216.0000338566471214 ) ) ;
#8792=CARTESIAN_POINT ( 'NONE',  ( -26.10238271615538252, -1.908654064438627174, -220.4792571320490708 ) ) ;
#8793=CARTESIAN_POINT ( 'NONE',  ( 12.47670316482120967, 2.249148913447538423, -227.4574095259895898 ) ) ;
#8794=CARTESIAN_POINT ( 'NONE',  ( 3.378648530876271039, 26.08525450992624428, -218.4319906442508454 ) ) ;
#8795=CARTESIAN_POINT ( 'NONE',  ( 5.466128392039544259, 27.94759090250835243, -223.5617905851570981 ) ) ;
#8796=VERTEX_POINT ( 'NONE', #11541 ) ;
#8797=CARTESIAN_POINT ( 'NONE',  ( 26.96734317869073294, -1.796611605495658681, -216.2358245450472509 ) ) ;
#8798=CARTESIAN_POINT ( 'NONE',  ( 21.53262694368047647, 11.06794636811408594, -231.8394491640143826 ) ) ;
#8799=CARTESIAN_POINT ( 'NONE',  ( -12.26337789213896201, 9.274758280606999250, -219.9806108963443876 ) ) ;
#8800=CARTESIAN_POINT ( 'NONE',  ( -19.58639255110637478, 14.91076398872931819, -217.1105532241463720 ) ) ;
#8801=CARTESIAN_POINT ( 'NONE',  ( -11.55581979318669639, -19.97716813486601239, -217.5317483122086912 ) ) ;
#8802=CARTESIAN_POINT ( 'NONE',  ( -28.17543631911187063, 3.557555778861649642, -230.1980773687482156 ) ) ;
#8805=CARTESIAN_POINT ( 'NONE',  ( 13.54927135793711557, 0.6749664302445949060, -222.0769159577524192 ) ) ;
#8806=CARTESIAN_POINT ( 'NONE',  ( -22.36207348798144778, 17.12313795477538036, -223.8571857210765472 ) ) ;
#8807=CARTESIAN_POINT ( 'NONE',  ( 18.65058977333779211, 24.40868228550881014, -219.3406275662563303 ) ) ;
#8808=CARTESIAN_POINT ( 'NONE',  ( -29.30406754532526037, 5.063969254119831120, -221.8212091093853076 ) ) ;
#8809=CARTESIAN_POINT ( 'NONE',  ( -17.01570095888788003, -2.024181990473361115, -234.1256067144893791 ) ) ;
#8811=CARTESIAN_POINT ( 'NONE',  ( -14.76610802599379291, -3.249507257478274180, -230.1617063156812719 ) ) ;
#8812=CARTESIAN_POINT ( 'NONE',  ( -8.716816145717144693, 12.22834664005217675, -231.7124508691059646 ) ) ;
#8813=CARTESIAN_POINT ( 'NONE',  ( -15.17658589853145479, -26.64966442869902252, -226.8090782225333442 ) ) ;
#8814=CARTESIAN_POINT ( 'NONE',  ( 4.543450689403089271, 15.91052110650461771, -218.9437823786444426 ) ) ;
#8815=CARTESIAN_POINT ( 'NONE',  ( 21.94513595990333954, -23.27941424421253203, -222.2428713697011631 ) ) ;
#8817=CARTESIAN_POINT ( 'NONE',  ( -29.16153046926437753, 6.356672163541281506, -226.4393515956758165 ) ) ;
#8818=CARTESIAN_POINT ( 'NONE',  ( -7.928079932584687128, 26.12067226064367986, -221.2051195461628197 ) ) ;
#8819=CARTESIAN_POINT ( 'NONE',  ( 12.15450584778660570, 2.288537795953278220, -225.7049340319972828 ) ) ;
#8820=CARTESIAN_POINT ( 'NONE',  ( 15.76910524310159900, 5.601482066865847820, -220.3440822020379528 ) ) ;
#8821=CARTESIAN_POINT ( 'NONE',  ( 12.47670316482120967, 2.249148913447538423, -227.4574095259895898 ) ) ;
#8822=CARTESIAN_POINT ( 'NONE',  ( 0.4137397183702169468, -14.31347623323147289, -219.6167997211809393 ) ) ;
#8823=CARTESIAN_POINT ( 'NONE',  ( 7.651502705057454889, 16.60422307457919544, -215.4679461133464144 ) ) ;
#8824=CARTESIAN_POINT ( 'NONE',  ( 20.58703255433590940, 0.4816031003617209372, -231.9427175861361263 ) ) ;
#8825=CARTESIAN_POINT ( 'NONE',  ( 0.8130732720878883768, -26.02312037787507393, -216.7203152272084878 ) ) ;
#8826=CARTESIAN_POINT ( 'NONE',  ( -5.775873073292457249, 17.47547275616994256, -218.7209647771908578 ) ) ;
#8827=CARTESIAN_POINT ( 'NONE',  ( 12.98364502352995942, 13.67380631913144029, -233.1535077318696096 ) ) ;
#8828=CARTESIAN_POINT ( 'NONE',  ( -27.85133024402786006, -1.794102530182491773, -229.4204807338591081 ) ) ;
#8829=CARTESIAN_POINT ( 'NONE',  ( -22.53796032816233463, 16.84148256071415872, -226.0516062466300582 ) ) ;
#8830=CARTESIAN_POINT ( 'NONE',  ( -4.365576370787875859, 13.02741211227440665, -230.2897948137907917 ) ) ;
#8831=CARTESIAN_POINT ( 'NONE',  ( 27.08994772491946890, 9.675875910685000747, -221.3471992134593336 ) ) ;
#8833=CARTESIAN_POINT ( 'NONE',  ( 6.900253619295916963, -14.54306101932516881, -223.7596260804713211 ) ) ;
#8836=CARTESIAN_POINT ( 'NONE',  ( 19.78534257568999166, -22.00365353819481840, -227.2618024355658974 ) ) ;
#8837=CARTESIAN_POINT ( 'NONE',  ( -5.600903697806950632, 21.62055466701630735, -218.6671277943675307 ) ) ;
#8840=CARTESIAN_POINT ( 'NONE',  ( 7.762960416026701616, 12.60702317161859121, -221.9096828323375235 ) ) ;
#8841=CARTESIAN_POINT ( 'NONE',  ( 22.03647168421188240, 0.3315607655626218175, -232.0572713672587213 ) ) ;
#8842=CARTESIAN_POINT ( 'NONE',  ( -1.489322793389167288, -21.37773154815333498, -215.8826219457350817 ) ) ;
#8843=CARTESIAN_POINT ( 'NONE',  ( -1.632242579688942596, -13.62074943359385415, -221.1585305289511041 ) ) ;
#8844=CARTESIAN_POINT ( 'NONE',  ( -3.926352947695993745, 17.69140300707508473, -220.1607884481205986 ) ) ;
#8846=CARTESIAN_POINT ( 'NONE',  ( 23.44063276014420794, 13.61134749381700182, -229.1061940987080732 ) ) ;
#8847=CARTESIAN_POINT ( 'NONE',  ( -7.189383125363055349, 14.28512618638020548, -231.7475838278701303 ) ) ;
#8848=CARTESIAN_POINT ( 'NONE',  ( -6.208492967940078877, 16.71913201805454463, -230.4912298573936766 ) ) ;
#8849=CARTESIAN_POINT ( 'NONE',  ( 2.703362520412529779, 29.60004130108520215, -225.6165589735000481 ) ) ;
#8850=CARTESIAN_POINT ( 'NONE',  ( -19.11923763334766946, 1.257783214997954202, -219.7591028439344711 ) ) ;
#8851=CARTESIAN_POINT ( 'NONE',  ( 18.15173157547545557, 23.32481284044927961, -217.8532150843729482 ) ) ;
#8852=CARTESIAN_POINT ( 'NONE',  ( 6.260833139380572732, -16.02228513277848876, -219.5457089733663736 ) ) ;
#8855=ORIENTED_EDGE ( 'NONE', *, *, #11743, .T. ) ;
#8858=CARTESIAN_POINT ( 'NONE',  ( -10.45786516112131892, 23.61456281964591852, -233.2869923610001592 ) ) ;
#8859=CARTESIAN_POINT ( 'NONE',  ( 23.75342044390781027, -1.773323855525749781, -231.1605140052801630 ) ) ;
#8861=CARTESIAN_POINT ( 'NONE',  ( 20.34032485158648029, 2.741617426884598530, -217.9827731991294968 ) ) ;
#8862=CARTESIAN_POINT ( 'NONE',  ( -29.95012366401462955, 4.746560250930182967, -224.6954343660969471 ) ) ;
#8863=CARTESIAN_POINT ( 'NONE',  ( 5.953549895739506326, -12.70069413479034104, -221.3143591192976203 ) ) ;
#8864=CARTESIAN_POINT ( 'NONE',  ( -7.429838964355703901, 14.87322129099639234, -232.2632863647814077 ) ) ;
#8866=CARTESIAN_POINT ( 'NONE',  ( -25.29098058636142810, 5.014641116111857144, -217.4658967307323110 ) ) ;
#8867=CARTESIAN_POINT ( 'NONE',  ( -7.872599071444734697, -12.17161831996831367, -225.5779045487515191 ) ) ;
#8871=CARTESIAN_POINT ( 'NONE',  ( -13.98136146596813845, 3.850743984385103680, -228.7620665878280590 ) ) ;
#8872=CARTESIAN_POINT ( 'NONE',  ( 13.74877878529187747, -9.499568690286848138, -221.9332727739125346 ) ) ;
#8875=CARTESIAN_POINT ( 'NONE',  ( 17.42772712443221650, 11.35756022693713341, -231.2166398222404382 ) ) ;
#8876=CARTESIAN_POINT ( 'NONE',  ( -5.861205904341304951, 14.21969934012253312, -219.3213214613830644 ) ) ;
#8878=CARTESIAN_POINT ( 'NONE',  ( 13.55451907249704213, 16.71566520821242818, -219.1474322952048226 ) ) ;
#8879=CARTESIAN_POINT ( 'NONE',  ( -0.3443283949127196042, -14.50397496964243516, -224.4114361181996458 ) ) ;
#8880=CARTESIAN_POINT ( 'NONE',  ( 30.27398588404266633, 0.3550328743180605762, -224.9805995843073561 ) ) ;
#8882=CARTESIAN_POINT ( 'NONE',  ( 22.69522586737246783, 3.669837464059151344, -234.0947686933411944 ) ) ;
#8883=CARTESIAN_POINT ( 'NONE',  ( -4.715783688792956063, 28.29821729825949816, -228.0423900005874600 ) ) ;
#8884=CARTESIAN_POINT ( 'NONE',  ( -21.47149190714903710, 3.672831083387290363, -231.0833634068433469 ) ) ;
#8885=CARTESIAN_POINT ( 'NONE',  ( -20.49711526797010208, 7.006997077916217620, -215.3369776077118445 ) ) ;
#8886=CARTESIAN_POINT ( 'NONE',  ( -14.27150057966913721, -8.785576370668652046, -221.5154223125717579 ) ) ;
#8888=ORIENTED_EDGE ( 'NONE', *, *, #8464, .T. ) ;
#8889=CARTESIAN_POINT ( 'NONE',  ( 16.49791052269847569, 3.745513941566326999, -220.1874559167976884 ) ) ;
#8890=CARTESIAN_POINT ( 'NONE',  ( 7.465087220526423373, -26.16405931560015219, -221.3372167714960312 ) ) ;
#8891=CARTESIAN_POINT ( 'NONE',  ( 25.80927844399814930, 11.21489550116160316, -221.3538377621514996 ) ) ;
#8892=CARTESIAN_POINT ( 'NONE',  ( -9.171998067665157350, 9.395241133357435714, -226.3428046914542051 ) ) ;
#8893=CARTESIAN_POINT ( 'NONE',  ( 13.34963947135311102, 7.416462695144936390, -217.9359469527792044 ) ) ;
#8894=CARTESIAN_POINT ( 'NONE',  ( 5.169766346882679997, 29.28517558595074988, -221.5178724947562614 ) ) ;
#8896=CARTESIAN_POINT ( 'NONE',  ( -1.542335193334551491, -19.71915426430242135, -216.1352730594569209 ) ) ;
#8897=CARTESIAN_POINT ( 'NONE',  ( 24.80560757033128993, -15.22139526172250079, -221.3338856610240271 ) ) ;
#8900=CARTESIAN_POINT ( 'NONE',  ( -8.716816145717144693, 12.22834664005217675, -231.7124508691059646 ) ) ;
#8901=CARTESIAN_POINT ( 'NONE',  ( -22.93937586921525806, -8.311597057603599126, -230.3633560851501159 ) ) ;
#8902=CARTESIAN_POINT ( 'NONE',  ( 26.75666476377482539, 8.100664119735744961, -232.1611550320539834 ) ) ;
#8903=CARTESIAN_POINT ( 'NONE',  ( 5.955271202636533090, 21.50135983300913267, -233.0184468368920534 ) ) ;
#8904=CARTESIAN_POINT ( 'NONE',  ( -1.248802714212398968, 14.93471382136348602, -228.4293827518713158 ) ) ;
#8906=CARTESIAN_POINT ( 'NONE',  ( 15.43596206743521826, -16.12492210025319750, -235.0559386399467314 ) ) ;
#8908=CARTESIAN_POINT ( 'NONE',  ( 24.42567939027770407, 10.22651298688739097, -219.4562066833365748 ) ) ;
#8909=CARTESIAN_POINT ( 'NONE',  ( -12.99458409358603284, 11.56864380452031504, -232.0274663316965018 ) ) ;
#8910=CARTESIAN_POINT ( 'NONE',  ( -13.01696012539752445, 9.878799299062107409, -218.8446158128127195 ) ) ;
#8911=CARTESIAN_POINT ( 'NONE',  ( -30.29980174031923923, -2.072322947205907706, -221.9291348703773679 ) ) ;
#8912=CARTESIAN_POINT ( 'NONE',  ( -9.151299407007059017, 9.196974979111923076, -223.9483834032048719 ) ) ;
#8915=CARTESIAN_POINT ( 'NONE',  ( 13.10956039622986324, 4.581323766968698585, -221.0328522389722252 ) ) ;
#8916=CARTESIAN_POINT ( 'NONE',  ( -9.852301241816233457, 15.10013604187968461, -230.8124578431014697 ) ) ;
#8917=CARTESIAN_POINT ( 'NONE',  ( 8.681721411120292942, 8.442847255497570202, -228.0516816418615065 ) ) ;
#8919=CARTESIAN_POINT ( 'NONE',  ( -16.20072894238734307, 0.5024448614660336210, -230.4554067149722130 ) ) ;
#8920=CARTESIAN_POINT ( 'NONE',  ( -12.58473846644578664, -2.158129970029659006, -220.6199603830026206 ) ) ;
#8921=CARTESIAN_POINT ( 'NONE',  ( -13.83093441725390704, -7.146379636134302160, -230.0501880019394605 ) ) ;
#8922=CARTESIAN_POINT ( 'NONE',  ( -9.350291727197115321, 27.53754332352430367, -230.1504993026967441 ) ) ;
#8923=CARTESIAN_POINT ( 'NONE',  ( -3.734153817218577309, -19.72686645808614614, -233.9207428641194610 ) ) ;
#8924=CARTESIAN_POINT ( 'NONE',  ( 5.017623471397871349, 29.83561274492976878, -222.9769172135417250 ) ) ;
#8925=CARTESIAN_POINT ( 'NONE',  ( 4.248462565232024701, -14.07263755978623188, -232.0081791469470716 ) ) ;
#8927=CARTESIAN_POINT ( 'NONE',  ( -29.22672729369577738, 6.588740615114764054, -224.9915299386302934 ) ) ;
#8928=CARTESIAN_POINT ( 'NONE',  ( 0.9458336400950161371, 17.49535648476021876, -228.8359568483051589 ) ) ;
#8929=CARTESIAN_POINT ( 'NONE',  ( 13.71882454279727526, 6.278400000045776252, -230.2269611870541723 ) ) ;
#8930=CARTESIAN_POINT ( 'NONE',  ( 21.53262694368047647, 11.06794636811408594, -231.8394491640143826 ) ) ;
#8931=CARTESIAN_POINT ( 'NONE',  ( 22.16968511661519869, 1.542591969257184337, -234.6098499860488573 ) ) ;
#8932=CARTESIAN_POINT ( 'NONE',  ( -9.869267615102224056, -25.54258770546914903, -218.7733540664615930 ) ) ;
#8933=CARTESIAN_POINT ( 'NONE',  ( 6.812728368504421539, 14.35307019806973194, -216.7766581591129977 ) ) ;
#8935=CARTESIAN_POINT ( 'NONE',  ( 2.018545692720245643, -30.97649562252411215, -224.4812544443210811 ) ) ;
#8936=CARTESIAN_POINT ( 'NONE',  ( -9.810154340578240095, 25.84808829058669488, -220.5759521898573610 ) ) ;
#8937=CARTESIAN_POINT ( 'NONE',  ( 6.040050017043670394, 13.67534390435379699, -220.4759402345340504 ) ) ;
#8938=CARTESIAN_POINT ( 'NONE',  ( -27.09167109716269550, -0.2825935922571593539, -219.8389404328913486 ) ) ;
#8939=CARTESIAN_POINT ( 'NONE',  ( -15.95412330064426065, 13.09400588185824077, -218.6613039563597169 ) ) ;
#8942=CARTESIAN_POINT ( 'NONE',  ( -13.24620988741752825, 28.78239319002125285, -225.3527830703614256 ) ) ;
#8943=CARTESIAN_POINT ( 'NONE',  ( 22.42095341476093040, 9.457779162868732215, -232.6339572190428555 ) ) ;
#8945=CARTESIAN_POINT ( 'NONE',  ( 15.57652300565637482, -15.79620443381692496, -231.0117242343698081 ) ) ;
#8946=CARTESIAN_POINT ( 'NONE',  ( 17.47229821656412341, -21.26691171910925249, -219.4940788861217413 ) ) ;
#8947=CARTESIAN_POINT ( 'NONE',  ( -2.993956627714193353, 22.04778837082692178, -231.1741803919495339 ) ) ;
#8950=CARTESIAN_POINT ( 'NONE',  ( 10.83706092800007781, 10.12544885278926543, -227.1716144446442343 ) ) ;
#8951=CARTESIAN_POINT ( 'NONE',  ( -27.06886705769815649, 1.548837563602061262, -218.3554811309518868 ) ) ;
#8952=CARTESIAN_POINT ( 'NONE',  ( -24.92024473536680773, -13.74570206812420103, -220.1598944320903115 ) ) ;
#8953=CARTESIAN_POINT ( 'NONE',  ( -2.576162127940193169, -15.57202066281789321, -231.6911579627040396 ) ) ;
#8954=CARTESIAN_POINT ( 'NONE',  ( 0.1979841192334154676, 16.22068729745496540, -223.9539336445596973 ) ) ;
#8956=CARTESIAN_POINT ( 'NONE',  ( 25.01541028746040141, 13.78427203520734423, -225.9266837950359843 ) ) ;
#8957=CARTESIAN_POINT ( 'NONE',  ( -3.060450601941519189, 13.29454208326677289, -222.0135664617158682 ) ) ;
#8958=CARTESIAN_POINT ( 'NONE',  ( -6.573387563318148885, 17.69612765735440973, -231.1211991061559274 ) ) ;
#8959=CARTESIAN_POINT ( 'NONE',  ( 2.785859284650920031, 14.19821255961969619, -226.9946081512528906 ) ) ;
#8960=CARTESIAN_POINT ( 'NONE',  ( -16.27736488614644372, 5.941157768540612949, -228.4237983497913547 ) ) ;
#8961=CARTESIAN_POINT ( 'NONE',  ( 29.64577750251057608, 2.839131411071813549, -220.9704389295326905 ) ) ;
#8962=CARTESIAN_POINT ( 'NONE',  ( 5.511302051500400090, -18.01881380728196902, -231.5522404100356084 ) ) ;
#8963=CARTESIAN_POINT ( 'NONE',  ( 13.63685685255378743, 0.3474052042451960531, -228.2001920571242124 ) ) ;
#8965=CARTESIAN_POINT ( 'NONE',  ( 7.168644370073567806, 19.32044210858112265, -233.1278450877711634 ) ) ;
#8966=CARTESIAN_POINT ( 'NONE',  ( 17.78543650172321833, -3.538499054913423869, -220.4382406111031401 ) ) ;
#8968=CARTESIAN_POINT ( 'NONE',  ( 18.76922974182421555, 13.12635134380198210, -217.8010375391909008 ) ) ;
#8969=CARTESIAN_POINT ( 'NONE',  ( 8.257114973007913861, -25.39836461225790742, -232.6217252414676295 ) ) ;
#8971=CARTESIAN_POINT ( 'NONE',  ( -15.66530208164916260, 23.23467148471576849, -218.1250122661128046 ) ) ;
#8973=CARTESIAN_POINT ( 'NONE',  ( -19.18087294808806931, 21.32275554655070593, -230.8558978902391061 ) ) ;
#8975=CARTESIAN_POINT ( 'NONE',  ( -13.69675006931110417, 3.702342960760605539, -228.0723273272095355 ) ) ;
#8976=CARTESIAN_POINT ( 'NONE',  ( -11.55581979318669639, -19.97716813486601239, -217.5317483122086912 ) ) ;
#8979=CARTESIAN_POINT ( 'NONE',  ( -13.69675006931110417, 3.702342960760605539, -228.0723273272095355 ) ) ;
#8980=CARTESIAN_POINT ( 'NONE',  ( 3.247425482496454130, -26.49846316390620160, -232.4805733197358677 ) ) ;
#8984=CARTESIAN_POINT ( 'NONE',  ( 22.37742875470728876, 11.29804624588327577, -218.9256858961603882 ) ) ;
#8985=CARTESIAN_POINT ( 'NONE',  ( -21.50655177804914686, 20.61731362457859973, -218.7935603611527426 ) ) ;
#8987=CARTESIAN_POINT ( 'NONE',  ( 25.01541028746040141, 13.78427203520734423, -225.9266837950359843 ) ) ;
#8988=CARTESIAN_POINT ( 'NONE',  ( 2.219167932009094901, -23.00164214691015729, -217.1940376169840476 ) ) ;
#8990=CARTESIAN_POINT ( 'NONE',  ( -4.067324790461362305, 15.10342260507846746, -228.2464404076259257 ) ) ;
#8991=CARTESIAN_POINT ( 'NONE',  ( -13.58070052954164275, 11.19572749768420650, -220.2511552028196604 ) ) ;
#8992=CARTESIAN_POINT ( 'NONE',  ( 15.58465056415575312, 2.812367138262562349, -229.5090343034091234 ) ) ;
#8993=CARTESIAN_POINT ( 'NONE',  ( -15.14636561941736481, -8.091785236158230532, -228.8632199501622608 ) ) ;
#8996=CARTESIAN_POINT ( 'NONE',  ( 23.83082175545800752, 15.77842900014857896, -219.5351905769044834 ) ) ;
#8997=CARTESIAN_POINT ( 'NONE',  ( 6.629309777743229937, -15.42610274396934855, -227.9597969125812256 ) ) ;
#8998=CARTESIAN_POINT ( 'NONE',  ( 22.66390650824515873, 11.48342577402021725, -231.3155567808436217 ) ) ;
#8999=CARTESIAN_POINT ( 'NONE',  ( -22.99617382825321599, 17.18101613848176967, -230.9512687019100099 ) ) ;
#9000=CARTESIAN_POINT ( 'NONE',  ( 17.96045420455031305, -0.3746358454349600908, -217.9627609769914613 ) ) ;
#9001=CARTESIAN_POINT ( 'NONE',  ( 0.9908753270255351575, 13.79205759140780430, -228.0165926715089881 ) ) ;
#9002=CARTESIAN_POINT ( 'NONE',  ( 13.39702356564321306, 1.314794804900859537, -222.2999924150924187 ) ) ;
#9003=CARTESIAN_POINT ( 'NONE',  ( -7.531388159411753769, -21.98719092781708540, -216.0713624712111312 ) ) ;
#9004=CARTESIAN_POINT ( 'NONE',  ( 12.31511859722645852, -8.491226738247512174, -220.9006323875693738 ) ) ;
#9006=DIRECTION ( 'NONE',  ( 0.000000000000000000, 0.000000000000000000, -1.000000000000000000 ) ) ;
#9007=CARTESIAN_POINT ( 'NONE',  ( -7.686214453470440411, 10.71593237010305444, -228.8058998235944159 ) ) ;
#9008=CARTESIAN_POINT ( 'NONE',  ( -18.92071285517992507, -7.235402657652117320, -230.6453433565968680 ) ) ;
#9009=CARTESIAN_POINT ( 'NONE',  ( -12.62195384480319582, 9.244619650382723819, -228.6283004876635516 ) ) ;
#9010=CARTESIAN_POINT ( 'NONE',  ( 8.860681144154234801, 27.11956268701432293, -229.8503778060109823 ) ) ;
#9011=CARTESIAN_POINT ( 'NONE',  ( -0.7292515499105728383, 28.18841485102515776, -220.8637599502617093 ) ) ;
#9013=CARTESIAN_POINT ( 'NONE',  ( 26.46513128492211564, -16.79977778982552650, -229.3906297761492681 ) ) ;
#9015=CARTESIAN_POINT ( 'NONE',  ( 13.03557269046774714, 7.519834803053426775, -226.9490612297269081 ) ) ;
#9016=CARTESIAN_POINT ( 'NONE',  ( -11.40916210110096962, 20.01996232974788725, -234.3205435716851923 ) ) ;
#9017=CARTESIAN_POINT ( 'NONE',  ( -16.09559989144903369, 12.31939076846282966, -216.7948290530243298 ) ) ;
#9018=CARTESIAN_POINT ( 'NONE',  ( -15.92941692657317354, -7.780888323563449838, -232.0381278758927976 ) ) ;
#9019=ADVANCED_FACE ( 'NONE', ( #9640 ), #5402, .F. ) ;
#9020=CARTESIAN_POINT ( 'NONE',  ( -17.79285498209129202, 9.187865686019035749, -216.3798185811636756 ) ) ;
#9021=CLOSED_SHELL ( 'NONE', ( #15347, #18775, #11417, #1620, #9019, #12924, #6565, #19148, #11460, #16952 ) ) ;
#9024=CARTESIAN_POINT ( 'NONE',  ( 12.25122766587143630, 4.035812653434439845, -225.7709573147497224 ) ) ;
#9025=CARTESIAN_POINT ( 'NONE',  ( -9.969679877803788060, 12.84542071557917176, -220.4758784541224657 ) ) ;
#9026=CARTESIAN_POINT ( 'NONE',  ( 19.48863273024974418, 12.80680990455712909, -215.0408095016468053 ) ) ;
#9027=CARTESIAN_POINT ( 'NONE',  ( -13.98136146596813845, 3.850743984385103680, -228.7620665878280590 ) ) ;
#9028=CARTESIAN_POINT ( 'NONE',  ( -20.48546531633906298, -12.23885716989380157, -214.8851912114337210 ) ) ;
#9029=CARTESIAN_POINT ( 'NONE',  ( -30.29980174031923923, -2.072322947205907706, -221.9291348703773679 ) ) ;
#9030=CARTESIAN_POINT ( 'NONE',  ( 2.482746429915354547, 16.41797261123590346, -229.5599230346982154 ) ) ;
#9031=CARTESIAN_POINT ( 'NONE',  ( -6.870552667427666904, -18.85419487977974029, -216.2130481585807047 ) ) ;
#9032=CARTESIAN_POINT ( 'NONE',  ( 12.04687593227112430, 27.54339840196571743, -224.6466266724203820 ) ) ;
#9033=CARTESIAN_POINT ( 'NONE',  ( 11.86117213253061387, -14.68998886196529874, -215.0859965227146802 ) ) ;
#9035=CARTESIAN_POINT ( 'NONE',  ( -18.14952719657095415, 1.368063294522122275, -218.0005379682515922 ) ) ;
#9037=CARTESIAN_POINT ( 'NONE',  ( -2.532302712337851425, 16.54370602006230939, -228.1940632970506613 ) ) ;
#9038=CARTESIAN_POINT ( 'NONE',  ( 16.48801037644500056, 3.165716804515234628, -216.8169430726136113 ) ) ;
#9039=CARTESIAN_POINT ( 'NONE',  ( 26.24002132888527328, 11.62331517472360964, -222.5300873157218859 ) ) ;
#9040=CARTESIAN_POINT ( 'NONE',  ( 24.20411255886326529, 12.66254860825103634, -218.0144359054998802 ) ) ;
#9041=CARTESIAN_POINT ( 'NONE',  ( -5.646690751453034451, -19.25001164140187981, -233.5706237494638913 ) ) ;
#9042=CARTESIAN_POINT ( 'NONE',  ( 2.804048525646705148, 30.59371477727813726, -220.6614663749232363 ) ) ;
#9044=CARTESIAN_POINT ( 'NONE',  ( -4.398080837965281376, -27.92536303359771566, -232.3360949592949112 ) ) ;
#9045=CARTESIAN_POINT ( 'NONE',  ( -4.691002462566371101, 21.98518063340150164, -232.2516024630330094 ) ) ;
#9046=CARTESIAN_POINT ( 'NONE',  ( 15.26539804565921621, 9.309431686815628382, -232.9129599938668207 ) ) ;
#9047=CARTESIAN_POINT ( 'NONE',  ( -12.69709334397052203, 10.59859500067950400, -221.6107941937004568 ) ) ;
#9048=CARTESIAN_POINT ( 'NONE',  ( -4.378220565073127624, 31.53459173284372952, -222.0564199190954753 ) ) ;
#9049=CARTESIAN_POINT ( 'NONE',  ( 26.53121369294028042, 10.74560293343441586, -229.2288136770759195 ) ) ;
#9050=CARTESIAN_POINT ( 'NONE',  ( 18.44909377000590922, -20.66544815256419199, -223.5047567001167863 ) ) ;
#9052=CARTESIAN_POINT ( 'NONE',  ( 7.876378987416962296, -12.17572650474792617, -223.4643623724329018 ) ) ;
#9053=CARTESIAN_POINT ( 'NONE',  ( -5.706122936196527107, 15.14201253431006045, -228.6865785740211550 ) ) ;
#9057=CARTESIAN_POINT ( 'NONE',  ( 17.97843143658897347, 22.12221935793617078, -220.9346589834416079 ) ) ;
#9058=CARTESIAN_POINT ( 'NONE',  ( 28.33476664927451338, -0.7768526459456059907, -228.3750448408243869 ) ) ;
#9059=CARTESIAN_POINT ( 'NONE',  ( -14.76273180397945772, -6.370707202906876532, -220.0066229284273334 ) ) ;
#9060=CARTESIAN_POINT ( 'NONE',  ( 2.378655016347637652, -14.31292064579845302, -219.9942319014987220 ) ) ;
#9061=CARTESIAN_POINT ( 'NONE',  ( -1.158668551263366986, 23.31492692626720853, -219.2372600964201865 ) ) ;
#9063=CARTESIAN_POINT ( 'NONE',  ( 27.30736127486511577, 7.960716467858479639, -228.6121938484450595 ) ) ;
#9064=CARTESIAN_POINT ( 'NONE',  ( -18.47334320050258327, 24.79293862780133040, -226.9986786077537317 ) ) ;
#9065=CARTESIAN_POINT ( 'NONE',  ( -11.11821474075380678, 16.53100589793018926, -232.3736596382188395 ) ) ;
#9067=CARTESIAN_POINT ( 'NONE',  ( 7.213476267053916757, 16.78447451494783138, -217.5857052077849687 ) ) ;
#9068=CARTESIAN_POINT ( 'NONE',  ( -21.18474081038989354, 8.486062504918864491, -230.7949373529753530 ) ) ;
#9069=CARTESIAN_POINT ( 'NONE',  ( 21.06229272850552547, 3.434461253538921621, -234.1452885155528918 ) ) ;
#9070=CARTESIAN_POINT ( 'NONE',  ( 9.020349274477036161, -13.22217574948208529, -220.4173403795374213 ) ) ;
#9073=CARTESIAN_POINT ( 'NONE',  ( 4.883314309504700468, 19.06839645569368358, -217.0171359871271193 ) ) ;
#9074=CARTESIAN_POINT ( 'NONE',  ( 25.63739587761438088, -9.098054415140415685, -222.2988516439644968 ) ) ;
#9077=CARTESIAN_POINT ( 'NONE',  ( 21.31262902390056624, 0.4111834581965390645, -232.0572713672585792 ) ) ;
#9078=CARTESIAN_POINT ( 'NONE',  ( 0.7326557587344989519, -29.96088689026728602, -229.4725774697800205 ) ) ;
#9080=CARTESIAN_POINT ( 'NONE',  ( -20.18153419852512442, 14.25141268122526483, -233.5059133483111964 ) ) ;
#9081=CARTESIAN_POINT ( 'NONE',  ( -16.28135616697389310, 20.98764039357472200, -216.9434553755565958 ) ) ;
#9082=CARTESIAN_POINT ( 'NONE',  ( -14.87984907657228639, 0.2138881189739126887, -228.7773920408832282 ) ) ;
#9083=CARTESIAN_POINT ( 'NONE',  ( -12.35609710479046441, -10.83622032031252758, -230.4552079900997228 ) ) ;
#9085=CARTESIAN_POINT ( 'NONE',  ( -27.90314475660494153, 12.48829126175061077, -223.3300566725355338 ) ) ;
#9086=CARTESIAN_POINT ( 'NONE',  ( 9.500235314199413139, -15.98409598254677455, -218.3811512014305265 ) ) ;
#9091=CARTESIAN_POINT ( 'NONE',  ( 16.23850682336481199, 8.051046992137072422, -219.2473483181185827 ) ) ;
#9092=CARTESIAN_POINT ( 'NONE',  ( -7.626320092023432196, 21.25423560278784407, -233.8867968595558295 ) ) ;
#9094=CARTESIAN_POINT ( 'NONE',  ( 12.60818910183731489, 13.02403301690871729, -229.3305689548085695 ) ) ;
#9095=CARTESIAN_POINT ( 'NONE',  ( -6.479026444546563290, -23.11309618162032820, -231.4158670874050756 ) ) ;
#9097=CARTESIAN_POINT ( 'NONE',  ( -5.365396334125453137, 16.47374957271378904, -219.4721119688156534 ) ) ;
#9098=CARTESIAN_POINT ( 'NONE',  ( -17.65560862077320081, 21.92186454631220371, -221.3776075196718693 ) ) ;
#9099=CARTESIAN_POINT ( 'NONE',  ( -31.12406087576577463, 7.316399946619934092, -225.0171288978685027 ) ) ;
#9101=CARTESIAN_POINT ( 'NONE',  ( -17.99186107021003167, -20.03292934477192944, -228.1636640080403424 ) ) ;
#9103=VERTEX_POINT ( 'NONE', #18726 ) ;
#9104=CARTESIAN_POINT ( 'NONE',  ( -28.59157645096996347, 5.137867505054540374, -220.4667042235044505 ) ) ;
#9105=CARTESIAN_POINT ( 'NONE',  ( 7.724698117049915602, -20.76727510557136469, -231.0612438369181518 ) ) ;
#9106=CARTESIAN_POINT ( 'NONE',  ( 17.00168025137501004, 6.212099629982537508, -219.0548246536471595 ) ) ;
#9107=CARTESIAN_POINT ( 'NONE',  ( 4.883314309504700468, 19.06839645569368358, -217.0171359871271193 ) ) ;
#9111=CARTESIAN_POINT ( 'NONE',  ( -21.16281446184100545, 3.810576631694648775, -218.4455094643457187 ) ) ;
#9112=CARTESIAN_POINT ( 'NONE',  ( 8.329997790135040603, 12.51216704542961899, -228.7022893680961602 ) ) ;
#9114=CARTESIAN_POINT ( 'NONE',  ( -6.052919920376759855, -15.38051382379660836, -218.0337201863237624 ) ) ;
#9115=CARTESIAN_POINT ( 'NONE',  ( 18.55298002304457228, -12.22359628793950570, -216.9137843736221782 ) ) ;
#9118=CARTESIAN_POINT ( 'NONE',  ( -11.10150084103673684, 3.549415896002023896, -226.0408865487038952 ) ) ;
#9119=CARTESIAN_POINT ( 'NONE',  ( -22.88587990158785601, -12.52061884883742238, -220.5813279352508687 ) ) ;
#9122=CARTESIAN_POINT ( 'NONE',  ( -18.94992041651601156, 14.87246523864368974, -232.0280096192260828 ) ) ;
#9123=CARTESIAN_POINT ( 'NONE',  ( 13.48097272627202159, 8.509510470709432894, -231.5257201610278059 ) ) ;
#9124=CARTESIAN_POINT ( 'NONE',  ( -1.582540545905128049, 14.52388882916313584, -222.9138157219475147 ) ) ;
#9126=CARTESIAN_POINT ( 'NONE',  ( 15.68748001070188458, -20.89997441943167900, -216.2583427777263125 ) ) ;
#9128=CARTESIAN_POINT ( 'NONE',  ( 14.32085100525799248, 9.220655089380342062, -219.9006227404039464 ) ) ;
#9129=CARTESIAN_POINT ( 'NONE',  ( -5.340143745732740754, 22.10628181454592678, -235.0476201740528097 ) ) ;
#9130=CARTESIAN_POINT ( 'NONE',  ( -8.123851230256436295, 20.56863949923577550, -215.0796075421103239 ) ) ;
#9131=CARTESIAN_POINT ( 'NONE',  ( -12.88620494227545343, -3.269292211592822461, -225.1464181993036391 ) ) ;
#9132=CARTESIAN_POINT ( 'NONE',  ( -11.67631226053870996, 6.737291529340801333, -227.3110382950315227 ) ) ;
#9137=CARTESIAN_POINT ( 'NONE',  ( -12.69709334397052203, 10.59859500067950400, -221.6107941937004568 ) ) ;
#9138=CARTESIAN_POINT ( 'NONE',  ( 18.50073117969547098, -1.889592114545683987, -232.6396648696776026 ) ) ;
#9139=CARTESIAN_POINT ( 'NONE',  ( -15.15110768032078070, 3.517015312212880218, -219.5479300368539270 ) ) ;
#9141=CARTESIAN_POINT ( 'NONE',  ( 11.57669841200422134, 10.63052136557218574, -228.9489978335593889 ) ) ;
#9142=CARTESIAN_POINT ( 'NONE',  ( -22.25980993584449408, -3.522148912989541802, -233.7954546715351398 ) ) ;
#9144=CARTESIAN_POINT ( 'NONE',  ( 1.313727069624702981, 17.80710275190598324, -219.4197901500037062 ) ) ;
#9145=CARTESIAN_POINT ( 'NONE',  ( -6.512931564893298386, -17.32529878264574563, -216.7284160531958719 ) ) ;
#9146=CARTESIAN_POINT ( 'NONE',  ( 17.19674704922021391, 23.07334190050143974, -228.8256488842130238 ) ) ;
#9147=CARTESIAN_POINT ( 'NONE',  ( 7.117641012966415381, -28.94820313438933113, -231.4073019955615393 ) ) ;
#9149=CARTESIAN_POINT ( 'NONE',  ( -14.94667331530454213, 6.325011500478772142, -230.0242139990887154 ) ) ;
#9150=CARTESIAN_POINT ( 'NONE',  ( 15.07245478799217686, -4.018468087397350175, -231.0118529037252699 ) ) ;
#9151=CARTESIAN_POINT ( 'NONE',  ( 7.804112641607792611, 19.76858558208418515, -218.6463059509973164 ) ) ;
#9152=CARTESIAN_POINT ( 'NONE',  ( -16.81936022032888545, 5.700806722825413786, -218.5726178058217215 ) ) ;
#9153=CARTESIAN_POINT ( 'NONE',  ( 20.58703255433590940, 0.4816031003617209372, -231.9427175861361263 ) ) ;
#9154=CARTESIAN_POINT ( 'NONE',  ( -11.33724117040414647, -11.57131516804904159, -228.9094961685112537 ) ) ;
#9156=CARTESIAN_POINT ( 'NONE',  ( 14.75291830987536557, 13.43762972591284033, -235.1407057970265839 ) ) ;
#9159=CARTESIAN_POINT ( 'NONE',  ( -3.456580335739853016, -11.82839499582713749, -226.8096787805597501 ) ) ;
#9160=CARTESIAN_POINT ( 'NONE',  ( -8.030397104878142400, 15.90963402996711373, -230.6518438502475590 ) ) ;
#9161=CARTESIAN_POINT ( 'NONE',  ( 8.821742718405863215, 10.82866050966069160, -221.4785132813277642 ) ) ;
#9162=CARTESIAN_POINT ( 'NONE',  ( -14.20363567091065349, 7.857660128015216294, -223.4151327167956822 ) ) ;
#9163=CARTESIAN_POINT ( 'NONE',  ( -10.30034651166687887, 25.05454868506992838, -216.5587736482213188 ) ) ;
#9164=CARTESIAN_POINT ( 'NONE',  ( 14.21126657910812874, 6.833562750302326627, -220.2783117037562874 ) ) ;
#9166=CARTESIAN_POINT ( 'NONE',  ( 10.74448773353722686, -20.82765299830942851, -219.2305132457354659 ) ) ;
#9168=CARTESIAN_POINT ( 'NONE',  ( 9.009845654114897684, -15.13764346805314354, -231.2790349225496129 ) ) ;
#9169=CARTESIAN_POINT ( 'NONE',  ( -5.764806379010653181, 14.19340719117484007, -223.8851086052821415 ) ) ;
#9173=CARTESIAN_POINT ( 'NONE',  ( 27.40550551777678123, 5.967061366481472895, -228.7463788799179554 ) ) ;
#9174=CARTESIAN_POINT ( 'NONE',  ( 23.12216041205843453, 0.2121350054995089496, -232.0572713672589202 ) ) ;
#9175=CARTESIAN_POINT ( 'NONE',  ( -15.27057301462635408, -17.00912219741827514, -233.6288396447818627 ) ) ;
#9176=CARTESIAN_POINT ( 'NONE',  ( -7.531388159411753769, -21.98719092781708540, -216.0713624712111312 ) ) ;
#9177=CARTESIAN_POINT ( 'NONE',  ( 9.094331215210646135, 23.85463374792894342, -219.7669638091879847 ) ) ;
#9179=CARTESIAN_POINT ( 'NONE',  ( -29.98527381603928887, 6.316825171121390525, -230.1108345570740994 ) ) ;
#9180=CARTESIAN_POINT ( 'NONE',  ( -9.749377714296398878, 10.28442384816749922, -229.3722863967025205 ) ) ;
#9181=CARTESIAN_POINT ( 'NONE',  ( 3.528957931946373971, 27.43889307663531696, -223.4805233499528185 ) ) ;
#9183=CARTESIAN_POINT ( 'NONE',  ( 5.833753951408669813, 12.47745132051510453, -226.2508980627489450 ) ) ;
#9184=CARTESIAN_POINT ( 'NONE',  ( -24.48812334466693486, 4.469247780253509106, -230.3044243311433945 ) ) ;
#9185=CARTESIAN_POINT ( 'NONE',  ( 12.08790845148079640, 6.355304031620478078, -220.0087475230167229 ) ) ;
#9186=CARTESIAN_POINT ( 'NONE',  ( 10.46316887740464985, -17.92901728017801233, -232.6108895528913081 ) ) ;
#9189=CARTESIAN_POINT ( 'NONE',  ( 8.812073984913094904, 13.12649198322903210, -229.9172071780580495 ) ) ;
#9190=CARTESIAN_POINT ( 'NONE',  ( -22.13988250630526267, 1.271659148212506141, -215.1660654604927458 ) ) ;
#9194=CARTESIAN_POINT ( 'NONE',  ( 15.60497028854143764, -26.39208911975253002, -225.8550158017044112 ) ) ;
#9195=CARTESIAN_POINT ( 'NONE',  ( -9.250876228778270871, 9.538614635316015722, -227.1332118982684563 ) ) ;
#9196=CARTESIAN_POINT ( 'NONE',  ( -8.005900519654911562, 11.01772743098285545, -228.7074549843708269 ) ) ;
#9198=CARTESIAN_POINT ( 'NONE',  ( -8.966714183099560032, 19.05224306381768073, -234.0879867025980445 ) ) ;
#9199=CARTESIAN_POINT ( 'NONE',  ( -7.786003226018990198, -12.23758553950863082, -224.1954257758910671 ) ) ;
#9203=CARTESIAN_POINT ( 'NONE',  ( -10.84997096467605182, 25.01800101807719301, -232.4518260228253155 ) ) ;
#9204=CARTESIAN_POINT ( 'NONE',  ( 4.150966869518468272, -13.66845483776041092, -221.7292245539943565 ) ) ;
#9206=CARTESIAN_POINT ( 'NONE',  ( -17.39699619235753048, 15.64332637722790054, -216.0406373264262641 ) ) ;
#9207=CARTESIAN_POINT ( 'NONE',  ( 13.17424634425744046, 10.51488364724239588, -221.4616598107521099 ) ) ;
#9208=CARTESIAN_POINT ( 'NONE',  ( -16.58369694688956741, 24.75758513462668375, -230.3405478298966784 ) ) ;
#9210=CARTESIAN_POINT ( 'NONE',  ( -18.09994298044773942, 1.383435435878707320, -215.7801353739235708 ) ) ;
#9211=CARTESIAN_POINT ( 'NONE',  ( -11.04629350503636864, -16.47921676447750983, -219.6257371594006145 ) ) ;
#9214=CARTESIAN_POINT ( 'NONE',  ( -7.250603130619442283, 20.89725557392719324, -217.7893896917081520 ) ) ;
#9215=CARTESIAN_POINT ( 'NONE',  ( -8.316505849089994129, 18.84563905716333210, -217.0138378867507640 ) ) ;
#9216=CARTESIAN_POINT ( 'NONE',  ( -13.44241955326339166, 15.88952131657459965, -217.2587743382015901 ) ) ;
#9217=CARTESIAN_POINT ( 'NONE',  ( -10.71434429704389046, -13.39337408441371124, -228.3296939239235428 ) ) ;
#9220=CARTESIAN_POINT ( 'NONE',  ( -20.43618815875133521, 1.403378831510147196, -232.9646741665398224 ) ) ;
#9221=CARTESIAN_POINT ( 'NONE',  ( 6.477082923917054202, -23.79794467951758108, -219.1375485160026813 ) ) ;
#9222=CARTESIAN_POINT ( 'NONE',  ( 15.85665641241444668, 18.24713744004561988, -217.7195292979064902 ) ) ;
#9223=CARTESIAN_POINT ( 'NONE',  ( 5.343558017910363667, 26.29639771561252459, -218.1010331760174665 ) ) ;
#9226=CARTESIAN_POINT ( 'NONE',  ( -25.48569860171343748, 4.299098795181173216, -219.7804659532078801 ) ) ;
#9227=CARTESIAN_POINT ( 'NONE',  ( 16.11883106748507188, 21.48229216499086291, -233.4985352728212433 ) ) ;
#9229=CARTESIAN_POINT ( 'NONE',  ( 15.89706143421296147, 10.57416387607782227, -218.3862415393350318 ) ) ;
#9230=CARTESIAN_POINT ( 'NONE',  ( 13.66960652149700728, 1.853972107162461080, -222.6386165551958811 ) ) ;
#9231=CARTESIAN_POINT ( 'NONE',  ( -19.50907964299920039, -17.77536300509877876, -217.8007844881196320 ) ) ;
#9232=CARTESIAN_POINT ( 'NONE',  ( 6.166782020495575445, -26.61202787628535660, -217.6604608484729795 ) ) ;
#9233=CARTESIAN_POINT ( 'NONE',  ( -21.94776718874820176, -0.4748437386657589632, -216.1214812709574176 ) ) ;
#9235=CARTESIAN_POINT ( 'NONE',  ( -26.12939716039095117, 11.33146045174629357, -233.1192402782019997 ) ) ;
#9236=CARTESIAN_POINT ( 'NONE',  ( -17.04360437375341419, -3.174793268193519591, -228.4680687138289841 ) ) ;
#9237=CARTESIAN_POINT ( 'NONE',  ( -14.94667331530454213, 6.325011500478772142, -230.0242139990887154 ) ) ;
#9238=CARTESIAN_POINT ( 'NONE',  ( 16.10596270516584028, 24.75152718569329835, -228.9330127594856492 ) ) ;
#9239=CARTESIAN_POINT ( 'NONE',  ( 16.49020573214642837, 22.44566021525517741, -224.7841662740084701 ) ) ;
#9241=CARTESIAN_POINT ( 'NONE',  ( 17.10065829945946092, -7.211672327051211084, -215.1948405133616404 ) ) ;
#9242=CARTESIAN_POINT ( 'NONE',  ( 15.05360126642391450, 1.481754003466396963, -222.9454997252120734 ) ) ;
#9243=CARTESIAN_POINT ( 'NONE',  ( 3.044038000507106378, 30.22621415828681180, -231.1553244844465382 ) ) ;
#9244=CARTESIAN_POINT ( 'NONE',  ( -19.18087294808806931, 21.32275554655070593, -230.8558978902391061 ) ) ;
#9245=CARTESIAN_POINT ( 'NONE',  ( -13.08346052978740914, -7.620079078745922274, -220.3923444982454498 ) ) ;
#9246=CARTESIAN_POINT ( 'NONE',  ( -15.48255455842386219, 10.01793346089237069, -233.1197357361336913 ) ) ;
#9248=CARTESIAN_POINT ( 'NONE',  ( 28.22932473237819551, -8.039268142081398949, -226.6539694142420558 ) ) ;
#9249=CARTESIAN_POINT ( 'NONE',  ( 1.833772325875588027, 13.50593961039006707, -219.8748197804281119 ) ) ;
#9250=CARTESIAN_POINT ( 'NONE',  ( 14.81258087342262364, 2.398747990731791013, -230.9000679928271040 ) ) ;
#9251=CARTESIAN_POINT ( 'NONE',  ( 17.28149325064817887, -1.074788064772476792, -229.5315781944399305 ) ) ;
#9252=CARTESIAN_POINT ( 'NONE',  ( 4.389496648589924277, 14.47660514356954131, -220.6151178996808540 ) ) ;
#9253=CARTESIAN_POINT ( 'NONE',  ( -14.31049420963804586, -8.435107166214018903, -218.7432863707801403 ) ) ;
#9255=CARTESIAN_POINT ( 'NONE',  ( -7.834600152078401436, 27.83486203824852012, -220.1209588485844222 ) ) ;
#9256=CARTESIAN_POINT ( 'NONE',  ( -1.632242579688942596, -13.62074943359385415, -221.1585305289511041 ) ) ;
#9257=CARTESIAN_POINT ( 'NONE',  ( 4.559463107227270662, 13.27337529356814017, -226.9596205199204633 ) ) ;
#9258=CARTESIAN_POINT ( 'NONE',  ( 22.25403255790844881, -22.02690323431350450, -229.4561893391075671 ) ) ;
#9261=CARTESIAN_POINT ( 'NONE',  ( -9.988594796049140356, 11.34066464990972811, -226.6453149279956563 ) ) ;
#9262=( NAMED_UNIT ( * ) PLANE_ANGLE_UNIT ( ) SI_UNIT ( $, .RADIAN. ) );
#9263=CARTESIAN_POINT ( 'NONE',  ( 26.38334502096500245, -3.352420239867627494, -217.3603908026431384 ) ) ;
#9264=CARTESIAN_POINT ( 'NONE',  ( 15.50648685944955218, 24.16641006378193168, -224.4827813270165393 ) ) ;
#9265=CARTESIAN_POINT ( 'NONE',  ( -26.38808873681881906, 13.30696350521622939, -225.1492950792419663 ) ) ;
#9266=CARTESIAN_POINT ( 'NONE',  ( 14.98418162551161714, 4.450317369940187895, -227.9894155827521161 ) ) ;
#9267=CARTESIAN_POINT ( 'NONE',  ( -20.83288780491947279, -19.75659621676223665, -225.4831129403879117 ) ) ;
#9268=CARTESIAN_POINT ( 'NONE',  ( 25.30941179858102430, 8.661697827793627624, -216.7530520919057722 ) ) ;
#9270=CARTESIAN_POINT ( 'NONE',  ( -15.15102066082706678, -13.26725641419114510, -214.8414790003043322 ) ) ;
#9271=CARTESIAN_POINT ( 'NONE',  ( 3.378648530876271039, 26.08525450992624428, -218.4319906442508454 ) ) ;
#9272=CARTESIAN_POINT ( 'NONE',  ( 16.21758812354607215, 4.665393561625732488, -232.5634757513959983 ) ) ;
#9273=CARTESIAN_POINT ( 'NONE',  ( -6.804439720554941395, 15.25609613835249156, -218.7834354895107651 ) ) ;
#9274=CARTESIAN_POINT ( 'NONE',  ( -5.568057711815838751, 28.69723585065299076, -232.1518503103610271 ) ) ;
#9275=CARTESIAN_POINT ( 'NONE',  ( 18.69835413980967687, -1.262199651413310031, -230.6153330080101966 ) ) ;
#9276=CARTESIAN_POINT ( 'NONE',  ( 3.940243381406264511, -15.52098910442465041, -222.4744391328516144 ) ) ;
#9278=CARTESIAN_POINT ( 'NONE',  ( 10.46316887740464985, -17.92901728017801233, -232.6108895528913081 ) ) ;
#9280=CARTESIAN_POINT ( 'NONE',  ( 21.39553407250273054, 8.453402029343234148, -217.9531594780983141 ) ) ;
#9281=CARTESIAN_POINT ( 'NONE',  ( 29.17814965709308694, -1.309718763918959139, -225.2029557489520926 ) ) ;
#9282=CARTESIAN_POINT ( 'NONE',  ( -16.76449091996730090, -6.021196472930381738, -231.5810252088758432 ) ) ;
#9283=CARTESIAN_POINT ( 'NONE',  ( -1.608171596096409806, -16.77465153034988887, -217.4618546331240054 ) ) ;
#9284=CARTESIAN_POINT ( 'NONE',  ( 7.042184411928968935, 23.28260216771182556, -230.5707103145148267 ) ) ;
#9285=CARTESIAN_POINT ( 'NONE',  ( -24.79170285622992509, 4.551775110860766915, -234.5907228154019322 ) ) ;
#9286=CARTESIAN_POINT ( 'NONE',  ( -18.09776816382430908, 23.50806826204562583, -229.9568677523880638 ) ) ;
#9287=CARTESIAN_POINT ( 'NONE',  ( 1.030230143518703345, 18.27887886751213387, -229.5791973322770616 ) ) ;
#9288=CARTESIAN_POINT ( 'NONE',  ( 15.12095272344708263, -0.3261452966805281073, -219.6280520283587805 ) ) ;
#9291=CARTESIAN_POINT ( 'NONE',  ( 12.96449997971774870, 8.285709878278680662, -230.9518598506670628 ) ) ;
#9292=CARTESIAN_POINT ( 'NONE',  ( -15.07599795178976443, 12.40109266655585429, -218.9921934537110815 ) ) ;
#9293=CARTESIAN_POINT ( 'NONE',  ( 15.87399429023076003, -1.683916961781461552, -230.8621029165058758 ) ) ;
#9294=CARTESIAN_POINT ( 'NONE',  ( -5.693514143275418604, -18.22526881224050754, -218.3451910747569968 ) ) ;
#9297=CARTESIAN_POINT ( 'NONE',  ( 17.19674704922021391, 23.07334190050143974, -228.8256488842130238 ) ) ;
#9298=CARTESIAN_POINT ( 'NONE',  ( 14.68060984531904012, -6.704174034294832829, -225.1581031080203559 ) ) ;
#9299=CARTESIAN_POINT ( 'NONE',  ( -14.06164063153489252, 2.050767714179807744, -227.2881998904968270 ) ) ;
#9302=CARTESIAN_POINT ( 'NONE',  ( 6.741123954526870854, -14.00899218320067341, -219.0418835583997179 ) ) ;
#9303=CARTESIAN_POINT ( 'NONE',  ( 2.837900457371055563, 25.11342719071438978, -232.9871906064174709 ) ) ;
#9304=CARTESIAN_POINT ( 'NONE',  ( -17.94782256308196366, 19.07396065564992682, -232.7143578890335220 ) ) ;
#9306=CARTESIAN_POINT ( 'NONE',  ( -15.66530208164916260, 23.23467148471576849, -218.1250122661128046 ) ) ;
#9307=CARTESIAN_POINT ( 'NONE',  ( -11.24961133108761935, -10.18645864713539950, -228.7780882195199013 ) ) ;
#9310=CARTESIAN_POINT ( 'NONE',  ( -3.326157069579807946, 13.92020081821418565, -220.5733722327383930 ) ) ;
#9311=CARTESIAN_POINT ( 'NONE',  ( 3.737871636182809265, -14.23896033977216113, -229.0757302894822942 ) ) ;
#9312=CARTESIAN_POINT ( 'NONE',  ( 14.50031142556784580, -1.551246135476861188, -222.4318553185507028 ) ) ;
#9313=CARTESIAN_POINT ( 'NONE',  ( -24.24202834850560606, 19.05981756344202438, -226.6980666352953335 ) ) ;
#9314=CARTESIAN_POINT ( 'NONE',  ( -22.10934047915441170, 0.9940043559354162506, -215.0000000000000000 ) ) ;
#9315=CARTESIAN_POINT ( 'NONE',  ( -2.043230952238195286, 23.63069326910348877, -232.6835180461029040 ) ) ;
#9318=CARTESIAN_POINT ( 'NONE',  ( 15.04029996350473830, 7.457450192165341107, -220.5007084872782173 ) ) ;
#9319=CARTESIAN_POINT ( 'NONE',  ( -13.63268120803286720, -13.08481847960132249, -219.9337478264210404 ) ) ;
#9321=CARTESIAN_POINT ( 'NONE',  ( 2.893760225568064115, 14.39521026618305477, -227.6654023557511550 ) ) ;
#9322=CARTESIAN_POINT ( 'NONE',  ( -13.41250421226414069, 17.27419134292087577, -217.6844171132545966 ) ) ;
#9323=CARTESIAN_POINT ( 'NONE',  ( -19.01002492504315811, 19.85266905124972681, -219.0021410556803687 ) ) ;
#9324=CARTESIAN_POINT ( 'NONE',  ( -21.61315260466662380, -9.974349528768403417, -231.2583083768228960 ) ) ;
#9327=CARTESIAN_POINT ( 'NONE',  ( -14.70651859537745487, 4.211702956367679107, -230.0357207626005334 ) ) ;
#9328=CARTESIAN_POINT ( 'NONE',  ( 8.129749879387842881, -22.89596468334109147, -230.6606593278197295 ) ) ;
#9329=CARTESIAN_POINT ( 'NONE',  ( 16.64225601860865211, 1.926018578292457928, -220.2177910260893725 ) ) ;
#9330=CARTESIAN_POINT ( 'NONE',  ( -3.855805549595750392, 26.68244055262801950, -232.4569730455296508 ) ) ;
#9332=CARTESIAN_POINT ( 'NONE',  ( -16.29666348338687953, 2.994680995215331709, -221.2421885839926006 ) ) ;
#9333=CARTESIAN_POINT ( 'NONE',  ( 17.81160404892403193, 9.939217752910943560, -216.9646549374535311 ) ) ;
#9334=CARTESIAN_POINT ( 'NONE',  ( 23.04897566969193079, 17.95862962700741861, -223.6438515760422661 ) ) ;
#9336=CARTESIAN_POINT ( 'NONE',  ( -8.491902988188710921, -10.37035003683405066, -223.9502466269643435 ) ) ;
#9337=CARTESIAN_POINT ( 'NONE',  ( 3.342529885312644833, -17.78621320651278737, -216.7788622297345853 ) ) ;
#9341=CARTESIAN_POINT ( 'NONE',  ( -7.834600152078401436, 27.83486203824852012, -220.1209588485844222 ) ) ;
#9342=CARTESIAN_POINT ( 'NONE',  ( 27.25858960103340323, -9.764658377823966617, -217.2703135185301448 ) ) ;
#9343=CARTESIAN_POINT ( 'NONE',  ( 17.00614511541963836, -1.958782916976874233, -219.4638360731791806 ) ) ;
#9344=CARTESIAN_POINT ( 'NONE',  ( 13.20340559785743828, 9.575208899273587093, -218.1210831379648312 ) ) ;
#9345=CARTESIAN_POINT ( 'NONE',  ( 11.73428189025226942, 12.46434742632455084, -228.1539301014595083 ) ) ;
#9347=CARTESIAN_POINT ( 'NONE',  ( 24.73665505496147432, -17.48642391317526190, -218.9253764065177847 ) ) ;
#9349=CARTESIAN_POINT ( 'NONE',  ( 3.744112528862662881, 31.76296354843916703, -227.8872370379487506 ) ) ;
#9350=CARTESIAN_POINT ( 'NONE',  ( -10.83439284573031536, 18.36737820296253432, -234.3014274143859836 ) ) ;
#9351=CARTESIAN_POINT ( 'NONE',  ( -12.96708845633950347, -3.368725568741437026, -223.5528514750533873 ) ) ;
#9352=CARTESIAN_POINT ( 'NONE',  ( -22.11084984981285118, 10.96048252433489623, -216.6117774006995376 ) ) ;
#9354=CARTESIAN_POINT ( 'NONE',  ( 16.06750045776299629, -1.909440863493336860, -220.4398626676318713 ) ) ;
#9355=CARTESIAN_POINT ( 'NONE',  ( 1.220475224794998370, 29.83033731899746144, -230.4224274340063801 ) ) ;
#9356=CARTESIAN_POINT ( 'NONE',  ( 18.03440114592047649, 4.755211820135348155, -216.3599228381250157 ) ) ;
#9357=CARTESIAN_POINT ( 'NONE',  ( -10.65455960636934662, 10.37188583052882862, -219.5197110153079620 ) ) ;
#9358=CARTESIAN_POINT ( 'NONE',  ( 13.69275646168278371, 8.674223198772375909, -220.8699857572541987 ) ) ;
#9361=CARTESIAN_POINT ( 'NONE',  ( 5.365126951644291431, 19.60085171667039816, -218.9155869426879519 ) ) ;
#9362=CARTESIAN_POINT ( 'NONE',  ( -11.20272313682045073, -7.956653478762055087, -225.3025344850567819 ) ) ;
#9363=CARTESIAN_POINT ( 'NONE',  ( 19.72515656911863147, 14.02277373989196541, -218.0718040828188009 ) ) ;
#9364=CARTESIAN_POINT ( 'NONE',  ( 2.898952953659251985, -22.97888022809681274, -215.2852275949887826 ) ) ;
#9366=CARTESIAN_POINT ( 'NONE',  ( -15.30295614572244922, 9.661125001905515930, -218.8475896279880146 ) ) ;
#9367=CARTESIAN_POINT ( 'NONE',  ( 23.17317677245511831, -6.950782331930943414, -233.5406539459643227 ) ) ;
#9368=CARTESIAN_POINT ( 'NONE',  ( 3.182992543297812560, 16.68308636702302650, -221.9272281984358415 ) ) ;
#9369=CARTESIAN_POINT ( 'NONE',  ( -11.35482716595652875, 11.86850131893102223, -220.6599844941370350 ) ) ;
#9370=CARTESIAN_POINT ( 'NONE',  ( -18.67456582549428390, 11.07053394491094345, -214.7114755712704550 ) ) ;
#9371=CARTESIAN_POINT ( 'NONE',  ( -6.532222827695542300, -22.16123078269809099, -233.6760793125601481 ) ) ;
#9372=CARTESIAN_POINT ( 'NONE',  ( 20.96405783751201213, 6.249056650590980588, -215.6254004080763309 ) ) ;
#9374=CARTESIAN_POINT ( 'NONE',  ( -11.84714279977019125, -8.528511525072332233, -232.0239825124074002 ) ) ;
#9375=CARTESIAN_POINT ( 'NONE',  ( -4.715783688792956063, 28.29821729825949816, -228.0423900005874600 ) ) ;
#9376=CARTESIAN_POINT ( 'NONE',  ( 12.81769551943392393, 4.437328497131001193, -221.7762769673541072 ) ) ;
#9378=CARTESIAN_POINT ( 'NONE',  ( -13.41250421226414069, 17.27419134292087577, -217.6844171132545966 ) ) ;
#9379=CARTESIAN_POINT ( 'NONE',  ( 4.914880347045685660, 14.54749271951947698, -232.8668677254037789 ) ) ;
#9380=CARTESIAN_POINT ( 'NONE',  ( 2.245945009347994237, -28.59251958642781233, -226.9771193766267743 ) ) ;
#9381=CARTESIAN_POINT ( 'NONE',  ( 1.102456202203287550, -23.13885590315818064, -232.0370787247644557 ) ) ;
#9383=CARTESIAN_POINT ( 'NONE',  ( 25.33562512631297281, 12.25422971834577268, -228.6777356031426791 ) ) ;
#9384=CARTESIAN_POINT ( 'NONE',  ( 12.70477135646371281, -9.814387909761604689, -230.3443492180780652 ) ) ;
#9385=CARTESIAN_POINT ( 'NONE',  ( -13.05629324012484282, -10.24599397043673221, -218.7452066004821347 ) ) ;
#9386=CARTESIAN_POINT ( 'NONE',  ( -15.27057301462635408, -17.00912219741827514, -233.6288396447818627 ) ) ;
#9387=CARTESIAN_POINT ( 'NONE',  ( 3.191455400233187412, 17.67480163422566619, -220.7055581859663107 ) ) ;
#9389=CARTESIAN_POINT ( 'NONE',  ( -11.36937006530106586, 5.486019310970209339, -224.0742584078730033 ) ) ;
#9390=CARTESIAN_POINT ( 'NONE',  ( 4.543450689403089271, 15.91052110650461771, -218.9437823786444426 ) ) ;
#9391=CARTESIAN_POINT ( 'NONE',  ( 3.182992543297812560, 16.68308636702302650, -221.9272281984358415 ) ) ;
#9392=CARTESIAN_POINT ( 'NONE',  ( 13.79223148755288797, -4.990905483784310981, -230.8248327435212559 ) ) ;
#9394=CARTESIAN_POINT ( 'NONE',  ( 8.821742718405863215, 10.82866050966069160, -221.4785132813277642 ) ) ;
#9395=CARTESIAN_POINT ( 'NONE',  ( -12.96364545172611571, 10.77137376900670063, -221.1208843751685720 ) ) ;
#9396=CARTESIAN_POINT ( 'NONE',  ( 20.96405783751201213, 6.249056650590980588, -215.6254004080763309 ) ) ;
#9397=CARTESIAN_POINT ( 'NONE',  ( 1.525817648051120967, -14.82969601928396841, -225.8796824437346515 ) ) ;
#9400=CARTESIAN_POINT ( 'NONE',  ( 3.449504654906655254, 27.59247159270940841, -231.3461799890608859 ) ) ;
#9401=CARTESIAN_POINT ( 'NONE',  ( 15.64298904066490259, -12.83894575744357880, -230.8789486217465594 ) ) ;
#9404=CARTESIAN_POINT ( 'NONE',  ( -11.07688804854283049, -12.81333559660784971, -232.1241261852632363 ) ) ;
#9405=CARTESIAN_POINT ( 'NONE',  ( 4.354034006296288339, 14.09944204372416188, -221.2519525881239417 ) ) ;
#9406=CARTESIAN_POINT ( 'NONE',  ( -0.3984245442872364484, 11.77931270252508789, -223.1826369159892920 ) ) ;
#9408=CARTESIAN_POINT ( 'NONE',  ( -16.39453490553961856, 20.24836633112041184, -233.1722131570092245 ) ) ;
#9409=CARTESIAN_POINT ( 'NONE',  ( 22.35566739451469331, -4.954007294914331894, -217.4158986454943374 ) ) ;
#9412=CARTESIAN_POINT ( 'NONE',  ( -9.171998067665157350, 9.395241133357435714, -226.3428046914542051 ) ) ;
#9413=CARTESIAN_POINT ( 'NONE',  ( -8.649444225544010934, -13.15555178350489918, -216.8547715670961509 ) ) ;
#9415=CARTESIAN_POINT ( 'NONE',  ( -16.39453490553961856, 20.24836633112041184, -233.1722131570092245 ) ) ;
#9417=CARTESIAN_POINT ( 'NONE',  ( 20.62963957373278134, 2.372686805184054837, -232.5966151263358483 ) ) ;
#9419=CARTESIAN_POINT ( 'NONE',  ( -9.350291727197115321, 27.53754332352430367, -230.1504993026967441 ) ) ;
#9420=CARTESIAN_POINT ( 'NONE',  ( 13.80743592543072396, -3.637675435010108906E-12, -228.0000000000000568 ) ) ;
#9421=CARTESIAN_POINT ( 'NONE',  ( 24.96615890023450035, 5.871290975262302148, -218.1661911638112201 ) ) ;
#9422=CARTESIAN_POINT ( 'NONE',  ( -18.79436262126649027, -19.56097393442729526, -222.1480387859219547 ) ) ;
#9425=CARTESIAN_POINT ( 'NONE',  ( 8.860681144154234801, 27.11956268701432293, -229.8503778060109823 ) ) ;
#9426=CARTESIAN_POINT ( 'NONE',  ( -17.75632171729475317, 14.45153669854845901, -218.6240360064753929 ) ) ;
#9427=CARTESIAN_POINT ( 'NONE',  ( -12.39654240422350462, 9.886262337642440556, -219.1620329226848014 ) ) ;
#9430=CARTESIAN_POINT ( 'NONE',  ( -22.94312929380076937, -2.351969141711130806, -217.0768970835230505 ) ) ;
#9434=CARTESIAN_POINT ( 'NONE',  ( -16.71711190488355570, 0.6105529133557690002, -230.9511258789794681 ) ) ;
#9435=CARTESIAN_POINT ( 'NONE',  ( -11.90549671174648694, -23.44716645851259784, -216.8989558407570257 ) ) ;
#9436=CARTESIAN_POINT ( 'NONE',  ( 13.47977767379887659, 1.040845183112855787, -227.8169118424926296 ) ) ;
#9437=CARTESIAN_POINT ( 'NONE',  ( 0.2389779871941385414, 16.64595486589868045, -218.1658233406367629 ) ) ;
#9439=CARTESIAN_POINT ( 'NONE',  ( -20.84243560023798736, 1.479777185913828230, -230.9766426496277631 ) ) ;
#9440=CARTESIAN_POINT ( 'NONE',  ( 9.851209273476317918, 25.48401176094959553, -233.7173763849377792 ) ) ;
#9441=SHAPE_REPRESENTATION_RELATIONSHIP ( 'NONE' , 'NONE' ,  #1546, #20907 ) ;
#9443=CARTESIAN_POINT ( 'NONE',  ( 15.87442104186276381, 8.674488492264579520, -230.9702037640878416 ) ) ;
#9445=CARTESIAN_POINT ( 'NONE',  ( -25.64743926792790063, -18.08564893845128907, -228.9187414798782925 ) ) ;
#9446=CARTESIAN_POINT ( 'NONE',  ( -9.625604265899946554, -19.21123364792547505, -233.9327940972253259 ) ) ;
#9450=CARTESIAN_POINT ( 'NONE',  ( -1.582540545905128049, 14.52388882916313584, -222.9138157219475147 ) ) ;
#9451=CARTESIAN_POINT ( 'NONE',  ( 18.12061937846576853, -10.14999073105125227, -235.3098052193838612 ) ) ;
#9452=CARTESIAN_POINT ( 'NONE',  ( 14.68556740487494849, -6.365102927765655672, -229.6664356779805587 ) ) ;
#9453=CARTESIAN_POINT ( 'NONE',  ( -13.75208518020500748, 5.661250135068270239, -227.6647651141479685 ) ) ;
#9454=CARTESIAN_POINT ( 'NONE',  ( 10.70175380652492336, 7.370128018021000038, -224.3479584370086286 ) ) ;
#9455=CARTESIAN_POINT ( 'NONE',  ( 8.647507700742417924, 16.42978512283924175, -220.3082116258600536 ) ) ;
#9457=CARTESIAN_POINT ( 'NONE',  ( 6.889583945421565048, -13.03635046449108081, -231.0237689561592731 ) ) ;
#9460=CARTESIAN_POINT ( 'NONE',  ( -4.845359737286285551, 16.85396349487340117, -233.9229833851842670 ) ) ;
#9461=CARTESIAN_POINT ( 'NONE',  ( -9.578110717394128670, 23.64032677849093034, -215.7669555765890550 ) ) ;
#9462=CARTESIAN_POINT ( 'NONE',  ( 23.53402537799887284, -10.66620622184993650, -219.3119847637072439 ) ) ;
#9463=CARTESIAN_POINT ( 'NONE',  ( -3.003186468682855104, 15.63968344752823469, -231.5301608670590667 ) ) ;
#9465=CARTESIAN_POINT ( 'NONE',  ( 0.1866476013601106043, 25.93503619265524307, -233.5574764272258790 ) ) ;
#9466=CARTESIAN_POINT ( 'NONE',  ( 17.98589043827631428, 2.945998030785370592, -233.4030907785035538 ) ) ;
#9467=CARTESIAN_POINT ( 'NONE',  ( -9.151299407007059017, 9.196974979111923076, -223.9483834032048719 ) ) ;
#9468=CARTESIAN_POINT ( 'NONE',  ( 15.42212722119060864, 5.401662248084913465, -220.8333402320903645 ) ) ;
#9471=CARTESIAN_POINT ( 'NONE',  ( -21.94776718874820176, -0.4748437386657589632, -216.1214812709574176 ) ) ;
#9472=CARTESIAN_POINT ( 'NONE',  ( -2.129100187576105530, 26.11057959790866789, -231.5939360033278547 ) ) ;
#9473=CARTESIAN_POINT ( 'NONE',  ( -10.11868820210310282, -13.51996935893276053, -218.1704188629865371 ) ) ;
#9474=CARTESIAN_POINT ( 'NONE',  ( 24.42567939027770407, 10.22651298688739097, -219.4562066833365748 ) ) ;
#9475=CARTESIAN_POINT ( 'NONE',  ( -7.732225105831920686, -12.76821222370703346, -228.2562058524068220 ) ) ;
#9477=CARTESIAN_POINT ( 'NONE',  ( -13.97943781666340790, 5.798109546139844639, -228.2992319913466019 ) ) ;
#9479=CARTESIAN_POINT ( 'NONE',  ( 12.75766869239441803, -12.84633107758633663, -232.0853690516983079 ) ) ;
#9480=CARTESIAN_POINT ( 'NONE',  ( 8.686008240521225332, 26.11221116136006515, -227.6539570933143466 ) ) ;
#9481=CARTESIAN_POINT ( 'NONE',  ( -14.94667331530454213, 6.325011500478772142, -230.0242139990887154 ) ) ;
#9482=CARTESIAN_POINT ( 'NONE',  ( -25.32262741784088078, 2.623212696197013472, -234.6011982779809841 ) ) ;
#9483=CARTESIAN_POINT ( 'NONE',  ( -17.95722789764597849, -8.907256384892455969, -219.4045086951509518 ) ) ;
#9484=CARTESIAN_POINT ( 'NONE',  ( 25.41781277602550304, 19.49958712797920057, -223.1230538376805441 ) ) ;
#9487=CARTESIAN_POINT ( 'NONE',  ( -15.30224200789663946, -6.308083384910589508, -216.9633489813582514 ) ) ;
#9488=CARTESIAN_POINT ( 'NONE',  ( 3.312424284731937618, 15.29837714273186045, -229.5209971419123747 ) ) ;
#9489=CARTESIAN_POINT ( 'NONE',  ( 17.66525298603349370, 4.919957226727790456, -233.3736646485340032 ) ) ;
#9490=CARTESIAN_POINT ( 'NONE',  ( -6.127117917506272882, 18.94558806480136681, -232.9763641438055117 ) ) ;
#9491=CARTESIAN_POINT ( 'NONE',  ( 19.66122710937851537, 22.83208755991274330, -220.0578523118790883 ) ) ;
#9493=CARTESIAN_POINT ( 'NONE',  ( -5.077014288276974874, -29.41487918302398796, -226.0100937268998962 ) ) ;
#9495=CARTESIAN_POINT ( 'NONE',  ( -1.097449620509919788, -25.21235133823365260, -218.6697740411501059 ) ) ;
#9496=CARTESIAN_POINT ( 'NONE',  ( 20.34032485158648029, 2.741617426884598530, -217.9827731991294968 ) ) ;
#9497=CARTESIAN_POINT ( 'NONE',  ( 20.38902395782249144, -18.95772103455488633, -230.9098670703349967 ) ) ;
#9498=CARTESIAN_POINT ( 'NONE',  ( 13.45252989138277400, -0.3779036657139918098, -224.7462000225944792 ) ) ;
#9499=CARTESIAN_POINT ( 'NONE',  ( -20.83683780809167629, -19.66850649927503625, -219.7460615899071570 ) ) ;
#9500=CARTESIAN_POINT ( 'NONE',  ( 8.686008240521225332, 26.11221116136006515, -227.6539570933143466 ) ) ;
#9501=DIRECTION ( 'NONE',  ( -0.9940043559354330149, -0.1093404791528966163, -6.737719923507020479E-14 ) ) ;
#9502=CARTESIAN_POINT ( 'NONE',  ( 16.55609572527610851, 2.729108819536508967, -230.5704679660131831 ) ) ;
#9504=CARTESIAN_POINT ( 'NONE',  ( 5.623554730548537606, 15.65270319720736225, -231.3185741195121068 ) ) ;
#9505=CARTESIAN_POINT ( 'NONE',  ( -3.015877970456246615, 27.27456613555083464, -227.6995284396757313 ) ) ;
#9506=CARTESIAN_POINT ( 'NONE',  ( 17.11616244378571494, -1.720737510755655064, -232.0394440302203236 ) ) ;
#9508=CARTESIAN_POINT ( 'NONE',  ( 23.21336156720804667, 12.57464006230432574, -232.9346648124233070 ) ) ;
#9509=CARTESIAN_POINT ( 'NONE',  ( -23.77327857871830830, 11.53128597905896768, -221.0855018166512025 ) ) ;
#9510=CARTESIAN_POINT ( 'NONE',  ( -25.19195624009214640, 10.50676406307063182, -220.0954552869889937 ) ) ;
#9511=CARTESIAN_POINT ( 'NONE',  ( -1.434166139689934338, -16.90223958437590213, -219.9603817157532433 ) ) ;
#9514=CARTESIAN_POINT ( 'NONE',  ( 14.68783945462866924, 9.535285537539673228, -219.4694094309942045 ) ) ;
#9515=CARTESIAN_POINT ( 'NONE',  ( 13.81930941494936782, -14.31252807618095879, -218.6132940872857375 ) ) ;
#9517=CARTESIAN_POINT ( 'NONE',  ( -1.778254167844783851, -12.78790610364390012, -225.9413532495922254 ) ) ;
#9519=CARTESIAN_POINT ( 'NONE',  ( -1.881996891245037995, 28.05344686410985489, -218.6379207300106202 ) ) ;
#9521=CARTESIAN_POINT ( 'NONE',  ( 4.719925043692215993, 22.16918918211828782, -214.6883144083888908 ) ) ;
#9523=CARTESIAN_POINT ( 'NONE',  ( -7.189383125363055349, 14.28512618638020548, -231.7475838278701303 ) ) ;
#9524=CARTESIAN_POINT ( 'NONE',  ( 26.42472234358771033, -2.855770380922216134, -231.8949512018254211 ) ) ;
#9528=CARTESIAN_POINT ( 'NONE',  ( -12.90983082593748676, 14.84936372681532823, -233.8009687022269532 ) ) ;
#9529=CARTESIAN_POINT ( 'NONE',  ( -21.38010734112553024, -21.14131910627544997, -218.4623475309535365 ) ) ;
#9530=CARTESIAN_POINT ( 'NONE',  ( 15.05686526350529775, -5.555778903407086133, -220.1433349335996468 ) ) ;
#9531=CARTESIAN_POINT ( 'NONE',  ( -26.74045434827795020, 12.41518252455047744, -220.4617428697642652 ) ) ;
#9532=CARTESIAN_POINT ( 'NONE',  ( -12.45629340980802269, 5.675423426979704367, -220.8874502847910719 ) ) ;
#9533=CARTESIAN_POINT ( 'NONE',  ( 4.936777854427027989, 27.97379167488809060, -227.0886654730259124 ) ) ;
#9535=CARTESIAN_POINT ( 'NONE',  ( -11.78887577478644566, 1.715692547334320084, -224.3106172711415525 ) ) ;
#9536=CARTESIAN_POINT ( 'NONE',  ( -7.149118023545313783, -16.86598457999096823, -220.1902049135764514 ) ) ;
#9539=CARTESIAN_POINT ( 'NONE',  ( 8.379126514044342500, 15.76264856365358646, -232.1787896114811360 ) ) ;
#9540=CARTESIAN_POINT ( 'NONE',  ( -2.917590128672695293, 18.81591489065672818, -216.3635620530855022 ) ) ;
#9541=CARTESIAN_POINT ( 'NONE',  ( -17.19162585816985001, -4.675655174483583032, -230.6997921109560821 ) ) ;
#9546=CARTESIAN_POINT ( 'NONE',  ( 21.83031488337932657, -1.542591969257240070, -231.3901500139511427 ) ) ;
#9547=CARTESIAN_POINT ( 'NONE',  ( -5.472810246302690196, -26.30400724048815420, -218.4657170016378416 ) ) ;
#9548=CARTESIAN_POINT ( 'NONE',  ( 25.69300549816939494, 5.947472783069708946, -230.6131061331718115 ) ) ;
#9549=CARTESIAN_POINT ( 'NONE',  ( -1.249406995060579062, 25.48934319316224162, -216.9406480707515072 ) ) ;
#9552=CARTESIAN_POINT ( 'NONE',  ( -16.40443871513620522, 4.023423476741658789, -228.9829044427089002 ) ) ;
#9553=CARTESIAN_POINT ( 'NONE',  ( 8.730612144237051453, 13.93563980088501886, -217.1627566045470132 ) ) ;
#9555=CARTESIAN_POINT ( 'NONE',  ( 19.72515656911863147, 14.02277373989196541, -218.0718040828188009 ) ) ;
#9557=CARTESIAN_POINT ( 'NONE',  ( 25.61231557635624156, -8.129803667132245337, -228.3450084804328242 ) ) ;
#9558=CARTESIAN_POINT ( 'NONE',  ( -17.21167111787709914, -1.850592482912338799, -230.8442569545952665 ) ) ;
#9562=CARTESIAN_POINT ( 'NONE',  ( -5.861205904341304951, 14.21969934012253312, -219.3213214613830644 ) ) ;
#9563=CARTESIAN_POINT ( 'NONE',  ( 26.97873870420736253, -17.71910932852193454, -225.8965020979516964 ) ) ;
#9564=CARTESIAN_POINT ( 'NONE',  ( 23.36729170583618398, -5.500043712341283531, -232.1593072787115375 ) ) ;
#9565=CARTESIAN_POINT ( 'NONE',  ( -28.31595744342370580, 5.786754998807587924, -229.0820962600229223 ) ) ;
#9566=CARTESIAN_POINT ( 'NONE',  ( 14.69879291197755222, 10.86005690695417236, -216.7815908316746913 ) ) ;
#9567=CARTESIAN_POINT ( 'NONE',  ( 11.16964468591631920, 25.71443501674299981, -224.7497461878887464 ) ) ;
#9569=CARTESIAN_POINT ( 'NONE',  ( 5.701450259358237460, -28.73672391946437088, -229.2085834618566196 ) ) ;
#9570=CARTESIAN_POINT ( 'NONE',  ( 20.58703255433590940, 0.4816031003617209372, -231.9427175861361263 ) ) ;
#9571=CARTESIAN_POINT ( 'NONE',  ( -4.334570222994868161, 11.62786715207288601, -222.6396919303362267 ) ) ;
#9572=CARTESIAN_POINT ( 'NONE',  ( -8.329232059016652201, 11.81357365351366617, -230.1839637212758021 ) ) ;
#9573=CARTESIAN_POINT ( 'NONE',  ( 14.36131679319511001, -8.144601358551431858, -221.7207256223857144 ) ) ;
#9574=CARTESIAN_POINT ( 'NONE',  ( -2.208416658185406334, 29.10348627872611615, -219.8480645685746424 ) ) ;
#9577=CARTESIAN_POINT ( 'NONE',  ( 2.469769522101480597, 18.85781121334172639, -215.5372409425634430 ) ) ;
#9578=CARTESIAN_POINT ( 'NONE',  ( 14.17826651990317188, -1.167225063855702683, -222.4240311848849387 ) ) ;
#9579=CARTESIAN_POINT ( 'NONE',  ( -15.58461825850822180, 18.91734573546571951, -233.7691177939990723 ) ) ;
#9580=CARTESIAN_POINT ( 'NONE',  ( 15.89706143421296147, 10.57416387607782227, -218.3862415393350318 ) ) ;
#9581=CARTESIAN_POINT ( 'NONE',  ( 1.820119372073704112, 23.17972341190215246, -230.7270437017659503 ) ) ;
#9582=CARTESIAN_POINT ( 'NONE',  ( -27.06419889410506485, -1.187659473326917237, -217.6367138431444630 ) ) ;
#9584=CARTESIAN_POINT ( 'NONE',  ( 16.49020573214642837, 22.44566021525517741, -224.7841662740084701 ) ) ;
#9585=CARTESIAN_POINT ( 'NONE',  ( -20.11874861854083463, -21.11755179634840474, -229.7504124090357323 ) ) ;
#9586=CARTESIAN_POINT ( 'NONE',  ( 11.57669841200422134, 10.63052136557218574, -228.9489978335593889 ) ) ;
#9587=CARTESIAN_POINT ( 'NONE',  ( -0.2114165566986584699, -18.43750818655219703, -233.9360633499430833 ) ) ;
#9590=CARTESIAN_POINT ( 'NONE',  ( -17.39737143130126285, 7.531548707695031375, -232.0788227848755696 ) ) ;
#9591=CARTESIAN_POINT ( 'NONE',  ( 10.52067862919218832, -10.34113464825721351, -228.4460540958991714 ) ) ;
#9592=CARTESIAN_POINT ( 'NONE',  ( 7.067550969709256670, 17.75197616922148569, -219.3387126207321955 ) ) ;
#9593=CARTESIAN_POINT ( 'NONE',  ( -20.57288920227272655, 16.51351902378409520, -230.8484733908063333 ) ) ;
#9594=CARTESIAN_POINT ( 'NONE',  ( -31.84745724608465522, 5.474219582435353004, -224.7210333253351564 ) ) ;
#9595=CARTESIAN_POINT ( 'NONE',  ( -26.02538399328502905, -8.003917019953526335, -222.3553134616452098 ) ) ;
#9596=CARTESIAN_POINT ( 'NONE',  ( 12.48419387172699579, 6.663456953110941328, -219.2717027540951165 ) ) ;
#9598=CARTESIAN_POINT ( 'NONE',  ( -14.30218759248275084, -10.01744029472290620, -234.2423117832250341 ) ) ;
#9599=CARTESIAN_POINT ( 'NONE',  ( 8.674175678922351196, 20.85307874897338110, -216.6688793998777101 ) ) ;
#9601=CARTESIAN_POINT ( 'NONE',  ( 21.77183241683778547, 12.04504704525620085, -233.6005549158834640 ) ) ;
#9602=CARTESIAN_POINT ( 'NONE',  ( -10.65640919150578192, 23.79238421564942740, -218.1088542024188826 ) ) ;
#9603=CARTESIAN_POINT ( 'NONE',  ( 19.97628502126439187, 24.50819884991013708, -224.8824979922784735 ) ) ;
#9604=CARTESIAN_POINT ( 'NONE',  ( 3.323726671003152777, -15.99176757603385823, -228.1400570273458186 ) ) ;
#9605=CARTESIAN_POINT ( 'NONE',  ( -6.454554286546707154, -27.99704349260872149, -227.4356265632874852 ) ) ;
#9606=CARTESIAN_POINT ( 'NONE',  ( 14.80394259695730064, 1.224172658189580432, -225.4564070658925061 ) ) ;
#9607=CARTESIAN_POINT ( 'NONE',  ( 21.53087031351596892, -21.03550532031109555, -227.1077645633325233 ) ) ;
#9608=CARTESIAN_POINT ( 'NONE',  ( 15.12095272344708263, -0.3261452966805281073, -219.6280520283587805 ) ) ;
#9609=CARTESIAN_POINT ( 'NONE',  ( -11.20272313682045073, -7.956653478762055087, -225.3025344850567819 ) ) ;
#9610=CARTESIAN_POINT ( 'NONE',  ( 3.198229568054530070, 16.42319727383711481, -222.3960047798183552 ) ) ;
#9612=CARTESIAN_POINT ( 'NONE',  ( -20.05025075566126702, 1.207204931470905018, -215.1628017022767949 ) ) ;
#9613=CARTESIAN_POINT ( 'NONE',  ( 4.354034006296288339, 14.09944204372416188, -221.2519525881239417 ) ) ;
#9614=CARTESIAN_POINT ( 'NONE',  ( 1.296323513242173542, 20.09034598902932345, -230.5712631353794961 ) ) ;
#9615=CARTESIAN_POINT ( 'NONE',  ( 14.31773767102621875, -28.01644431351170894, -220.7875045263454865 ) ) ;
#9616=CARTESIAN_POINT ( 'NONE',  ( 27.79746884017060538, 13.63637251724950339, -226.5788410723774575 ) ) ;
#9617=CARTESIAN_POINT ( 'NONE',  ( -17.65560862077320081, 21.92186454631220371, -221.3776075196718693 ) ) ;
#9618=CARTESIAN_POINT ( 'NONE',  ( -20.84243560023798736, 1.479777185913828230, -230.9766426496277631 ) ) ;
#9619=CARTESIAN_POINT ( 'NONE',  ( -7.086613078029399659, -28.17108726511417771, -223.6412629831645233 ) ) ;
#9622=CARTESIAN_POINT ( 'NONE',  ( 17.99029889091409018, 9.613712288440757092, -232.0298403238024036 ) ) ;
#9623=CARTESIAN_POINT ( 'NONE',  ( 19.77988345122896163, -10.57228134044703793, -230.8608254296808866 ) ) ;
#9626=CARTESIAN_POINT ( 'NONE',  ( -11.06377138986482933, -15.30386857868810857, -217.0411070525910873 ) ) ;
#9627=CARTESIAN_POINT ( 'NONE',  ( 1.773982976645536835, 19.12448993322812285, -233.2315972735944172 ) ) ;
#9628=CARTESIAN_POINT ( 'NONE',  ( 4.754245974719506940, 31.05377813473586102, -220.6166503949300193 ) ) ;
#9630=CARTESIAN_POINT ( 'NONE',  ( -22.99617382825321599, 17.18101613848176967, -230.9512687019100099 ) ) ;
#9631=CARTESIAN_POINT ( 'NONE',  ( -12.96708845633950347, -3.368725568741437026, -223.5528514750533873 ) ) ;
#9632=CARTESIAN_POINT ( 'NONE',  ( 30.81364357021286793, -2.580535071768633060, -224.0234450364292513 ) ) ;
#9634=CARTESIAN_POINT ( 'NONE',  ( -6.474151797443945533, 21.29193859232740138, -215.9573456447696458 ) ) ;
#9635=CARTESIAN_POINT ( 'NONE',  ( -6.154316005079235374, -31.08134634390615503, -226.4265589226172892 ) ) ;
#9636=CARTESIAN_POINT ( 'NONE',  ( 18.22947608839760747, -6.525328669204546905, -217.7409786913911205 ) ) ;
#9637=CARTESIAN_POINT ( 'NONE',  ( -9.749377714296398878, 10.28442384816749922, -229.3722863967025205 ) ) ;
#9638=CARTESIAN_POINT ( 'NONE',  ( 16.26115440404298340, 3.800605480264513059, -219.2833057824682612 ) ) ;
#9639=CARTESIAN_POINT ( 'NONE',  ( 5.104697752190542559, 17.18208638613223016, -220.3923334988619445 ) ) ;
#9640=FACE_OUTER_BOUND ( 'NONE', #15439, .T. ) ;
#9641=CARTESIAN_POINT ( 'NONE',  ( -21.39667546302236900, 3.687493526428279100, -235.1435990565495047 ) ) ;
#9642=CARTESIAN_POINT ( 'NONE',  ( -9.770823421170108602, -12.84821564276127503, -225.3905567659999178 ) ) ;
#9644=CARTESIAN_POINT ( 'NONE',  ( -10.02095171162140019, 11.02119725306997111, -224.1251327387667516 ) ) ;
#9645=CARTESIAN_POINT ( 'NONE',  ( 16.55626903245587656, 22.80423546114836952, -218.9884947126587633 ) ) ;
#9646=CARTESIAN_POINT ( 'NONE',  ( 5.773563157792669820, 21.63217468058455140, -235.0383461317610170 ) ) ;
#9648=CARTESIAN_POINT ( 'NONE',  ( 15.91397826126795323, -3.183288324723350549, -218.2846031002558504 ) ) ;
#9651=CARTESIAN_POINT ( 'NONE',  ( -23.52999999174766543, 19.39566142560855866, -221.9446938626390704 ) ) ;
#9652=CARTESIAN_POINT ( 'NONE',  ( -2.927465716848487887, -13.57531311500885352, -224.4053031992201852 ) ) ;
#9654=CARTESIAN_POINT ( 'NONE',  ( 11.67669251569587985, 24.04736029062789981, -218.5856804285192254 ) ) ;
#9657=CARTESIAN_POINT ( 'NONE',  ( -17.15943377049709184, 17.77880916606822836, -233.2929083076029144 ) ) ;
#9659=CARTESIAN_POINT ( 'NONE',  ( 24.81668481317358399, 17.11438712655213124, -222.1096362285750274 ) ) ;
#9660=SURFACE_STYLE_FILL_AREA ( #15065 ) ;
#9661=CARTESIAN_POINT ( 'NONE',  ( 13.61857686585203275, 0.5573421744009137146, -222.0497554577703170 ) ) ;
#9662=CARTESIAN_POINT ( 'NONE',  ( 10.55627441269396094, 10.31758739525044888, -223.1990319438957613 ) ) ;
#9664=CARTESIAN_POINT ( 'NONE',  ( 19.77988345122896163, -10.57228134044703793, -230.8608254296808866 ) ) ;
#9665=CARTESIAN_POINT ( 'NONE',  ( -15.46216926290318305, -2.495270579625169738, -221.2150947962298631 ) ) ;
#9668=CARTESIAN_POINT ( 'NONE',  ( -1.316322971969275502, 14.13179993441458215, -224.9782367179667233 ) ) ;
#9669=CARTESIAN_POINT ( 'NONE',  ( 17.10065829945946092, -7.211672327051211084, -215.1948405133616404 ) ) ;
#9670=CARTESIAN_POINT ( 'NONE',  ( 13.82188917133564132, -5.740199443570373816, -227.9076376976435654 ) ) ;
#9671=CARTESIAN_POINT ( 'NONE',  ( -17.43458823433387650, 2.804998135793385750, -231.8077100320880959 ) ) ;
#9672=CARTESIAN_POINT ( 'NONE',  ( 14.46993441875745390, 0.2699826811589002284, -230.0986938382904157 ) ) ;
#9673=CARTESIAN_POINT ( 'NONE',  ( 8.961491954973460849, 17.27041174997091844, -219.7661252763212474 ) ) ;
#9675=CARTESIAN_POINT ( 'NONE',  ( 0.2144678239183100965, -16.00554277676860693, -220.6792656679080267 ) ) ;
#9677=CARTESIAN_POINT ( 'NONE',  ( -17.22166590524039265, 4.587137274468266135, -215.4863060638890033 ) ) ;
#9678=CARTESIAN_POINT ( 'NONE',  ( 5.501756899793208255, 15.97909684020861043, -233.9380718515096191 ) ) ;
#9679=CARTESIAN_POINT ( 'NONE',  ( -1.302381543002304687, 18.65968181418110206, -215.1730913991678449 ) ) ;
#9680=CARTESIAN_POINT ( 'NONE',  ( 13.49585564903807722, -8.492623513249517586, -227.3331091713134811 ) ) ;
#9681=CARTESIAN_POINT ( 'NONE',  ( 0.2389779871941385414, 16.64595486589868045, -218.1658233406367629 ) ) ;
#9682=CARTESIAN_POINT ( 'NONE',  ( -15.23434562258889891, -0.4010941804143903222, -220.4743703065900036 ) ) ;
#9683=CARTESIAN_POINT ( 'NONE',  ( -5.629016366058284149, 14.31889596247328633, -229.4177297515988414 ) ) ;
#9684=CARTESIAN_POINT ( 'NONE',  ( -28.00010259152825398, 3.831607968041374157, -225.8381323513402208 ) ) ;
#9685=CARTESIAN_POINT ( 'NONE',  ( -13.83274569775339202, 16.20364235096346661, -234.0851861771356539 ) ) ;
#9686=CARTESIAN_POINT ( 'NONE',  ( 18.50911814746675788, 15.92944434255054453, -232.0449215596906072 ) ) ;
#9687=CARTESIAN_POINT ( 'NONE',  ( 3.755404788550845474, 24.96758616565139022, -220.0839658302907935 ) ) ;
#9689=CARTESIAN_POINT ( 'NONE',  ( 11.87550186346493497, 14.27797038184677270, -220.2068243228838185 ) ) ;
#9690=CARTESIAN_POINT ( 'NONE',  ( -13.88883449434014672, -11.15328429608096172, -217.8357414694029046 ) ) ;
#9691=CARTESIAN_POINT ( 'NONE',  ( 21.53262694368047647, 11.06794636811408594, -231.8394491640143826 ) ) ;
#9692=CARTESIAN_POINT ( 'NONE',  ( 2.374937041136545801, -21.24827930241302099, -215.2851479487023312 ) ) ;
#9694=CARTESIAN_POINT ( 'NONE',  ( -8.611121136347097860, 17.46802294375265419, -231.5575697815534113 ) ) ;
#9696=CARTESIAN_POINT ( 'NONE',  ( 12.31594623278127720, -7.047777776961618557, -228.0736214755532956 ) ) ;
#9698=CARTESIAN_POINT ( 'NONE',  ( 13.25330606581809789, 10.40242132629824034, -230.9170765704288044 ) ) ;
#9699=CARTESIAN_POINT ( 'NONE',  ( -8.407534899841293097, 16.91942258446019665, -231.3029992963236339 ) ) ;
#9700=CARTESIAN_POINT ( 'NONE',  ( -15.39319649241581800, 0.3563955590804028795, -232.4397289486159082 ) ) ;
#9701=CARTESIAN_POINT ( 'NONE',  ( -21.44067990442788840, -11.35877574734454143, -219.4569350636155605 ) ) ;
#9703=CARTESIAN_POINT ( 'NONE',  ( -24.05551141223569545, 2.266836731622281498, -230.7594878221277384 ) ) ;
#9705=CARTESIAN_POINT ( 'NONE',  ( -13.27281469842883688, -16.60017218729922561, -235.3541344917538254 ) ) ;
#9706=CARTESIAN_POINT ( 'NONE',  ( 18.23116248274160256, 13.99874872632082123, -216.0593560670294835 ) ) ;
#9707=CARTESIAN_POINT ( 'NONE',  ( 14.00715608756928532, 4.299235856235253728, -230.2440235370780215 ) ) ;
#9708=CARTESIAN_POINT ( 'NONE',  ( -11.13829636790841704, 14.30978168460582189, -218.6922574227322400 ) ) ;
#9709=CARTESIAN_POINT ( 'NONE',  ( 4.401501667365108617, 18.53594119471695123, -215.1186850315663150 ) ) ;
#9711=CARTESIAN_POINT ( 'NONE',  ( -0.4195811904800660352, -16.41067541138124852, -229.4634529720845819 ) ) ;
#9713=CARTESIAN_POINT ( 'NONE',  ( -3.176860551132370425, -19.01962362838126452, -231.5826211182368297 ) ) ;
#9714=CARTESIAN_POINT ( 'NONE',  ( -12.13692969104051400, -0.3108940857385004697, -222.6170402347994184 ) ) ;
#9715=CARTESIAN_POINT ( 'NONE',  ( 15.84759643368428428, -7.142586963752317608, -231.1761396821659673 ) ) ;
#9716=CARTESIAN_POINT ( 'NONE',  ( -17.21167111787709914, -1.850592482912338799, -230.8442569545952665 ) ) ;
#9717=CARTESIAN_POINT ( 'NONE',  ( -13.88883449434014672, -11.15328429608096172, -217.8357414694029046 ) ) ;
#9718=CARTESIAN_POINT ( 'NONE',  ( 16.43556216695724004, 8.397919695511960825, -216.7971521583719152 ) ) ;
#9720=CARTESIAN_POINT ( 'NONE',  ( -11.05707385098054729, 9.265475627845670914, -220.9763772784480693 ) ) ;
#9721=CARTESIAN_POINT ( 'NONE',  ( 1.217121169770782663, 15.31158828575123110, -230.6845728599757308 ) ) ;
#9722=CARTESIAN_POINT ( 'NONE',  ( 15.74259730902452858, 17.40808440793174583, -232.1327802909178786 ) ) ;
#9723=CARTESIAN_POINT ( 'NONE',  ( 10.15560415551905749, -12.94826033684588928, -216.3500876866647502 ) ) ;
#9724=CARTESIAN_POINT ( 'NONE',  ( 12.98364502352995942, 13.67380631913144029, -233.1535077318696096 ) ) ;
#9725=CARTESIAN_POINT ( 'NONE',  ( -16.51501534778698854, 10.61825396983174485, -230.5082364903317966 ) ) ;
#9726=CARTESIAN_POINT ( 'NONE',  ( -1.198425787605166715, -24.00698511249634137, -218.1862405767648170 ) ) ;
#9728=CARTESIAN_POINT ( 'NONE',  ( -22.00000000000137490, -2.602085213965210642E-15, -216.9999999999999716 ) ) ;
#9729=CARTESIAN_POINT ( 'NONE',  ( 26.24002132888527328, 11.62331517472360964, -222.5300873157218859 ) ) ;
#9730=CARTESIAN_POINT ( 'NONE',  ( 10.49228353591056262, -11.88598183233882644, -227.3718921454133124 ) ) ;
#9732=CARTESIAN_POINT ( 'NONE',  ( -1.890995374385051608, -13.09686096954197509, -227.5694739903412085 ) ) ;
#9734=CARTESIAN_POINT ( 'NONE',  ( -4.104500432947460808, 15.73223271406093460, -218.0734292856946297 ) ) ;
#9736=CARTESIAN_POINT ( 'NONE',  ( 3.982203626615636427, 14.63895582687697150, -217.4952312584269123 ) ) ;
#9738=CARTESIAN_POINT ( 'NONE',  ( 1.217121169770782663, 15.31158828575123110, -230.6845728599757308 ) ) ;
#9739=CARTESIAN_POINT ( 'NONE',  ( -29.74115761720981510, -1.844952462305729401, -220.6656484738778943 ) ) ;
#9742=CARTESIAN_POINT ( 'NONE',  ( -3.643097910890548796, 22.16888955197135047, -233.9701981029593298 ) ) ;
#9743=CARTESIAN_POINT ( 'NONE',  ( -5.131528111146875126, -19.01772154664624992, -215.2265844479019563 ) ) ;
#9744=CARTESIAN_POINT ( 'NONE',  ( 7.486336813247038258, -29.35413437595724773, -221.4114973598149447 ) ) ;
#9745=CARTESIAN_POINT ( 'NONE',  ( 16.85953475301105442, -7.801609028127129086, -231.9437213283852941 ) ) ;
#9746=CARTESIAN_POINT ( 'NONE',  ( -29.98527381603928887, 6.316825171121390525, -230.1108345570740994 ) ) ;
#9747=CARTESIAN_POINT ( 'NONE',  ( 5.466128392039544259, 27.94759090250835243, -223.5617905851570981 ) ) ;
#9748=CARTESIAN_POINT ( 'NONE',  ( -17.84981083811007707, 0.8485253248287054628, -231.8041300026935119 ) ) ;
#9749=CARTESIAN_POINT ( 'NONE',  ( -27.12694304224540076, 7.756125161462346540, -217.3817363082233101 ) ) ;
#9750=CARTESIAN_POINT ( 'NONE',  ( -18.84435272498963343, -14.36455033211084498, -230.7675749430951555 ) ) ;
#9751=CARTESIAN_POINT ( 'NONE',  ( -15.30295614572244922, 9.661125001905515930, -218.8475896279880146 ) ) ;
#9752=CARTESIAN_POINT ( 'NONE',  ( 8.175342817246784577, 19.41817470142738244, -216.6818271833384699 ) ) ;
#9753=CARTESIAN_POINT ( 'NONE',  ( -4.651113456395510326, 27.58151660986499110, -218.3072938287727141 ) ) ;
#9754=CARTESIAN_POINT ( 'NONE',  ( -28.68324149884075780, -4.473022182960058934, -227.9839418391680681 ) ) ;
#9757=CARTESIAN_POINT ( 'NONE',  ( -27.90314475660494153, 12.48829126175061077, -223.3300566725355338 ) ) ;
#9758=CARTESIAN_POINT ( 'NONE',  ( -18.06397433365231819, -19.82544507610489859, -216.4780239895989951 ) ) ;
#9759=CARTESIAN_POINT ( 'NONE',  ( 15.34286276367735979, 1.557318373440422565, -222.4358706187587416 ) ) ;
#9760=CARTESIAN_POINT ( 'NONE',  ( 15.91295838535984331, 21.88410254487826379, -230.9583961155862823 ) ) ;
#9762=CARTESIAN_POINT ( 'NONE',  ( 15.05686526350529775, -5.555778903407086133, -220.1433349335996468 ) ) ;
#9763=CARTESIAN_POINT ( 'NONE',  ( -16.88427011841620029, 9.219900108593305887, -231.9155403335099948 ) ) ;
#9764=CARTESIAN_POINT ( 'NONE',  ( 15.90795275983908574, 2.546196724714939297, -229.0855319561646297 ) ) ;
#9765=PRESENTATION_STYLE_ASSIGNMENT (( #16519 ) ) ;
#9767=DIRECTION ( 'NONE',  ( 1.000000000000000000, 0.000000000000000000, 0.000000000000000000 ) ) ;
#9768=CARTESIAN_POINT ( 'NONE',  ( 21.60524407607017849, 3.028118258437591415, -217.8361640396714449 ) ) ;
#9770=CARTESIAN_POINT ( 'NONE',  ( 24.34559900986324621, -8.951716371391148286, -220.6604487471163623 ) ) ;
#9771=CARTESIAN_POINT ( 'NONE',  ( -23.84209965496292227, -7.976777114481962805, -232.1458837748831456 ) ) ;
#9775=CARTESIAN_POINT ( 'NONE',  ( -16.96626096607909417, 26.06638125783293347, -227.3272535207661349 ) ) ;
#9776=CARTESIAN_POINT ( 'NONE',  ( 10.87654225111433526, -5.446269956799608458, -227.9455542281931741 ) ) ;
#9777=CARTESIAN_POINT ( 'NONE',  ( 16.08921376350389920, -2.840750994787607731, -229.5571464835293796 ) ) ;
#9778=CARTESIAN_POINT ( 'NONE',  ( -13.93825237094548619, 9.044872709574327985, -220.1275804576921757 ) ) ;
#9779=CARTESIAN_POINT ( 'NONE',  ( 17.57135037026572277, 0.09191994211922807634, -232.8447871904542410 ) ) ;
#9780=CARTESIAN_POINT ( 'NONE',  ( 20.59763700141659015, 7.383112456150029423, -232.0722244125682039 ) ) ;
#9781=CARTESIAN_POINT ( 'NONE',  ( 8.773758653197093693, -22.96626044227292951, -216.4280442219689178 ) ) ;
#9782=CARTESIAN_POINT ( 'NONE',  ( 21.31262902390056624, 0.4111834581965390645, -232.0572713672585792 ) ) ;
#9783=CARTESIAN_POINT ( 'NONE',  ( -22.04004491965229207, 12.41871177236473578, -215.2165492276571115 ) ) ;
#9786=CARTESIAN_POINT ( 'NONE',  ( 12.03015173539790617, 23.46358517874481109, -216.0611092640310744 ) ) ;
#9787=CARTESIAN_POINT ( 'NONE',  ( 4.228809304811371739, 12.93497549386982470, -230.7917784105561907 ) ) ;
#9788=CARTESIAN_POINT ( 'NONE',  ( 15.74534598441689504, -4.714293076379259873, -220.2687296774407173 ) ) ;
#9789=CARTESIAN_POINT ( 'NONE',  ( -4.620781219515533778, 16.99182040716223696, -217.1278208835672672 ) ) ;
#9790=CARTESIAN_POINT ( 'NONE',  ( -25.29098058636142810, 5.014641116111857144, -217.4658967307323110 ) ) ;
#9792=CARTESIAN_POINT ( 'NONE',  ( 15.79748369401691122, 19.19631269170049137, -215.0096632418193963 ) ) ;
#9793=CARTESIAN_POINT ( 'NONE',  ( -13.63002737749749826, 6.315035547785179837, -227.0490028799284516 ) ) ;
#9794=CARTESIAN_POINT ( 'NONE',  ( -11.02345917017863464, 29.02019856777526741, -223.9475008740665771 ) ) ;
#9795=CARTESIAN_POINT ( 'NONE',  ( 22.66390650824515873, 11.48342577402021725, -231.3155567808436217 ) ) ;
#9796=CARTESIAN_POINT ( 'NONE',  ( 7.508136856874425114, 24.19512352541684663, -230.0608033085341617 ) ) ;
#9797=CARTESIAN_POINT ( 'NONE',  ( 14.90979066288448429, -1.927202206923867234, -222.7790985701595616 ) ) ;
#9799=CARTESIAN_POINT ( 'NONE',  ( -16.64477864544768337, -2.947896226079009807, -219.6737919733007516 ) ) ;
#9801=CARTESIAN_POINT ( 'NONE',  ( 10.83706092800007781, 10.12544885278926543, -227.1716144446442343 ) ) ;
#9802=CARTESIAN_POINT ( 'NONE',  ( -0.3220389361364618397, -21.73025720764451663, -234.5721229173148856 ) ) ;
#9806=CARTESIAN_POINT ( 'NONE',  ( -14.87932799058895128, 18.71706570923887369, -231.8731726670167745 ) ) ;
#9808=CARTESIAN_POINT ( 'NONE',  ( 7.640685522499278903, -12.22373526560700441, -226.1755943870604710 ) ) ;
#9809=CARTESIAN_POINT ( 'NONE',  ( 11.44717363687632528, 10.34477785005100969, -220.4550508611108341 ) ) ;
#9810=CARTESIAN_POINT ( 'NONE',  ( -4.386767007475907754, 14.39570986262862107, -223.2690175027443615 ) ) ;
#9811=CARTESIAN_POINT ( 'NONE',  ( -28.76901170826145560, 13.32870333992657663, -228.6722616467874616 ) ) ;
#9812=CARTESIAN_POINT ( 'NONE',  ( -16.08069336251900339, -10.46797077187589231, -230.6200287382480383 ) ) ;
#9814=CARTESIAN_POINT ( 'NONE',  ( -22.32700334442577272, 3.978587747811427988, -218.4803616146862453 ) ) ;
#9816=CARTESIAN_POINT ( 'NONE',  ( 23.12216041205843453, 0.2121350054995089496, -232.0572713672589202 ) ) ;
#9817=CARTESIAN_POINT ( 'NONE',  ( 5.803912621764987456, 13.01725692290267844, -221.8367675400179166 ) ) ;
#9819=CARTESIAN_POINT ( 'NONE',  ( -21.18474081038989354, 8.486062504918864491, -230.7949373529753530 ) ) ;
#9821=CARTESIAN_POINT ( 'NONE',  ( 5.773563157792669820, 21.63217468058455140, -235.0383461317610170 ) ) ;
#9823=CARTESIAN_POINT ( 'NONE',  ( 4.213939275857851108, 16.79797086795582928, -215.8378124706958943 ) ) ;
#9824=CARTESIAN_POINT ( 'NONE',  ( -11.81612593381754728, -27.26444769731668671, -229.3107067943240338 ) ) ;
#9826=CARTESIAN_POINT ( 'NONE',  ( 1.304950495335150507, -16.28913491483048759, -229.3926418476436027 ) ) ;
#9827=CARTESIAN_POINT ( 'NONE',  ( -9.722597143579921664, 7.159547510896417499, -227.5730737101346222 ) ) ;
#9828=CARTESIAN_POINT ( 'NONE',  ( 20.98776729843937972, -13.55153944770713359, -217.5092423276211946 ) ) ;
#9829=CARTESIAN_POINT ( 'NONE',  ( 26.13397685888192257, -0.5417465609251845837, -217.5756777990261526 ) ) ;
#9830=CARTESIAN_POINT ( 'NONE',  ( -10.11868820210310282, -13.51996935893276053, -218.1704188629865371 ) ) ;
#9831=CARTESIAN_POINT ( 'NONE',  ( 9.931717191100288389, 12.93133689537362940, -228.8926047089119038 ) ) ;
#9832=DIRECTION ( 'NONE',  ( 0.1093404791528972547, -0.9940043559354329039, 0.000000000000000000 ) ) ;
#9833=CARTESIAN_POINT ( 'NONE',  ( -26.47501633019681577, 13.84484755257420119, -230.0154374881822719 ) ) ;
#9834=CARTESIAN_POINT ( 'NONE',  ( 21.24820809707834357, 20.59746639607275398, -225.8540969741923732 ) ) ;
#9835=CARTESIAN_POINT ( 'NONE',  ( 10.50530447320976535, 20.19629329636330084, -217.1354359361034767 ) ) ;
#9836=CARTESIAN_POINT ( 'NONE',  ( 21.24820809707834357, 20.59746639607275398, -225.8540969741923732 ) ) ;
#9837=CARTESIAN_POINT ( 'NONE',  ( 27.24384134789437439, -15.00887433271272364, -228.9543321217944083 ) ) ;
#9839=CARTESIAN_POINT ( 'NONE',  ( 17.23498165643884761, 6.576565757823654934, -216.5785374982484655 ) ) ;
#9840=CARTESIAN_POINT ( 'NONE',  ( -12.67136363292824086, 22.56975222910433843, -219.0840033572168011 ) ) ;
#9841=CARTESIAN_POINT ( 'NONE',  ( -1.585416880194127520, 15.28258783379090424, -231.0852564988603319 ) ) ;
#9842=CARTESIAN_POINT ( 'NONE',  ( -19.65071121466273496, -22.30814805266854606, -225.1308016072272267 ) ) ;
#9843=CARTESIAN_POINT ( 'NONE',  ( -29.88125065636863198, 4.504452993877526623, -226.2048141718237275 ) ) ;
#9845=CARTESIAN_POINT ( 'NONE',  ( 12.99034161053428349, 11.71468708507361889, -230.9043293568357740 ) ) ;
#9846=CARTESIAN_POINT ( 'NONE',  ( 7.337960271553932046, -12.57654522398025065, -224.9099165242034530 ) ) ;
#9847=CARTESIAN_POINT ( 'NONE',  ( -14.94667331530454213, 6.325011500478772142, -230.0242139990887154 ) ) ;
#9848=CARTESIAN_POINT ( 'NONE',  ( -1.542335193334551491, -19.71915426430242135, -216.1352730594569209 ) ) ;
#9849=CARTESIAN_POINT ( 'NONE',  ( -16.98287383830707142, 1.584866439881522648, -221.5391863673846444 ) ) ;
#9850=CARTESIAN_POINT ( 'NONE',  ( -4.424820997438546399, 11.84746159238278373, -221.7815792475208525 ) ) ;
#9852=CARTESIAN_POINT ( 'NONE',  ( 2.008896548638861024, 20.64812324442097591, -233.5818019448501843 ) ) ;
#9853=CARTESIAN_POINT ( 'NONE',  ( -14.76610802599379291, -3.249507257478274180, -230.1617063156812719 ) ) ;
#9856=CARTESIAN_POINT ( 'NONE',  ( -3.673551555920188783, 29.81207051619892923, -228.8770490300152005 ) ) ;
#9857=CARTESIAN_POINT ( 'NONE',  ( -11.40836237951390508, -18.42461209671423816, -214.6264694599774430 ) ) ;
#9858=CARTESIAN_POINT ( 'NONE',  ( 13.36656406724190305, -19.73987914515934960, -233.3798509643240209 ) ) ;
#9859=CARTESIAN_POINT ( 'NONE',  ( 20.89700225552940793, -4.547446057044195911, -232.3806459760843666 ) ) ;
#9860=CARTESIAN_POINT ( 'NONE',  ( -15.57505478537380306, 24.84242291948262249, -225.5907943047649837 ) ) ;
#9861=CARTESIAN_POINT ( 'NONE',  ( 12.94599882983645145, 15.82237817288049442, -219.3332542656393116 ) ) ;
#9863=CARTESIAN_POINT ( 'NONE',  ( -11.05707385098054729, 9.265475627845670914, -220.9763772784480693 ) ) ;
#9864=CARTESIAN_POINT ( 'NONE',  ( -22.93762879021373280, -16.04239672171475206, -226.2337446402420653 ) ) ;
#9865=CARTESIAN_POINT ( 'NONE',  ( -15.51982305277792307, 19.76957551617798359, -231.4018974401358832 ) ) ;
#9866=CARTESIAN_POINT ( 'NONE',  ( 30.60340911705754863, 5.703403611927857497, -225.1938343315648297 ) ) ;
#9867=CARTESIAN_POINT ( 'NONE',  ( -1.585416880194127520, 15.28258783379090424, -231.0852564988603319 ) ) ;
#9868=CARTESIAN_POINT ( 'NONE',  ( 24.57161139520042781, -7.530326316930160857, -232.9949629211864419 ) ) ;
#9871=CARTESIAN_POINT ( 'NONE',  ( -16.39453490553961856, 20.24836633112041184, -233.1722131570092245 ) ) ;
#9872=CARTESIAN_POINT ( 'NONE',  ( -11.81612593381754728, -27.26444769731668671, -229.3107067943240338 ) ) ;
#9875=CARTESIAN_POINT ( 'NONE',  ( 17.19674704922021391, 23.07334190050143974, -228.8256488842130238 ) ) ;
#9877=CARTESIAN_POINT ( 'NONE',  ( 25.54997870115619207, -2.097555195297153841, -218.7002440566220400 ) ) ;
#9878=CARTESIAN_POINT ( 'NONE',  ( -13.55591840520136770, 8.363404288414606924, -231.2690188357804857 ) ) ;
#9880=CARTESIAN_POINT ( 'NONE',  ( -11.01414002179357610, 8.614420160880040811, -226.3770540798392972 ) ) ;
#9881=CARTESIAN_POINT ( 'NONE',  ( 17.76485367938521875, 4.373152267827974171, -218.8623009891758215 ) ) ;
#9882=FACE_OUTER_BOUND ( 'NONE', #2414, .T. ) ;
#9884=CARTESIAN_POINT ( 'NONE',  ( -14.10849459794400751, -0.2436790717799666162, -223.1085195285415921 ) ) ;
#9885=CARTESIAN_POINT ( 'NONE',  ( 17.02517607141322031, -4.660589389729973497, -229.0519452290894833 ) ) ;
#9886=CARTESIAN_POINT ( 'NONE',  ( -18.34948365288241590, -1.907751280579004893, -231.5848060246952116 ) ) ;
#9889=CARTESIAN_POINT ( 'NONE',  ( 11.21155440434494643, 24.57152134148167733, -221.7155903571010356 ) ) ;
#9890=CARTESIAN_POINT ( 'NONE',  ( 3.924989892941122438, -14.79802789183876044, -219.9433972157300445 ) ) ;
#9892=CARTESIAN_POINT ( 'NONE',  ( 12.73130673999417795, -23.76414828096303467, -217.7386337832039942 ) ) ;
#9894=CARTESIAN_POINT ( 'NONE',  ( -13.70798801564395752, 13.71024986321384809, -218.3360451569033955 ) ) ;
#9895=CARTESIAN_POINT ( 'NONE',  ( 21.04928763009552384, -0.2309942901367783852, -233.9427286327411366 ) ) ;
#9896=CARTESIAN_POINT ( 'NONE',  ( 23.74723497152361062, 5.524508269105988134, -217.6012181427065002 ) ) ;
#9898=CARTESIAN_POINT ( 'NONE',  ( 5.229904874806564408, -24.29892824652383609, -233.0630010234598046 ) ) ;
#9900=CARTESIAN_POINT ( 'NONE',  ( -17.58289524052909414, 0.7988212499981205417, -233.9567931471624149 ) ) ;
#9902=CARTESIAN_POINT ( 'NONE',  ( 10.35958063030883025, 8.003303894222913328, -225.9303204057916048 ) ) ;
#9903=CARTESIAN_POINT ( 'NONE',  ( -0.3984245442872364484, 11.77931270252508789, -223.1826369159892920 ) ) ;
#9904=CARTESIAN_POINT ( 'NONE',  ( 21.28979032490934031, -14.07620925358629727, -230.4022181401844875 ) ) ;
#9905=CARTESIAN_POINT ( 'NONE',  ( -7.825349071214003693, 24.14595706726266755, -216.5959661901539732 ) ) ;
#9906=CARTESIAN_POINT ( 'NONE',  ( -15.20262116893801974, 8.038155052917188570, -217.6767387945475036 ) ) ;
#9909=CARTESIAN_POINT ( 'NONE',  ( 6.523529190399725231, 13.69551997595937465, -217.3678933099786832 ) ) ;
#9911=CARTESIAN_POINT ( 'NONE',  ( -23.43012680803641956, 15.46310457140252304, -230.0052977649806962 ) ) ;
#9912=CARTESIAN_POINT ( 'NONE',  ( -9.517741096562200909, 20.63709896626785678, -234.1036702156204967 ) ) ;
#9914=CARTESIAN_POINT ( 'NONE',  ( 6.225744896574323839, 14.38227537199079720, -224.8391693295998266 ) ) ;
#9915=CARTESIAN_POINT ( 'NONE',  ( 16.08921376350389920, -2.840750994787607731, -229.5571464835293796 ) ) ;
#9918=CARTESIAN_POINT ( 'NONE',  ( 18.46552355142154411, 5.019711608606525211, -231.5099115070375433 ) ) ;
#9919=CARTESIAN_POINT ( 'NONE',  ( -19.73058714482073128, -19.33240507441191625, -228.8766180877602494 ) ) ;
#9921=CARTESIAN_POINT ( 'NONE',  ( -4.067324790461362305, 15.10342260507846746, -228.2464404076259257 ) ) ;
#9922=CARTESIAN_POINT ( 'NONE',  ( 10.05733608402134216, -9.620616164199983444, -224.9449885650552119 ) ) ;
#9923=CARTESIAN_POINT ( 'NONE',  ( 12.49127101283658803, 6.474961340449192804, -221.2149164507559078 ) ) ;
#9924=CARTESIAN_POINT ( 'NONE',  ( -7.873497077133136735, 15.44270125396616677, -230.2562282217168672 ) ) ;
#9925=CARTESIAN_POINT ( 'NONE',  ( -8.328662059352005542, 28.53523473722178139, -221.4280032538016201 ) ) ;
#9927=CARTESIAN_POINT ( 'NONE',  ( -16.25683815890624473, -3.869351682469674980, -222.5551530127839044 ) ) ;
#9930=CARTESIAN_POINT ( 'NONE',  ( -20.84243560023798736, 1.479777185913828230, -230.9766426496277631 ) ) ;
#9932=CARTESIAN_POINT ( 'NONE',  ( -29.78324924674133456, -0.2661018803894699136, -229.0431670511964057 ) ) ;
#9933=CARTESIAN_POINT ( 'NONE',  ( 11.01659168199870287, 19.17922986229587323, -233.3715978632214387 ) ) ;
#9934=CARTESIAN_POINT ( 'NONE',  ( -15.82036597035495795, 4.920771916499852239, -223.0095317795067160 ) ) ;
#9935=CARTESIAN_POINT ( 'NONE',  ( 2.770531592831002143, 22.28948935999365943, -215.1307751200139649 ) ) ;
#9936=CARTESIAN_POINT ( 'NONE',  ( 22.37138132874926910, 6.723028048925958622, -217.7073806909121743 ) ) ;
#9940=CARTESIAN_POINT ( 'NONE',  ( -19.49800774256867086, -24.03546784425654792, -228.3621204403185061 ) ) ;
#9942=CARTESIAN_POINT ( 'NONE',  ( -19.75205891382245227, -22.10994567413457546, -223.7241504221178729 ) ) ;
#9943=CARTESIAN_POINT ( 'NONE',  ( -29.15345109632842124, 14.07532767497844262, -225.0972140442887621 ) ) ;
#9944=CARTESIAN_POINT ( 'NONE',  ( 8.818493748348606331, -10.89961555176610375, -227.9481955143288303 ) ) ;
#9945=CARTESIAN_POINT ( 'NONE',  ( -29.27492217116574480, -1.185422171198730501, -224.8132346143397342 ) ) ;
#9946=CARTESIAN_POINT ( 'NONE',  ( -14.73155177304599306, -1.817590056890399763, -226.9769936995019748 ) ) ;
#9947=CARTESIAN_POINT ( 'NONE',  ( 24.49559427486850893, 14.86117239466233642, -230.3058416388274736 ) ) ;
#9950=CARTESIAN_POINT ( 'NONE',  ( -21.95649697515285581, 20.70968357470995258, -226.9638023349746447 ) ) ;
#9951=CARTESIAN_POINT ( 'NONE',  ( 13.41709597927210496, 19.57823531746157997, -218.2666972400567147 ) ) ;
#9952=CARTESIAN_POINT ( 'NONE',  ( 8.496844655769807630, 14.66037471857024599, -219.1631158796573118 ) ) ;
#9953=CARTESIAN_POINT ( 'NONE',  ( 15.50648685944955218, 24.16641006378193168, -224.4827813270165393 ) ) ;
#9954=CARTESIAN_POINT ( 'NONE',  ( 14.71544223636061410, -24.97731814513734605, -232.6985170686097320 ) ) ;
#9955=CARTESIAN_POINT ( 'NONE',  ( -9.222253059793434460, 13.27185325399938165, -229.0864811363590547 ) ) ;
#9956=CARTESIAN_POINT ( 'NONE',  ( -16.71711190488355570, 0.6105529133557690002, -230.9511258789794681 ) ) ;
#9958=CARTESIAN_POINT ( 'NONE',  ( 10.78187269046063435, 10.73871010366167944, -221.9206544238666368 ) ) ;
#9959=CARTESIAN_POINT ( 'NONE',  ( 11.40994021191102092, -13.94644022156852969, -230.1289083636806936 ) ) ;
#9960=CARTESIAN_POINT ( 'NONE',  ( -13.37045227479810094, 5.250293981428504786, -224.2914120185227205 ) ) ;
#9961=CARTESIAN_POINT ( 'NONE',  ( 9.336393807558161839, 27.79372469574263960, -228.5913636680961361 ) ) ;
#9962=CARTESIAN_POINT ( 'NONE',  ( -18.53787071664277519, -6.556543064843903146, -232.5192140591401824 ) ) ;
#9963=CARTESIAN_POINT ( 'NONE',  ( -19.67797246974518544, 1.229961341702398681, -219.4743747885323160 ) ) ;
#9964=CARTESIAN_POINT ( 'NONE',  ( 19.66580438618080251, 15.18147523775131624, -233.5153994334876586 ) ) ;
#9966=CARTESIAN_POINT ( 'NONE',  ( 5.331555957413248059, 27.50712867803999728, -219.0801070358024276 ) ) ;
#9967=CARTESIAN_POINT ( 'NONE',  ( 23.10971261601581617, -16.35996695089516706, -224.5402406813554421 ) ) ;
#9968=CARTESIAN_POINT ( 'NONE',  ( 15.07245478799217686, -4.018468087397350175, -231.0118529037252699 ) ) ;
#9970=CARTESIAN_POINT ( 'NONE',  ( -2.934221234790329369, 15.07857928364152222, -230.9558365497803720 ) ) ;
#9971=CARTESIAN_POINT ( 'NONE',  ( -27.72233273893307981, -16.15685914833838410, -223.8945077613443289 ) ) ;
#9972=CARTESIAN_POINT ( 'NONE',  ( 6.131461862964278531, -15.14974102410872625, -231.6805438559109973 ) ) ;
#9973=CARTESIAN_POINT ( 'NONE',  ( 9.104026917753444081, -10.66572815660443041, -221.9193219976906448 ) ) ;
#9974=CARTESIAN_POINT ( 'NONE',  ( -16.65220264499505376, 11.77543314451157563, -216.3149620944649030 ) ) ;
#9975=CARTESIAN_POINT ( 'NONE',  ( 9.280831573919673616, 14.67893982993557422, -228.6940810986570796 ) ) ;
#9976=CARTESIAN_POINT ( 'NONE',  ( -20.43618815875133521, 1.403378831510147196, -232.9646741665398224 ) ) ;
#9977=CARTESIAN_POINT ( 'NONE',  ( -24.79170285622992509, 4.551775110860766915, -234.5907228154019322 ) ) ;
#9978=CARTESIAN_POINT ( 'NONE',  ( -14.51900513504577717, -8.991447007532661573, -221.0515111571761793 ) ) ;
#9980=CARTESIAN_POINT ( 'NONE',  ( -12.78923236353123727, 15.53885160143439315, -231.8946633672937878 ) ) ;
#9981=CARTESIAN_POINT ( 'NONE',  ( 21.77183241683778547, 12.04504704525620085, -233.6005549158834640 ) ) ;
#9982=CARTESIAN_POINT ( 'NONE',  ( -5.629016366058284149, 14.31889596247328633, -229.4177297515988414 ) ) ;
#9984=CARTESIAN_POINT ( 'NONE',  ( 13.39541376241636783, -3.462025909069690321, -228.4300562622815391 ) ) ;
#9987=CARTESIAN_POINT ( 'NONE',  ( -15.66530208164916260, 23.23467148471576849, -218.1250122661128046 ) ) ;
#9988=CARTESIAN_POINT ( 'NONE',  ( -13.00317340065129557, -2.278067296278880161, -219.8118061108488916 ) ) ;
#9990=CARTESIAN_POINT ( 'NONE',  ( 12.58590500897257947, 11.38573988265384607, -230.4867078522624695 ) ) ;
#9992=CARTESIAN_POINT ( 'NONE',  ( 24.05826999138443156, -14.97270453765939102, -220.1026142722873260 ) ) ;
#9993=CARTESIAN_POINT ( 'NONE',  ( -16.71711190488355570, 0.6105529133557690002, -230.9511258789794681 ) ) ;
#9994=CARTESIAN_POINT ( 'NONE',  ( -18.41237742040652847, 14.06446039901721790, -216.7469276929859632 ) ) ;
#9995=CARTESIAN_POINT ( 'NONE',  ( 28.62253243811995418, 3.652502539191337494, -225.4068779441649326 ) ) ;
#9996=CARTESIAN_POINT ( 'NONE',  ( -0.8337089444836248697, -27.22572500676309559, -220.1932236949194532 ) ) ;
#10000=CARTESIAN_POINT ( 'NONE',  ( 17.01404819207892061, -3.492736430306117690, -221.2516733069050190 ) ) ;
#10001=CARTESIAN_POINT ( 'NONE',  ( -14.40111287326894640, -6.123720356435734757, -220.5571602876142094 ) ) ;
#10004=CARTESIAN_POINT ( 'NONE',  ( 7.951191770265756631, 20.55701948568933091, -231.2149185317973661 ) ) ;
#10005=CARTESIAN_POINT ( 'NONE',  ( 4.286954182150454429, -15.41507397180808425, -219.0323159710399352 ) ) ;
#10006=CARTESIAN_POINT ( 'NONE',  ( 19.68037530048075112, -17.97179847169212508, -231.8517058357153076 ) ) ;
#10007=CARTESIAN_POINT ( 'NONE',  ( -10.32994309255856535, 16.55762392127841665, -218.3313395458419279 ) ) ;
#10008=CARTESIAN_POINT ( 'NONE',  ( 20.13946171159960841, -0.1427001808266660232, -233.7987036390019853 ) ) ;
#10009=CARTESIAN_POINT ( 'NONE',  ( 24.52860916307685457, 12.75391509163817361, -221.3604763108436941 ) ) ;
#10010=CARTESIAN_POINT ( 'NONE',  ( -11.27700245477877772, -16.92453807419676792, -219.4498264308321609 ) ) ;
#10012=CARTESIAN_POINT ( 'NONE',  ( -22.61701582078733708, 5.416317966792455252, -214.6955127214549748 ) ) ;
#10014=CARTESIAN_POINT ( 'NONE',  ( 9.533850545951205291, 16.09136358716069637, -215.9093469876620475 ) ) ;
#10015=CARTESIAN_POINT ( 'NONE',  ( 22.40610909459028122, -16.32493987272327018, -222.3848458449739951 ) ) ;
#10016=CARTESIAN_POINT ( 'NONE',  ( 1.382955251742491898, 16.46353944795171032, -231.7743150979565030 ) ) ;
#10017=CARTESIAN_POINT ( 'NONE',  ( -17.84981083811007707, 0.8485253248287054628, -231.8041300026935119 ) ) ;
#10019=CARTESIAN_POINT ( 'NONE',  ( 17.65694480011521250, 15.62497337860048674, -235.2008064134603273 ) ) ;
#10020=CARTESIAN_POINT ( 'NONE',  ( -18.91027996815576628, 5.295101183552822555, -231.2253513302548527 ) ) ;
#10022=CARTESIAN_POINT ( 'NONE',  ( -6.282398543089500187, 12.01615879894893801, -228.5121145169883903 ) ) ;
#10024=CARTESIAN_POINT ( 'NONE',  ( 3.281983756374524663, 15.83593597903271721, -223.8697822987047346 ) ) ;
#10025=CARTESIAN_POINT ( 'NONE',  ( 29.17814965709308694, -1.309718763918959139, -225.2029557489520926 ) ) ;
#10028=CARTESIAN_POINT ( 'NONE',  ( 19.20300624114736721, 0.6066039755357417462, -231.5046416827383950 ) ) ;
#10029=CARTESIAN_POINT ( 'NONE',  ( -21.59231333450971135, -13.53975872187591989, -230.0942117760813517 ) ) ;
#10032=CARTESIAN_POINT ( 'NONE',  ( -11.16203726658389606, 26.27101666727781648, -227.8592829514190612 ) ) ;
#10033=CARTESIAN_POINT ( 'NONE',  ( 5.380811198380419214, -14.52623441703906160, -221.9013399998540024 ) ) ;
#10034=CARTESIAN_POINT ( 'NONE',  ( 13.60311248493089131, 7.003372205918751092, -219.1738832909067867 ) ) ;
#10035=CARTESIAN_POINT ( 'NONE',  ( -9.627017372966443887, 15.60690227900018279, -218.8878023709062859 ) ) ;
#10036=CARTESIAN_POINT ( 'NONE',  ( -23.70973587455150522, 20.45398817402440983, -228.9005348699235469 ) ) ;
#10039=CARTESIAN_POINT ( 'NONE',  ( 27.82583766398256486, 0.7543585032809253521, -232.9329547162639358 ) ) ;
#10040=CARTESIAN_POINT ( 'NONE',  ( 10.66614775643814994, 26.29080367171353672, -230.0818785118670178 ) ) ;
#10041=CARTESIAN_POINT ( 'NONE',  ( -27.11599398522282911, 10.60460483532474996, -224.7310548435675912 ) ) ;
#10042=CARTESIAN_POINT ( 'NONE',  ( -16.90857133559978465, -0.4126725064255206687, -221.6276144895144569 ) ) ;
#10044=CARTESIAN_POINT ( 'NONE',  ( -30.11338598929818389, -8.317867968210222784, -227.6364879822423006 ) ) ;
#10045=CARTESIAN_POINT ( 'NONE',  ( 11.64932556965463561, 7.668732705389711413, -229.0406978839571366 ) ) ;
#10046=CARTESIAN_POINT ( 'NONE',  ( -26.87016840655871874, 6.086699737350822481, -222.9228935003981746 ) ) ;
#10047=CARTESIAN_POINT ( 'NONE',  ( 1.833772325875588027, 13.50593961039006707, -219.8748197804281119 ) ) ;
#10048=CARTESIAN_POINT ( 'NONE',  ( 18.55287065739596031, 7.869864349944380777, -232.8430408253643691 ) ) ;
#10049=CARTESIAN_POINT ( 'NONE',  ( -10.04615645102154886, -9.695712423306433791, -230.4834384258168996 ) ) ;
#10051=CARTESIAN_POINT ( 'NONE',  ( -14.03072379416114757, -18.13329758221107824, -232.5220584501505812 ) ) ;
#10052=CARTESIAN_POINT ( 'NONE',  ( -11.79271689233719478, 3.876813423829604144, -228.6816298097564299 ) ) ;
#10053=CARTESIAN_POINT ( 'NONE',  ( 5.953549895739506326, -12.70069413479034104, -221.3143591192976203 ) ) ;
#10054=CARTESIAN_POINT ( 'NONE',  ( -3.082945806077231676, 30.69897765966285874, -224.2387254578930822 ) ) ;
#10055=CARTESIAN_POINT ( 'NONE',  ( 21.04926289057418742, -6.455467962217539934, -215.4677037730695872 ) ) ;
#10056=CARTESIAN_POINT ( 'NONE',  ( -13.72709560065558421, -5.132649126379569715, -227.9317987811764965 ) ) ;
#10057=CARTESIAN_POINT ( 'NONE',  ( 14.29768887814754663, 10.87030385293788548, -231.8067013864770161 ) ) ;
#10058=CARTESIAN_POINT ( 'NONE',  ( -9.403561938624596550, 12.70246821120386471, -220.7484614495429582 ) ) ;
#10059=CARTESIAN_POINT ( 'NONE',  ( 10.49810582199713416, 9.357428619962972149, -224.5466107281195605 ) ) ;
#10060=CARTESIAN_POINT ( 'NONE',  ( 12.99034161053428349, 11.71468708507361889, -230.9043293568357740 ) ) ;
#10061=CARTESIAN_POINT ( 'NONE',  ( 10.98110116949302828, 13.70618071521442971, -230.2797640191687378 ) ) ;
#10062=CARTESIAN_POINT ( 'NONE',  ( 9.867031390707305505, -6.965612358230354850, -226.9368589251366188 ) ) ;
#10063=CARTESIAN_POINT ( 'NONE',  ( -2.047892494109819328, 12.88402507277750786, -223.5104301352110951 ) ) ;
#10064=CARTESIAN_POINT ( 'NONE',  ( -13.10651848559790444, 3.262242204071156948, -224.3513854875720597 ) ) ;
#10067=CARTESIAN_POINT ( 'NONE',  ( 8.716925653960343467, -14.61958666771473858, -219.5525962724747444 ) ) ;
#10068=CARTESIAN_POINT ( 'NONE',  ( -19.74163224554151697, 8.726897413558679872, -232.6665747339030190 ) ) ;
#10069=CARTESIAN_POINT ( 'NONE',  ( -3.494873682963683059, 27.70407912598904687, -220.5214894769905243 ) ) ;
#10070=CARTESIAN_POINT ( 'NONE',  ( -15.22366728182010043, -5.552021002219007961, -230.2511309519622671 ) ) ;
#10071=CARTESIAN_POINT ( 'NONE',  ( -21.48978835671764287, 1.062155088816892468, -219.0000000007146355 ) ) ;
#10072=CARTESIAN_POINT ( 'NONE',  ( 24.78222556642275620, 17.97262539535998371, -226.6641400693514470 ) ) ;
#10074=CARTESIAN_POINT ( 'NONE',  ( 4.883314309504700468, 19.06839645569368358, -217.0171359871271193 ) ) ;
#10075=CARTESIAN_POINT ( 'NONE',  ( 11.60500945006145024, -11.05507752957471190, -226.0500390094313730 ) ) ;
#10076=CARTESIAN_POINT ( 'NONE',  ( 17.44158214791148964, -8.186237638883257617, -216.9355394212118995 ) ) ;
#10078=CARTESIAN_POINT ( 'NONE',  ( -1.881996891245037995, 28.05344686410985489, -218.6379207300106202 ) ) ;
#10079=CARTESIAN_POINT ( 'NONE',  ( -9.664312646807834639, -7.057764824546099547, -227.2890491868971594 ) ) ;
#10080=CARTESIAN_POINT ( 'NONE',  ( -13.60146639818222702, -25.11808310587244009, -230.9974232610874196 ) ) ;
#10081=CARTESIAN_POINT ( 'NONE',  ( 21.30961698559626427, -20.48616475849644303, -228.5322376518520002 ) ) ;
#10082=CARTESIAN_POINT ( 'NONE',  ( -21.75607741976026333, 20.26169853110213381, -228.4128163609909450 ) ) ;
#10083=CARTESIAN_POINT ( 'NONE',  ( 14.12692363916921146, 20.59586666873830296, -230.0804552526094540 ) ) ;
#10084=CARTESIAN_POINT ( 'NONE',  ( -23.49379658590067876, 11.46840048879614393, -217.2519070826072323 ) ) ;
#10085=CARTESIAN_POINT ( 'NONE',  ( -12.45629340980802269, 5.675423426979704367, -220.8874502847910719 ) ) ;
#10086=CARTESIAN_POINT ( 'NONE',  ( -13.68888474783054399, -8.264665463295720826, -223.0168115903771024 ) ) ;
#10088=CARTESIAN_POINT ( 'NONE',  ( -4.490213599459100813, 14.55066867058898694, -222.6488251579668827 ) ) ;
#10089=CARTESIAN_POINT ( 'NONE',  ( 14.63115627273841923, 9.024791562541032874, -232.5054678133655841 ) ) ;
#10090=CARTESIAN_POINT ( 'NONE',  ( 10.86206282953156510, 30.27427353967719981, -226.0953027964478110 ) ) ;
#10091=CARTESIAN_POINT ( 'NONE',  ( 17.44158214791148964, -8.186237638883257617, -216.9355394212118995 ) ) ;
#10095=CARTESIAN_POINT ( 'NONE',  ( -22.11084984981285118, 10.96048252433489623, -216.6117774006995376 ) ) ;
#10096=CARTESIAN_POINT ( 'NONE',  ( -14.84991717770350661, -12.66914290363892270, -234.6513150936106626 ) ) ;
#10098=CARTESIAN_POINT ( 'NONE',  ( 10.55627441269396094, 10.31758739525044888, -223.1990319438957613 ) ) ;
#10100=CARTESIAN_POINT ( 'NONE',  ( 12.13827923251525220, -9.172799829723585319, -229.1860353116090891 ) ) ;
#10102=CARTESIAN_POINT ( 'NONE',  ( -27.90314475660494153, 12.48829126175061077, -223.3300566725355338 ) ) ;
#10103=CARTESIAN_POINT ( 'NONE',  ( 16.20788843645364352, 6.828976201867700269, -231.6689701909764665 ) ) ;
#10104=CARTESIAN_POINT ( 'NONE',  ( -13.53581065110708970, -26.13331550560631555, -224.9773145811678887 ) ) ;
#10107=CARTESIAN_POINT ( 'NONE',  ( 14.63113973005795643, 4.926264598692385199, -222.4866305912601945 ) ) ;
#10108=CARTESIAN_POINT ( 'NONE',  ( 10.49228353591056262, -11.88598183233882644, -227.3718921454133124 ) ) ;
#10109=CARTESIAN_POINT ( 'NONE',  ( 14.16658675964390923, -1.854297863920779221, -227.3584270016860103 ) ) ;
#10111=CARTESIAN_POINT ( 'NONE',  ( 8.162622027327667951, 13.88735946031204094, -224.7165241036068153 ) ) ;
#10112=CARTESIAN_POINT ( 'NONE',  ( 2.914696262605396715, 19.49933023975583879, -231.6035545612375017 ) ) ;
#10114=CARTESIAN_POINT ( 'NONE',  ( 9.772444363920737231, -9.146208674228628155, -219.7841758423534486 ) ) ;
#10115=CARTESIAN_POINT ( 'NONE',  ( 14.18709644517307922, -11.45356969546147496, -232.2178450427173004 ) ) ;
#10117=CARTESIAN_POINT ( 'NONE',  ( -11.05032764129755840, 11.65053160594169945, -221.1796278216217218 ) ) ;
#10118=CARTESIAN_POINT ( 'NONE',  ( 26.91963614581376874, 6.107751173605064920, -232.2246916053503298 ) ) ;
#10119=CARTESIAN_POINT ( 'NONE',  ( 14.03916608299427082, 11.26328028684000415, -220.2447382113059007 ) ) ;
#10121=CARTESIAN_POINT ( 'NONE',  ( -3.614824051224299950, -15.07124992037100064, -223.1721701483932065 ) ) ;
#10123=CARTESIAN_POINT ( 'NONE',  ( -20.02994071726468661, 1.326980477106467271, -234.9527056834518532 ) ) ;
#10125=CARTESIAN_POINT ( 'NONE',  ( 18.39533937270110187, 14.26564464607222504, -233.9088367426310242 ) ) ;
#10126=CARTESIAN_POINT ( 'NONE',  ( 11.72806877847873253, -14.77654346318461975, -220.1368134445341695 ) ) ;
#10127=CARTESIAN_POINT ( 'NONE',  ( 7.743212835174657194, 11.90778931056080481, -226.0491028376908105 ) ) ;
#10128=CARTESIAN_POINT ( 'NONE',  ( -12.78558550453068854, 7.693178343823584342, -230.0800953344970878 ) ) ;
#10129=CARTESIAN_POINT ( 'NONE',  ( 25.12984891811676036, 19.96069634721137476, -226.7154725927711070 ) ) ;
#10130=CARTESIAN_POINT ( 'NONE',  ( -23.30382222616342247, 9.914163031146200566, -218.5285240371296425 ) ) ;
#10132=CARTESIAN_POINT ( 'NONE',  ( -0.9414827276148034496, 23.96885519606619752, -216.4491898092606164 ) ) ;
#10133=FACE_OUTER_BOUND ( 'NONE', #6623, .T. ) ;
#10134=CARTESIAN_POINT ( 'NONE',  ( -0.1947256686167265494, -30.94043057420685727, -223.1178397439027492 ) ) ;
#10137=CARTESIAN_POINT ( 'NONE',  ( -18.53787071664277519, -6.556543064843903146, -232.5192140591401824 ) ) ;
#10138=CARTESIAN_POINT ( 'NONE',  ( -21.85741505224184777, 1.741064654082184582, -235.1654459941842390 ) ) ;
#10139=CARTESIAN_POINT ( 'NONE',  ( -16.08690871037762449, -24.16943144049835368, -222.8355329163958345 ) ) ;
#10142=CARTESIAN_POINT ( 'NONE',  ( 5.452943511046377090, -14.64908918772281865, -221.6090591728701611 ) ) ;
#10143=CARTESIAN_POINT ( 'NONE',  ( 10.25308675723727347, 13.16459519580956972, -229.3963488176951273 ) ) ;
#10144=CARTESIAN_POINT ( 'NONE',  ( -14.94618804342693075, 22.09718979644185666, -219.6454806548149463 ) ) ;
#10145=CARTESIAN_POINT ( 'NONE',  ( -17.81561310496929806, 18.25637658208611569, -215.7745954696244439 ) ) ;
#10147=CARTESIAN_POINT ( 'NONE',  ( 12.24504971509987072, -1.481354005294047926, -221.9045230856115438 ) ) ;
#10149=CARTESIAN_POINT ( 'NONE',  ( 15.33737796850231305, 13.57479350230705428, -232.3313557812109025 ) ) ;
#10150=CARTESIAN_POINT ( 'NONE',  ( -18.91027996815576628, 5.295101183552822555, -231.2253513302548527 ) ) ;
#10151=CARTESIAN_POINT ( 'NONE',  ( 29.21307215008108216, 4.139194015751272104, -229.9658791484231699 ) ) ;
#10154=CARTESIAN_POINT ( 'NONE',  ( 7.018811797190238622, 13.93862807232938472, -230.2855929063610176 ) ) ;
#10155=CARTESIAN_POINT ( 'NONE',  ( -23.52458685063474420, 4.195399146287285497, -230.7490123595086970 ) ) ;
#10156=CARTESIAN_POINT ( 'NONE',  ( -5.566280468132954518, 29.91920859341914962, -222.2705790733167817 ) ) ;
#10157=CARTESIAN_POINT ( 'NONE',  ( 24.34047711160105720, 17.90454708687460794, -228.1939002122307159 ) ) ;
#10158=CARTESIAN_POINT ( 'NONE',  ( -5.902345112435694041, -11.50736153130091388, -224.0878888885884805 ) ) ;
#10161=CARTESIAN_POINT ( 'NONE',  ( -6.266309075335420253, -15.78290365675015572, -230.2363798222519051 ) ) ;
#10162=CARTESIAN_POINT ( 'NONE',  ( -17.92628912275201003, -0.6090139417824500523, -215.7724435048976943 ) ) ;
#10163=CARTESIAN_POINT ( 'NONE',  ( 8.510712203779903007, -27.79691582975998898, -230.5316902582456180 ) ) ;
#10164=CARTESIAN_POINT ( 'NONE',  ( -3.843007962268670585, 27.94983497691806917, -231.4302614368887703 ) ) ;
#10165=CARTESIAN_POINT ( 'NONE',  ( 13.42973690470193837, -10.83953015014330035, -233.9990574442320224 ) ) ;
#10166=CARTESIAN_POINT ( 'NONE',  ( -22.20848920810297855, -2.028924892417935055, -232.4401719831211039 ) ) ;
#10167=CARTESIAN_POINT ( 'NONE',  ( 21.27834046766391651, 19.84195992785746654, -221.8454931627593965 ) ) ;
#10169=CARTESIAN_POINT ( 'NONE',  ( -19.01002492504315811, 19.85266905124972681, -219.0021410556803687 ) ) ;
#10170=CARTESIAN_POINT ( 'NONE',  ( 12.54860906168727652, 6.077542143275485031, -228.1605930327268368 ) ) ;
#10171=CARTESIAN_POINT ( 'NONE',  ( 14.31308345469695453, 12.76656023072872159, -231.9445021321040770 ) ) ;
#10172=CARTESIAN_POINT ( 'NONE',  ( 14.61121792518381390, 23.81825453963186590, -227.9329146581663110 ) ) ;
#10173=CARTESIAN_POINT ( 'NONE',  ( 5.326148043627311424, -14.37544986528147639, -217.4292808685971750 ) ) ;
#10174=CARTESIAN_POINT ( 'NONE',  ( -13.14888680331901583, 26.03314517226533908, -227.7900104434697539 ) ) ;
#10176=CARTESIAN_POINT ( 'NONE',  ( 21.60524407607017849, 3.028118258437591415, -217.8361640396714449 ) ) ;
#10177=CARTESIAN_POINT ( 'NONE',  ( 4.343570314325058135, -14.31236505836544026, -220.3716640818165615 ) ) ;
#10178=CARTESIAN_POINT ( 'NONE',  ( -18.94992041651601156, 14.87246523864368974, -232.0280096192260828 ) ) ;
#10179=CARTESIAN_POINT ( 'NONE',  ( -4.866400999161825780, 25.69921167300892861, -231.0100031340613782 ) ) ;
#10181=CARTESIAN_POINT ( 'NONE',  ( -14.13781561609191328, -15.90667165809925621, -233.6615929499251649 ) ) ;
#10182=CARTESIAN_POINT ( 'NONE',  ( 15.51129552754472307, 0.2180314803830030457, -231.3815478022924879 ) ) ;
#10183=CARTESIAN_POINT ( 'NONE',  ( 7.739849882373770917, 11.59357455229016409, -219.5521933286238720 ) ) ;
#10184=CARTESIAN_POINT ( 'NONE',  ( 15.12287735332712835, 21.03907941686458116, -231.7894952627153202 ) ) ;
#10185=CARTESIAN_POINT ( 'NONE',  ( 22.30453140437255044, -8.121595866981794032, -232.1448055058014575 ) ) ;
#10186=CARTESIAN_POINT ( 'NONE',  ( 16.80562970167152415, -4.609754314392994878, -232.4812892975905356 ) ) ;
#10188=CARTESIAN_POINT ( 'NONE',  ( -0.1571923090946999446, 19.34188126963334398, -216.6893131123363787 ) ) ;
#10189=CARTESIAN_POINT ( 'NONE',  ( -29.73963803141277396, -7.146848409970624871, -220.9878827551818858 ) ) ;
#10190=CARTESIAN_POINT ( 'NONE',  ( -11.06377138986482933, -15.30386857868810857, -217.0411070525910873 ) ) ;
#10192=CARTESIAN_POINT ( 'NONE',  ( 9.584731462935641488, -12.36622837314704348, -230.4796538097028531 ) ) ;
#10194=CARTESIAN_POINT ( 'NONE',  ( -13.30451247859013897, 19.85560227862636040, -232.3493821534129609 ) ) ;
#10195=CARTESIAN_POINT ( 'NONE',  ( 5.549682179574114471, 15.11687613544382280, -226.9959476502473308 ) ) ;
#10196=CARTESIAN_POINT ( 'NONE',  ( -13.11494368899652052, 3.355507568391938200, -225.9121440085824304 ) ) ;
#10197=CARTESIAN_POINT ( 'NONE',  ( -26.47501633019681577, 13.84484755257420119, -230.0154374881822719 ) ) ;
#10198=CARTESIAN_POINT ( 'NONE',  ( -12.84507615163359873, -10.94093879717347129, -227.8208865714805142 ) ) ;
#10199=EDGE_LOOP ( 'NONE', ( #2549, #6551, #14923, #2408, #17381, #12582, #817 ) ) ;
#10200=CARTESIAN_POINT ( 'NONE',  ( -13.51991436508781597, 16.61129329384914755, -232.1184346153593197 ) ) ;
#10201=CARTESIAN_POINT ( 'NONE',  ( 21.38922145650625239, 17.10616209967719215, -217.8354246241890451 ) ) ;
#10202=CARTESIAN_POINT ( 'NONE',  ( 21.77779027533950540, 18.43917590911969029, -232.9503911151153659 ) ) ;
#10203=CARTESIAN_POINT ( 'NONE',  ( 12.85536293311005451, -7.423602990911125410, -229.4216632760384300 ) ) ;
#10206=CARTESIAN_POINT ( 'NONE',  ( -1.881996891245037995, 28.05344686410985489, -218.6379207300106202 ) ) ;
#10207=CARTESIAN_POINT ( 'NONE',  ( -9.208465596459861402, -9.574166310164313742, -220.4340298767933177 ) ) ;
#10209=CARTESIAN_POINT ( 'NONE',  ( 15.89706143421296147, 10.57416387607782227, -218.3862415393350318 ) ) ;
#10210=CARTESIAN_POINT ( 'NONE',  ( -14.87984907657228639, 0.2138881189739126887, -228.7773920408832282 ) ) ;
#10212=CARTESIAN_POINT ( 'NONE',  ( 11.43609017326686050, -13.06727081285745307, -217.8903327850316316 ) ) ;
#10213=CARTESIAN_POINT ( 'NONE',  ( -14.00380962569832199, 8.747390586476997854, -231.7950903513155936 ) ) ;
#10214=CARTESIAN_POINT ( 'NONE',  ( 16.49791052269847569, 3.745513941566326999, -220.1874559167976884 ) ) ;
#10215=CARTESIAN_POINT ( 'NONE',  ( -2.609511328024065602, -16.97143768612226822, -230.2205646068415490 ) ) ;
#10217=CARTESIAN_POINT ( 'NONE',  ( 22.18132842682159733, 5.591149267797686839, -232.0584733989884114 ) ) ;
#10218=CARTESIAN_POINT ( 'NONE',  ( -15.23434562258889891, -0.4010941804143903222, -220.4743703065900036 ) ) ;
#10219=CARTESIAN_POINT ( 'NONE',  ( 11.49416291172809856, -12.02598964588280595, -221.0946228713814889 ) ) ;
#10220=CARTESIAN_POINT ( 'NONE',  ( 13.16198298396986743, -2.194854683017246622, -227.0464278254075623 ) ) ;
#10223=CARTESIAN_POINT ( 'NONE',  ( 10.12648780932046755, 24.76571117977573522, -228.8499436907259792 ) ) ;
#10224=CARTESIAN_POINT ( 'NONE',  ( 5.563568780623874943, 21.86458082533069103, -218.6474243140849012 ) ) ;
#10225=CARTESIAN_POINT ( 'NONE',  ( 8.556785575048143855, -8.471343838569373119, -226.7940772732511050 ) ) ;
#10226=CARTESIAN_POINT ( 'NONE',  ( 20.38902395782249144, -18.95772103455488633, -230.9098670703349967 ) ) ;
#10227=ORIENTED_EDGE ( 'NONE', *, *, #1264, .T. ) ;
#10228=CARTESIAN_POINT ( 'NONE',  ( -10.91003322996498071, 12.84665145358222382, -229.9786893781767958 ) ) ;
#10229=CARTESIAN_POINT ( 'NONE',  ( -21.26441444091935296, 10.69428164102106926, -219.3434466924981336 ) ) ;
#10230=CARTESIAN_POINT ( 'NONE',  ( 19.79854089336508594, 4.557290221971136646, -217.3342919181881143 ) ) ;
#10232=CARTESIAN_POINT ( 'NONE',  ( -13.20043892455957746, -23.63849784199488369, -228.2145582502841989 ) ) ;
#10233=CARTESIAN_POINT ( 'NONE',  ( 15.50884165284638705, 1.028647572718199843, -227.8181348745474679 ) ) ;
#10236=CARTESIAN_POINT ( 'NONE',  ( 13.89183999136464820, 6.553741795688899252, -220.8646181278399752 ) ) ;
#10237=CARTESIAN_POINT ( 'NONE',  ( 13.77063830053042892, -24.19668776886549821, -225.6207953771408086 ) ) ;
#10238=EDGE_CURVE ( 'NONE', #3103, #4932, #17133, .T. ) ;
#10239=CARTESIAN_POINT ( 'NONE',  ( 4.543450689403089271, 15.91052110650461771, -218.9437823786444426 ) ) ;
#10240=CARTESIAN_POINT ( 'NONE',  ( -15.66530208164916260, 23.23467148471576849, -218.1250122661128046 ) ) ;
#10241=CARTESIAN_POINT ( 'NONE',  ( 7.359401564398577733, 15.81697286067417707, -215.8326977948377987 ) ) ;
#10242=CARTESIAN_POINT ( 'NONE',  ( -18.70090456008720992, 23.36146401084868884, -220.3989740370807056 ) ) ;
#10243=CARTESIAN_POINT ( 'NONE',  ( -2.808235066048971440, 30.42019778760651150, -222.6481917607299295 ) ) ;
#10246=CARTESIAN_POINT ( 'NONE',  ( 4.201723131641114328, -20.76291977712905279, -215.9522215885928347 ) ) ;
#10250=CARTESIAN_POINT ( 'NONE',  ( -25.95884575339096401, -1.972114683626720044, -231.2145524501483749 ) ) ;
#10251=CARTESIAN_POINT ( 'NONE',  ( 18.60971343765040942, 2.368090295052050820, -218.6871071987073094 ) ) ;
#10252=CARTESIAN_POINT ( 'NONE',  ( -16.33212578464095799, -13.18764990320557118, -218.7248530738716283 ) ) ;
#10253=CARTESIAN_POINT ( 'NONE',  ( 1.366658787427950772, -15.59113167952139456, -228.2894046839634257 ) ) ;
#10254=CARTESIAN_POINT ( 'NONE',  ( -25.44919589272258520, 4.740781954932180575, -232.0725131810460766 ) ) ;
#10255=CARTESIAN_POINT ( 'NONE',  ( -2.435715273212520238, 23.41098772907853132, -217.6796576669356966 ) ) ;
#10256=CARTESIAN_POINT ( 'NONE',  ( -8.894613172508529786, 25.42460746921206294, -232.3150764041658363 ) ) ;
#10258=CARTESIAN_POINT ( 'NONE',  ( 23.66932040738428356, 1.377632087272899541, -234.6098499860491415 ) ) ;
#10260=CARTESIAN_POINT ( 'NONE',  ( 20.41153371889344825, 17.18812948447019551, -230.7531656956970778 ) ) ;
#10261=CARTESIAN_POINT ( 'NONE',  ( -26.47320305716024791, 9.675235842009668019, -228.3542180911597654 ) ) ;
#10262=CARTESIAN_POINT ( 'NONE',  ( -11.39536650977235510, 9.246300577217761330, -228.4898727004871546 ) ) ;
#10263=CARTESIAN_POINT ( 'NONE',  ( -14.34029329777712469, -14.57793623142476669, -217.2545494607695389 ) ) ;
#10269=CARTESIAN_POINT ( 'NONE',  ( -21.47149190714903710, 3.672831083387290363, -231.0833634068433469 ) ) ;
#10270=CARTESIAN_POINT ( 'NONE',  ( 12.48419387172699579, 6.663456953110941328, -219.2717027540951165 ) ) ;
#10271=CARTESIAN_POINT ( 'NONE',  ( 16.49791052269847569, 3.745513941566326999, -220.1874559167976884 ) ) ;
#10272=CARTESIAN_POINT ( 'NONE',  ( -15.77287877451090203, -21.23371664991514152, -233.2776952697515185 ) ) ;
#10274=CARTESIAN_POINT ( 'NONE',  ( -19.02606456345395358, -20.49905271945607055, -219.9673098173381902 ) ) ;
#10275=CARTESIAN_POINT ( 'NONE',  ( -10.14083745617744547, 19.87482866967577877, -216.0596634563153486 ) ) ;
#10276=CARTESIAN_POINT ( 'NONE',  ( 8.115778909262310492, -29.92983049028717346, -224.5060555478150377 ) ) ;
#10277=CARTESIAN_POINT ( 'NONE',  ( -11.33137429837660193, 27.25022425932026238, -230.1650924901870212 ) ) ;
#10278=CARTESIAN_POINT ( 'NONE',  ( 13.62633932172415641, -0.5436634383532278347, -227.0682007726617542 ) ) ;
#10279=CARTESIAN_POINT ( 'NONE',  ( -14.78079095050690661, -5.416970230978240153, -229.7193632018645246 ) ) ;
#10281=CARTESIAN_POINT ( 'NONE',  ( -15.30864812529618391, 1.596444765892653717, -220.3859421844601627 ) ) ;
#10283=CARTESIAN_POINT ( 'NONE',  ( -7.366083718505351818, 19.86648438590005838, -231.8662444779758971 ) ) ;
#10284=CARTESIAN_POINT ( 'NONE',  ( 15.89621445970763070, 6.639162626453350313, -232.5295318698041456 ) ) ;
#10285=CARTESIAN_POINT ( 'NONE',  ( 16.38151749656409351, 8.902090001712490874, -231.2955017965201989 ) ) ;
#10286=CARTESIAN_POINT ( 'NONE',  ( 13.60311248493089131, 7.003372205918751092, -219.1738832909067867 ) ) ;
#10287=CARTESIAN_POINT ( 'NONE',  ( -3.482364789216947809, -21.46714584935086023, -216.0234696677019883 ) ) ;
#10288=CARTESIAN_POINT ( 'NONE',  ( 9.169328349715531346, 20.85917603618721472, -214.7000934853629133 ) ) ;
#10290=CARTESIAN_POINT ( 'NONE',  ( 8.479858146824877707, -14.20649975585062563, -220.0175458633526091 ) ) ;
#10291=CARTESIAN_POINT ( 'NONE',  ( -20.97727766418175932, 9.381545086430262970, -232.5968905491617420 ) ) ;
#10293=CARTESIAN_POINT ( 'NONE',  ( -1.301562195391901877, 16.19210386685474390, -220.0867867038183192 ) ) ;
#10294=CARTESIAN_POINT ( 'NONE',  ( -28.30937415889876618, -7.921132361018833556, -222.9755670691803857 ) ) ;
#10295=CARTESIAN_POINT ( 'NONE',  ( -15.83894155097017631, 1.950284868793920712, -224.5615909987450038 ) ) ;
#10296=CARTESIAN_POINT ( 'NONE',  ( 16.71272566993619080, 8.989703107375911273, -217.4612081447889125 ) ) ;
#10298=CARTESIAN_POINT ( 'NONE',  ( 4.656903975822286768, 13.45000048768594780, -227.6722060245555497 ) ) ;
#10299=CARTESIAN_POINT ( 'NONE',  ( 21.81705645104102587, -16.14081802208856686, -221.4047148572338131 ) ) ;
#10300=CARTESIAN_POINT ( 'NONE',  ( 11.20610455198612598, -10.15455062626793037, -220.8168162286965526 ) ) ;
#10302=CARTESIAN_POINT ( 'NONE',  ( 12.18657022793382794, 26.76558097653315471, -221.8882195427397335 ) ) ;
#10303=CARTESIAN_POINT ( 'NONE',  ( -27.27535713358387781, -16.47971293676793181, -227.4585470903502653 ) ) ;
#10304=CARTESIAN_POINT ( 'NONE',  ( -14.84823930505322132, -23.35465403802561823, -218.3226235040776260 ) ) ;
#10305=CARTESIAN_POINT ( 'NONE',  ( 8.785770181087007913, -10.38731345016515917, -223.4272116603623317 ) ) ;
#10306=CARTESIAN_POINT ( 'NONE',  ( -13.71158422780231056, 12.21432067443984693, -232.9166272955793033 ) ) ;
#10307=CARTESIAN_POINT ( 'NONE',  ( 18.14488609917747652, 6.993670804558928644, -231.4804853770579882 ) ) ;
#10308=CARTESIAN_POINT ( 'NONE',  ( -12.31207293045244988, 6.732038552366256923, -221.0952066824360713 ) ) ;
#10309=CARTESIAN_POINT ( 'NONE',  ( -8.115738378024497379, 16.90402287339461296, -219.0833473190803034 ) ) ;
#10310=CARTESIAN_POINT ( 'NONE',  ( -20.79829908948044448, -4.820361304162784855, -232.2223801333801703 ) ) ;
#10312=CARTESIAN_POINT ( 'NONE',  ( -8.611121136347097860, 17.46802294375265419, -231.5575697815534113 ) ) ;
#10314=CARTESIAN_POINT ( 'NONE',  ( 27.69955354773053458, 12.81264626165819287, -221.7750850138309602 ) ) ;
#10315=CARTESIAN_POINT ( 'NONE',  ( 10.22554538262735413, 24.20440706210576209, -215.6176527921760737 ) ) ;
#10316=CARTESIAN_POINT ( 'NONE',  ( 16.80562970167152415, -4.609754314392994878, -232.4812892975905356 ) ) ;
#10319=CARTESIAN_POINT ( 'NONE',  ( -3.082945806077231676, 30.69897765966285874, -224.2387254578930822 ) ) ;
#10320=CARTESIAN_POINT ( 'NONE',  ( -14.65326448616001898, -2.737518208283025167, -217.6605647598149744 ) ) ;
#10322=CARTESIAN_POINT ( 'NONE',  ( 15.87442104186276381, 8.674488492264579520, -230.9702037640878416 ) ) ;
#10323=CARTESIAN_POINT ( 'NONE',  ( -28.99926036811508467, 3.909990568804979194, -228.9613767892386988 ) ) ;
#10324=CARTESIAN_POINT ( 'NONE',  ( 15.84759643368428428, -7.142586963752317608, -231.1761396821659673 ) ) ;
#10325=CARTESIAN_POINT ( 'NONE',  ( -26.74045434827795020, 12.41518252455047744, -220.4617428697642652 ) ) ;
#10327=CARTESIAN_POINT ( 'NONE',  ( -27.82842955277035202, 11.70195273568964112, -227.9294339757464911 ) ) ;
#10328=CARTESIAN_POINT ( 'NONE',  ( 1.167080303844580058, -21.82675117811238152, -232.1335090276773485 ) ) ;
#10332=CARTESIAN_POINT ( 'NONE',  ( 21.15565078817875388, -13.66792796406074295, -219.8984673185389624 ) ) ;
#10333=CARTESIAN_POINT ( 'NONE',  ( 13.05726252127442244, -2.202320777661724183, -222.9558992616623812 ) ) ;
#10335=CARTESIAN_POINT ( 'NONE',  ( 10.48640380280471618, 25.27581435651469022, -227.8976696013017715 ) ) ;
#10336=CARTESIAN_POINT ( 'NONE',  ( 3.100794261777709782, 20.70580715608724276, -231.8781843337728219 ) ) ;
#10337=CARTESIAN_POINT ( 'NONE',  ( 5.902215564816073012, -11.20991439657816358, -226.4118943921501170 ) ) ;
#10338=CARTESIAN_POINT ( 'NONE',  ( 11.90144651507291051, -8.898305237537579515, -228.5592478859710184 ) ) ;
#10340=CARTESIAN_POINT ( 'NONE',  ( -11.16203726658389606, 26.27101666727781648, -227.8592829514190612 ) ) ;
#10341=CARTESIAN_POINT ( 'NONE',  ( -20.41147829968989313, 3.432784889297933795, -230.9611049257633510 ) ) ;
#10342=CARTESIAN_POINT ( 'NONE',  ( -24.69837543585720141, 12.57569301576483589, -232.4521327773205428 ) ) ;
#10344=CARTESIAN_POINT ( 'NONE',  ( -12.44689724543316522, -19.26441470091720731, -219.1960634559673622 ) ) ;
#10347=CARTESIAN_POINT ( 'NONE',  ( 13.59483335902903178, 5.678732573479117640, -228.5032236586631313 ) ) ;
#10348=CARTESIAN_POINT ( 'NONE',  ( 12.66847874168482591, -12.52481328540277161, -229.3043100997535646 ) ) ;
#10349=CARTESIAN_POINT ( 'NONE',  ( 15.91295838535984331, 21.88410254487826379, -230.9583961155862823 ) ) ;
#10350=CARTESIAN_POINT ( 'NONE',  ( -7.429838964355703901, 14.87322129099639234, -232.2632863647814077 ) ) ;
#10352=CARTESIAN_POINT ( 'NONE',  ( 13.85207896949186335, 7.847214149978243292, -217.3457543576531066 ) ) ;
#10353=CARTESIAN_POINT ( 'NONE',  ( 0.6364901924797052857, 13.89978473517355617, -221.8840706290426397 ) ) ;
#10354=DIRECTION ( 'NONE',  ( 0.000000000000000000, 0.000000000000000000, -1.000000000000000000 ) ) ;
#10355=CARTESIAN_POINT ( 'NONE',  ( 3.342529885312644833, -17.78621320651278737, -216.7788622297345853 ) ) ;
#10356=CARTESIAN_POINT ( 'NONE',  ( 25.46470895113276711, -14.41152162994631070, -228.1811935238409035 ) ) ;
#10359=CARTESIAN_POINT ( 'NONE',  ( -25.32262741784088078, 2.623212696197013472, -234.6011982779809841 ) ) ;
#10360=CARTESIAN_POINT ( 'NONE',  ( -12.55242351043508542, -12.71283815946331686, -230.7436264644880737 ) ) ;
#10361=CARTESIAN_POINT ( 'NONE',  ( 11.12240951639491549, -23.90857633046665853, -218.9373339142375130 ) ) ;
#10362=CARTESIAN_POINT ( 'NONE',  ( -24.79507334250576278, 6.844873424762779379, -218.1074956078844878 ) ) ;
#10363=CARTESIAN_POINT ( 'NONE',  ( 7.772443558932104146, 25.24620711463332157, -231.7813173736589931 ) ) ;
#10364=CARTESIAN_POINT ( 'NONE',  ( -5.607934827417612844, 15.68271927908880770, -232.1026723719274969 ) ) ;
#10366=CARTESIAN_POINT ( 'NONE',  ( 12.49911899277810434, -1.774523103166953497, -229.0731493570444002 ) ) ;
#10368=CARTESIAN_POINT ( 'NONE',  ( 22.86997486125673618, 17.56009411325475966, -222.3578648042903296 ) ) ;
#10369=CARTESIAN_POINT ( 'NONE',  ( -11.39536650977235510, 9.246300577217761330, -228.4898727004871546 ) ) ;
#10370=CARTESIAN_POINT ( 'NONE',  ( -25.94982248293519689, 10.67899231259548287, -221.1273147719203962 ) ) ;
#10371=CARTESIAN_POINT ( 'NONE',  ( -8.011291865669539547, -12.94570094964118923, -221.6322823144945744 ) ) ;
#10374=CARTESIAN_POINT ( 'NONE',  ( 20.05202556141620107, 8.012988804822112954, -215.8722494878839200 ) ) ;
#10375=CARTESIAN_POINT ( 'NONE',  ( -18.09605518090995702, 22.22778748761825085, -222.5443354630425290 ) ) ;
#10376=CARTESIAN_POINT ( 'NONE',  ( 14.82579616070250417, 22.96152595385638762, -233.8920860146931489 ) ) ;
#10377=CARTESIAN_POINT ( 'NONE',  ( 24.78222556642275620, 17.97262539535998371, -226.6641400693514470 ) ) ;
#10378=CARTESIAN_POINT ( 'NONE',  ( -27.51824122704870135, -10.15715933399136617, -232.3556155038515669 ) ) ;
#10380=CARTESIAN_POINT ( 'NONE',  ( -6.776147227169700749, -16.68571135823561846, -231.0772860317820232 ) ) ;
#10383=CARTESIAN_POINT ( 'NONE',  ( -13.17897211815351000, 23.48099580033777301, -217.3415693533541173 ) ) ;
#10384=CARTESIAN_POINT ( 'NONE',  ( 8.709470447750865318, -17.43408031369701661, -216.5121658579468829 ) ) ;
#10385=CARTESIAN_POINT ( 'NONE',  ( 1.382955251742491898, 16.46353944795171032, -231.7743150979565030 ) ) ;
#10386=CARTESIAN_POINT ( 'NONE',  ( 18.17041142304332624, -16.27896884253082987, -234.9734867155044356 ) ) ;
#10387=CARTESIAN_POINT ( 'NONE',  ( -14.76273180397945772, -6.370707202906876532, -220.0066229284273334 ) ) ;
#10389=CARTESIAN_POINT ( 'NONE',  ( -21.43408368508570305, 3.680162304907783621, -233.1134812316964542 ) ) ;
#10391=CARTESIAN_POINT ( 'NONE',  ( -2.015708574708954259, 26.78900769828807782, -221.5371848586876808 ) ) ;
#10392=CARTESIAN_POINT ( 'NONE',  ( -25.44919589272258520, 4.740781954932180575, -232.0725131810460766 ) ) ;
#10393=CARTESIAN_POINT ( 'NONE',  ( 13.43170911749896490, 19.07691563292472026, -232.7497845103644636 ) ) ;
#10394=CARTESIAN_POINT ( 'NONE',  ( 22.22999428328319382, 14.15012104770485557, -232.1858878619060249 ) ) ;
#10395=CARTESIAN_POINT ( 'NONE',  ( 5.521532699605532279, -19.36944961733043513, -235.0341191922501594 ) ) ;
#10396=CARTESIAN_POINT ( 'NONE',  ( 2.631948090663005946, 31.21493676147814611, -222.3107766067421380 ) ) ;
#10398=CARTESIAN_POINT ( 'NONE',  ( 1.345830553852720657, -29.56269728401072783, -219.9360760428637604 ) ) ;
#10399=CARTESIAN_POINT ( 'NONE',  ( -17.08384421609436643, 23.56421365837046622, -225.2902702884460666 ) ) ;
#10400=CARTESIAN_POINT ( 'NONE',  ( -1.975202609796049336, 20.81351768191813889, -217.5779402428482001 ) ) ;
#10401=CARTESIAN_POINT ( 'NONE',  ( -21.80830016239255897, -4.781675611938959847, -217.4666014280278148 ) ) ;
#10402=CARTESIAN_POINT ( 'NONE',  ( -24.40185606299549192, 11.66496215664722236, -221.9473669705449765 ) ) ;
#10403=CARTESIAN_POINT ( 'NONE',  ( -10.95054816480499760, 8.339404316518379545, -224.1596700080921778 ) ) ;
#10404=CARTESIAN_POINT ( 'NONE',  ( 19.66122710937851537, 22.83208755991274330, -220.0578523118790883 ) ) ;
#10405=CARTESIAN_POINT ( 'NONE',  ( 10.50530447320976535, 20.19629329636330084, -217.1354359361034767 ) ) ;
#10406=CARTESIAN_POINT ( 'NONE',  ( 14.36131679319511001, -8.144601358551431858, -221.7207256223857144 ) ) ;
#10408=CARTESIAN_POINT ( 'NONE',  ( 24.96165930385824794, -17.14663603160204275, -224.2745859498249672 ) ) ;
#10409=CARTESIAN_POINT ( 'NONE',  ( -2.693916085894628942, 18.86613858709357672, -230.4911878356387263 ) ) ;
#10411=CARTESIAN_POINT ( 'NONE',  ( 14.32085100525799248, 9.220655089380342062, -219.9006227404039464 ) ) ;
#10412=CARTESIAN_POINT ( 'NONE',  ( -18.70843642779997040, -17.48186590846855992, -215.2841814587906981 ) ) ;
#10413=CARTESIAN_POINT ( 'NONE',  ( -1.633632075387274840, -15.48245080501611071, -218.5193615163172751 ) ) ;
#10414=CARTESIAN_POINT ( 'NONE',  ( 15.11994912051959972, -12.48385213956034079, -232.8079920308188377 ) ) ;
#10415=CARTESIAN_POINT ( 'NONE',  ( -3.504118661534079582, 16.69899759879061918, -221.4378787282527128 ) ) ;
#10417=CARTESIAN_POINT ( 'NONE',  ( 14.72648027392381387, 10.15511732729369676, -229.5776536674053716 ) ) ;
#10418=CARTESIAN_POINT ( 'NONE',  ( -14.00380962569832199, 8.747390586476997854, -231.7950903513155936 ) ) ;
#10419=CARTESIAN_POINT ( 'NONE',  ( -15.63515374589483109, 24.59141623553136569, -226.9057426066772507 ) ) ;
#10420=CARTESIAN_POINT ( 'NONE',  ( 30.81364357021286793, -2.580535071768633060, -224.0234450364292513 ) ) ;
#10421=CARTESIAN_POINT ( 'NONE',  ( 1.939863782649466017, 28.20584428268631783, -229.4487744520996273 ) ) ;
#10422=CARTESIAN_POINT ( 'NONE',  ( -20.41147829968989313, 3.432784889297933795, -230.9611049257633510 ) ) ;
#10423=CARTESIAN_POINT ( 'NONE',  ( 11.13671218404335761, 30.21738803452449673, -224.2405745632392211 ) ) ;
#10424=CARTESIAN_POINT ( 'NONE',  ( 4.823266655078461085, -13.86048651889774241, -224.7145696108100026 ) ) ;
#10427=CARTESIAN_POINT ( 'NONE',  ( -6.474151797443945533, 21.29193859232740138, -215.9573456447696458 ) ) ;
#10428=CARTESIAN_POINT ( 'NONE',  ( -10.76816654174163368, -5.786055782404167402, -221.6662823521482437 ) ) ;
#10431=CARTESIAN_POINT ( 'NONE',  ( 26.29894631880581812, 12.29609390142961090, -226.3100047295820332 ) ) ;
#10432=CARTESIAN_POINT ( 'NONE',  ( -29.88125065636863198, 4.504452993877526623, -226.2048141718237275 ) ) ;
#10433=CARTESIAN_POINT ( 'NONE',  ( 18.00123703865980218, -15.82960056198189491, -233.0014896689109776 ) ) ;
#10435=CARTESIAN_POINT ( 'NONE',  ( -11.02345917017863464, 29.02019856777526741, -223.9475008740665771 ) ) ;
#10436=CARTESIAN_POINT ( 'NONE',  ( -28.13472254077564116, 12.33996625515159629, -224.9141344439281909 ) ) ;
#10437=CARTESIAN_POINT ( 'NONE',  ( -1.615718423935818437, -15.01490656935555812, -223.2481059054151729 ) ) ;
#10439=CARTESIAN_POINT ( 'NONE',  ( 16.91879448796214191, 0.8271603773820436212, -230.0510230802265710 ) ) ;
#10440=CARTESIAN_POINT ( 'NONE',  ( -16.63766460830045091, 5.158675778507696208, -232.1659425527909093 ) ) ;
#10441=CARTESIAN_POINT ( 'NONE',  ( 17.09791731880535437, -14.50769433911838568, -231.1780219065761059 ) ) ;
#10442=CARTESIAN_POINT ( 'NONE',  ( 13.78122601621266519, -1.862995838536092519, -227.3514709470891546 ) ) ;
#10444=CARTESIAN_POINT ( 'NONE',  ( 15.70179827786738969, 6.572001003133339125, -229.5476218741844434 ) ) ;
#10445=CARTESIAN_POINT ( 'NONE',  ( -12.19796877179171446, 17.24929682309303658, -234.5722138766719809 ) ) ;
#10446=CARTESIAN_POINT ( 'NONE',  ( 14.37653162493774239, 9.985418694807894013, -229.1686718965858063 ) ) ;
#10447=CARTESIAN_POINT ( 'NONE',  ( 3.722478027540565559, -17.18860102498078390, -232.3439289206262686 ) ) ;
#10448=CARTESIAN_POINT ( 'NONE',  ( 14.15946391865398013, -0.7413617426029489588, -228.5799580636366670 ) ) ;
#10450=CARTESIAN_POINT ( 'NONE',  ( 1.939863782649466017, 28.20584428268631783, -229.4487744520996273 ) ) ;
#10451=CARTESIAN_POINT ( 'NONE',  ( -15.32935061426341861, 5.146212415319166844, -225.5669090095357774 ) ) ;
#10452=CARTESIAN_POINT ( 'NONE',  ( -22.28357709049062407, 7.264818440526320309, -215.3877468064711707 ) ) ;
#10453=CARTESIAN_POINT ( 'NONE',  ( -3.373690338999510985, -20.30281967708846125, -218.2431319494177160 ) ) ;
#10456=CARTESIAN_POINT ( 'NONE',  ( 16.71272566993619080, 8.989703107375911273, -217.4612081447889125 ) ) ;
#10457=CARTESIAN_POINT ( 'NONE',  ( 17.63166870185818169, -20.21345786093278107, -221.6360081359454739 ) ) ;
#10458=CARTESIAN_POINT ( 'NONE',  ( 4.484811161826725900, 15.38298568785217313, -219.4617573400562662 ) ) ;
#10459=CARTESIAN_POINT ( 'NONE',  ( -20.18153419852512442, 14.25141268122526483, -233.5059133483111964 ) ) ;
#10460=CARTESIAN_POINT ( 'NONE',  ( 19.48863273024974418, 12.80680990455712909, -215.0408095016468053 ) ) ;
#10461=CARTESIAN_POINT ( 'NONE',  ( 8.812073984913094904, 13.12649198322903210, -229.9172071780580495 ) ) ;
#10463=CARTESIAN_POINT ( 'NONE',  ( -1.632242579688942596, -13.62074943359385415, -221.1585305289511041 ) ) ;
#10464=CARTESIAN_POINT ( 'NONE',  ( 21.53087031351596892, -21.03550532031109555, -227.1077645633325233 ) ) ;
#10467=CARTESIAN_POINT ( 'NONE',  ( -18.07648963816576781, 14.36622924931724654, -235.1425738388569187 ) ) ;
#10468=CARTESIAN_POINT ( 'NONE',  ( -27.92538795710911259, -2.661554249663629079, -224.6264721727631581 ) ) ;
#10469=CARTESIAN_POINT ( 'NONE',  ( -29.22672729369577738, 6.588740615114764054, -224.9915299386302934 ) ) ;
#10470=CARTESIAN_POINT ( 'NONE',  ( -1.038524475621362075, 14.89017051181998141, -222.3948816610352139 ) ) ;
#10471=CARTESIAN_POINT ( 'NONE',  ( 3.755480357635514022, 24.23367984900377436, -231.4105847235276201 ) ) ;
#10473=CARTESIAN_POINT ( 'NONE',  ( 30.80938026993025503, 0.02210899415489638725, -229.5596456628577187 ) ) ;
#10474=CARTESIAN_POINT ( 'NONE',  ( 7.168644370073567806, 19.32044210858112265, -233.1278450877711634 ) ) ;
#10475=CARTESIAN_POINT ( 'NONE',  ( -21.66801938871533650, 16.28801167444048659, -218.5240035253498547 ) ) ;
#10476=CARTESIAN_POINT ( 'NONE',  ( -26.47320305716024791, 9.675235842009668019, -228.3542180911597654 ) ) ;
#10477=CARTESIAN_POINT ( 'NONE',  ( -18.38002254392888446, -21.81807606669838506, -229.0374583293157968 ) ) ;
#10481=CARTESIAN_POINT ( 'NONE',  ( 28.03290210476798094, 13.48017620089690638, -224.9212082181537937 ) ) ;
#10482=CARTESIAN_POINT ( 'NONE',  ( -13.23768812067001477, 12.78288831771969569, -230.4179793829127902 ) ) ;
#10483=CARTESIAN_POINT ( 'NONE',  ( 13.32754126089433377, 12.31312334927721963, -234.6033665822900218 ) ) ;
#10484=CARTESIAN_POINT ( 'NONE',  ( -16.71711190488355570, 0.6105529133557690002, -230.9511258789794681 ) ) ;
#10485=CARTESIAN_POINT ( 'NONE',  ( -10.57293828068126373, -5.503282544971903611, -227.1466070594375708 ) ) ;
#10488=CARTESIAN_POINT ( 'NONE',  ( -12.96708845633950347, -3.368725568741437026, -223.5528514750533873 ) ) ;
#10489=CARTESIAN_POINT ( 'NONE',  ( -5.383332542724544645, 15.12651309054520432, -231.5699995578976313 ) ) ;
#10490=CARTESIAN_POINT ( 'NONE',  ( -11.28700884291539630, -21.85791790461604478, -233.5354093188319951 ) ) ;
#10491=CARTESIAN_POINT ( 'NONE',  ( -6.201839134465864767, 11.37481922992157379, -223.7040893475979146 ) ) ;
#10492=CARTESIAN_POINT ( 'NONE',  ( 14.85580775603058079, -28.43502054068834894, -222.5810199743787905 ) ) ;
#10495=CARTESIAN_POINT ( 'NONE',  ( -18.88895772509644644, 1.306698388790553444, -217.6272550812279292 ) ) ;
#10496=CARTESIAN_POINT ( 'NONE',  ( -5.706122936196527107, 15.14201253431006045, -228.6865785740211550 ) ) ;
#10497=CARTESIAN_POINT ( 'NONE',  ( 12.89118769162836031, 6.140251663080722899, -228.8792332048833771 ) ) ;
#10499=CARTESIAN_POINT ( 'NONE',  ( 20.89184612657454920, 5.404957034965973683, -232.0952743654565609 ) ) ;
#10500=CARTESIAN_POINT ( 'NONE',  ( 13.06430160593375689, 2.561628050526134182, -220.6026188403641299 ) ) ;
#10501=CARTESIAN_POINT ( 'NONE',  ( -4.538939863750555581, -15.27574540357637112, -231.4384328720293524 ) ) ;
#10502=CARTESIAN_POINT ( 'NONE',  ( 2.000982021813747291, 12.72833461843010205, -228.3416607300594308 ) ) ;
#10504=CARTESIAN_POINT ( 'NONE',  ( -4.110806133445755961, -12.94090688063470473, -230.1197724001632992 ) ) ;
#10505=CARTESIAN_POINT ( 'NONE',  ( -7.284474494690100776, 13.60812129561547046, -227.7414351104868331 ) ) ;
#10507=CARTESIAN_POINT ( 'NONE',  ( 21.26803326031697949, 19.54255073453192892, -230.5813148908474659 ) ) ;
#10509=CARTESIAN_POINT ( 'NONE',  ( -16.20471097821853235, -2.781505378741172319, -220.1484675126197317 ) ) ;
#10510=CARTESIAN_POINT ( 'NONE',  ( -17.00819119081011266, 8.904695857470725784, -219.7915043529501133 ) ) ;
#10511=CARTESIAN_POINT ( 'NONE',  ( -11.40916210110096962, 20.01996232974788725, -234.3205435716851923 ) ) ;
#10512=CARTESIAN_POINT ( 'NONE',  ( 16.40130693394614525, -0.1574073183566240264, -221.9481963320051534 ) ) ;
#10514=CARTESIAN_POINT ( 'NONE',  ( 8.587407344280324040, -17.24386586482343375, -219.6634241328915209 ) ) ;
#10516=CARTESIAN_POINT ( 'NONE',  ( 5.037691872308702301, -15.96383311541683270, -230.0422288358542460 ) ) ;
#10517=CARTESIAN_POINT ( 'NONE',  ( -3.015877970456246615, 27.27456613555083464, -227.6995284396757313 ) ) ;
#10518=CARTESIAN_POINT ( 'NONE',  ( 7.995304978256253747, 13.28024228361502779, -220.6535174700288451 ) ) ;
#10519=CARTESIAN_POINT ( 'NONE',  ( 15.13105790938820228, -1.902449014147146178, -222.1588331224812407 ) ) ;
#10520=CARTESIAN_POINT ( 'NONE',  ( -5.178973235464019886, -24.35492185057628944, -233.6431870320687381 ) ) ;
#10521=CARTESIAN_POINT ( 'NONE',  ( -0.8413160509385254615, -28.71376977722865931, -218.8117683208458288 ) ) ;
#10522=CARTESIAN_POINT ( 'NONE',  ( -8.752190949579933488, 24.25633523490762755, -230.6624101830059885 ) ) ;
#10524=CARTESIAN_POINT ( 'NONE',  ( 15.88536911906737181, 12.85343532334862893, -218.9532478288372204 ) ) ;
#10525=CARTESIAN_POINT ( 'NONE',  ( -28.13472254077564116, 12.33996625515159629, -224.9141344439281909 ) ) ;
#10526=CARTESIAN_POINT ( 'NONE',  ( -13.44241955326339166, 15.88952131657459965, -217.2587743382015901 ) ) ;
#10530=CARTESIAN_POINT ( 'NONE',  ( 3.192353461299334061, 22.13718518159985393, -217.1103300728619843 ) ) ;
#10531=CARTESIAN_POINT ( 'NONE',  ( -21.48978835671764287, 1.062155088816892468, -219.0000000007146355 ) ) ;
#10532=CARTESIAN_POINT ( 'NONE',  ( 8.546572992885776543, 19.06776382077057974, -214.7173484156796519 ) ) ;
#10533=CARTESIAN_POINT ( 'NONE',  ( 12.78854151797817451, -25.92021405714643123, -222.0152117995072842 ) ) ;
#10536=CARTESIAN_POINT ( 'NONE',  ( 0.2389779871941385414, 16.64595486589868045, -218.1658233406367629 ) ) ;
#10537=CARTESIAN_POINT ( 'NONE',  ( 17.75464445068659458, -4.950329359371821170, -229.7529072665692240 ) ) ;
#10538=CARTESIAN_POINT ( 'NONE',  ( 29.12543877365354916, -1.475122899492763873, -224.0746120762670444 ) ) ;
#10539=CARTESIAN_POINT ( 'NONE',  ( 17.34727976380017722, 4.822939981779328811, -230.8836217450937909 ) ) ;
#10540=CARTESIAN_POINT ( 'NONE',  ( -14.70651859537745487, 4.211702956367679107, -230.0357207626005334 ) ) ;
#10541=CARTESIAN_POINT ( 'NONE',  ( 5.609436632608550966, -13.11664087352601094, -229.3324225951633650 ) ) ;
#10543=CARTESIAN_POINT ( 'NONE',  ( -7.395406416482832590, 12.93623984139929739, -219.2606224730616873 ) ) ;
#10546=CARTESIAN_POINT ( 'NONE',  ( -17.84981083811007707, 0.8485253248287054628, -231.8041300026935119 ) ) ;
#10547=CARTESIAN_POINT ( 'NONE',  ( -8.326748185965973548, -13.59788789161040512, -220.4531618457016862 ) ) ;
#10551=CARTESIAN_POINT ( 'NONE',  ( -24.24202834850560606, 19.05981756344202438, -226.6980666352953335 ) ) ;
#10552=CARTESIAN_POINT ( 'NONE',  ( 23.68557655437113141, -13.81416892717991551, -227.4080549258873987 ) ) ;
#10554=CARTESIAN_POINT ( 'NONE',  ( 14.23294950300690331, 6.961167337017927892, -222.0879133937260974 ) ) ;
#10555=CARTESIAN_POINT ( 'NONE',  ( -16.89013823391154290, 26.38860451648245231, -225.6449744083545852 ) ) ;
#10557=CARTESIAN_POINT ( 'NONE',  ( 12.84032013659066251, 19.10303921738740485, -230.8110334357214128 ) ) ;
#10558=CARTESIAN_POINT ( 'NONE',  ( -7.536234698756538286, -25.83616497442384130, -229.4709156672317363 ) ) ;
#10559=CARTESIAN_POINT ( 'NONE',  ( 28.89510310306777541, -0.2847990887752292477, -220.1812426115722303 ) ) ;
#10561=CARTESIAN_POINT ( 'NONE',  ( 1.104227501629593045, 25.05528885094460989, -231.9808705443460326 ) ) ;
#10562=CARTESIAN_POINT ( 'NONE',  ( -22.36207348798144778, 17.12313795477538036, -223.8571857210765472 ) ) ;
#10563=CARTESIAN_POINT ( 'NONE',  ( -26.41026844077819291, 5.012316129610852933, -233.8406020309487872 ) ) ;
#10564=CARTESIAN_POINT ( 'NONE',  ( -23.21124258271143503, -15.80671483884278317, -224.0808897361354468 ) ) ;
#10568=CARTESIAN_POINT ( 'NONE',  ( 18.55287065739596031, 7.869864349944380777, -232.8430408253643691 ) ) ;
#10569=CARTESIAN_POINT ( 'NONE',  ( 3.499756879752360827, -15.16424639601953039, -225.9472731234413061 ) ) ;
#10570=CARTESIAN_POINT ( 'NONE',  ( 20.41153371889344825, 17.18812948447019551, -230.7531656956970778 ) ) ;
#10572=CARTESIAN_POINT ( 'NONE',  ( -14.00380962569832199, 8.747390586476997854, -231.7950903513155936 ) ) ;
#10573=CARTESIAN_POINT ( 'NONE',  ( 29.64577750251057608, 2.839131411071813549, -220.9704389295326905 ) ) ;
#10574=CARTESIAN_POINT ( 'NONE',  ( 7.743212835174657194, 11.90778931056080481, -226.0491028376908105 ) ) ;
#10576=CARTESIAN_POINT ( 'NONE',  ( 1.541778504653760429, -23.48174737203985529, -233.9922866444541967 ) ) ;
#10577=CARTESIAN_POINT ( 'NONE',  ( 15.05686526350529775, -5.555778903407086133, -220.1433349335996468 ) ) ;
#10581=CARTESIAN_POINT ( 'NONE',  ( -7.694246740028670928, 10.31295298368923063, -221.9989544301487001 ) ) ;
#10582=CARTESIAN_POINT ( 'NONE',  ( -26.34963598119476913, -8.267085687785165504, -223.3493716711078889 ) ) ;
#10583=CARTESIAN_POINT ( 'NONE',  ( -18.04772061096520375, 5.916925414182395038, -217.8829197293425750 ) ) ;
#10584=CARTESIAN_POINT ( 'NONE',  ( 2.951582164238582440, 19.39026647431845873, -217.4356918981242472 ) ) ;
#10585=CARTESIAN_POINT ( 'NONE',  ( -2.665457046508036942, 16.94988614842223029, -218.7621057649994896 ) ) ;
#10587=CARTESIAN_POINT ( 'NONE',  ( 8.556785575048143855, -8.471343838569373119, -226.7940772732511050 ) ) ;
#10589=CARTESIAN_POINT ( 'NONE',  ( 25.18785298611088308, 3.974282393449815931, -218.7636041058819956 ) ) ;
#10590=CARTESIAN_POINT ( 'NONE',  ( -9.251743101293765648, 14.06372330290396278, -232.4239003576353468 ) ) ;
#10591=EDGE_CURVE ( 'NONE', #13407, #6170, #352, .T. ) ;
#10592=CARTESIAN_POINT ( 'NONE',  ( -25.19195624009214640, 10.50676406307063182, -220.0954552869889937 ) ) ;
#10593=CARTESIAN_POINT ( 'NONE',  ( -11.96638064467250473, -24.81952708901905069, -229.8544473269683692 ) ) ;
#10594=CARTESIAN_POINT ( 'NONE',  ( -13.58874046263339608, 12.73011668665171392, -216.5659449791897941 ) ) ;
#10596=CARTESIAN_POINT ( 'NONE',  ( 20.10109416526603709, 2.018147939476731434, -216.1034161917718848 ) ) ;
#10598=CARTESIAN_POINT ( 'NONE',  ( -18.36252859017411510, 21.06344830687906367, -228.5073589488702623 ) ) ;
#10600=CARTESIAN_POINT ( 'NONE',  ( 16.84354851290083133, 10.42424693870724361, -215.2582953371023109 ) ) ;
#10601=CARTESIAN_POINT ( 'NONE',  ( -18.08305592660031991, 4.022743421239192152, -217.2335041149100050 ) ) ;
#10602=CARTESIAN_POINT ( 'NONE',  ( -27.90711606799872513, 0.4679914357742857023, -216.8754026763949128 ) ) ;
#10603=CARTESIAN_POINT ( 'NONE',  ( -26.76734473129764069, -3.453818734898710829, -232.3222361544058003 ) ) ;
#10604=CARTESIAN_POINT ( 'NONE',  ( -4.450022810944913587, 12.45400981846350597, -225.2098051417536340 ) ) ;
#10605=CARTESIAN_POINT ( 'NONE',  ( -11.40116373163465369, -15.95513543764466213, -216.7841692646331353 ) ) ;
#10606=CARTESIAN_POINT ( 'NONE',  ( 4.907833106823921376, 13.98151846258800290, -229.0190609869640923 ) ) ;
#10607=CARTESIAN_POINT ( 'NONE',  ( 19.49551695935633688, -21.73806820219217428, -217.5227155576580742 ) ) ;
#10609=CARTESIAN_POINT ( 'NONE',  ( 20.47387447818710271, 7.390772095927000684, -234.0991886097562258 ) ) ;
#10611=CARTESIAN_POINT ( 'NONE',  ( -3.010752168931037698, 15.84372070116375575, -223.4060793985500482 ) ) ;
#10612=CARTESIAN_POINT ( 'NONE',  ( 28.53243699394185384, 6.329221954355706004, -218.6437889135959267 ) ) ;
#10613=CARTESIAN_POINT ( 'NONE',  ( 14.19800769603076240, 4.587407146151301518, -224.2928935459285071 ) ) ;
#10614=CARTESIAN_POINT ( 'NONE',  ( 18.30177952310522471, 1.918278963380847468, -233.8574151782075887 ) ) ;
#10615=CARTESIAN_POINT ( 'NONE',  ( -7.242471263717580321, -12.67345288765796774, -222.7008556220510229 ) ) ;
#10618=CARTESIAN_POINT ( 'NONE',  ( 15.89102655998366664, 24.10108298038447572, -232.7733025413564008 ) ) ;
#10620=CARTESIAN_POINT ( 'NONE',  ( -6.773088999562194346, -28.54379939428971369, -218.3283227997898450 ) ) ;
#10621=CARTESIAN_POINT ( 'NONE',  ( -16.57767831947938575, 23.50485984366324388, -222.7977068309636763 ) ) ;
#10622=CARTESIAN_POINT ( 'NONE',  ( 12.96449997971774870, 8.285709878278680662, -230.9518598506670628 ) ) ;
#10624=CARTESIAN_POINT ( 'NONE',  ( -28.42127686227592420, -0.6461176296494712812, -221.6028628238154567 ) ) ;
#10625=CARTESIAN_POINT ( 'NONE',  ( -21.01242583983345469, 16.60754347445175227, -220.8286358486543293 ) ) ;
#10626=CARTESIAN_POINT ( 'NONE',  ( 0.1645309800062008665, 15.56029994314186382, -233.1129172884685943 ) ) ;
#10627=CARTESIAN_POINT ( 'NONE',  ( 16.20788843645364352, 6.828976201867700269, -231.6689701909764665 ) ) ;
#10629=CARTESIAN_POINT ( 'NONE',  ( 13.43173494629961517, -24.23096015178613172, -223.5315588962966160 ) ) ;
#10632=CARTESIAN_POINT ( 'NONE',  ( 13.65368867897269389, -25.84127502057983605, -227.3223880387346867 ) ) ;
#10633=CARTESIAN_POINT ( 'NONE',  ( -9.060146982536336324, 27.14942986116457746, -225.6568961786626062 ) ) ;
#10636=CARTESIAN_POINT ( 'NONE',  ( 15.12287735332712835, 21.03907941686458116, -231.7894952627153202 ) ) ;
#10637=CARTESIAN_POINT ( 'NONE',  ( 17.95694455891925756, -3.510678534943489026, -231.2643001502910067 ) ) ;
#10638=CARTESIAN_POINT ( 'NONE',  ( -20.18470553695442860, -13.13924840112635195, -232.9662461559857718 ) ) ;
#10639=CARTESIAN_POINT ( 'NONE',  ( 0.04660897052267574947, -31.13860575300111577, -224.7746869833732717 ) ) ;
#10640=CARTESIAN_POINT ( 'NONE',  ( -1.796846813493219619, 26.08418332695505271, -220.7262848173578504 ) ) ;
#10642=CARTESIAN_POINT ( 'NONE',  ( 14.04819512851487673, 6.831178966487911453, -222.6676118107292552 ) ) ;
#10643=CARTESIAN_POINT ( 'NONE',  ( -8.501641725227710111, 25.47064987787527102, -217.3358698761548737 ) ) ;
#10644=CARTESIAN_POINT ( 'NONE',  ( -5.125319492185865577, 20.53749879880200524, -218.7557759432853288 ) ) ;
#10646=CARTESIAN_POINT ( 'NONE',  ( 8.175342817246784577, 19.41817470142738244, -216.6818271833384699 ) ) ;
#10647=CARTESIAN_POINT ( 'NONE',  ( -15.37153448429513602, 5.014568651886798456, -224.5085656291724945 ) ) ;
#10648=CARTESIAN_POINT ( 'NONE',  ( 28.41961022423218353, 10.76616830294286409, -220.2698681100053193 ) ) ;
#10649=CARTESIAN_POINT ( 'NONE',  ( 9.759123193367146953, -21.89695672029116480, -217.8292787338521919 ) ) ;
#10654=CARTESIAN_POINT ( 'NONE',  ( -6.282398543089500187, 12.01615879894893801, -228.5121145169883903 ) ) ;
#10655=CARTESIAN_POINT ( 'NONE',  ( 16.72004689093256857, -4.507886829375356008, -228.6412576449023959 ) ) ;
#10657=CARTESIAN_POINT ( 'NONE',  ( 24.03642272140365677, 3.646960756862087205, -218.2320643939070806 ) ) ;
#10658=CARTESIAN_POINT ( 'NONE',  ( 8.332496243628455090, -29.79192972398156769, -226.1452587264855367 ) ) ;
#10660=CARTESIAN_POINT ( 'NONE',  ( -9.151299407007059017, 9.196974979111923076, -223.9483834032048719 ) ) ;
#10661=CARTESIAN_POINT ( 'NONE',  ( -12.15711705271618470, 28.08001788883979799, -220.3431297925021681 ) ) ;
#10663=CARTESIAN_POINT ( 'NONE',  ( -27.90314475660494153, 12.48829126175061077, -223.3300566725355338 ) ) ;
#10664=CARTESIAN_POINT ( 'NONE',  ( -17.60306105620566441, -10.62493847279374926, -216.8163279515337649 ) ) ;
#10667=CARTESIAN_POINT ( 'NONE',  ( -23.52999999174766543, 19.39566142560855866, -221.9446938626390704 ) ) ;
#10668=CARTESIAN_POINT ( 'NONE',  ( 0.3555517721839966394, -12.99484957898737569, -222.7951259809431974 ) ) ;
#10670=CARTESIAN_POINT ( 'NONE',  ( 14.75355577798158713, -1.671605614104410886, -222.5078368351397842 ) ) ;
#10672=CARTESIAN_POINT ( 'NONE',  ( 15.88536911906737181, 12.85343532334862893, -218.9532478288372204 ) ) ;
#10674=CARTESIAN_POINT ( 'NONE',  ( -23.66836017558062011, 21.44695383684080525, -223.6245772351065568 ) ) ;
#10676=CARTESIAN_POINT ( 'NONE',  ( 15.99247752609008444, 10.72268246046808216, -230.5614800526110173 ) ) ;
#10677=CARTESIAN_POINT ( 'NONE',  ( -0.09985864093865706725, -15.05342968659714309, -222.4585048042796132 ) ) ;
#10680=CARTESIAN_POINT ( 'NONE',  ( -4.334015487506815312, 18.19775486192265390, -231.4387392399519285 ) ) ;
#10681=CARTESIAN_POINT ( 'NONE',  ( -16.48883219358909713, 20.84100960965193394, -219.4392138569792507 ) ) ;
#10682=CARTESIAN_POINT ( 'NONE',  ( -25.98311979368102342, 15.13734258059737670, -220.6162231662327429 ) ) ;
#10683=CARTESIAN_POINT ( 'NONE',  ( -22.54540532658949914, -16.00113133426942724, -227.3151344909721843 ) ) ;
#10686=CARTESIAN_POINT ( 'NONE',  ( 21.14441169763230732, 12.98245189690719315, -217.0976687089155064 ) ) ;
#10687=CARTESIAN_POINT ( 'NONE',  ( 5.446054363465077763, -20.62119468428589997, -218.5301445808800622 ) ) ;
#10688=CARTESIAN_POINT ( 'NONE',  ( 14.39473142419577023, 15.98257177912839389, -217.4557725731239373 ) ) ;
#10689=CARTESIAN_POINT ( 'NONE',  ( -18.09776816382430908, 23.50806826204562583, -229.9568677523880638 ) ) ;
#10690=CARTESIAN_POINT ( 'NONE',  ( 13.70863938672594529, 6.616599615120571265, -232.1343637516268643 ) ) ;
#10691=CARTESIAN_POINT ( 'NONE',  ( 2.539761864897490007, 23.64215977235053501, -233.4645566207487661 ) ) ;
#10693=CARTESIAN_POINT ( 'NONE',  ( -8.514447835183077018, -10.26590951297754195, -225.5321622820681569 ) ) ;
#10694=CARTESIAN_POINT ( 'NONE',  ( 12.13827923251525220, -9.172799829723585319, -229.1860353116090891 ) ) ;
#10696=FACE_OUTER_BOUND ( 'NONE', #6578, .T. ) ;
#10697=CARTESIAN_POINT ( 'NONE',  ( -17.81561310496929806, 18.25637658208611569, -215.7745954696244439 ) ) ;
#10698=CARTESIAN_POINT ( 'NONE',  ( -17.01759357405825668, -4.262369086395770168, -221.2289172648622184 ) ) ;
#10699=CARTESIAN_POINT ( 'NONE',  ( -16.74094048923576494, 16.03040267675914521, -217.9177456399057178 ) ) ;
#10700=CARTESIAN_POINT ( 'NONE',  ( 4.303123380281038024, 17.66787810618728827, -231.9745698734655832 ) ) ;
#10701=CARTESIAN_POINT ( 'NONE',  ( 4.482815116226093188, 26.97722808566452812, -229.2080185206130238 ) ) ;
#10703=CARTESIAN_POINT ( 'NONE',  ( 10.74287257054252720, -16.14773823008032849, -215.8883494958819824 ) ) ;
#10705=CARTESIAN_POINT ( 'NONE',  ( 14.68783945462866924, 9.535285537539673228, -219.4694094309942045 ) ) ;
#10706=CARTESIAN_POINT ( 'NONE',  ( -10.83439284573031536, 18.36737820296253432, -234.3014274143859836 ) ) ;
#10707=CARTESIAN_POINT ( 'NONE',  ( -17.00265675087485917, 7.324244386240115645, -218.5600005870616656 ) ) ;
#10708=CARTESIAN_POINT ( 'NONE',  ( -22.25980993584449408, -3.522148912989541802, -233.7954546715351398 ) ) ;
#10709=CARTESIAN_POINT ( 'NONE',  ( -17.75316132689678383, 25.03468689048078843, -222.1645193425721061 ) ) ;
#10712=CARTESIAN_POINT ( 'NONE',  ( 27.79746884017060538, 13.63637251724950339, -226.5788410723774575 ) ) ;
#10713=CARTESIAN_POINT ( 'NONE',  ( -22.53796032816233463, 16.84148256071415872, -226.0516062466300582 ) ) ;
#10714=CARTESIAN_POINT ( 'NONE',  ( 10.00603923119254723, 9.610873433734882454, -231.2388095806506669 ) ) ;
#10715=CARTESIAN_POINT ( 'NONE',  ( 28.09488075336259527, 3.911739131332936381, -227.7543364642411632 ) ) ;
#10716=CARTESIAN_POINT ( 'NONE',  ( -30.74480097515601074, -10.13586512673612106, -225.7096819839593707 ) ) ;
#10717=CARTESIAN_POINT ( 'NONE',  ( -21.50522087930578152, -16.03150550247721640, -231.4768288373508369 ) ) ;
#10718=CARTESIAN_POINT ( 'NONE',  ( -23.70973587455150522, 20.45398817402440983, -228.9005348699235469 ) ) ;
#10719=CARTESIAN_POINT ( 'NONE',  ( -15.62091161899253855, -26.00636881980398840, -222.1463585103649905 ) ) ;
#10720=CARTESIAN_POINT ( 'NONE',  ( 18.29617186523616468, 23.20920553663278341, -223.4372550713720216 ) ) ;
#10721=CARTESIAN_POINT ( 'NONE',  ( 15.13450096816097634, -26.20215934980152639, -231.3023426574493726 ) ) ;
#10723=CARTESIAN_POINT ( 'NONE',  ( 22.16327814861754675, 7.634676377199016706, -234.0520676664821735 ) ) ;
#10725=CARTESIAN_POINT ( 'NONE',  ( -2.554014161526931392, 17.56271496069470572, -229.4905841158208659 ) ) ;
#10726=CARTESIAN_POINT ( 'NONE',  ( -18.04772061096520375, 5.916925414182395038, -217.8829197293425750 ) ) ;
#10727=CARTESIAN_POINT ( 'NONE',  ( 15.05360126642391450, 1.481754003466396963, -222.9454997252120734 ) ) ;
#10728=CARTESIAN_POINT ( 'NONE',  ( 16.43556216695724004, 8.397919695511960825, -216.7971521583719152 ) ) ;
#10729=CARTESIAN_POINT ( 'NONE',  ( -10.96310611394154755, -12.59072721579616605, -220.6792497830813318 ) ) ;
#10730=CARTESIAN_POINT ( 'NONE',  ( 5.179557175392591972, 10.46258103618983881, -224.6216839350439614 ) ) ;
#10732=CARTESIAN_POINT ( 'NONE',  ( -9.037518995728490268, -13.81466884781966620, -216.3195389756191673 ) ) ;
#10733=CARTESIAN_POINT ( 'NONE',  ( -4.170472558179216804, 16.67407401355319152, -230.2690496885289804 ) ) ;
#10734=CARTESIAN_POINT ( 'NONE',  ( 13.20340559785743828, 9.575208899273587093, -218.1210831379648312 ) ) ;
#10735=CARTESIAN_POINT ( 'NONE',  ( -17.55809605150417951, 6.636094600389130349, -229.8856864643722986 ) ) ;
#10737=CARTESIAN_POINT ( 'NONE',  ( -12.15711705271618470, 28.08001788883979799, -220.3431297925021681 ) ) ;
#10738=CARTESIAN_POINT ( 'NONE',  ( 13.15438416660314225, 5.520603777723624539, -227.0878346348094681 ) ) ;
#10739=CARTESIAN_POINT ( 'NONE',  ( 8.290903921942224031, -23.90349455650518351, -230.1727405421096364 ) ) ;
#10741=CARTESIAN_POINT ( 'NONE',  ( 10.52067862919218832, -10.34113464825721351, -228.4460540958991714 ) ) ;
#10742=CARTESIAN_POINT ( 'NONE',  ( -8.881241380679488984, 27.18697625135247975, -224.4474391433207927 ) ) ;
#10744=CARTESIAN_POINT ( 'NONE',  ( 10.50530447320976535, 20.19629329636330084, -217.1354359361034767 ) ) ;
#10745=CARTESIAN_POINT ( 'NONE',  ( -25.32359575169976296, -0.6821277435459325300, -233.2512658769913969 ) ) ;
#10746=CARTESIAN_POINT ( 'NONE',  ( -11.88525712185471050, -8.925198460467992589, -221.0951487055306472 ) ) ;
#10747=CARTESIAN_POINT ( 'NONE',  ( -6.642805165258356404, -28.12267032419628521, -230.9452027245340560 ) ) ;
#10748=CARTESIAN_POINT ( 'NONE',  ( -5.560972518124746244, 14.60655266358653215, -227.5460946431043681 ) ) ;
#10750=CARTESIAN_POINT ( 'NONE',  ( 23.24653631066306048, 11.83805845626388020, -219.6020901153134162 ) ) ;
#10751=CARTESIAN_POINT ( 'NONE',  ( -6.201839134465864767, 11.37481922992157379, -223.7040893475979146 ) ) ;
#10752=CARTESIAN_POINT ( 'NONE',  ( -8.112279890008961658, 11.99566605360304727, -225.9834628568286519 ) ) ;
#10755=CARTESIAN_POINT ( 'NONE',  ( -1.301562195391901877, 16.19210386685474390, -220.0867867038183192 ) ) ;
#10756=CARTESIAN_POINT ( 'NONE',  ( -18.42638600874552424, 7.060399206045774534, -230.3991437614443214 ) ) ;
#10757=CARTESIAN_POINT ( 'NONE',  ( 17.85905871012913693, 8.463974683125162102, -234.6532732619751300 ) ) ;
#10758=CARTESIAN_POINT ( 'NONE',  ( 9.037704487505543227, -20.74919929927824214, -217.6023494967207625 ) ) ;
#10761=CARTESIAN_POINT ( 'NONE',  ( 8.496844655769807630, 14.66037471857024599, -219.1631158796573118 ) ) ;
#10762=CARTESIAN_POINT ( 'NONE',  ( 26.31881739696682843, -8.664992621510689830, -226.4435203923285655 ) ) ;
#10764=CARTESIAN_POINT ( 'NONE',  ( 17.07668571305246985, 2.037405138410691485, -219.7626854147787867 ) ) ;
#10765=CARTESIAN_POINT ( 'NONE',  ( 1.752757082432757185, -17.15725705531007250, -232.7539178101738742 ) ) ;
#10766=CARTESIAN_POINT ( 'NONE',  ( -11.49049084071896409, 11.06834963248926940, -218.3354249205727058 ) ) ;
#10767=CARTESIAN_POINT ( 'NONE',  ( -19.98042543492610079, 23.51949599776966693, -226.6701036947414138 ) ) ;
#10768=CARTESIAN_POINT ( 'NONE',  ( -14.70651859537745487, 4.211702956367679107, -230.0357207626005334 ) ) ;
#10769=CARTESIAN_POINT ( 'NONE',  ( -19.43452863239301820, -21.19996443032342626, -221.1427059245750399 ) ) ;
#10772=CARTESIAN_POINT ( 'NONE',  ( -22.99617382825321599, 17.18101613848176967, -230.9512687019100099 ) ) ;
#10773=CARTESIAN_POINT ( 'NONE',  ( 7.808093059109005196, -25.57408461116448706, -218.1679985877120487 ) ) ;
#10775=CARTESIAN_POINT ( 'NONE',  ( 18.51425713624010427, 11.82474821235740592, -231.3645840199355632 ) ) ;
#10776=CARTESIAN_POINT ( 'NONE',  ( -8.653738780971721667, 11.12943719949617893, -219.7525355316396087 ) ) ;
#10778=CARTESIAN_POINT ( 'NONE',  ( 19.67070349224072956, 16.44307963282299312, -220.0378483479504439 ) ) ;
#10779=CARTESIAN_POINT ( 'NONE',  ( 3.098311947274309919, -13.44192016451707872, -223.0038505953381502 ) ) ;
#10782=CARTESIAN_POINT ( 'NONE',  ( -4.466732464217805898, 19.42663028452474450, -231.9485309169485561 ) ) ;
#10783=CARTESIAN_POINT ( 'NONE',  ( -15.07599795178976443, 12.40109266655585429, -218.9921934537110815 ) ) ;
#10784=CARTESIAN_POINT ( 'NONE',  ( -14.83095329101371540, 1.580869236763225549, -217.8331819987577660 ) ) ;
#10786=CARTESIAN_POINT ( 'NONE',  ( -13.53417258903678722, -8.044363197357762729, -224.1542709308240546 ) ) ;
#10789=CARTESIAN_POINT ( 'NONE',  ( 17.89221702206198117, 0.2742047965568425449, -220.2420650470893122 ) ) ;
#10790=CARTESIAN_POINT ( 'NONE',  ( 2.737864789122675280, -26.51934750686404385, -230.0373452194950517 ) ) ;
#10791=CARTESIAN_POINT ( 'NONE',  ( 18.04365516558436866, 6.721233635139160612, -218.4376093631473168 ) ) ;
#10792=CARTESIAN_POINT ( 'NONE',  ( -3.501680520304516264, 14.31538576447642264, -219.8967178229432307 ) ) ;
#10794=CARTESIAN_POINT ( 'NONE',  ( 25.70350299105564318, 4.008313962570879241, -233.1578316763087173 ) ) ;
#10795=CARTESIAN_POINT ( 'NONE',  ( 8.689059922489732912, 15.18271246186214363, -218.7354841152034908 ) ) ;
#10798=CARTESIAN_POINT ( 'NONE',  ( -18.44715843167851688, -19.86029123650958184, -231.9563062773970046 ) ) ;
#10799=CARTESIAN_POINT ( 'NONE',  ( 15.50779141722566656, -5.694711448414747856, -219.6385356284298211 ) ) ;
#10801=CARTESIAN_POINT ( 'NONE',  ( -21.73153953336191790, 8.758376218440917071, -235.2971293019126051 ) ) ;
#10802=CARTESIAN_POINT ( 'NONE',  ( -21.44067990442788840, -11.35877574734454143, -219.4569350636155605 ) ) ;
#10803=CARTESIAN_POINT ( 'NONE',  ( -13.96147744945181124, 5.260363697127891314, -222.3342733685200301 ) ) ;
#10804=CARTESIAN_POINT ( 'NONE',  ( 16.55626903245587656, 22.80423546114836952, -218.9884947126587633 ) ) ;
#10805=CARTESIAN_POINT ( 'NONE',  ( 5.585286719045844173, 27.51657303716567426, -222.4190945945824751 ) ) ;
#10807=CARTESIAN_POINT ( 'NONE',  ( 22.41656803062015157, -8.700679067278056067, -214.8043567724421337 ) ) ;
#10809=CARTESIAN_POINT ( 'NONE',  ( 28.57344184061583192, 5.631897254180425527, -225.1192013637692355 ) ) ;
#10810=CARTESIAN_POINT ( 'NONE',  ( -18.41237742040652847, 14.06446039901721790, -216.7469276929859632 ) ) ;
#10811=CARTESIAN_POINT ( 'NONE',  ( -13.41298582792616934, 27.85383138489214616, -228.6457525465575884 ) ) ;
#10812=CARTESIAN_POINT ( 'NONE',  ( -13.68337831708448782, -3.656824064325736590, -221.3737413816871538 ) ) ;
#10813=CARTESIAN_POINT ( 'NONE',  ( -13.56774755469388616, 7.311522441667196226, -219.1912666243428021 ) ) ;
#10816=CARTESIAN_POINT ( 'NONE',  ( 16.08921376350389920, -2.840750994787607731, -229.5571464835293796 ) ) ;
#10817=CARTESIAN_POINT ( 'NONE',  ( -14.46024998630872282, 14.54669730493860946, -231.4156670963686508 ) ) ;
#10818=CARTESIAN_POINT ( 'NONE',  ( 28.41961022423218353, 10.76616830294286409, -220.2698681100053193 ) ) ;
#10819=CARTESIAN_POINT ( 'NONE',  ( -29.88125065636863198, 4.504452993877526623, -226.2048141718237275 ) ) ;
#10820=CARTESIAN_POINT ( 'NONE',  ( 10.57926812561479757, 10.00910231482511215, -225.8341706491384286 ) ) ;
#10821=CARTESIAN_POINT ( 'NONE',  ( -14.28784611495131784, -7.281039336628973402, -230.6208668958216208 ) ) ;
#10822=CARTESIAN_POINT ( 'NONE',  ( 5.720314275582434327, 25.17872937134267630, -219.7530083620574430 ) ) ;
#10823=CARTESIAN_POINT ( 'NONE',  ( -4.670971249126254499, -22.80666086768999890, -234.0323572959307512 ) ) ;
#10824=CARTESIAN_POINT ( 'NONE',  ( 11.33210854356620523, 22.81476816607802149, -217.8536224460118262 ) ) ;
#10825=CARTESIAN_POINT ( 'NONE',  ( 7.844578353157877437, -11.10597526584381356, -230.9016046914076128 ) ) ;
#10826=CARTESIAN_POINT ( 'NONE',  ( -14.57944476639264764, 6.129437248167259433, -229.4766146696829310 ) ) ;
#10828=CARTESIAN_POINT ( 'NONE',  ( -28.68324149884075780, -4.473022182960058934, -227.9839418391680681 ) ) ;
#10829=CARTESIAN_POINT ( 'NONE',  ( 3.755404788550845474, 24.96758616565139022, -220.0839658302907935 ) ) ;
#10830=CARTESIAN_POINT ( 'NONE',  ( -21.19360951076126653, 12.15251088906093457, -217.9482185194656552 ) ) ;
#10831=CARTESIAN_POINT ( 'NONE',  ( 22.66390650824515873, 11.48342577402021725, -231.3155567808436217 ) ) ;
#10832=CARTESIAN_POINT ( 'NONE',  ( -11.81856518996410088, -14.35937779267807279, -219.1576658967449305 ) ) ;
#10833=CARTESIAN_POINT ( 'NONE',  ( 15.51445714770079931, 9.275596138242290678, -215.8565574371285436 ) ) ;
#10835=CARTESIAN_POINT ( 'NONE',  ( -4.051702682916754839, -14.52120462818199798, -217.8402208339018671 ) ) ;
#10836=CARTESIAN_POINT ( 'NONE',  ( -9.627017372966443887, 15.60690227900018279, -218.8878023709062859 ) ) ;
#10837=CARTESIAN_POINT ( 'NONE',  ( 17.97920459523930958, 17.43922474653955490, -233.2737719749805763 ) ) ;
#10839=CARTESIAN_POINT ( 'NONE',  ( -25.20870746202117729, 11.68425842440532136, -223.9066764530103342 ) ) ;
#10840=CARTESIAN_POINT ( 'NONE',  ( 0.6332696906856497554, 18.74964962670039625, -234.8596399859513042 ) ) ;
#10841=CARTESIAN_POINT ( 'NONE',  ( 17.28149325064817887, -1.074788064772476792, -229.5315781944399305 ) ) ;
#10842=CARTESIAN_POINT ( 'NONE',  ( 11.82295278175540787, -22.41907685134884076, -220.1071383070178342 ) ) ;
#10843=CARTESIAN_POINT ( 'NONE',  ( 9.020349274477036161, -13.22217574948208529, -220.4173403795374213 ) ) ;
#10844=CARTESIAN_POINT ( 'NONE',  ( 0.6289891638115701067, 16.47510600144228832, -227.0521699048171342 ) ) ;
#10847=CARTESIAN_POINT ( 'NONE',  ( 18.54610009393809023, 0.6523581019769808531, -231.1787333216317677 ) ) ;
#10848=CARTESIAN_POINT ( 'NONE',  ( -14.27185570462694919, -0.4134134650712557035, -229.5903738612280449 ) ) ;
#10849=CARTESIAN_POINT ( 'NONE',  ( -8.514447835183077018, -10.26590951297754195, -225.5321622820681569 ) ) ;
#10850=CARTESIAN_POINT ( 'NONE',  ( 2.513843158659109456, -14.78137297724497401, -219.3443999184743518 ) ) ;
#10851=CARTESIAN_POINT ( 'NONE',  ( -2.532302712337851425, 16.54370602006230939, -228.1940632970506613 ) ) ;
#10853=CARTESIAN_POINT ( 'NONE',  ( -12.12559971566433958, 1.856299769312002912, -227.8748781050665286 ) ) ;
#10854=CARTESIAN_POINT ( 'NONE',  ( -2.735889804569492600, 12.71735652435744512, -225.1194195722198117 ) ) ;
#10855=CARTESIAN_POINT ( 'NONE',  ( 0.04449911090679885967, 16.51968908208873899, -222.9067194156212111 ) ) ;
#10858=CARTESIAN_POINT ( 'NONE',  ( -3.223980134944351317, 26.83284996841001302, -219.5167893230652965 ) ) ;
#10859=CARTESIAN_POINT ( 'NONE',  ( 20.13946171159960841, -0.1427001808266660232, -233.7987036390019853 ) ) ;
#10860=CARTESIAN_POINT ( 'NONE',  ( 16.77642802340811556, -0.6192566135115280535, -218.8326447441449432 ) ) ;
#10861=CARTESIAN_POINT ( 'NONE',  ( 7.640685522499278903, -12.22373526560700441, -226.1755943870604710 ) ) ;
#10863=DIRECTION ( 'NONE',  ( 0.1093404791528972547, -0.9940043559354329039, 0.000000000000000000 ) ) ;
#10865=CARTESIAN_POINT ( 'NONE',  ( 5.623554730548537606, 15.65270319720736225, -231.3185741195121068 ) ) ;
#10866=CARTESIAN_POINT ( 'NONE',  ( 20.55466028792283240, -8.067975053177056211, -219.1472888552992799 ) ) ;
#10869=CARTESIAN_POINT ( 'NONE',  ( 7.486336813247038258, -29.35413437595724773, -221.4114973598149447 ) ) ;
#10870=CARTESIAN_POINT ( 'NONE',  ( -11.33137429837660193, 27.25022425932026238, -230.1650924901870212 ) ) ;
#10871=CARTESIAN_POINT ( 'NONE',  ( -10.33514150881494942, 13.62639309082336503, -216.9544063991933172 ) ) ;
#10873=CARTESIAN_POINT ( 'NONE',  ( -7.395406416482832590, 12.93623984139929739, -219.2606224730616873 ) ) ;
#10874=CARTESIAN_POINT ( 'NONE',  ( -10.39692419770002552, -10.11462123336039021, -222.6538761800393047 ) ) ;
#10876=CARTESIAN_POINT ( 'NONE',  ( -9.740348021262962064, 16.12529029871877384, -216.4361617420699702 ) ) ;
#10877=CARTESIAN_POINT ( 'NONE',  ( 9.552164729858477088, -28.54380927792562872, -224.2925619065192677 ) ) ;
#10880=CARTESIAN_POINT ( 'NONE',  ( -17.79285498209129202, 9.187865686019035749, -216.3798185811636756 ) ) ;
#10882=CARTESIAN_POINT ( 'NONE',  ( 15.54095364727189299, 10.52000078266145700, -230.2714373371992735 ) ) ;
#10883=CARTESIAN_POINT ( 'NONE',  ( -11.23881320317003407, 15.84151802331611236, -234.2799649731619809 ) ) ;
#10885=CARTESIAN_POINT ( 'NONE',  ( 16.07044873961816123, 22.39643131523411412, -226.8512752114033901 ) ) ;
#10886=CARTESIAN_POINT ( 'NONE',  ( -6.954422770286640798, -15.70181985945210634, -221.3390676453758488 ) ) ;
#10888=CARTESIAN_POINT ( 'NONE',  ( 2.808299412262623473, 18.06245856371233316, -217.9832661743849656 ) ) ;
#10889=CARTESIAN_POINT ( 'NONE',  ( -13.14888680331901583, 26.03314517226533908, -227.7900104434697539 ) ) ;
#10890=CARTESIAN_POINT ( 'NONE',  ( -16.65220264499505376, 11.77543314451157563, -216.3149620944649030 ) ) ;
#10892=CARTESIAN_POINT ( 'NONE',  ( -19.48378335617362112, -12.36282430725977655, -218.8185104403611945 ) ) ;
#10895=CARTESIAN_POINT ( 'NONE',  ( -13.92046207272054303, -0.1600067567908077248, -224.5811699126800818 ) ) ;
#10896=CARTESIAN_POINT ( 'NONE',  ( 6.772180301198498675, -16.47206380092378097, -229.1778777248402719 ) ) ;
#10897=CARTESIAN_POINT ( 'NONE',  ( 15.76910524310159900, 5.601482066865847820, -220.3440822020379528 ) ) ;
#10898=CARTESIAN_POINT ( 'NONE',  ( -1.881996891245037995, 28.05344686410985489, -218.6379207300106202 ) ) ;
#10901=CARTESIAN_POINT ( 'NONE',  ( -17.59913672443795463, -0.5356773789333074687, -220.7342471185320960 ) ) ;
#10903=CARTESIAN_POINT ( 'NONE',  ( 24.34047711160105720, 17.90454708687460794, -228.1939002122307159 ) ) ;
#10904=CARTESIAN_POINT ( 'NONE',  ( 18.50911814746675788, 15.92944434255054453, -232.0449215596906072 ) ) ;
#10906=CARTESIAN_POINT ( 'NONE',  ( -11.28700884291539630, -21.85791790461604478, -233.5354093188319951 ) ) ;
#10907=CARTESIAN_POINT ( 'NONE',  ( 4.682724365302521896, -22.35092628325669750, -215.9543778044225348 ) ) ;
#10910=CARTESIAN_POINT ( 'NONE',  ( -7.329856113536736828, 10.17606210583481818, -226.3085553030691415 ) ) ;
#10911=CARTESIAN_POINT ( 'NONE',  ( -15.83567870103663466, -7.501751145129069265, -221.2716155488439824 ) ) ;
#10915=CARTESIAN_POINT ( 'NONE',  ( -19.65084584916038324, 18.01805631773661176, -219.5040736310571106 ) ) ;
#10916=CARTESIAN_POINT ( 'NONE',  ( 11.01659168199870287, 19.17922986229587323, -233.3715978632214387 ) ) ;
#10917=CARTESIAN_POINT ( 'NONE',  ( 0.7903203334012884884, 21.30772501796948859, -217.9064416298261619 ) ) ;
#10919=CARTESIAN_POINT ( 'NONE',  ( 17.65733440236621732, -13.95165017647719452, -214.8231966952668301 ) ) ;
#10920=CARTESIAN_POINT ( 'NONE',  ( 15.52719855059926424, 1.633696074270991172, -221.7349885876216433 ) ) ;
#10921=CARTESIAN_POINT ( 'NONE',  ( 1.557078628722260438, 24.20011951319323273, -235.1441088220640268 ) ) ;
#10922=CARTESIAN_POINT ( 'NONE',  ( -19.27153818831731158, 23.75761453444584248, -221.9111479746408975 ) ) ;
#10923=CARTESIAN_POINT ( 'NONE',  ( -29.90835019730369737, -3.078401082523886334, -228.7630230812432046 ) ) ;
#10924=CARTESIAN_POINT ( 'NONE',  ( -23.98802705797876200, 19.46654170242919690, -223.5293093576406989 ) ) ;
#10926=CARTESIAN_POINT ( 'NONE',  ( 16.50235023187294203, -3.000022380394500310, -230.0447763498268614 ) ) ;
#10928=CARTESIAN_POINT ( 'NONE',  ( -4.974038791218384326, 28.61915055369004079, -219.5057940952933961 ) ) ;
#10929=CARTESIAN_POINT ( 'NONE',  ( 21.75737151495493649, -2.205713500382455283, -233.2756072794337285 ) ) ;
#10930=CARTESIAN_POINT ( 'NONE',  ( -20.26851768784797869, -0.8260594303982465858, -217.1279713726092098 ) ) ;
#10932=CARTESIAN_POINT ( 'NONE',  ( 11.62313423782632782, 11.98467543564608029, -219.7293303032897995 ) ) ;
#10933=CARTESIAN_POINT ( 'NONE',  ( -22.54883021006152433, -16.50439104605484530, -230.5104955902558004 ) ) ;
#10934=CARTESIAN_POINT ( 'NONE',  ( -1.582540545905128049, 14.52388882916313584, -222.9138157219475147 ) ) ;
#10935=CARTESIAN_POINT ( 'NONE',  ( -7.800954605602409053, -29.95157606033723496, -226.5906573908930000 ) ) ;
#10936=CARTESIAN_POINT ( 'NONE',  ( 7.995304978256253747, 13.28024228361502779, -220.6535174700288451 ) ) ;
#10937=CARTESIAN_POINT ( 'NONE',  ( 4.956111054478943068, -16.91316901532391270, -234.1076498343193748 ) ) ;
#10939=CARTESIAN_POINT ( 'NONE',  ( -17.49393085256189906, 10.63366922396483361, -217.7502683347138657 ) ) ;
#10940=SURFACE_STYLE_FILL_AREA ( #5534 ) ;
#10941=CARTESIAN_POINT ( 'NONE',  ( -22.16366393984728234, -4.852915104599624385, -232.2864540303542924 ) ) ;
#10943=CARTESIAN_POINT ( 'NONE',  ( 4.152856881432678726, 16.71326706899027670, -228.3712188091315909 ) ) ;
#10944=CARTESIAN_POINT ( 'NONE',  ( -23.20103936322198024, 10.64725167743880085, -231.7714206262400864 ) ) ;
#10945=CARTESIAN_POINT ( 'NONE',  ( 15.61962121506769385, 4.525360868525488911, -229.0684696061408090 ) ) ;
#10946=CARTESIAN_POINT ( 'NONE',  ( -20.23770393675990675, -19.63250941609856426, -227.7987059506201319 ) ) ;
#10947=CARTESIAN_POINT ( 'NONE',  ( 23.07558131619435571, 16.33594519118144817, -217.0553921114837124 ) ) ;
#10950=CARTESIAN_POINT ( 'NONE',  ( -18.70843642779997040, -17.48186590846855992, -215.2841814587906981 ) ) ;
#10951=CARTESIAN_POINT ( 'NONE',  ( 10.40160332990717151, 27.59713857063802323, -221.5374724512453213 ) ) ;
#10952=CARTESIAN_POINT ( 'NONE',  ( 19.40629804599390340, 15.10110417999774057, -216.3942729496570223 ) ) ;
#10953=CARTESIAN_POINT ( 'NONE',  ( -11.69222874857179484, 25.57550432052970280, -219.9467848335519591 ) ) ;
#10954=CARTESIAN_POINT ( 'NONE',  ( -8.995433708001568718, 13.44373928221519243, -231.9251680978426577 ) ) ;
#10955=CARTESIAN_POINT ( 'NONE',  ( 21.83031488337932657, -1.542591969257240070, -231.3901500139511427 ) ) ;
#10957=CARTESIAN_POINT ( 'NONE',  ( 14.94332666820587008, -17.95933738324940165, -219.3037465242801147 ) ) ;
#10959=CARTESIAN_POINT ( 'NONE',  ( 10.73531068932428667, -10.59494929936097307, -229.0901643129046192 ) ) ;
#10962=CARTESIAN_POINT ( 'NONE',  ( -21.89065952084861522, -0.9940043559354512226, -215.0000000000000000 ) ) ;
#10963=CARTESIAN_POINT ( 'NONE',  ( -13.58432508418311180, -0.3977623232610293935, -228.1278904906119465 ) ) ;
#10964=CARTESIAN_POINT ( 'NONE',  ( -25.61235545225478560, -15.41032726095661509, -226.9890212492312855 ) ) ;
#10965=CARTESIAN_POINT ( 'NONE',  ( -1.308474130992312023, -24.58654860180777391, -216.2430112183533026 ) ) ;
#10967=CARTESIAN_POINT ( 'NONE',  ( 8.632180352507942800, 16.83956698119041917, -230.4752415867875186 ) ) ;
#10969=CARTESIAN_POINT ( 'NONE',  ( -31.04267853410473421, 7.029517189377418873, -226.8060334161593516 ) ) ;
#10970=CARTESIAN_POINT ( 'NONE',  ( -3.205260335674071648, 17.52234722004434531, -232.9754319808710363 ) ) ;
#10971=CARTESIAN_POINT ( 'NONE',  ( 2.021807401899061496, 24.17554150923399092, -230.4042646614662146 ) ) ;
#10972=CARTESIAN_POINT ( 'NONE',  ( 18.65267415280877117, -0.4843198157805662651, -217.0419311198673711 ) ) ;
#10975=CARTESIAN_POINT ( 'NONE',  ( 14.69879291197755222, 10.86005690695417236, -216.7815908316746913 ) ) ;
#10976=CARTESIAN_POINT ( 'NONE',  ( -18.67270963783218463, 15.11229250701181925, -218.9067109956068578 ) ) ;
#10977=CARTESIAN_POINT ( 'NONE',  ( 13.85822045549773129, -1.469587484828172919, -226.8778453516271156 ) ) ;
#10978=CARTESIAN_POINT ( 'NONE',  ( -3.176860551132370425, -19.01962362838126452, -231.5826211182368297 ) ) ;
#10981=CARTESIAN_POINT ( 'NONE',  ( 15.12287735332712835, 21.03907941686458116, -231.7894952627153202 ) ) ;
#10982=CARTESIAN_POINT ( 'NONE',  ( -32.05942529185317369, -1.254016050025921425, -226.3193970476597485 ) ) ;
#10983=CARTESIAN_POINT ( 'NONE',  ( -18.05576253097465766, 2.935622250037499104, -232.1557308718028594 ) ) ;
#10986=CARTESIAN_POINT ( 'NONE',  ( 11.14834367153813233, -21.42845646353120870, -216.4520112529555718 ) ) ;
#10988=CARTESIAN_POINT ( 'NONE',  ( 0.9046320824004248085, 13.39785254849979701, -226.4815711199935890 ) ) ;
#10989=CARTESIAN_POINT ( 'NONE',  ( -11.27928845652762213, 14.86256579634383002, -216.2427993537644966 ) ) ;
#10991=CARTESIAN_POINT ( 'NONE',  ( -9.749377714296398878, 10.28442384816749922, -229.3722863967025205 ) ) ;
#10992=CARTESIAN_POINT ( 'NONE',  ( -23.85568197540453994, -15.41036827548725618, -219.8503866864575969 ) ) ;
#10995=CARTESIAN_POINT ( 'NONE',  ( -14.73016414256368911, 22.23431809695627237, -217.1425123644553707 ) ) ;
#10996=CARTESIAN_POINT ( 'NONE',  ( 7.896007729111394369, -13.22437314876957437, -221.6501328817743683 ) ) ;
#10998=CARTESIAN_POINT ( 'NONE',  ( -15.48255455842386219, 10.01793346089237069, -233.1197357361336913 ) ) ;
#11001=CARTESIAN_POINT ( 'NONE',  ( -11.36937006530106586, 5.486019310970209339, -224.0742584078730033 ) ) ;
#11002=CARTESIAN_POINT ( 'NONE',  ( -1.946052076048385482, 22.23149728939677061, -232.8927760318659068 ) ) ;
#11004=CARTESIAN_POINT ( 'NONE',  ( 19.10353041285295816, 2.510539514498965730, -232.1135168369976896 ) ) ;
#11005=CARTESIAN_POINT ( 'NONE',  ( -10.44804907229818980, -15.26164834479392240, -220.3887109030195859 ) ) ;
#11008=CARTESIAN_POINT ( 'NONE',  ( 5.803912621764987456, 13.01725692290267844, -221.8367675400179166 ) ) ;
#11009=CARTESIAN_POINT ( 'NONE',  ( -11.86888352782322897, 15.29489941890347282, -218.1379771575364259 ) ) ;
#11010=CARTESIAN_POINT ( 'NONE',  ( -8.463283775975803280, 12.69606588598396613, -228.6351674091961286 ) ) ;
#11011=CARTESIAN_POINT ( 'NONE',  ( -15.91852731338648752, -4.625608912867816613, -229.2691880628015895 ) ) ;
#11014=CARTESIAN_POINT ( 'NONE',  ( 15.70515172005171323, -0.7403987186381333352, -226.4590404369862995 ) ) ;
#11015=CARTESIAN_POINT ( 'NONE',  ( 6.726326701167932853, -14.50135447204537087, -224.8733857281379755 ) ) ;
#11016=CARTESIAN_POINT ( 'NONE',  ( 22.02796522526679723, 16.41909032291435366, -220.1590600991317217 ) ) ;
#11017=CARTESIAN_POINT ( 'NONE',  ( 5.331555957413248059, 27.50712867803999728, -219.0801070358024276 ) ) ;
#11019=CARTESIAN_POINT ( 'NONE',  ( -22.18165477997343871, 9.502253276305026475, -218.0070055737419636 ) ) ;
#11020=CARTESIAN_POINT ( 'NONE',  ( 19.66580438618080251, 15.18147523775131624, -233.5153994334876586 ) ) ;
#11021=CARTESIAN_POINT ( 'NONE',  ( 10.57926812561479757, 10.00910231482511215, -225.8341706491384286 ) ) ;
#11023=CARTESIAN_POINT ( 'NONE',  ( -11.49803752765619258, -8.459563989871591971, -222.4296168992866853 ) ) ;
#11024=CARTESIAN_POINT ( 'NONE',  ( 8.510712203779903007, -27.79691582975998898, -230.5316902582456180 ) ) ;
#11028=CARTESIAN_POINT ( 'NONE',  ( -16.58369694688956741, 24.75758513462668375, -230.3405478298966784 ) ) ;
#11029=CARTESIAN_POINT ( 'NONE',  ( 11.86238739854314872, -1.469869507039519130, -223.6725020993723660 ) ) ;
#11030=CARTESIAN_POINT ( 'NONE',  ( 24.59129902578158067, -8.191391589517788674, -218.4338547727923299 ) ) ;
#11031=CARTESIAN_POINT ( 'NONE',  ( 21.38922145650625239, 17.10616209967719215, -217.8354246241890451 ) ) ;
#11032=CARTESIAN_POINT ( 'NONE',  ( 10.64724148863252395, 12.28344647332184181, -223.6549461381946173 ) ) ;
#11034=CARTESIAN_POINT ( 'NONE',  ( 12.30978816035033496, -6.276705103789536722, -231.2162571060900405 ) ) ;
#11035=CARTESIAN_POINT ( 'NONE',  ( 14.19800769603076240, 4.587407146151301518, -224.2928935459285071 ) ) ;
#11037=CARTESIAN_POINT ( 'NONE',  ( 1.920320557106582893, 25.99317453242502296, -234.5637964893073217 ) ) ;
#11038=CARTESIAN_POINT ( 'NONE',  ( -8.005900519654911562, 11.01772743098285545, -228.7074549843708269 ) ) ;
#11039=CARTESIAN_POINT ( 'NONE',  ( -21.94776718874828347, -0.4748437386657700099, -216.1214812709574176 ) ) ;
#11040=CARTESIAN_POINT ( 'NONE',  ( -18.47334320050258327, 24.79293862780133040, -226.9986786077537317 ) ) ;
#11042=CARTESIAN_POINT ( 'NONE',  ( 24.59129902578158067, -8.191391589517788674, -218.4338547727923299 ) ) ;
#11043=CARTESIAN_POINT ( 'NONE',  ( -6.388048297418547961, 21.92257289597608150, -233.3290245341164848 ) ) ;
#11044=CARTESIAN_POINT ( 'NONE',  ( 22.17049319811867036, 0.5483778423327810847, -216.5715983009590673 ) ) ;
#11045=CARTESIAN_POINT ( 'NONE',  ( -12.31207293045244988, 6.732038552366256923, -221.0952066824360713 ) ) ;
#11046=CARTESIAN_POINT ( 'NONE',  ( 19.19288224840068935, 10.13059690604263174, -232.1906135022504998 ) ) ;
#11047=CARTESIAN_POINT ( 'NONE',  ( -28.12632608809566293, -1.403418003803144742, -218.5233027210585988 ) ) ;
#11049=CARTESIAN_POINT ( 'NONE',  ( 2.914696262605396715, 19.49933023975583879, -231.6035545612375017 ) ) ;
#11050=CARTESIAN_POINT ( 'NONE',  ( -14.78079095050690661, -5.416970230978240153, -229.7193632018645246 ) ) ;
#11051=CARTESIAN_POINT ( 'NONE',  ( 4.301648988406530094, 13.23079486486395240, -223.2766268961034655 ) ) ;
#11052=CARTESIAN_POINT ( 'NONE',  ( -7.242471263717580321, -12.67345288765796774, -222.7008556220510229 ) ) ;
#11054=CARTESIAN_POINT ( 'NONE',  ( -13.51406939156936104, 10.04301168678160749, -230.1761202643687056 ) ) ;
#11055=CARTESIAN_POINT ( 'NONE',  ( -29.43130594997593974, -3.977420319584657360, -224.3854249914923571 ) ) ;
#11056=CARTESIAN_POINT ( 'NONE',  ( 3.528957931946373971, 27.43889307663531696, -223.4805233499528185 ) ) ;
#11057=CARTESIAN_POINT ( 'NONE',  ( -14.69827142695382527, 14.49176359921644597, -217.9600391472806109 ) ) ;
#11058=CARTESIAN_POINT ( 'NONE',  ( -24.77996431573922820, 10.49354383977773786, -234.1655613096203581 ) ) ;
#11059=CARTESIAN_POINT ( 'NONE',  ( -9.870642741937645681, -28.68889699630894441, -223.8025096038410879 ) ) ;
#11060=CARTESIAN_POINT ( 'NONE',  ( 25.12984891811676036, 19.96069634721137476, -226.7154725927711070 ) ) ;
#11062=CARTESIAN_POINT ( 'NONE',  ( -18.68851093906118521, -8.564152624513159395, -215.1804141040323941 ) ) ;
#11063=CARTESIAN_POINT ( 'NONE',  ( -1.772400894765090662, 19.49811434610897010, -217.8797837662441168 ) ) ;
#11064=CARTESIAN_POINT ( 'NONE',  ( -22.10934047915413814, 0.9940043559354462266, -218.9999999999999716 ) ) ;
#11065=CARTESIAN_POINT ( 'NONE',  ( -5.854583994961135573, 13.10358817970001866, -222.4168379437668648 ) ) ;
#11067=CARTESIAN_POINT ( 'NONE',  ( 19.20222574149634909, 21.83532798770326266, -218.6913543321078919 ) ) ;
#11069=CARTESIAN_POINT ( 'NONE',  ( -3.159549884399295294, -15.02780241139942952, -220.2520066652115531 ) ) ;
#11070=CARTESIAN_POINT ( 'NONE',  ( 3.619268272960482591, -21.10655420957111517, -217.8630709410095108 ) ) ;
#11073=CARTESIAN_POINT ( 'NONE',  ( 25.69300549816939494, 5.947472783069708946, -230.6131061331718115 ) ) ;
#11074=CARTESIAN_POINT ( 'NONE',  ( 20.80196158924851701, -7.261721507697286526, -217.3074963141844194 ) ) ;
#11076=CARTESIAN_POINT ( 'NONE',  ( -9.078153229956912540, -10.71731945587431056, -228.5228069477245469 ) ) ;
#11077=CARTESIAN_POINT ( 'NONE',  ( -6.512931564893298386, -17.32529878264574563, -216.7284160531958719 ) ) ;
#11078=CARTESIAN_POINT ( 'NONE',  ( 8.179023008129211902, 20.84698146175953681, -218.6376653143925921 ) ) ;
#11080=CARTESIAN_POINT ( 'NONE',  ( 22.24262848503957812, 2.205713500382371794, -232.7243927205662430 ) ) ;
#11081=CARTESIAN_POINT ( 'NONE',  ( -6.282398543089500187, 12.01615879894893801, -228.5121145169883903 ) ) ;
#11082=CARTESIAN_POINT ( 'NONE',  ( 3.614175329767659761, 21.98488100320606264, -219.0898850257099753 ) ) ;
#11083=CARTESIAN_POINT ( 'NONE',  ( 15.97952439233267263, -1.339455371059026456, -231.0376074705642395 ) ) ;
#11085=CARTESIAN_POINT ( 'NONE',  ( 11.01659168199870287, 19.17922986229587323, -233.3715978632214387 ) ) ;
#11086=CARTESIAN_POINT ( 'NONE',  ( -17.30580402557236752, 11.30149179219993982, -230.8639894634705172 ) ) ;
#11087=CARTESIAN_POINT ( 'NONE',  ( 29.08100487150598212, 12.14819438347179670, -226.9621620069135020 ) ) ;
#11088=CARTESIAN_POINT ( 'NONE',  ( -1.380908993000753648, -20.21092959135559752, -218.0995018783601438 ) ) ;
#11091=CARTESIAN_POINT ( 'NONE',  ( 17.97843143658897347, 22.12221935793617078, -220.9346589834416079 ) ) ;
#11092=CARTESIAN_POINT ( 'NONE',  ( 20.16749130626988773, -19.72590806003585229, -223.0880382675181579 ) ) ;
#11093=CARTESIAN_POINT ( 'NONE',  ( -20.45797657813638182, 1.164962349958370336, -217.1306074022350572 ) ) ;
#11095=CARTESIAN_POINT ( 'NONE',  ( -10.42804209284631156, -14.08702332024887305, -217.7386024361820489 ) ) ;
#11096=CARTESIAN_POINT ( 'NONE',  ( 4.389496648589924277, 14.47660514356954131, -220.6151178996808540 ) ) ;
#11097=CARTESIAN_POINT ( 'NONE',  ( -0.8357710952364670876, 15.48480697989137234, -216.9118565312697910 ) ) ;
#11098=EDGE_LOOP ( 'NONE', ( #20681, #16985, #18711, #3859, #4740, #3491 ) ) ;
#11099=CARTESIAN_POINT ( 'NONE',  ( -21.02719846458807851, 18.12262440796364871, -218.0220709499931502 ) ) ;
#11100=CARTESIAN_POINT ( 'NONE',  ( 26.82025090637478115, -4.850230565203020205, -219.1860060474940042 ) ) ;
#11103=CARTESIAN_POINT ( 'NONE',  ( -6.201839134465864767, 11.37481922992157379, -223.7040893475979146 ) ) ;
#11104=CARTESIAN_POINT ( 'NONE',  ( 2.018545692720245643, -30.97649562252411215, -224.4812544443210811 ) ) ;
#11105=CARTESIAN_POINT ( 'NONE',  ( 15.50779141722566656, -5.694711448414747856, -219.6385356284298211 ) ) ;
#11106=CARTESIAN_POINT ( 'NONE',  ( -13.83274569775339202, 16.20364235096346661, -234.0851861771356539 ) ) ;
#11107=CARTESIAN_POINT ( 'NONE',  ( -13.34869474643618581, 6.516017165032126357, -231.2228057326931321 ) ) ;
#11108=CARTESIAN_POINT ( 'NONE',  ( -1.973648319964989462, 15.33498294326524203, -220.9958390492969329 ) ) ;
#11111=CARTESIAN_POINT ( 'NONE',  ( 21.43345597994050777, 2.294722475943265838, -232.7243927205661294 ) ) ;
#11112=CARTESIAN_POINT ( 'NONE',  ( -14.02781974392415165, -24.18658813864446344, -225.1634145543362706 ) ) ;
#11114=CARTESIAN_POINT ( 'NONE',  ( 17.24952650401854370, 25.19767938110938843, -224.5319471861414797 ) ) ;
#11115=CARTESIAN_POINT ( 'NONE',  ( -8.900302563431933933, 20.17395648083808268, -216.9116515890487733 ) ) ;
#11116=CARTESIAN_POINT ( 'NONE',  ( -9.115411286166651195, 13.66191091052436235, -230.3338332872444312 ) ) ;
#11117=CARTESIAN_POINT ( 'NONE',  ( -29.37537067777813604, -4.151788015186005154, -225.5750753894876368 ) ) ;
#11120=CARTESIAN_POINT ( 'NONE',  ( 17.47660375112063491, 0.1533180678384444551, -220.6249646429494931 ) ) ;
#11121=CARTESIAN_POINT ( 'NONE',  ( -4.075588186332946172, -27.83231707117609588, -229.7735430035053810 ) ) ;
#11122=CARTESIAN_POINT ( 'NONE',  ( 27.04607490430786854, 4.607450003618843049, -220.3758934308003461 ) ) ;
#11123=CARTESIAN_POINT ( 'NONE',  ( -3.205260335674071648, 17.52234722004434531, -232.9754319808710363 ) ) ;
#11124=CARTESIAN_POINT ( 'NONE',  ( 15.02522163627726037, -2.279509738242128769, -223.0471089487919585 ) ) ;
#11125=CARTESIAN_POINT ( 'NONE',  ( -28.00010259152825398, 3.831607968041374157, -225.8381323513402208 ) ) ;
#11126=CARTESIAN_POINT ( 'NONE',  ( 7.116434306140963173, 9.967665124511082553, -224.4990387090310833 ) ) ;
#11127=CARTESIAN_POINT ( 'NONE',  ( 22.02796522526679723, 16.41909032291435366, -220.1590600991317217 ) ) ;
#11129=CARTESIAN_POINT ( 'NONE',  ( -12.00435701841128022, -1.798699874815819166, -227.7674894005143074 ) ) ;
#11130=CARTESIAN_POINT ( 'NONE',  ( -21.28605893225895684, -20.43870967537180050, -221.0356759888913700 ) ) ;
#11131=CARTESIAN_POINT ( 'NONE',  ( 6.260999666360449467, -13.19315344885661645, -220.2890618333529744 ) ) ;
#11134=CARTESIAN_POINT ( 'NONE',  ( -2.043230952238195286, 23.63069326910348877, -232.6835180461029040 ) ) ;
#11135=CARTESIAN_POINT ( 'NONE',  ( 29.01190720243894461, 0.5135883731763817295, -231.9442528450179566 ) ) ;
#11136=CARTESIAN_POINT ( 'NONE',  ( 13.28406271702445274, -5.237238614233280742, -225.2640488721434622 ) ) ;
#11137=CARTESIAN_POINT ( 'NONE',  ( -18.74633356284308761, 11.17209001323738704, -217.5809474206552068 ) ) ;
#11138=CARTESIAN_POINT ( 'NONE',  ( 16.64575860537911112, 25.12688477742292648, -227.5050599151411745 ) ) ;
#11139=CARTESIAN_POINT ( 'NONE',  ( 14.12692363916921146, 20.59586666873830296, -230.0804552526094540 ) ) ;
#11141=CARTESIAN_POINT ( 'NONE',  ( 4.746237488610151267, -29.30821474977460639, -222.1257927337785247 ) ) ;
#11143=CARTESIAN_POINT ( 'NONE',  ( -12.15711705271618470, 28.08001788883979799, -220.3431297925021681 ) ) ;
#11144=CARTESIAN_POINT ( 'NONE',  ( -13.24620988741752825, 28.78239319002125285, -225.3527830703614256 ) ) ;
#11145=CARTESIAN_POINT ( 'NONE',  ( -14.84457943406284208, -4.054717634150219574, -219.4128920803699430 ) ) ;
#11146=CARTESIAN_POINT ( 'NONE',  ( -7.429838964355703901, 14.87322129099639234, -232.2632863647814077 ) ) ;
#11149=CARTESIAN_POINT ( 'NONE',  ( 20.80196158924851701, -7.261721507697286526, -217.3074963141844194 ) ) ;
#11150=CARTESIAN_POINT ( 'NONE',  ( -5.854583994961135573, 13.10358817970001866, -222.4168379437668648 ) ) ;
#11151=CARTESIAN_POINT ( 'NONE',  ( 20.64287812348744566, 0.2024751443801864337, -216.7518974727033481 ) ) ;
#11152=CARTESIAN_POINT ( 'NONE',  ( -15.82069055112642353, 8.315535108674763976, -217.2800172218543935 ) ) ;
#11153=CARTESIAN_POINT ( 'NONE',  ( 26.29894631880581812, 12.29609390142961090, -226.3100047295820332 ) ) ;
#11154=CARTESIAN_POINT ( 'NONE',  ( 15.63557944520553988, 0.5893374091412190152, -227.9430452042592208 ) ) ;
#11156=CARTESIAN_POINT ( 'NONE',  ( 5.066530254613678785, 15.76189963344335254, -222.1234037505291781 ) ) ;
#11157=CARTESIAN_POINT ( 'NONE',  ( -18.75993824683981970, -9.028840681436806292, -217.1556094966459227 ) ) ;
#11158=CARTESIAN_POINT ( 'NONE',  ( 26.24002132888527328, 11.62331517472360964, -222.5300873157218859 ) ) ;
#11159=CARTESIAN_POINT ( 'NONE',  ( 0.2060740257213805326, -13.46849591350090947, -221.0879548523055860 ) ) ;
#11161=CARTESIAN_POINT ( 'NONE',  ( -21.66803296057637951, 19.04503900041684616, -222.6603677762044526 ) ) ;
#11162=CARTESIAN_POINT ( 'NONE',  ( 10.05661706967825353, -14.25456047934742365, -218.9909083857680230 ) ) ;
#11163=CARTESIAN_POINT ( 'NONE',  ( 15.56183105618911355, 23.93598532278018354, -223.2746693648072664 ) ) ;
#11164=CARTESIAN_POINT ( 'NONE',  ( -14.24491355791863612, 5.286533920242113105, -221.7104936369346433 ) ) ;
#11165=CARTESIAN_POINT ( 'NONE',  ( -29.15345109632842124, 14.07532767497844262, -225.0972140442887621 ) ) ;
#11166=CARTESIAN_POINT ( 'NONE',  ( -16.33212578464095799, -13.18764990320557118, -218.7248530738716283 ) ) ;
#11167=CARTESIAN_POINT ( 'NONE',  ( 16.84354851290083133, 10.42424693870724361, -215.2582953371023109 ) ) ;
#11169=CARTESIAN_POINT ( 'NONE',  ( -21.92622494339052608, -22.07770017127804962, -220.0303431275545165 ) ) ;
#11170=CARTESIAN_POINT ( 'NONE',  ( 3.846342036506673612, 16.55327908958690131, -231.1358846258000597 ) ) ;
#11171=CARTESIAN_POINT ( 'NONE',  ( 26.59731715018858011, 13.56210517473685329, -229.5787264587298466 ) ) ;
#11172=CARTESIAN_POINT ( 'NONE',  ( -13.06839468023815165, 25.32320678245788059, -229.0099538679170053 ) ) ;
#11173=CARTESIAN_POINT ( 'NONE',  ( 3.672031556878595282, 11.54613252248376831, -227.4694100414545801 ) ) ;
#11176=CARTESIAN_POINT ( 'NONE',  ( -5.579930056231209967, -28.86398153493815144, -221.8494056429758814 ) ) ;
#11178=CARTESIAN_POINT ( 'NONE',  ( 6.869068212838696397, -24.78254998730118430, -231.2855974421026986 ) ) ;
#11179=CARTESIAN_POINT ( 'NONE',  ( 24.57222455393806015, 12.08236629421828212, -229.7319216558644541 ) ) ;
#11180=CARTESIAN_POINT ( 'NONE',  ( 11.43609017326686050, -13.06727081285745307, -217.8903327850316316 ) ) ;
#11181=CARTESIAN_POINT ( 'NONE',  ( 14.01369322398082851, -0.3099216430074364093, -221.6784101578248283 ) ) ;
#11182=CARTESIAN_POINT ( 'NONE',  ( -17.42499862437977853, -18.98713029041037004, -232.7811807006768845 ) ) ;
#11183=CARTESIAN_POINT ( 'NONE',  ( 15.56183105618911355, 23.93598532278018354, -223.2746693648072664 ) ) ;
#11185=CARTESIAN_POINT ( 'NONE',  ( 18.39384604806649648, 2.566915855367216004, -231.7421336352533103 ) ) ;
#11186=CARTESIAN_POINT ( 'NONE',  ( 0.4042326456706432647, 15.50845657815858303, -219.2680337625893401 ) ) ;
#11187=CARTESIAN_POINT ( 'NONE',  ( 7.508136856874425114, 24.19512352541684663, -230.0608033085341617 ) ) ;
#11188=CARTESIAN_POINT ( 'NONE',  ( 22.24262848504226042, 2.205713500382400216, -232.7243927205662999 ) ) ;
#11190=CARTESIAN_POINT ( 'NONE',  ( 10.70175380652492336, 7.370128018021000038, -224.3479584370086286 ) ) ;
#11191=CARTESIAN_POINT ( 'NONE',  ( -14.46024998630872282, 14.54669730493860946, -231.4156670963686508 ) ) ;
#11192=CARTESIAN_POINT ( 'NONE',  ( -27.32994399549947673, 3.379920396491164603, -227.9326384921875217 ) ) ;
#11194=CARTESIAN_POINT ( 'NONE',  ( 1.268102448827562068, -18.18084990330622830, -231.0699201170278911 ) ) ;
#11197=CARTESIAN_POINT ( 'NONE',  ( 4.354034006296288339, 14.09944204372416188, -221.2519525881239417 ) ) ;
#11198=CARTESIAN_POINT ( 'NONE',  ( 17.09791731880535437, -14.50769433911838568, -231.1780219065761059 ) ) ;
#11200=CARTESIAN_POINT ( 'NONE',  ( -8.514447835183077018, -10.26590951297754195, -225.5321622820681569 ) ) ;
#11201=CARTESIAN_POINT ( 'NONE',  ( -3.501680520304516264, 14.31538576447642264, -219.8967178229432307 ) ) ;
#11203=CARTESIAN_POINT ( 'NONE',  ( -4.378220565073127624, 31.53459173284372952, -222.0564199190954753 ) ) ;
#11205=CARTESIAN_POINT ( 'NONE',  ( -9.540790481621398200, 9.981116473660406996, -228.6478862620407995 ) ) ;
#11206=CARTESIAN_POINT ( 'NONE',  ( -21.27082149447729620, -6.316573346028001801, -216.2864220516500779 ) ) ;
#11207=CARTESIAN_POINT ( 'NONE',  ( 29.82766783012230505, -1.714217446056379934, -229.3564438616236316 ) ) ;
#11209=CARTESIAN_POINT ( 'NONE',  ( -13.83274569775339202, 16.20364235096346661, -234.0851861771356539 ) ) ;
#11210=CARTESIAN_POINT ( 'NONE',  ( -22.35094797335686678, -23.29487558099128108, -223.4832390375085538 ) ) ;
#11212=CARTESIAN_POINT ( 'NONE',  ( -22.17339560624464312, 16.26550580028390769, -232.0582861498566274 ) ) ;
#11214=CARTESIAN_POINT ( 'NONE',  ( -12.12559971566433958, 1.856299769312002912, -227.8748781050665286 ) ) ;
#11215=CARTESIAN_POINT ( 'NONE',  ( 1.313727069624702981, 17.80710275190598324, -219.4197901500037062 ) ) ;
#11217=CARTESIAN_POINT ( 'NONE',  ( -21.07387565400155438, 1.107905485989369554, -215.0000000023499069 ) ) ;
#11218=CARTESIAN_POINT ( 'NONE',  ( -16.14140970932308505, -18.57031478189210816, -230.2506069696216287 ) ) ;
#11220=CARTESIAN_POINT ( 'NONE',  ( 10.49811526528768368, 13.26166588535847701, -217.9009921269571919 ) ) ;
#11221=CARTESIAN_POINT ( 'NONE',  ( 1.773237071419721422, 13.09828209437875302, -220.6531024550077404 ) ) ;
#11222=CARTESIAN_POINT ( 'NONE',  ( -13.40354389326479456, 23.35336998323175450, -219.8517474526506987 ) ) ;
#11224=CARTESIAN_POINT ( 'NONE',  ( -25.45695634607983848, -10.72451519803311015, -228.5848280742264933 ) ) ;
#11226=CARTESIAN_POINT ( 'NONE',  ( 17.28149325064817887, -1.074788064772476792, -229.5315781944399305 ) ) ;
#11227=CARTESIAN_POINT ( 'NONE',  ( -3.159549884399295294, -15.02780241139942952, -220.2520066652115531 ) ) ;
#11228=CARTESIAN_POINT ( 'NONE',  ( 15.61962121506769385, 4.525360868525488911, -229.0684696061408090 ) ) ;
#11229=CARTESIAN_POINT ( 'NONE',  ( 4.543450689403089271, 15.91052110650461771, -218.9437823786444426 ) ) ;
#11230=CARTESIAN_POINT ( 'NONE',  ( 14.81724556832271311, -2.803809140094828400, -226.0847343491304855 ) ) ;
#11231=CARTESIAN_POINT ( 'NONE',  ( -15.10760069511485604, 3.026516874529453283, -224.5685390982118861 ) ) ;
#11232=CARTESIAN_POINT ( 'NONE',  ( 11.84598249547323690, 10.36127485500543699, -218.5481300776139904 ) ) ;
#11235=CARTESIAN_POINT ( 'NONE',  ( 21.39553407250273054, 8.453402029343234148, -217.9531594780983141 ) ) ;
#11237=CARTESIAN_POINT ( 'NONE',  ( 27.51601410384567359, -3.359424968747257711, -222.6356212526655725 ) ) ;
#11238=CARTESIAN_POINT ( 'NONE',  ( -18.11268275035277853, -3.459088653808292335, -218.4233329573673359 ) ) ;
#11241=CARTESIAN_POINT ( 'NONE',  ( -9.439286754415764591, 28.32957437491962338, -228.7842975624562598 ) ) ;
#11242=CARTESIAN_POINT ( 'NONE',  ( 29.53814377227115884, -10.02285884041311270, -220.1614914916521286 ) ) ;
#11243=CARTESIAN_POINT ( 'NONE',  ( 24.96294718070021901, -13.86220829677249178, -229.4442241490162075 ) ) ;
#11244=CARTESIAN_POINT ( 'NONE',  ( -16.27882490622757672, 1.520697279646460398, -219.2607721384596289 ) ) ;
#11245=CARTESIAN_POINT ( 'NONE',  ( 8.592982993077152187, 10.20906991731218838, -226.0923132092261483 ) ) ;
#11246=CARTESIAN_POINT ( 'NONE',  ( 21.07144422417032104, 18.33581350331571969, -223.6711752364813890 ) ) ;
#11249=CARTESIAN_POINT ( 'NONE',  ( 0.3267584840439746174, -16.39795729406718650, -220.1296710765888065 ) ) ;
#11252=CARTESIAN_POINT ( 'NONE',  ( 3.982203626615636427, 14.63895582687697150, -217.4952312584269123 ) ) ;
#11253=CARTESIAN_POINT ( 'NONE',  ( -7.403072389817287657, 18.92851032520892929, -215.2068968469505137 ) ) ;
#11254=CARTESIAN_POINT ( 'NONE',  ( 23.56599333006272445, -4.960096179470117050, -217.5996013647105372 ) ) ;
#11255=CARTESIAN_POINT ( 'NONE',  ( -4.104500432947460808, 15.73223271406093460, -218.0734292856946297 ) ) ;
#11258=CARTESIAN_POINT ( 'NONE',  ( -1.884624261322229266, 13.00421381464247084, -226.7648460381863345 ) ) ;
#11259=CARTESIAN_POINT ( 'NONE',  ( -16.23590288079963173, 0.2625226423351309513, -226.8300841971807813 ) ) ;
#11260=CARTESIAN_POINT ( 'NONE',  ( -12.90983082593748676, 14.84936372681532823, -233.8009687022269532 ) ) ;
#11261=CARTESIAN_POINT ( 'NONE',  ( 12.85408565574548412, 7.821283853063205171, -223.1248833997948111 ) ) ;
#11263=CARTESIAN_POINT ( 'NONE',  ( 4.555016420009541989, 17.65848956729471197, -229.5875910199184204 ) ) ;
#11266=CARTESIAN_POINT ( 'NONE',  ( 8.250760074138732136, 14.96691001493985951, -221.7548416114337613 ) ) ;
#11267=CARTESIAN_POINT ( 'NONE',  ( -8.878187501988019648, -11.23476449186280846, -221.0271673637577123 ) ) ;
#11268=CARTESIAN_POINT ( 'NONE',  ( 23.04897566969193079, 17.95862962700741861, -223.6438515760422661 ) ) ;
#11269=CARTESIAN_POINT ( 'NONE',  ( -4.538939863750555581, -15.27574540357637112, -231.4384328720293524 ) ) ;
#11271=CARTESIAN_POINT ( 'NONE',  ( -16.07193224038526580, 12.24477688577882439, -232.1409653212175499 ) ) ;
#11273=CARTESIAN_POINT ( 'NONE',  ( 24.68599888815047194, -16.20242508705913309, -228.6174911781957633 ) ) ;
#11274=CARTESIAN_POINT ( 'NONE',  ( 3.388180927852674884, 15.71154068801650538, -224.9339660840813053 ) ) ;
#11275=CARTESIAN_POINT ( 'NONE',  ( -13.51406939156936104, 10.04301168678160749, -230.1761202643687056 ) ) ;
#11276=CARTESIAN_POINT ( 'NONE',  ( -15.35982698007958724, 5.508237851081846159, -233.6994028941782631 ) ) ;
#11277=CARTESIAN_POINT ( 'NONE',  ( -22.93937586921525806, -8.311597057603599126, -230.3633560851501159 ) ) ;
#11278=CARTESIAN_POINT ( 'NONE',  ( 13.32754126089433377, 12.31312334927721963, -234.6033665822900218 ) ) ;
#11281=CARTESIAN_POINT ( 'NONE',  ( -7.264683844434491000, -10.24731347617596100, -229.2886802738593985 ) ) ;
#11282=CARTESIAN_POINT ( 'NONE',  ( 10.31623634631035991, 26.83927646318382898, -220.2315638557092541 ) ) ;
#11283=CARTESIAN_POINT ( 'NONE',  ( 17.29648694364601980, 10.20782262162153842, -233.8400727604031317 ) ) ;
#11284=CARTESIAN_POINT ( 'NONE',  ( -10.07004052286948337, 22.64471483900350179, -217.4645417110143626 ) ) ;
#11285=CARTESIAN_POINT ( 'NONE',  ( 4.966801760238292118, 27.41406605988239420, -216.4490579899774900 ) ) ;
#11286=CARTESIAN_POINT ( 'NONE',  ( 0.1655890855189643129, -14.86936674525315993, -225.9040401458518943 ) ) ;
#11288=CARTESIAN_POINT ( 'NONE',  ( 5.920190106170357680, -27.41802839654005197, -221.0732524667164114 ) ) ;
#11289=CARTESIAN_POINT ( 'NONE',  ( 16.00819137755116373, 4.595691552992191120, -229.5669508871464757 ) ) ;
#11290=CARTESIAN_POINT ( 'NONE',  ( 13.96958060839473958, -9.488587112651741151, -218.7731372952745232 ) ) ;
#11291=CARTESIAN_POINT ( 'NONE',  ( -28.87859926594958537, -0.8320174534291842061, -222.6356913548140142 ) ) ;
#11292=CARTESIAN_POINT ( 'NONE',  ( -8.491902988188710921, -10.37035003683405066, -223.9502466269643435 ) ) ;
#11294=CARTESIAN_POINT ( 'NONE',  ( 13.41709597927210496, 19.57823531746157997, -218.2666972400567147 ) ) ;
#11296=CARTESIAN_POINT ( 'NONE',  ( 19.79854089336508594, 4.557290221971136646, -217.3342919181881143 ) ) ;
#11298=CARTESIAN_POINT ( 'NONE',  ( -0.1571923090946999446, 19.34188126963334398, -216.6893131123363787 ) ) ;
#11299=CARTESIAN_POINT ( 'NONE',  ( -0.6272116608575281083, 20.18031380156121202, -219.3960054794027030 ) ) ;
#11300=CARTESIAN_POINT ( 'NONE',  ( 12.77158894069672357, -20.43488010613652150, -235.1868042311012914 ) ) ;
#11301=CARTESIAN_POINT ( 'NONE',  ( 11.43247012502872728, 12.44034019618676190, -231.9336559008378629 ) ) ;
#11302=CARTESIAN_POINT ( 'NONE',  ( -18.59263364681495290, 22.28600439725833482, -224.9897462721271779 ) ) ;
#11303=CARTESIAN_POINT ( 'NONE',  ( -19.50431861204945605, -0.7624880359591150736, -219.4666829195064395 ) ) ;
#11304=CARTESIAN_POINT ( 'NONE',  ( 1.167080303844580058, -21.82675117811238152, -232.1335090276773485 ) ) ;
#11308=CARTESIAN_POINT ( 'NONE',  ( 26.48990917286906921, 12.16675355942207659, -225.0153622588060216 ) ) ;
#11309=CARTESIAN_POINT ( 'NONE',  ( 14.07866085257239419, -11.11077054092157645, -229.4139412770749971 ) ) ;
#11311=CARTESIAN_POINT ( 'NONE',  ( -11.40116373163465369, -15.95513543764466213, -216.7841692646331353 ) ) ;
#11313=CARTESIAN_POINT ( 'NONE',  ( -3.368164009525018265, 19.03203264544105622, -233.5986411977714567 ) ) ;
#11314=CARTESIAN_POINT ( 'NONE',  ( 3.744112528862662881, 31.76296354843916703, -227.8872370379487506 ) ) ;
#11316=CARTESIAN_POINT ( 'NONE',  ( -18.70100282803782576, 16.58357028540773115, -216.4425743468854080 ) ) ;
#11317=CARTESIAN_POINT ( 'NONE',  ( -28.09913862414779473, -9.456046895945956265, -221.0065986266286870 ) ) ;
#11319=CARTESIAN_POINT ( 'NONE',  ( 27.12528000378512871, -1.050705938820645224, -232.4139529590446784 ) ) ;
#11321=CARTESIAN_POINT ( 'NONE',  ( -8.172572110426221670, 16.86653848210977813, -233.4220330256369493 ) ) ;
#11322=CARTESIAN_POINT ( 'NONE',  ( -6.616223485457675579, -9.589312190179589024, -225.7195100648197581 ) ) ;
#11323=CARTESIAN_POINT ( 'NONE',  ( 19.06212547406409641, -9.287000003594721775, -232.7453815625877667 ) ) ;
#11324=CARTESIAN_POINT ( 'NONE',  ( -22.11084984981285118, 10.96048252433489623, -216.6117774006995376 ) ) ;
#11325=CARTESIAN_POINT ( 'NONE',  ( -20.05025075566126702, 1.207204931470905018, -215.1628017022767949 ) ) ;
#11326=CARTESIAN_POINT ( 'NONE',  ( 5.585286719045844173, 27.51657303716567426, -222.4190945945824751 ) ) ;
#11328=CARTESIAN_POINT ( 'NONE',  ( -14.99655511003079233, 2.316638599135941945, -232.4215266639120046 ) ) ;
#11329=CARTESIAN_POINT ( 'NONE',  ( -7.469054245001129466, -18.21857363335801594, -219.2823717272210047 ) ) ;
#11331=CARTESIAN_POINT ( 'NONE',  ( -10.29720673141181209, 11.14783905173092649, -222.8560683878917530 ) ) ;
#11332=CARTESIAN_POINT ( 'NONE',  ( 7.772443558932104146, 25.24620711463332157, -231.7813173736589931 ) ) ;
#11333=CARTESIAN_POINT ( 'NONE',  ( -5.762781846020777365, 12.94769902409342777, -223.1319556069387886 ) ) ;
#11335=CARTESIAN_POINT ( 'NONE',  ( 22.46263922039936745, -3.404486942579552089, -216.1438077301478415 ) ) ;
#11339=CARTESIAN_POINT ( 'NONE',  ( -22.17339560624464312, 16.26550580028390769, -232.0582861498566274 ) ) ;
#11340=CARTESIAN_POINT ( 'NONE',  ( -12.42003616114091358, -24.71691410793946986, -217.8239624370676779 ) ) ;
#11342=CARTESIAN_POINT ( 'NONE',  ( 11.57669841200422134, 10.63052136557218574, -228.9489978335593889 ) ) ;
#11344=CARTESIAN_POINT ( 'NONE',  ( 14.95834318372430083, -1.617016552789838801, -229.6306532055809271 ) ) ;
#11345=CARTESIAN_POINT ( 'NONE',  ( 24.78222556642275620, 17.97262539535998371, -226.6641400693514470 ) ) ;
#11346=( LENGTH_UNIT ( ) NAMED_UNIT ( * ) SI_UNIT ( .MILLI., .METRE. ) );
#11347=CARTESIAN_POINT ( 'NONE',  ( 15.42019186727181257, 1.458536399438582043, -222.3758756028272785 ) ) ;
#11349=CARTESIAN_POINT ( 'NONE',  ( 18.23324537670537993, 23.47692953258263771, -224.8333321331434433 ) ) ;
#11351=CARTESIAN_POINT ( 'NONE',  ( 15.35804315687698107, -7.528275283329426415, -228.0874909612831232 ) ) ;
#11352=CARTESIAN_POINT ( 'NONE',  ( -25.42089018817326007, -6.263968923056941307, -218.6542964065910439 ) ) ;
#11356=CARTESIAN_POINT ( 'NONE',  ( -7.312583518931054627, 16.22063427959223958, -217.3454962955413521 ) ) ;
#11357=CARTESIAN_POINT ( 'NONE',  ( 12.24504971509987072, -1.481354005294047926, -221.9045230856115438 ) ) ;
#11358=CARTESIAN_POINT ( 'NONE',  ( 29.12543877365354916, -1.475122899492763873, -224.0746120762670444 ) ) ;
#11359=CARTESIAN_POINT ( 'NONE',  ( -27.92885697401080591, 6.962042978589167319, -220.9552227796709190 ) ) ;
#11360=CARTESIAN_POINT ( 'NONE',  ( 13.30790133003807441, 0.6370684082013071681, -222.3495379725305270 ) ) ;
#11361=CARTESIAN_POINT ( 'NONE',  ( 19.59567110982616001, 18.11097967140601028, -228.7314497914969706 ) ) ;
#11363=CARTESIAN_POINT ( 'NONE',  ( 5.902215564816073012, -11.20991439657816358, -226.4118943921501170 ) ) ;
#11365=CARTESIAN_POINT ( 'NONE',  ( -26.98548179121306845, 3.096138561569834913, -233.8324893795610251 ) ) ;
#11366=CARTESIAN_POINT ( 'NONE',  ( 11.00045714400293306, 20.20239058357963913, -215.1666500215986275 ) ) ;
#11367=CARTESIAN_POINT ( 'NONE',  ( 0.9169988354999972779, 20.59043933275470550, -235.2854195559275752 ) ) ;
#11368=CARTESIAN_POINT ( 'NONE',  ( 26.82025090637478115, -4.850230565203020205, -219.1860060474940042 ) ) ;
#11369=CARTESIAN_POINT ( 'NONE',  ( -2.772442535524381579, 13.75675912271027457, -228.9770533867650215 ) ) ;
#11373=CARTESIAN_POINT ( 'NONE',  ( -6.415689407129693045, 29.32186846096819011, -228.3852515614991887 ) ) ;
#11374=CARTESIAN_POINT ( 'NONE',  ( -14.58670098223046629, 7.239570004716886942, -229.3284954533748135 ) ) ;
#11375=CARTESIAN_POINT ( 'NONE',  ( -17.65835845419170624, 22.55329142274348442, -231.2673511165784532 ) ) ;
#11376=CARTESIAN_POINT ( 'NONE',  ( 23.04897566969193079, 17.95862962700741861, -223.6438515760422661 ) ) ;
#11377=CARTESIAN_POINT ( 'NONE',  ( 8.829458998963966465, 22.90677303676718779, -219.2026791561175685 ) ) ;
#11379=CARTESIAN_POINT ( 'NONE',  ( 12.94599882983645145, 15.82237817288049442, -219.3332542656393116 ) ) ;
#11380=CARTESIAN_POINT ( 'NONE',  ( -16.75313578746775889, -14.38352658620038937, -216.6304878158699978 ) ) ;
#11381=CARTESIAN_POINT ( 'NONE',  ( 15.61962121506769385, 4.525360868525488911, -229.0684696061408090 ) ) ;
#11382=CARTESIAN_POINT ( 'NONE',  ( -6.532222827695542300, -22.16123078269809099, -233.6760793125601481 ) ) ;
#11384=CARTESIAN_POINT ( 'NONE',  ( -9.627017372966443887, 15.60690227900018279, -218.8878023709062859 ) ) ;
#11386=CARTESIAN_POINT ( 'NONE',  ( 16.43596176044053081, -17.06621466254232544, -232.8418678805942648 ) ) ;
#11387=CARTESIAN_POINT ( 'NONE',  ( 19.13999328532042910, 9.776920959053244431, -216.1190985676915375 ) ) ;
#11388=CARTESIAN_POINT ( 'NONE',  ( -15.51982305277792307, 19.76957551617798359, -231.4018974401358832 ) ) ;
#11389=CARTESIAN_POINT ( 'NONE',  ( -23.68377094563794572, 13.02263794644603578, -215.9752901280847652 ) ) ;
#11390=CARTESIAN_POINT ( 'NONE',  ( -14.27403737459813193, -10.90264666745762057, -220.2309642783388597 ) ) ;
#11391=CARTESIAN_POINT ( 'NONE',  ( -18.93763370444446181, -0.7340653299870684156, -219.7345063954518594 ) ) ;
#11393=CARTESIAN_POINT ( 'NONE',  ( -18.15502857810558268, -5.877683472035677426, -234.3930847616834683 ) ) ;
#11394=CARTESIAN_POINT ( 'NONE',  ( -4.855966894080006035, 26.75753167227873064, -230.1547293463117114 ) ) ;
#11395=CARTESIAN_POINT ( 'NONE',  ( -19.11923763334766946, 1.257783214997954202, -219.7591028439344711 ) ) ;
#11396=CARTESIAN_POINT ( 'NONE',  ( -9.679547659771646551, 14.60131434979866505, -230.4338124916943968 ) ) ;
#11397=CARTESIAN_POINT ( 'NONE',  ( 3.889974896201825239, 13.98719620150063214, -218.1465764473210527 ) ) ;
#11399=CARTESIAN_POINT ( 'NONE',  ( -4.075588186332946172, -27.83231707117609588, -229.7735430035053810 ) ) ;
#11401=CARTESIAN_POINT ( 'NONE',  ( -1.434166139689934338, -16.90223958437590213, -219.9603817157532433 ) ) ;
#11402=CARTESIAN_POINT ( 'NONE',  ( -31.84745724608465522, 5.474219582435353004, -224.7210333253351564 ) ) ;
#11403=CARTESIAN_POINT ( 'NONE',  ( 13.04434844185555420, -10.19049307777131297, -230.8679447648462713 ) ) ;
#11404=CARTESIAN_POINT ( 'NONE',  ( 23.45680152528306550, 2.072154465955917235, -232.7243927205664704 ) ) ;
#11405=CARTESIAN_POINT ( 'NONE',  ( -6.870552667427666904, -18.85419487977974029, -216.2130481585807047 ) ) ;
#11406=CARTESIAN_POINT ( 'NONE',  ( 4.044213993247089967, 16.45246633354041421, -227.9255899743332918 ) ) ;
#11408=CARTESIAN_POINT ( 'NONE',  ( -15.05930145804884290, 24.78193219970826533, -223.0510781988847953 ) ) ;
#11409=CARTESIAN_POINT ( 'NONE',  ( 12.10245006109274080, 26.02147364279441888, -220.6079829738538649 ) ) ;
#11410=CARTESIAN_POINT ( 'NONE',  ( 9.575488824002899690, 13.89846378187365694, -220.1158735840035945 ) ) ;
#11411=CARTESIAN_POINT ( 'NONE',  ( 11.58852274881379962, -8.803378160360782800, -231.6724139265004965 ) ) ;
#11412=CARTESIAN_POINT ( 'NONE',  ( 8.554868430186942874, 10.42313681336814568, -223.0114508542762621 ) ) ;
#11413=CARTESIAN_POINT ( 'NONE',  ( -13.91323058514953637, 8.006348396443080162, -225.5064972756604220 ) ) ;
#11414=CARTESIAN_POINT ( 'NONE',  ( -3.515149843921121509, -20.22121776728782550, -231.9652171757311123 ) ) ;
#11417=ADVANCED_FACE ( 'NONE', ( #191 ), #12330, .F. ) ;
#11418=CARTESIAN_POINT ( 'NONE',  ( 15.87442104186276381, 8.674488492264579520, -230.9702037640878416 ) ) ;
#11419=CARTESIAN_POINT ( 'NONE',  ( 19.11859169356911536, -17.02155004481861411, -230.1485466288596911 ) ) ;
#11421=CARTESIAN_POINT ( 'NONE',  ( -3.734153817218577309, -19.72686645808614614, -233.9207428641194610 ) ) ;
#11423=CARTESIAN_POINT ( 'NONE',  ( -2.808235066048971440, 30.42019778760651150, -222.6481917607299295 ) ) ;
#11424=CARTESIAN_POINT ( 'NONE',  ( -0.6224962293416278492, 14.12372964796689701, -218.2103911528446645 ) ) ;
#11426=CARTESIAN_POINT ( 'NONE',  ( -3.082945806077231676, 30.69897765966285874, -224.2387254578930822 ) ) ;
#11427=CARTESIAN_POINT ( 'NONE',  ( 21.75737151495774313, -2.205713500382427750, -233.2756072794337285 ) ) ;
#11430=CARTESIAN_POINT ( 'NONE',  ( 4.603870848087811218, 30.13529352683433515, -225.9623629403671430 ) ) ;
#11431=CARTESIAN_POINT ( 'NONE',  ( -1.821616882984092411, -20.20372127477041246, -234.2708619787750308 ) ) ;
#11432=CARTESIAN_POINT ( 'NONE',  ( 24.96294718070021901, -13.86220829677249178, -229.4442241490162075 ) ) ;
#11433=CARTESIAN_POINT ( 'NONE',  ( -4.104500432947460808, 15.73223271406093460, -218.0734292856946297 ) ) ;
#11434=CARTESIAN_POINT ( 'NONE',  ( 21.43345597994050777, 2.294722475943265838, -232.7243927205661294 ) ) ;
#11435=CARTESIAN_POINT ( 'NONE',  ( 1.719513778997906694, 15.52930330544231730, -222.3959083836286368 ) ) ;
#11437=CARTESIAN_POINT ( 'NONE',  ( 19.79854089336508594, 4.557290221971136646, -217.3342919181881143 ) ) ;
#11438=CARTESIAN_POINT ( 'NONE',  ( -15.48718561803335625, -8.207282836869444154, -229.3046138068065147 ) ) ;
#11440=CARTESIAN_POINT ( 'NONE',  ( -18.74633356284308761, 11.17209001323738704, -217.5809474206552068 ) ) ;
#11441=CARTESIAN_POINT ( 'NONE',  ( 3.160467108836292116, 14.95099014189016629, -228.9242958482614370 ) ) ;
#11442=CARTESIAN_POINT ( 'NONE',  ( -1.806671251568986669, 13.52068930966770388, -228.3567401718105430 ) ) ;
#11444=CARTESIAN_POINT ( 'NONE',  ( -24.05661684749028240, -8.720095227435134433, -219.0096885115910084 ) ) ;
#11445=CARTESIAN_POINT ( 'NONE',  ( 13.80743592543072396, -3.637675435010108906E-12, -228.0000000000000568 ) ) ;
#11447=CARTESIAN_POINT ( 'NONE',  ( -12.90983082593748676, 14.84936372681532823, -233.8009687022269532 ) ) ;
#11448=CARTESIAN_POINT ( 'NONE',  ( -3.786803964513834941, -14.74062382431161566, -229.2965385003435586 ) ) ;
#11449=CARTESIAN_POINT ( 'NONE',  ( 15.35712710306588846, 1.253371448057428283, -227.7275853420972567 ) ) ;
#11450=CARTESIAN_POINT ( 'NONE',  ( 9.333020543840051531, 16.91085096921651143, -217.7308990335875762 ) ) ;
#11453=CARTESIAN_POINT ( 'NONE',  ( -19.98042543492610079, 23.51949599776966693, -226.6701036947414138 ) ) ;
#11454=CARTESIAN_POINT ( 'NONE',  ( 25.60482246989237609, 8.614967517510873307, -219.3103232513597618 ) ) ;
#11458=CARTESIAN_POINT ( 'NONE',  ( -23.67094103897667523, 1.103242709927489740, -215.1660654633311935 ) ) ;
#11459=CARTESIAN_POINT ( 'NONE',  ( -24.92024473536680773, -13.74570206812420103, -220.1598944320903115 ) ) ;
#11460=ADVANCED_FACE ( 'NONE', ( #10133 ), #15322, .F. ) ;
#11462=CARTESIAN_POINT ( 'NONE',  ( -13.17897211815351000, 23.48099580033777301, -217.3415693533541173 ) ) ;
#11463=CARTESIAN_POINT ( 'NONE',  ( 11.42868579270797369, -5.440147491673143598, -220.7688621915004603 ) ) ;
#11464=CARTESIAN_POINT ( 'NONE',  ( 29.17814965709308694, -1.309718763918959139, -225.2029557489520926 ) ) ;
#11465=CARTESIAN_POINT ( 'NONE',  ( -22.38347148959098121, 12.58966534755613687, -218.4978713241202399 ) ) ;
#11466=CARTESIAN_POINT ( 'NONE',  ( -21.48978835671764287, 1.062155088816892468, -219.0000000007146355 ) ) ;
#11467=CARTESIAN_POINT ( 'NONE',  ( 15.70200226922815290, 22.14006925444000018, -227.8255507828836244 ) ) ;
#11469=CARTESIAN_POINT ( 'NONE',  ( -0.6911605129178206575, -19.14003671809244267, -232.0914249810984131 ) ) ;
#11471=CARTESIAN_POINT ( 'NONE',  ( -12.61443312487471324, 8.399394471292156439, -217.5740162615319093 ) ) ;
#11472=CARTESIAN_POINT ( 'NONE',  ( 12.99334571784053338, 27.47142594410712846, -219.5003755906066658 ) ) ;
#11473=CARTESIAN_POINT ( 'NONE',  ( 3.672031556878595282, 11.54613252248376831, -227.4694100414545801 ) ) ;
#11474=CARTESIAN_POINT ( 'NONE',  ( 23.44453178257692727, -8.594063734448958769, -231.6993511358095361 ) ) ;
#11476=CARTESIAN_POINT ( 'NONE',  ( -3.501680520304516264, 14.31538576447642264, -219.8967178229432307 ) ) ;
#11477=CARTESIAN_POINT ( 'NONE',  ( -13.93333636822611155, 3.327141996558931947, -221.4468162587888287 ) ) ;
#11478=CARTESIAN_POINT ( 'NONE',  ( 18.65058977333779211, 24.40868228550881014, -219.3406275662563303 ) ) ;
#11479=CARTESIAN_POINT ( 'NONE',  ( -15.10760069511485604, 3.026516874529453283, -224.5685390982118861 ) ) ;
#11480=CARTESIAN_POINT ( 'NONE',  ( -19.25929423112888017, 9.818144317380269825, -216.1837936240308409 ) ) ;
#11481=CARTESIAN_POINT ( 'NONE',  ( 28.51464931495100785, 5.422321182929326966, -223.8116416110474347 ) ) ;
#11482=CARTESIAN_POINT ( 'NONE',  ( 7.487569386194327770, 15.49107591903592862, -229.0624668269501001 ) ) ;
#11485=CARTESIAN_POINT ( 'NONE',  ( 14.72046356508972309, 21.23077830076469041, -229.4562045376679578 ) ) ;
#11486=CARTESIAN_POINT ( 'NONE',  ( -13.21314811618155716, -9.038438575223175064, -230.6430079410957603 ) ) ;
#11487=CARTESIAN_POINT ( 'NONE',  ( 14.63113973005795643, 4.926264598692385199, -222.4866305912601945 ) ) ;
#11488=CARTESIAN_POINT ( 'NONE',  ( -3.482364789216947809, -21.46714584935086023, -216.0234696677019883 ) ) ;
#11490=CARTESIAN_POINT ( 'NONE',  ( -12.67219131930435694, 19.52425521811199971, -218.0046184995277372 ) ) ;
#11492=CARTESIAN_POINT ( 'NONE',  ( 10.73531068932428667, -10.59494929936097307, -229.0901643129046192 ) ) ;
#11493=CARTESIAN_POINT ( 'NONE',  ( 12.63974878616558328, 15.03448928898568759, -231.7036488814491406 ) ) ;
#11494=CARTESIAN_POINT ( 'NONE',  ( -10.70754874174748039, 23.84972878377777405, -230.7991598016655246 ) ) ;
#11495=CARTESIAN_POINT ( 'NONE',  ( -11.89542918462869103, -0.2773029175206048191, -224.4556830488584467 ) ) ;
#11496=CARTESIAN_POINT ( 'NONE',  ( -22.37826137345437871, -13.90312800710061047, -229.3506127454622572 ) ) ;
#11497=CARTESIAN_POINT ( 'NONE',  ( 27.08260752785270853, 4.114838227474355570, -232.2882281786467331 ) ) ;
#11499=CARTESIAN_POINT ( 'NONE',  ( -14.27185570462694919, -0.4134134650712557035, -229.5903738612280449 ) ) ;
#11500=CARTESIAN_POINT ( 'NONE',  ( 10.70175380652492336, 7.370128018021000038, -224.3479584370086286 ) ) ;
#11501=CARTESIAN_POINT ( 'NONE',  ( 14.33191776452776622, 5.147404080619256916, -219.0172570056664938 ) ) ;
#11502=CARTESIAN_POINT ( 'NONE',  ( 2.471991688031208945, 13.88348721647344419, -230.6707754746932437 ) ) ;
#11504=CARTESIAN_POINT ( 'NONE',  ( 17.10545320562996352, 22.53742678899184781, -232.4605876935045785 ) ) ;
#11505=CARTESIAN_POINT ( 'NONE',  ( 1.672997396509183110, -28.78979777605457713, -223.2908548649682814 ) ) ;
#11507=CARTESIAN_POINT ( 'NONE',  ( 7.074707374710634156, -26.72731565888815553, -229.5909540767539738 ) ) ;
#11508=CARTESIAN_POINT ( 'NONE',  ( -9.503027668167838726, 6.959046566381404730, -225.7241663910276941 ) ) ;
#11509=CARTESIAN_POINT ( 'NONE',  ( 13.28406271702445274, -5.237238614233280742, -225.2640488721434622 ) ) ;
#11510=CARTESIAN_POINT ( 'NONE',  ( -25.42089018817326007, -6.263968923056941307, -218.6542964065910439 ) ) ;
#11511=CARTESIAN_POINT ( 'NONE',  ( -12.44777057840899559, -8.577008958641105352, -229.4809580173677830 ) ) ;
#11512=CARTESIAN_POINT ( 'NONE',  ( 8.645835506124264214, 12.38899589144949687, -223.4673650485651990 ) ) ;
#11513=CARTESIAN_POINT ( 'NONE',  ( -14.01966324001334385, 10.60695606488527964, -217.6333332521996340 ) ) ;
#11514=CARTESIAN_POINT ( 'NONE',  ( 19.13999328532042910, 9.776920959053244431, -216.1190985676915375 ) ) ;
#11515=CARTESIAN_POINT ( 'NONE',  ( 2.008896548638861024, 20.64812324442097591, -233.5818019448501843 ) ) ;
#11516=CARTESIAN_POINT ( 'NONE',  ( 12.55473222622303986, 11.30320364856893001, -218.8964119182764989 ) ) ;
#11517=CARTESIAN_POINT ( 'NONE',  ( 10.88154471369483112, -8.002597937117323923, -230.2267818776996080 ) ) ;
#11518=CARTESIAN_POINT ( 'NONE',  ( 12.81769551943392393, 4.437328497131001193, -221.7762769673541072 ) ) ;
#11519=CARTESIAN_POINT ( 'NONE',  ( -2.508488193221233953, 16.03207605874066033, -217.8880952293912969 ) ) ;
#11520=EDGE_CURVE ( 'NONE', #7856, #161, #18114, .T. ) ;
#11521=CARTESIAN_POINT ( 'NONE',  ( -18.96646980336054611, -22.16549408654085696, -227.7928771762007329 ) ) ;
#11522=CARTESIAN_POINT ( 'NONE',  ( -14.29986196492902550, 0.06805469746732484282, -227.4167624117703213 ) ) ;
#11524=CARTESIAN_POINT ( 'NONE',  ( 17.00168025137501004, 6.212099629982537508, -219.0548246536471595 ) ) ;
#11525=CARTESIAN_POINT ( 'NONE',  ( 23.84477361619719105, -14.51625201957343592, -224.2863126538025540 ) ) ;
#11526=CARTESIAN_POINT ( 'NONE',  ( -21.66803296057637951, 19.04503900041684616, -222.6603677762044526 ) ) ;
#11527=CARTESIAN_POINT ( 'NONE',  ( -5.525229149912007642, -13.32411127922494742, -220.4018445532201440 ) ) ;
#11528=CARTESIAN_POINT ( 'NONE',  ( 20.76808360334631232, 5.412616674732960931, -234.1222385626545304 ) ) ;
#11529=CARTESIAN_POINT ( 'NONE',  ( 4.849508625227819003, 24.02665844953846275, -214.9607406399067315 ) ) ;
#11531=CARTESIAN_POINT ( 'NONE',  ( -11.26857159993117996, 28.96895336474501192, -225.6039696848669678 ) ) ;
#11532=CARTESIAN_POINT ( 'NONE',  ( -21.94776718874828347, -0.4748437386657700099, -216.1214812709574176 ) ) ;
#11535=CARTESIAN_POINT ( 'NONE',  ( -3.755296588130283553, 23.77975947300719284, -233.7323173085780752 ) ) ;
#11536=CARTESIAN_POINT ( 'NONE',  ( -10.76360437932642533, -14.08317586560949408, -234.4387784497120890 ) ) ;
#11537=CARTESIAN_POINT ( 'NONE',  ( 7.088126259304779353, -19.25156530781288566, -233.7785425911077937 ) ) ;
#11538=CARTESIAN_POINT ( 'NONE',  ( 15.02813183614916781, -2.406088413402002413, -227.6705652927927872 ) ) ;
#11539=CARTESIAN_POINT ( 'NONE',  ( -10.52776196018457711, 13.57482816453351937, -219.2327734183297423 ) ) ;
#11540=CARTESIAN_POINT ( 'NONE',  ( 16.01130065545721592, 20.79417322911648114, -220.9619135886794652 ) ) ;
#11541=CARTESIAN_POINT ( 'NONE',  ( 15.34286276367735979, 1.557318373440422565, -222.4358706187587416 ) ) ;
#11542=CARTESIAN_POINT ( 'NONE',  ( -13.71158422780231056, 12.21432067443984693, -232.9166272955793033 ) ) ;
#11543=CARTESIAN_POINT ( 'NONE',  ( -20.58582428111024853, -15.24952116403520463, -229.8418230779359135 ) ) ;
#11546=CARTESIAN_POINT ( 'NONE',  ( -4.334015487506815312, 18.19775486192265390, -231.4387392399519285 ) ) ;
#11547=CARTESIAN_POINT ( 'NONE',  ( 14.00715608756928532, 4.299235856235253728, -230.2440235370780215 ) ) ;
#11548=CARTESIAN_POINT ( 'NONE',  ( -2.047892494109819328, 12.88402507277750786, -223.5104301352110951 ) ) ;
#11549=CARTESIAN_POINT ( 'NONE',  ( 20.33239098169031323, -9.013719117183370599, -216.4483480702011775 ) ) ;
#11552=CARTESIAN_POINT ( 'NONE',  ( -14.83974801774860630, 13.71714848582103485, -216.0935642439352762 ) ) ;
#11553=CARTESIAN_POINT ( 'NONE',  ( -8.507187218596966360, -16.39771659352221533, -216.5221606441677977 ) ) ;
#11555=CARTESIAN_POINT ( 'NONE',  ( 9.586902571418640662, 24.43292817174309661, -231.9968623198229807 ) ) ;
#11558=CARTESIAN_POINT ( 'NONE',  ( -16.28135616697389310, 20.98764039357472200, -216.9434553755565958 ) ) ;
#11559=CARTESIAN_POINT ( 'NONE',  ( 15.21408433160105034, 3.021350230896802103, -222.3056493717910769 ) ) ;
#11562=CARTESIAN_POINT ( 'NONE',  ( 27.75679124201660741, 4.911524026080384075, -221.4430403652340829 ) ) ;
#11563=CARTESIAN_POINT ( 'NONE',  ( -20.26851768784797869, -0.8260594303982465858, -217.1279713726092098 ) ) ;
#11564=CARTESIAN_POINT ( 'NONE',  ( 22.26090851979669338, -3.689523054771738586, -218.9825289563843285 ) ) ;
#11565=CARTESIAN_POINT ( 'NONE',  ( -13.72709560065558421, -5.132649126379569715, -227.9317987811764965 ) ) ;
#11569=CARTESIAN_POINT ( 'NONE',  ( 4.238595127209166868, 26.19205419861516404, -230.1142052665570077 ) ) ;
#11570=CARTESIAN_POINT ( 'NONE',  ( 10.42186625103445152, -25.39807580958450473, -217.7675295214572202 ) ) ;
#11571=CARTESIAN_POINT ( 'NONE',  ( 15.10937218716165020, -26.44221868192832758, -222.7999243300199907 ) ) ;
#11572=CARTESIAN_POINT ( 'NONE',  ( -25.44919589272258520, 4.740781954932180575, -232.0725131810460766 ) ) ;
#11573=CARTESIAN_POINT ( 'NONE',  ( 20.05202556141620107, 8.012988804822112954, -215.8722494878839200 ) ) ;
#11574=CARTESIAN_POINT ( 'NONE',  ( 28.46362550855882745, 7.392895870364313282, -223.4682258299149566 ) ) ;
#11576=CARTESIAN_POINT ( 'NONE',  ( 3.436191426816104233, -15.97976940388950773, -231.4631329546418499 ) ) ;
#11578=CARTESIAN_POINT ( 'NONE',  ( -29.15345109632842124, 14.07532767497844262, -225.0972140442887621 ) ) ;
#11580=CARTESIAN_POINT ( 'NONE',  ( 20.05374812456133782, 24.17492691056345677, -223.1494843338164458 ) ) ;
#11581=CARTESIAN_POINT ( 'NONE',  ( 4.024086222410633518, 12.48004227094270746, -230.0177668608922374 ) ) ;
#11582=CARTESIAN_POINT ( 'NONE',  ( 14.12786214016513675, -4.771276416369937046, -223.8547069812204029 ) ) ;
#11583=CARTESIAN_POINT ( 'NONE',  ( -7.395406416482832590, 12.93623984139929739, -219.2606224730616873 ) ) ;
#11584=CARTESIAN_POINT ( 'NONE',  ( -13.65925618638770800, 3.289586759644148817, -222.1579143493116533 ) ) ;
#11587=CARTESIAN_POINT ( 'NONE',  ( 5.030854775705693172, 19.94152319263364603, -234.9034581965229336 ) ) ;
#11588=CARTESIAN_POINT ( 'NONE',  ( -22.18165477997343871, 9.502253276305026475, -218.0070055737419636 ) ) ;
#11589=CARTESIAN_POINT ( 'NONE',  ( -6.201839134465864767, 11.37481922992157379, -223.7040893475979146 ) ) ;
#11591=CARTESIAN_POINT ( 'NONE',  ( 3.746955526231565248, 25.82691596581962656, -220.7780764774678062 ) ) ;
#11592=CARTESIAN_POINT ( 'NONE',  ( 28.36095019830170472, -8.296631283839911220, -225.2861439608085448 ) ) ;
#11595=CARTESIAN_POINT ( 'NONE',  ( 22.02796522526679723, 16.41909032291435366, -220.1590600991317217 ) ) ;
#11596=CARTESIAN_POINT ( 'NONE',  ( -11.58793217866213787, -13.88438693436061477, -219.4860661588769801 ) ) ;
#11600=CARTESIAN_POINT ( 'NONE',  ( -8.857704405076667342, 24.20848540845601704, -218.8859504303524091 ) ) ;
#11602=CARTESIAN_POINT ( 'NONE',  ( 17.93010821528303822, -10.80507700282924688, -233.3968735006674251 ) ) ;
#11603=CARTESIAN_POINT ( 'NONE',  ( 13.17768061945195157, 6.810183613937965674, -219.8302315341053657 ) ) ;
#11604=CARTESIAN_POINT ( 'NONE',  ( -4.334015487506815312, 18.19775486192265390, -231.4387392399519285 ) ) ;
#11605=CARTESIAN_POINT ( 'NONE',  ( -9.290933312444883185, 29.15551353946876745, -225.8551562993724247 ) ) ;
#11607=CARTESIAN_POINT ( 'NONE',  ( -16.47483915600249205, -3.991485801086211538, -222.0851216934102297 ) ) ;
#11608=CARTESIAN_POINT ( 'NONE',  ( -21.28804099221702018, -0.9277163183344186992, -219.0000000002572733 ) ) ;
#11610=CARTESIAN_POINT ( 'NONE',  ( -30.26911233660276679, -7.575179034252494503, -222.6017624672529109 ) ) ;
#11611=CARTESIAN_POINT ( 'NONE',  ( 22.20554449732931346, 18.01468431515759860, -218.9348803756412849 ) ) ;
#11612=CARTESIAN_POINT ( 'NONE',  ( -27.28038240442402440, 5.683827137705129040, -226.0726697751923382 ) ) ;
#11614=CARTESIAN_POINT ( 'NONE',  ( -4.974038791218384326, 28.61915055369004079, -219.5057940952933961 ) ) ;
#11615=CARTESIAN_POINT ( 'NONE',  ( 15.33651282626308010, 7.807290788239344970, -218.6940806506825652 ) ) ;
#11616=VERTEX_POINT ( 'NONE', #18901 ) ;
#11617=CARTESIAN_POINT ( 'NONE',  ( -9.514686225151438137, -9.899715435889788751, -219.6589915062491229 ) ) ;
#11619=CARTESIAN_POINT ( 'NONE',  ( -13.02663300398358892, -17.15584419188240162, -232.5492131852532793 ) ) ;
#11621=CARTESIAN_POINT ( 'NONE',  ( -13.55637112341987383, 4.614880311503475774, -231.8130385267184010 ) ) ;
#11622=CARTESIAN_POINT ( 'NONE',  ( 8.649266908999912573, -10.50942778440553482, -226.4415026780416440 ) ) ;
#11623=CARTESIAN_POINT ( 'NONE',  ( 23.77009720158773831, -0.5966687509537305090, -216.6384684467892043 ) ) ;
#11624=CARTESIAN_POINT ( 'NONE',  ( -21.80830016239255897, -4.781675611938959847, -217.4666014280278148 ) ) ;
#11625=CARTESIAN_POINT ( 'NONE',  ( 20.85755584069816493, 20.53615333921957742, -227.2010381488614996 ) ) ;
#11627=CARTESIAN_POINT ( 'NONE',  ( -27.40681729237160269, 15.04232492504307572, -225.3323746796125704 ) ) ;
#11628=CARTESIAN_POINT ( 'NONE',  ( 16.97369223523349646, 15.19068754808448851, -217.0779026324121332 ) ) ;
#11629=CARTESIAN_POINT ( 'NONE',  ( 12.85408565574548412, 7.821283853063205171, -223.1248833997948111 ) ) ;
#11630=CARTESIAN_POINT ( 'NONE',  ( 12.11771628698343051, 17.56545729485151952, -218.0322663566023493 ) ) ;
#11631=CARTESIAN_POINT ( 'NONE',  ( 11.14866046433140490, -17.10865642060806024, -235.2771047445726822 ) ) ;
#11634=CARTESIAN_POINT ( 'NONE',  ( -13.01542355754912172, 26.77630951171455820, -225.1545229496516356 ) ) ;
#11637=CARTESIAN_POINT ( 'NONE',  ( 14.73698509926073186, 4.443590625350892331, -227.4062002049096236 ) ) ;
#11638=CARTESIAN_POINT ( 'NONE',  ( 7.357019007885960526, -24.37006613449481662, -217.4041786725384782 ) ) ;
#11639=CARTESIAN_POINT ( 'NONE',  ( -18.74633356284308761, 11.17209001323738704, -217.5809474206552068 ) ) ;
#11640=CARTESIAN_POINT ( 'NONE',  ( -3.996294969088721505, 28.80481464818193515, -222.8623509149411746 ) ) ;
#11641=CARTESIAN_POINT ( 'NONE',  ( -13.33530847390368024, -5.065163879519744228, -226.5386329521395226 ) ) ;
#11642=CARTESIAN_POINT ( 'NONE',  ( 14.50618777373884960, 4.375057440872940795, -230.8807389798650433 ) ) ;
#11643=CARTESIAN_POINT ( 'NONE',  ( 7.803634760976553508, 10.78293796201124266, -229.6314106675118865 ) ) ;
#11645=CARTESIAN_POINT ( 'NONE',  ( 1.382955251742491898, 16.46353944795171032, -231.7743150979565030 ) ) ;
#11646=CARTESIAN_POINT ( 'NONE',  ( 13.86395146404758982, -8.823451364178625411, -228.3963352256065491 ) ) ;
#11650=CARTESIAN_POINT ( 'NONE',  ( 4.389496648589924277, 14.47660514356954131, -220.6151178996808540 ) ) ;
#11651=CARTESIAN_POINT ( 'NONE',  ( -3.739406429132753562, -13.42303118918103344, -219.1969888661882635 ) ) ;
#11652=CARTESIAN_POINT ( 'NONE',  ( 15.34510829589250491, -24.56813251781886009, -230.1307231235174982 ) ) ;
#11653=CARTESIAN_POINT ( 'NONE',  ( 10.40291689048662782, -13.87512507945592333, -231.9656913702303029 ) ) ;
#11654=CARTESIAN_POINT ( 'NONE',  ( -19.01002492504315811, 19.85266905124972681, -219.0021410556803687 ) ) ;
#11655=CARTESIAN_POINT ( 'NONE',  ( 5.791579991237209235, 15.48299465423324861, -228.0203551130359472 ) ) ;
#11656=CARTESIAN_POINT ( 'NONE',  ( -15.23434562258889891, -0.4010941804143903222, -220.4743703065900036 ) ) ;
#11657=CARTESIAN_POINT ( 'NONE',  ( -12.39654240422350462, 9.886262337642440556, -219.1620329226848014 ) ) ;
#11658=CARTESIAN_POINT ( 'NONE',  ( -16.29786170208491924, -8.453292648900102790, -230.0691174225123632 ) ) ;
#11660=CARTESIAN_POINT ( 'NONE',  ( -7.873497077133136735, 15.44270125396616677, -230.2562282217168672 ) ) ;
#11661=CARTESIAN_POINT ( 'NONE',  ( 21.72366288329714834, 2.385777479048636351, -215.9150265590827757 ) ) ;
#11662=CARTESIAN_POINT ( 'NONE',  ( -5.727886109716582297, 15.25217619989539486, -230.5419623196804650 ) ) ;
#11663=CARTESIAN_POINT ( 'NONE',  ( 13.09169075717699293, -6.869491136113572871, -220.8313809912125691 ) ) ;
#11666=CARTESIAN_POINT ( 'NONE',  ( -15.82069055112642353, 8.315535108674763976, -217.2800172218543935 ) ) ;
#11667=CARTESIAN_POINT ( 'NONE',  ( -26.63259355655987548, -7.256793811979244779, -216.2488627322786101 ) ) ;
#11670=CARTESIAN_POINT ( 'NONE',  ( 7.762960416026701616, 12.60702317161859121, -221.9096828323375235 ) ) ;
#11673=CARTESIAN_POINT ( 'NONE',  ( 13.36656406724190305, -19.73987914515934960, -233.3798509643240209 ) ) ;
#11675=CARTESIAN_POINT ( 'NONE',  ( -16.63766460830045091, 5.158675778507696208, -232.1659425527909093 ) ) ;
#11676=CARTESIAN_POINT ( 'NONE',  ( -14.30586181932858914, 18.69563132175512266, -215.8217153853723573 ) ) ;
#11677=CARTESIAN_POINT ( 'NONE',  ( 22.44730228620155899, 3.608729811217749717, -232.0798239124179645 ) ) ;
#11678=CARTESIAN_POINT ( 'NONE',  ( -6.507186921339367380, -21.94905981650347826, -217.8194053188079238 ) ) ;
#11680=CARTESIAN_POINT ( 'NONE',  ( 16.00819137755116373, 4.595691552992191120, -229.5669508871464757 ) ) ;
#11682=CARTESIAN_POINT ( 'NONE',  ( 22.49864633775863609, -6.670857247392108391, -230.7634588385486438 ) ) ;
#11683=CARTESIAN_POINT ( 'NONE',  ( -24.15031621174628285, -13.05338392360020627, -219.0842748323915714 ) ) ;
#11686=CARTESIAN_POINT ( 'NONE',  ( 5.466128392039544259, 27.94759090250835243, -223.5617905851570981 ) ) ;
#11687=CARTESIAN_POINT ( 'NONE',  ( 5.503098680704820111, -17.53359096179937993, -217.0817822229213618 ) ) ;
#11689=CARTESIAN_POINT ( 'NONE',  ( 10.10435529162921853, -13.32996982371095918, -231.5224098423250894 ) ) ;
#11691=COLOUR_RGB ( '', 0.09019608, 0.27058824, 0.51372549) ;
#11692=CARTESIAN_POINT ( 'NONE',  ( -16.57767831947938575, 23.50485984366324388, -222.7977068309636763 ) ) ;
#11693=CARTESIAN_POINT ( 'NONE',  ( -17.64438593497130370, 2.824953307685432069, -229.4443205246391813 ) ) ;
#11694=CARTESIAN_POINT ( 'NONE',  ( 14.04819512851487673, 6.831178966487911453, -222.6676118107292552 ) ) ;
#11696=CARTESIAN_POINT ( 'NONE',  ( -13.60885102855131201, -21.92822159330905762, -220.4851091041354607 ) ) ;
#11698=CARTESIAN_POINT ( 'NONE',  ( -26.12939716039095117, 11.33146045174629357, -233.1192402782019997 ) ) ;
#11699=CARTESIAN_POINT ( 'NONE',  ( 8.730612144237051453, 13.93563980088501886, -217.1627566045470132 ) ) ;
#11700=CARTESIAN_POINT ( 'NONE',  ( 11.43327405580198608, -14.46863304034511799, -220.4355838810013495 ) ) ;
#11701=CARTESIAN_POINT ( 'NONE',  ( 5.343558017910363667, 26.29639771561252459, -218.1010331760174665 ) ) ;
#11702=CARTESIAN_POINT ( 'NONE',  ( -28.59157645096996347, 5.137867505054540374, -220.4667042235044505 ) ) ;
#11703=CARTESIAN_POINT ( 'NONE',  ( 5.179557175392591972, 10.46258103618983881, -224.6216839350439614 ) ) ;
#11705=CARTESIAN_POINT ( 'NONE',  ( -21.93223149637851677, 1.726402211042445067, -231.1052103444381203 ) ) ;
#11706=CARTESIAN_POINT ( 'NONE',  ( -14.73016414256368911, 22.23431809695627237, -217.1425123644553707 ) ) ;
#11707=DIRECTION ( 'NONE',  ( 1.000000000000000000, 0.000000000000000000, 0.000000000000000000 ) ) ;
#11708=CARTESIAN_POINT ( 'NONE',  ( 2.021807401899061496, 24.17554150923399092, -230.4042646614662146 ) ) ;
#11709=FACE_OUTER_BOUND ( 'NONE', #10199, .T. ) ;
#11711=CARTESIAN_POINT ( 'NONE',  ( -26.22594988380878789, -0.1068133454905619700, -219.1167922977186322 ) ) ;
#11712=CARTESIAN_POINT ( 'NONE',  ( 16.07305932912010960, 0.9253679043337685872, -229.0409936706996064 ) ) ;
#11713=CARTESIAN_POINT ( 'NONE',  ( -13.39502153392024475, -9.880902914596246589, -222.0112808355889342 ) ) ;
#11716=CARTESIAN_POINT ( 'NONE',  ( -4.466732464217805898, 19.42663028452474450, -231.9485309169485561 ) ) ;
#11717=CARTESIAN_POINT ( 'NONE',  ( 2.641673488600395636, -17.65289918763021149, -219.1873688300129288 ) ) ;
#11718=CARTESIAN_POINT ( 'NONE',  ( 16.97369223523349646, 15.19068754808448851, -217.0779026324121332 ) ) ;
#11719=CARTESIAN_POINT ( 'NONE',  ( -7.375127652145912371, 13.01042140126078195, -223.9959097520547004 ) ) ;
#11720=CARTESIAN_POINT ( 'NONE',  ( -8.653738780971721667, 11.12943719949617893, -219.7525355316396087 ) ) ;
#11722=CARTESIAN_POINT ( 'NONE',  ( 19.51310828881794990, -1.786742129898636344, -215.1201286626718741 ) ) ;
#11724=CARTESIAN_POINT ( 'NONE',  ( 15.85665641241444668, 18.24713744004561988, -217.7195292979064902 ) ) ;
#11726=CARTESIAN_POINT ( 'NONE',  ( -15.10760069511485604, 3.026516874529453283, -224.5685390982118861 ) ) ;
#11727=CARTESIAN_POINT ( 'NONE',  ( -26.70018640714903668, 3.110792036746048428, -228.8761207540193823 ) ) ;
#11729=CARTESIAN_POINT ( 'NONE',  ( -17.70471257751854921, -0.5540196600081067624, -232.9322037287452360 ) ) ;
#11730=CARTESIAN_POINT ( 'NONE',  ( 8.592982993077152187, 10.20906991731218838, -226.0923132092261483 ) ) ;
#11731=CARTESIAN_POINT ( 'NONE',  ( -13.91323058514953637, 8.006348396443080162, -225.5064972756604220 ) ) ;
#11732=CARTESIAN_POINT ( 'NONE',  ( 2.165130313308041288, 31.55305250914585002, -225.6791154433767304 ) ) ;
#11733=CARTESIAN_POINT ( 'NONE',  ( 13.14260364752544596, 5.866423290307341887, -222.7705901084601408 ) ) ;
#11736=CARTESIAN_POINT ( 'NONE',  ( -11.58651333402397476, -12.19597367159924595, -216.5418320517508448 ) ) ;
#11738=CARTESIAN_POINT ( 'NONE',  ( -10.39692419770002552, -10.11462123336039021, -222.6538761800393047 ) ) ;
#11739=CARTESIAN_POINT ( 'NONE',  ( -16.81617677814535128, 0.6259372974186930838, -233.5115673467681745 ) ) ;
#11740=CARTESIAN_POINT ( 'NONE',  ( 10.30328786010431052, -20.08430705480546408, -216.1847100135515802 ) ) ;
#11741=CARTESIAN_POINT ( 'NONE',  ( 13.79223148755288797, -4.990905483784310981, -230.8248327435212559 ) ) ;
#11742=CARTESIAN_POINT ( 'NONE',  ( -28.30937415889876618, -7.921132361018833556, -222.9755670691803857 ) ) ;
#11743=EDGE_CURVE ( 'NONE', #9103, #8796, #21525, .T. ) ;
#11744=CARTESIAN_POINT ( 'NONE',  ( 21.46274988498219471, 20.25395488059580984, -223.1777011585387243 ) ) ;
#11747=CARTESIAN_POINT ( 'NONE',  ( -25.00745438246740804, 14.90779342625281778, -219.2410538611701156 ) ) ;
#11748=CARTESIAN_POINT ( 'NONE',  ( 20.88350594575732799, 13.65521425050155813, -232.8060468608549911 ) ) ;
#11749=CARTESIAN_POINT ( 'NONE',  ( 7.762960416026701616, 12.60702317161859121, -221.9096828323375235 ) ) ;
#11750=CARTESIAN_POINT ( 'NONE',  ( 10.64798096806036121, 19.48085866535796740, -231.3996658690317361 ) ) ;
#11751=CARTESIAN_POINT ( 'NONE',  ( 21.94513595990333954, -23.27941424421253203, -222.2428713697011631 ) ) ;
#11752=CARTESIAN_POINT ( 'NONE',  ( -5.836418080594380164, 30.19240250712089590, -223.8354869487762357 ) ) ;
#11753=CARTESIAN_POINT ( 'NONE',  ( -29.30406754532526037, 5.063969254119831120, -221.8212091093853076 ) ) ;
#11756=CARTESIAN_POINT ( 'NONE',  ( 7.808093059109005196, -25.57408461116448706, -218.1679985877120487 ) ) ;
#11757=CARTESIAN_POINT ( 'NONE',  ( -12.05423124486310904, 12.38527783110887803, -219.7419643105747014 ) ) ;
#11759=CARTESIAN_POINT ( 'NONE',  ( 4.303123380281038024, 17.66787810618728827, -231.9745698734655832 ) ) ;
#11760=CARTESIAN_POINT ( 'NONE',  ( -22.23616899077527975, -11.51447210886970751, -217.5950109096934568 ) ) ;
#11761=CARTESIAN_POINT ( 'NONE',  ( -26.35007260221545877, 6.140745174321167177, -221.9336216792591188 ) ) ;
#11763=CARTESIAN_POINT ( 'NONE',  ( 17.04685026979186446, 18.05617612716381970, -216.0910122987878310 ) ) ;
#11765=CARTESIAN_POINT ( 'NONE',  ( 0.2389779871941385414, 16.64595486589868045, -218.1658233406367629 ) ) ;
#11766=CARTESIAN_POINT ( 'NONE',  ( 17.47462908134004422, -13.97354901070533906, -218.8807045398700666 ) ) ;
#11767=CARTESIAN_POINT ( 'NONE',  ( 20.07985072697885442, -15.33367264652052953, -217.4666949641080294 ) ) ;
#11769=CARTESIAN_POINT ( 'NONE',  ( 4.543450689403089271, 15.91052110650461771, -218.9437823786444426 ) ) ;
#11770=CARTESIAN_POINT ( 'NONE',  ( -15.94006964721192432, -5.209069452486915885, -233.2212940081757040 ) ) ;
#11771=CARTESIAN_POINT ( 'NONE',  ( -1.778254167844783851, -12.78790610364390012, -225.9413532495922254 ) ) ;
#11772=CARTESIAN_POINT ( 'NONE',  ( 13.47054497134856277, -24.75371201277411615, -218.7687119198782000 ) ) ;
#11773=CARTESIAN_POINT ( 'NONE',  ( -15.33438615632468149, 23.56248205204123991, -229.2747191038674544 ) ) ;
#11774=CARTESIAN_POINT ( 'NONE',  ( 8.539351012053531420, 16.03230746435535181, -220.6282946404833751 ) ) ;
#11775=CARTESIAN_POINT ( 'NONE',  ( -14.68037037322036475, 3.441677802729143920, -220.1396515630443389 ) ) ;
#11776=CARTESIAN_POINT ( 'NONE',  ( -9.982417347796181062, 8.907629238417765549, -225.5124013436514474 ) ) ;
#11777=CARTESIAN_POINT ( 'NONE',  ( -15.17770002056818868, -9.429316640439420638, -220.2566215541993699 ) ) ;
#11779=CARTESIAN_POINT ( 'NONE',  ( -9.233762381136051189, 19.18161952504991419, -232.0796851897838451 ) ) ;
#11780=CARTESIAN_POINT ( 'NONE',  ( 12.25122766587143630, 4.035812653434439845, -225.7709573147497224 ) ) ;
#11781=CARTESIAN_POINT ( 'NONE',  ( 8.373295497769937867, 8.203271496719947820, -226.1884629658694053 ) ) ;
#11782=CARTESIAN_POINT ( 'NONE',  ( 12.44471834243122466, -10.90083019301730083, -219.2211511521849161 ) ) ;
#11785=CARTESIAN_POINT ( 'NONE',  ( -13.55591840520136770, 8.363404288414606924, -231.2690188357804857 ) ) ;
#11786=CARTESIAN_POINT ( 'NONE',  ( -17.53163374842703703, -10.16025041587072764, -214.8411325589202647 ) ) ;
#11788=CARTESIAN_POINT ( 'NONE',  ( 7.639528166734322667, 11.92751229241157596, -224.6077814063189635 ) ) ;
#11790=CARTESIAN_POINT ( 'NONE',  ( 21.39922646226391478, -21.53954253117021977, -224.1701659532164967 ) ) ;
#11791=CARTESIAN_POINT ( 'NONE',  ( -21.93900267957129557, 7.862893636934532360, -233.4951761057262161 ) ) ;
#11792=CARTESIAN_POINT ( 'NONE',  ( -7.752954785937490989, 10.21341112307795385, -225.5135920495299615 ) ) ;
#11793=CARTESIAN_POINT ( 'NONE',  ( 15.57986488780344736, -0.6155558446892130942, -225.2777919203616932 ) ) ;
#11794=CARTESIAN_POINT ( 'NONE',  ( -5.980659577089002532, -19.45286470896024156, -217.9322865582606710 ) ) ;
#11796=CARTESIAN_POINT ( 'NONE',  ( 25.69300549816939494, 5.947472783069708946, -230.6131061331718115 ) ) ;
#11798=CARTESIAN_POINT ( 'NONE',  ( 13.81930941494936782, -14.31252807618095879, -218.6132940872857375 ) ) ;
#11799=CARTESIAN_POINT ( 'NONE',  ( 12.83912001598358898, -2.984904020217645115, -224.6440377188723687 ) ) ;
#11801=CARTESIAN_POINT ( 'NONE',  ( 8.647507700742417924, 16.42978512283924175, -220.3082116258600536 ) ) ;
#11802=CARTESIAN_POINT ( 'NONE',  ( 11.96323484613444599, -17.37820513000257350, -215.5071828020160183 ) ) ;
#11803=CARTESIAN_POINT ( 'NONE',  ( 11.43609017326686050, -13.06727081285745307, -217.8903327850316316 ) ) ;
#11805=CARTESIAN_POINT ( 'NONE',  ( -21.23733589435050817, 17.25275849955597351, -229.9547908233139708 ) ) ;
#11806=CARTESIAN_POINT ( 'NONE',  ( 21.72366288329714834, 2.385777479048636351, -215.9150265590827757 ) ) ;
#11807=CARTESIAN_POINT ( 'NONE',  ( 21.91535456744164279, 7.573568724377624406, -232.0371228855588868 ) ) ;
#11809=CARTESIAN_POINT ( 'NONE',  ( -11.18644257538908526, -20.90776414258732174, -230.8249452324125173 ) ) ;
#11811=CARTESIAN_POINT ( 'NONE',  ( -17.92628912275201003, -0.6090139417824500523, -215.7724435048976943 ) ) ;
#11812=CARTESIAN_POINT ( 'NONE',  ( 8.454338299486085617, 13.28844197278511530, -217.6979371188311632 ) ) ;
#11813=CARTESIAN_POINT ( 'NONE',  ( 20.29455491689504498, -15.47394441642566143, -219.8812143983372778 ) ) ;
#11814=CARTESIAN_POINT ( 'NONE',  ( 8.496844655769807630, 14.66037471857024599, -219.1631158796573118 ) ) ;
#11815=CARTESIAN_POINT ( 'NONE',  ( -20.54164754914381064, 7.122791156791981493, -233.5720402887671980 ) ) ;
#11817=CARTESIAN_POINT ( 'NONE',  ( 18.26039090677515375, 26.14311541888654844, -228.1864986152887127 ) ) ;
#11818=CARTESIAN_POINT ( 'NONE',  ( -26.47320305716024791, 9.675235842009668019, -228.3542180911597654 ) ) ;
#11819=CARTESIAN_POINT ( 'NONE',  ( -2.208416658185406334, 29.10348627872611615, -219.8480645685746424 ) ) ;
#11821=CARTESIAN_POINT ( 'NONE',  ( 0.7326557587344989519, -29.96088689026728602, -229.4725774697800205 ) ) ;
#11822=CARTESIAN_POINT ( 'NONE',  ( 17.00614511541963836, -1.958782916976874233, -219.4638360731791806 ) ) ;
#11825=CARTESIAN_POINT ( 'NONE',  ( -12.36382104905844592, -0.1264132474004772688, -228.0034406263598896 ) ) ;
#11826=CARTESIAN_POINT ( 'NONE',  ( -16.98436007432217920, -11.01716238098750544, -231.0196200964405193 ) ) ;
#11828=CARTESIAN_POINT ( 'NONE',  ( 9.037704487505543227, -20.74919929927824214, -217.6023494967207625 ) ) ;
#11830=CARTESIAN_POINT ( 'NONE',  ( 9.575488824002899690, 13.89846378187365694, -220.1158735840035945 ) ) ;
#11831=CARTESIAN_POINT ( 'NONE',  ( -4.224287562409271501, 29.03635716824519264, -224.1823526280761882 ) ) ;
#11832=CARTESIAN_POINT ( 'NONE',  ( -12.22073052649759184, 14.03927388329973525, -215.9097966823721606 ) ) ;
#11834=CARTESIAN_POINT ( 'NONE',  ( 31.43562455973156844, -0.2326399569828876968, -228.1442589022926484 ) ) ;
#11836=CARTESIAN_POINT ( 'NONE',  ( 10.55627441269396094, 10.31758739525044888, -223.1990319438957613 ) ) ;
#11838=CARTESIAN_POINT ( 'NONE',  ( -21.93223149637851677, 1.726402211042445067, -231.1052103444381203 ) ) ;
#11839=CARTESIAN_POINT ( 'NONE',  ( 16.77642802340811556, -0.6192566135115280535, -218.8326447441449432 ) ) ;
#11840=CARTESIAN_POINT ( 'NONE',  ( -20.69232116990083981, -0.6602618815637216754, -233.8806059993499957 ) ) ;
#11841=CARTESIAN_POINT ( 'NONE',  ( 6.491278574642851851, 13.23281603069746382, -229.0355254242266767 ) ) ;
#11842=CARTESIAN_POINT ( 'NONE',  ( -15.37153448429513602, 5.014568651886798456, -224.5085656291724945 ) ) ;
#11843=CARTESIAN_POINT ( 'NONE',  ( 7.359401564398577733, 15.81697286067417707, -215.8326977948377987 ) ) ;
#11844=CARTESIAN_POINT ( 'NONE',  ( 21.14441169763230732, 12.98245189690719315, -217.0976687089155064 ) ) ;
#11845=CARTESIAN_POINT ( 'NONE',  ( -8.507187218596966360, -16.39771659352221533, -216.5221606441677977 ) ) ;
#11847=CARTESIAN_POINT ( 'NONE',  ( -11.55581979318669639, -19.97716813486601239, -217.5317483122086912 ) ) ;
#11848=CARTESIAN_POINT ( 'NONE',  ( -30.17036082276531772, 5.959165309317525860, -219.4883053239162791 ) ) ;
#11849=CARTESIAN_POINT ( 'NONE',  ( 6.374306683232226156, -13.38367253400339330, -219.9651431149896723 ) ) ;
#11850=CARTESIAN_POINT ( 'NONE',  ( -2.817219543927646175, 14.13981714106644993, -229.6779615865167443 ) ) ;
#11851=CARTESIAN_POINT ( 'NONE',  ( 12.32676726801020450, -8.454629307895981327, -217.7935467833756036 ) ) ;
#11852=CARTESIAN_POINT ( 'NONE',  ( -18.34948365288241590, -1.907751280579004893, -231.5848060246952116 ) ) ;
#11853=CARTESIAN_POINT ( 'NONE',  ( 9.125049424194871861, 12.37796447639467523, -227.2539065556229332 ) ) ;
#11855=CARTESIAN_POINT ( 'NONE',  ( -16.65220264499505376, 11.77543314451157563, -216.3149620944649030 ) ) ;
#11856=CARTESIAN_POINT ( 'NONE',  ( 12.23475091788960434, 6.342242864926500800, -221.9572581868331156 ) ) ;
#11857=CARTESIAN_POINT ( 'NONE',  ( 11.62313423782632782, 11.98467543564608029, -219.7293303032897995 ) ) ;
#11858=CARTESIAN_POINT ( 'NONE',  ( 21.27834046766391651, 19.84195992785746654, -221.8454931627593965 ) ) ;
#11859=CARTESIAN_POINT ( 'NONE',  ( -3.168869516962652622, -26.26615012824360207, -217.0152745877844040 ) ) ;
#11860=CARTESIAN_POINT ( 'NONE',  ( -5.562203253303141359, 12.75725363875033302, -225.3078268727488478 ) ) ;
#11861=CARTESIAN_POINT ( 'NONE',  ( 18.54610009393809023, 0.6523581019769808531, -231.1787333216317677 ) ) ;
#11862=CARTESIAN_POINT ( 'NONE',  ( 3.247425482496454130, -26.49846316390620160, -232.4805733197358677 ) ) ;
#11863=CARTESIAN_POINT ( 'NONE',  ( -26.19327040236159831, 13.44417515682194875, -223.7810975255189874 ) ) ;
#11864=CARTESIAN_POINT ( 'NONE',  ( 9.880827190695510964, 24.82036951119805579, -218.1633337467656020 ) ) ;
#11866=CARTESIAN_POINT ( 'NONE',  ( -20.83683780809167629, -19.66850649927503625, -219.7460615899071570 ) ) ;
#11867=CARTESIAN_POINT ( 'NONE',  ( -23.99493126334580850, 6.052326449358573335, -219.7958990219547672 ) ) ;
#11868=CARTESIAN_POINT ( 'NONE',  ( 19.97628502126439187, 24.50819884991013708, -224.8824979922784735 ) ) ;
#11870=CARTESIAN_POINT ( 'NONE',  ( -11.33137429837660193, 27.25022425932026238, -230.1650924901870212 ) ) ;
#11871=CARTESIAN_POINT ( 'NONE',  ( 19.38320831645075870, -15.01455373846949293, -219.3474289024948689 ) ) ;
#11872=CARTESIAN_POINT ( 'NONE',  ( 21.50885124049339936, -13.38680967545814404, -232.7305552638522954 ) ) ;
#11874=CARTESIAN_POINT ( 'NONE',  ( 4.907833106823921376, 13.98151846258800290, -229.0190609869640923 ) ) ;
#11875=CARTESIAN_POINT ( 'NONE',  ( -23.12176686270140991, -7.251528982847554872, -234.5139663548038413 ) ) ;
#11876=CARTESIAN_POINT ( 'NONE',  ( -8.376153411442972541, -27.59911039556260448, -219.0729038785590888 ) ) ;
#11877=CARTESIAN_POINT ( 'NONE',  ( 11.43609017326686050, -13.06727081285745307, -217.8903327850316316 ) ) ;
#11878=CARTESIAN_POINT ( 'NONE',  ( -8.308618357598591686, 12.44656112581930785, -228.0014162119141474 ) ) ;
#11880=CARTESIAN_POINT ( 'NONE',  ( 11.05872493453861161, 12.09300746323778775, -226.7727269015348952 ) ) ;
#11881=CARTESIAN_POINT ( 'NONE',  ( -17.39699619235753048, 15.64332637722790054, -216.0406373264262641 ) ) ;
#11882=CARTESIAN_POINT ( 'NONE',  ( -10.46043650402819125, 8.998596506756641134, -222.4402691847174083 ) ) ;
#11883=CARTESIAN_POINT ( 'NONE',  ( -21.81769295881711557, -14.18202798484824534, -220.2668003432649471 ) ) ;
#11885=CARTESIAN_POINT ( 'NONE',  ( -7.965409144353247761, 13.56739834143082213, -221.6246244520798712 ) ) ;
#11886=CARTESIAN_POINT ( 'NONE',  ( 30.52813181070726856, 5.438803974502569361, -223.5441926215666513 ) ) ;
#11887=CARTESIAN_POINT ( 'NONE',  ( 13.32754126089433377, 12.31312334927721963, -234.6033665822900218 ) ) ;
#11888=CARTESIAN_POINT ( 'NONE',  ( 28.81324478616323148, -9.895151559995404966, -227.1624192579662918 ) ) ;
#11891=CARTESIAN_POINT ( 'NONE',  ( -3.855805549595750392, 26.68244055262801950, -232.4569730455296508 ) ) ;
#11892=CARTESIAN_POINT ( 'NONE',  ( -25.31373219958254595, -16.11658482301340811, -218.6250613297025609 ) ) ;
#11894=CARTESIAN_POINT ( 'NONE',  ( 14.19800769603076240, 4.587407146151301518, -224.2928935459285071 ) ) ;
#11896=CARTESIAN_POINT ( 'NONE',  ( 20.38902395782249144, -18.95772103455488633, -230.9098670703349967 ) ) ;
#11898=CARTESIAN_POINT ( 'NONE',  ( -11.67631226053870996, 6.737291529340801333, -227.3110382950315227 ) ) ;
#11899=CARTESIAN_POINT ( 'NONE',  ( 27.79670308438203108, 10.67628923451848877, -225.2981230784098727 ) ) ;
#11900=CARTESIAN_POINT ( 'NONE',  ( -0.1049609700611137120, -29.11428177772140558, -224.8408750893923411 ) ) ;
#11904=CARTESIAN_POINT ( 'NONE',  ( 13.43185000535467211, -22.27464880184020757, -218.9084381759842870 ) ) ;
#11905=CARTESIAN_POINT ( 'NONE',  ( -25.95884575339096401, -1.972114683626720044, -231.2145524501483749 ) ) ;
#11907=CARTESIAN_POINT ( 'NONE',  ( 15.20072702475037296, 19.31591084219522614, -219.7402199933931399 ) ) ;
#11909=CARTESIAN_POINT ( 'NONE',  ( 5.549682179574114471, 15.11687613544382280, -226.9959476502473308 ) ) ;
#11910=CARTESIAN_POINT ( 'NONE',  ( 8.821624174887295666, -16.56651460208862758, -234.0193988870521196 ) ) ;
#11911=CARTESIAN_POINT ( 'NONE',  ( 10.24538335401965661, -11.82980241027587276, -219.3753974371782363 ) ) ;
#11913=CARTESIAN_POINT ( 'NONE',  ( -7.965409144353247761, 13.56739834143082213, -221.6246244520798712 ) ) ;
#11914=CARTESIAN_POINT ( 'NONE',  ( -19.33106196848021341, 9.919700385716687663, -219.0532654734256255 ) ) ;
#11915=CARTESIAN_POINT ( 'NONE',  ( 12.98277799799954124, 10.30128574332056779, -221.9415428419440559 ) ) ;
#11917=CARTESIAN_POINT ( 'NONE',  ( -7.205518813659622879, -14.37210213534873482, -226.5338589405291998 ) ) ;
#11920=CARTESIAN_POINT ( 'NONE',  ( 16.10828274231666768, 3.530956590605524692, -220.6574330336208050 ) ) ;
#11921=CARTESIAN_POINT ( 'NONE',  ( 11.99204520814221553, -11.76515119196726467, -228.0494177468141572 ) ) ;
#11922=CARTESIAN_POINT ( 'NONE',  ( 8.329997790135040603, 12.51216704542961899, -228.7022893680961602 ) ) ;
#11923=CARTESIAN_POINT ( 'NONE',  ( -24.68906941503829700, 2.445024713909649705, -232.6803430500543755 ) ) ;
#11924=CARTESIAN_POINT ( 'NONE',  ( 11.20713200305815427, 28.28922876448651635, -219.1239564724620834 ) ) ;
#11925=CARTESIAN_POINT ( 'NONE',  ( -11.19223248830523332, 8.463078350427430507, -222.6400917074981578 ) ) ;
#11927=CARTESIAN_POINT ( 'NONE',  ( -3.843007962268670585, 27.94983497691806917, -231.4302614368887703 ) ) ;
#11929=CARTESIAN_POINT ( 'NONE',  ( -1.890995374385051608, -13.09686096954197509, -227.5694739903412085 ) ) ;
#11933=CARTESIAN_POINT ( 'NONE',  ( -24.76115377241536208, -2.015397159694146456, -231.8500816169410825 ) ) ;
#11934=CARTESIAN_POINT ( 'NONE',  ( -29.65068623107463708, 4.004319520977249525, -231.5200339834770773 ) ) ;
#11935=CARTESIAN_POINT ( 'NONE',  ( -17.60926409178586738, -17.65542935640887023, -231.2676365506119680 ) ) ;
#11938=CARTESIAN_POINT ( 'NONE',  ( 4.002939343642331949, -22.37368820207002429, -217.8631878264377804 ) ) ;
#11939=CARTESIAN_POINT ( 'NONE',  ( 12.15450584778660570, 2.288537795953278220, -225.7049340319972828 ) ) ;
#11940=CARTESIAN_POINT ( 'NONE',  ( -0.7041916573665241152, 14.60214745152014437, -226.3818583194645555 ) ) ;
#11941=CARTESIAN_POINT ( 'NONE',  ( -7.694246740028670928, 10.31295298368923063, -221.9989544301487001 ) ) ;
#11942=CARTESIAN_POINT ( 'NONE',  ( -18.99425472824626482, -3.261482901149847180, -230.2374083206451871 ) ) ;
#11944=CARTESIAN_POINT ( 'NONE',  ( 7.769483725421269860, 20.68783433326350263, -233.2348178266662728 ) ) ;
#11945=CARTESIAN_POINT ( 'NONE',  ( -18.94444594796027914, 3.458349568010113728, -218.9807021659310635 ) ) ;
#11946=CARTESIAN_POINT ( 'NONE',  ( -11.10182655035041144, 8.778638955377752850, -227.1050196202568827 ) ) ;
#11947=CARTESIAN_POINT ( 'NONE',  ( -10.94940667656068634, -10.80050631132953498, -220.7362776234490127 ) ) ;
#11950=CARTESIAN_POINT ( 'NONE',  ( 15.37089934297015503, 20.64239674606488961, -217.2018742121147170 ) ) ;
#11951=CARTESIAN_POINT ( 'NONE',  ( -17.30580402557236752, 11.30149179219993982, -230.8639894634705172 ) ) ;
#11952=CARTESIAN_POINT ( 'NONE',  ( 9.169328349715531346, 20.85917603618721472, -214.7000934853629133 ) ) ;
#11953=CARTESIAN_POINT ( 'NONE',  ( 15.18181359483165949, 6.369295616116027681, -230.7949408486033462 ) ) ;
#11955=CARTESIAN_POINT ( 'NONE',  ( -8.861553082841476581, -17.08180233781500590, -216.2529452235939402 ) ) ;
#11958=CARTESIAN_POINT ( 'NONE',  ( -10.35216574861945560, -14.43870810227675605, -231.1876371800402126 ) ) ;
#11960=CARTESIAN_POINT ( 'NONE',  ( -16.23478446547628096, 26.31175924651574149, -222.4178907105033431 ) ) ;
#11961=CARTESIAN_POINT ( 'NONE',  ( 5.982950994121768673, -14.58086824529316594, -231.1438280359330975 ) ) ;
#11962=CARTESIAN_POINT ( 'NONE',  ( -1.249406995060579062, 25.48934319316224162, -216.9406480707515072 ) ) ;
#11963=CARTESIAN_POINT ( 'NONE',  ( 18.64433268355766415, -12.21264687082605782, -214.8850304513305502 ) ) ;
#11964=CARTESIAN_POINT ( 'NONE',  ( -18.53787071664277519, -6.556543064843903146, -232.5192140591401824 ) ) ;
#11965=CARTESIAN_POINT ( 'NONE',  ( 12.47670316482120967, 2.249148913447538423, -227.4574095259895898 ) ) ;
#11966=CARTESIAN_POINT ( 'NONE',  ( -7.770318051073092036, 21.02940971564074957, -231.8751410922876630 ) ) ;
#11967=CARTESIAN_POINT ( 'NONE',  ( 14.29768887814754663, 10.87030385293788548, -231.8067013864770161 ) ) ;
#11968=CARTESIAN_POINT ( 'NONE',  ( 14.54149994592679107, 8.070685273005897997, -229.7292930672863349 ) ) ;
#11969=CARTESIAN_POINT ( 'NONE',  ( 11.75069299018312208, 6.043853022588032253, -224.2604610870103841 ) ) ;
#11970=CARTESIAN_POINT ( 'NONE',  ( 3.668385877085885927, -11.51845067838601366, -222.7629028536941291 ) ) ;
#11971=CARTESIAN_POINT ( 'NONE',  ( -8.985448925281199095, 11.82743561134668475, -224.1067108988273162 ) ) ;
#11974=CARTESIAN_POINT ( 'NONE',  ( 20.34032485158648029, 2.741617426884598530, -217.9827731991294968 ) ) ;
#11975=CARTESIAN_POINT ( 'NONE',  ( 3.881011284096109293, -13.04786028604701187, -224.6787317506201589 ) ) ;
#11976=CARTESIAN_POINT ( 'NONE',  ( -14.35594238341465889, 9.236863657925704629, -219.6542735655305307 ) ) ;
#11977=CARTESIAN_POINT ( 'NONE',  ( 3.367418898937407867, 27.20023797116225595, -219.3349021808245709 ) ) ;
#11978=CARTESIAN_POINT ( 'NONE',  ( -25.98129645912436914, -15.13773040547512139, -224.1390156429105787 ) ) ;
#11979=CARTESIAN_POINT ( 'NONE',  ( 12.25122766587143630, 4.035812653434439845, -225.7709573147497224 ) ) ;
#11980=CARTESIAN_POINT ( 'NONE',  ( 23.83082175545800752, 15.77842900014857896, -219.5351905769044834 ) ) ;
#11982=CARTESIAN_POINT ( 'NONE',  ( 18.23324537670537993, 23.47692953258263771, -224.8333321331434433 ) ) ;
#11983=CARTESIAN_POINT ( 'NONE',  ( 19.92157794555808437, -7.202678279460218214, -232.3584036642729416 ) ) ;
#11984=CARTESIAN_POINT ( 'NONE',  ( 16.26147397530412420, -13.20473954510486081, -216.9283256773164794 ) ) ;
#11986=CARTESIAN_POINT ( 'NONE',  ( 8.812073984913094904, 13.12649198322903210, -229.9172071780580495 ) ) ;
#11987=CARTESIAN_POINT ( 'NONE',  ( -14.44949936980387584, -0.9990553581641278269, -220.3450678990494964 ) ) ;
#11988=CARTESIAN_POINT ( 'NONE',  ( -2.576162127940193169, -15.57202066281789321, -231.6911579627040396 ) ) ;
#11990=CARTESIAN_POINT ( 'NONE',  ( 19.88636028791461641, -20.85574262981397453, -219.9907771812986823 ) ) ;
#11991=CARTESIAN_POINT ( 'NONE',  ( -15.63515374589483109, 24.59141623553136569, -226.9057426066772507 ) ) ;
#11992=CARTESIAN_POINT ( 'NONE',  ( 5.064106757301036765, 16.06517852189101703, -221.6413221086847329 ) ) ;
#11993=CARTESIAN_POINT ( 'NONE',  ( -27.90314475660494153, 12.48829126175061077, -223.3300566725355338 ) ) ;
#11994=CARTESIAN_POINT ( 'NONE',  ( -12.88152464663890306, 6.317716727793897924, -230.5294309895745073 ) ) ;
#11995=CARTESIAN_POINT ( 'NONE',  ( 25.90657540470570197, -10.31326923046670885, -218.6707845005603019 ) ) ;
#11998=CARTESIAN_POINT ( 'NONE',  ( -7.284474494690100776, 13.60812129561547046, -227.7414351104868331 ) ) ;
#11999=CARTESIAN_POINT ( 'NONE',  ( 25.38325563848796662, 11.05100313887457553, -217.8685524735130628 ) ) ;
#12000=CARTESIAN_POINT ( 'NONE',  ( 10.00603923119254723, 9.610873433734882454, -231.2388095806506669 ) ) ;
#12001=CARTESIAN_POINT ( 'NONE',  ( 12.75766869239441803, -12.84633107758633663, -232.0853690516983079 ) ) ;
#12004=CARTESIAN_POINT ( 'NONE',  ( -3.755296588130283553, 23.77975947300719284, -233.7323173085780752 ) ) ;
#12005=CARTESIAN_POINT ( 'NONE',  ( -8.731539701382653007, -8.828156491469059119, -227.3463890218280596 ) ) ;
#12007=CARTESIAN_POINT ( 'NONE',  ( 14.68783945462866924, 9.535285537539673228, -219.4694094309942045 ) ) ;
#12008=CARTESIAN_POINT ( 'NONE',  ( -14.68037037322036475, 3.441677802729143920, -220.1396515630443389 ) ) ;
#12010=CARTESIAN_POINT ( 'NONE',  ( 12.02378739738799140, -16.98783239109716092, -233.4545636224233931 ) ) ;
#12012=CARTESIAN_POINT ( 'NONE',  ( -11.79584727357715934, 6.509288465425584036, -222.6080315736180921 ) ) ;
#12014=CARTESIAN_POINT ( 'NONE',  ( -16.15126510923403202, -0.4755054218165427615, -219.3066569788202571 ) ) ;
#12015=CARTESIAN_POINT ( 'NONE',  ( -7.180402128846711918, -26.42159752827261698, -220.2116303544826224 ) ) ;
#12018=CARTESIAN_POINT ( 'NONE',  ( -13.92046207272054303, -0.1600067567908077248, -224.5811699126800818 ) ) ;
#12019=CARTESIAN_POINT ( 'NONE',  ( 10.81635663018848525, -11.46278932037511566, -222.6527676248099681 ) ) ;
#12020=CARTESIAN_POINT ( 'NONE',  ( 14.06870332774840193, -1.847654110632577229, -227.3635178367878780 ) ) ;
#12022=CARTESIAN_POINT ( 'NONE',  ( 19.59567110982616001, 18.11097967140601028, -228.7314497914969706 ) ) ;
#12023=CARTESIAN_POINT ( 'NONE',  ( 7.497537106193371770, 19.52448593130572618, -231.1338690134634248 ) ) ;
#12024=CARTESIAN_POINT ( 'NONE',  ( 20.22673842361927399, -24.21895433676095877, -222.6595898022596316 ) ) ;
#12025=CARTESIAN_POINT ( 'NONE',  ( 7.021536848793814123, -14.49751826649810482, -218.4909385705359455 ) ) ;
#12027=CARTESIAN_POINT ( 'NONE',  ( -10.40174557315337900, 22.75579539577861965, -231.4492192189165962 ) ) ;
#12028=CARTESIAN_POINT ( 'NONE',  ( -18.33565906012873725, 9.491905303418088025, -219.1855745749628568 ) ) ;
#12029=CARTESIAN_POINT ( 'NONE',  ( -13.34869474643618581, 6.516017165032126357, -231.2228057326931321 ) ) ;
#12031=CARTESIAN_POINT ( 'NONE',  ( -14.13544422886439911, -23.73189729233824252, -223.0800202563271171 ) ) ;
#12034=CARTESIAN_POINT ( 'NONE',  ( 13.14260364752544596, 5.866423290307341887, -222.7705901084601408 ) ) ;
#12035=CARTESIAN_POINT ( 'NONE',  ( 17.04113992636424513, -19.77713422747145700, -220.8032168804961373 ) ) ;
#12036=CARTESIAN_POINT ( 'NONE',  ( 10.50530447320976535, 20.19629329636330084, -217.1354359361034767 ) ) ;
#12037=CARTESIAN_POINT ( 'NONE',  ( -7.189383125363055349, 14.28512618638020548, -231.7475838278701303 ) ) ;
#12039=CARTESIAN_POINT ( 'NONE',  ( 18.59615491886314231, -0.2392802120807639710, -217.5848846836084078 ) ) ;
#12041=CARTESIAN_POINT ( 'NONE',  ( -8.172572110426221670, 16.86653848210977813, -233.4220330256369493 ) ) ;
#12043=CARTESIAN_POINT ( 'NONE',  ( 15.52719855059926424, 1.633696074270991172, -221.7349885876216433 ) ) ;
#12044=CARTESIAN_POINT ( 'NONE',  ( 8.532614294830283441, -28.73326933124977955, -229.1610356131385231 ) ) ;
#12046=CARTESIAN_POINT ( 'NONE',  ( 22.03647168421188240, 0.3315607655626218175, -232.0572713672587213 ) ) ;
#12047=DIRECTION ( 'NONE',  ( 1.000000000000000000, 0.000000000000000000, 0.000000000000000000 ) ) ;
#12048=CARTESIAN_POINT ( 'NONE',  ( -26.07210576407111446, -8.413030596423759278, -230.6002792590230115 ) ) ;
#12049=CARTESIAN_POINT ( 'NONE',  ( 18.54610009393809023, 0.6523581019769808531, -231.1787333216317677 ) ) ;
#12050=CARTESIAN_POINT ( 'NONE',  ( -14.91191843134457784, -11.59770670008449756, -219.5316993567479642 ) ) ;
#12051=CARTESIAN_POINT ( 'NONE',  ( 7.092430827040528740, -27.48041265710635628, -228.4891580147104548 ) ) ;
#12052=CARTESIAN_POINT ( 'NONE',  ( 17.41909632439413969, 2.006477695503792624, -233.4081875040758121 ) ) ;
#12053=CARTESIAN_POINT ( 'NONE',  ( 9.336393807558161839, 27.79372469574263960, -228.5913636680961361 ) ) ;
#12054=CARTESIAN_POINT ( 'NONE',  ( -20.38637754046084183, 19.95723714148678241, -217.5201383746364172 ) ) ;
#12056=CARTESIAN_POINT ( 'NONE',  ( 30.90240445905660138, -9.617167762261830788, -225.5262352394493064 ) ) ;
#12058=CARTESIAN_POINT ( 'NONE',  ( 13.43170911749896490, 19.07691563292472026, -232.7497845103644636 ) ) ;
#12059=CARTESIAN_POINT ( 'NONE',  ( -14.58084844870496966, 13.85720943031455832, -233.3219724312919254 ) ) ;
#12060=CARTESIAN_POINT ( 'NONE',  ( -22.70558257617108922, 14.65737936663030538, -230.9775454010380997 ) ) ;
#12061=CARTESIAN_POINT ( 'NONE',  ( -16.87231408860552051, -20.68405295654727993, -231.0270656955280515 ) ) ;
#12066=CARTESIAN_POINT ( 'NONE',  ( -20.29166677327761903, 16.18344358422343632, -220.0060062064338524 ) ) ;
#12067=CARTESIAN_POINT ( 'NONE',  ( 10.02118533929671074, 10.65166262057242008, -217.7534731326719566 ) ) ;
#12068=CARTESIAN_POINT ( 'NONE',  ( 12.56362091610784049, 9.747446748398973071, -231.6428467497164547 ) ) ;
#12069=CARTESIAN_POINT ( 'NONE',  ( -16.68014207497104451, -3.425858445063780788, -215.9332308579483595 ) ) ;
#12071=CARTESIAN_POINT ( 'NONE',  ( -5.056986327342952947, -15.36481113542577503, -220.7955371552936583 ) ) ;
#12072=CARTESIAN_POINT ( 'NONE',  ( -8.894613172508529786, 25.42460746921206294, -232.3150764041658363 ) ) ;
#12073=CARTESIAN_POINT ( 'NONE',  ( 11.14834367153813233, -21.42845646353120870, -216.4520112529555718 ) ) ;
#12074=CARTESIAN_POINT ( 'NONE',  ( -6.571166997218196748, 12.74865329367398736, -229.9840124400968762 ) ) ;
#12075=CARTESIAN_POINT ( 'NONE',  ( 24.71064586368820315, -12.65488197590634378, -232.9862317762581654 ) ) ;
#12077=CARTESIAN_POINT ( 'NONE',  ( -25.10035252441274167, -15.33546242866430198, -228.3913311683031964 ) ) ;
#12078=CARTESIAN_POINT ( 'NONE',  ( -15.83178333309709629, 2.467763724635483324, -230.4064772870105458 ) ) ;
#12080=CARTESIAN_POINT ( 'NONE',  ( -1.364406401035816785, 24.33111505239456918, -219.5658712396381418 ) ) ;
#12081=CARTESIAN_POINT ( 'NONE',  ( -14.06164063153489252, 2.050767714179807744, -227.2881998904968270 ) ) ;
#12082=CARTESIAN_POINT ( 'NONE',  ( 15.89706143421296147, 10.57416387607782227, -218.3862415393350318 ) ) ;
#12083=CARTESIAN_POINT ( 'NONE',  ( 21.17011458613547248, 1.652544727609948527, -234.6098499860487152 ) ) ;
#12084=CARTESIAN_POINT ( 'NONE',  ( 5.535251771770903773, -29.91249465213552128, -219.7039649384792028 ) ) ;
#12085=CARTESIAN_POINT ( 'NONE',  ( 13.79814099039094089, 16.09927043668092850, -214.6489469124405502 ) ) ;
#12087=CARTESIAN_POINT ( 'NONE',  ( -6.776294192501696401, -30.39940938379458046, -221.2799938066956997 ) ) ;
#12088=CARTESIAN_POINT ( 'NONE',  ( -10.30870167223346456, 11.95603877111467561, -228.4123369090513336 ) ) ;
#12090=CARTESIAN_POINT ( 'NONE',  ( 2.893760225568064115, 14.39521026618305477, -227.6654023557511550 ) ) ;
#12091=CARTESIAN_POINT ( 'NONE',  ( -20.76924187596804217, -21.50248317380421170, -228.3679492147379335 ) ) ;
#12092=CARTESIAN_POINT ( 'NONE',  ( -22.90687623753526125, 9.466200233939549236, -230.1557007022273638 ) ) ;
#12093=CARTESIAN_POINT ( 'NONE',  ( 25.02650711521362936, 17.58144575069911042, -223.6165279156031431 ) ) ;
#12095=CARTESIAN_POINT ( 'NONE',  ( 17.97843143658897347, 22.12221935793617078, -220.9346589834416079 ) ) ;
#12096=CARTESIAN_POINT ( 'NONE',  ( 17.78250599636351481, -9.160802950715318360, -218.6762383290621869 ) ) ;
#12098=CARTESIAN_POINT ( 'NONE',  ( 27.81506808824343580, -10.52944849582878106, -221.0913368219556503 ) ) ;
#12100=CARTESIAN_POINT ( 'NONE',  ( 19.72515656911863147, 14.02277373989196541, -218.0718040828188009 ) ) ;
#12101=CARTESIAN_POINT ( 'NONE',  ( -14.05955845762884238, -0.8719634938775207011, -221.0475910153949428 ) ) ;
#12102=CARTESIAN_POINT ( 'NONE',  ( -6.163092920833200594, -27.00835405423771007, -232.1022292408408987 ) ) ;
#12103=CARTESIAN_POINT ( 'NONE',  ( 21.05631363308661363, -21.50266115212419393, -222.6654548186096747 ) ) ;
#12104=CARTESIAN_POINT ( 'NONE',  ( 1.455106383990497187, 21.12056149333958999, -230.8076663600630241 ) ) ;
#12106=CARTESIAN_POINT ( 'NONE',  ( 15.08139719848974103, 12.15862464477973504, -219.3112749338812080 ) ) ;
#12107=CARTESIAN_POINT ( 'NONE',  ( -10.65455960636934662, 10.37188583052882862, -219.5197110153079620 ) ) ;
#12108=CARTESIAN_POINT ( 'NONE',  ( -6.769588938507062004, 18.22485903270490937, -231.3660928915624879 ) ) ;
#12109=CARTESIAN_POINT ( 'NONE',  ( 28.46281617689634302, -10.50803404096709137, -222.5507679334694728 ) ) ;
#12110=CARTESIAN_POINT ( 'NONE',  ( 3.160467108836292116, 14.95099014189016629, -228.9242958482614370 ) ) ;
#12111=CARTESIAN_POINT ( 'NONE',  ( 13.16746181015946959, 0.3897807143096829741, -227.1676274388083243 ) ) ;
#12112=CARTESIAN_POINT ( 'NONE',  ( 11.38520239593705163, 18.87760105923376486, -235.3435298574111130 ) ) ;
#12113=CARTESIAN_POINT ( 'NONE',  ( 13.07616324839670341, -23.69356132834180784, -230.7206382488779184 ) ) ;
#12116=CARTESIAN_POINT ( 'NONE',  ( -7.395406416482832590, 12.93623984139929739, -219.2606224730616873 ) ) ;
#12117=CARTESIAN_POINT ( 'NONE',  ( -22.42461747750134293, -16.81348984091923171, -233.1118345967658172 ) ) ;
#12119=CARTESIAN_POINT ( 'NONE',  ( 21.39553407250273054, 8.453402029343234148, -217.9531594780983141 ) ) ;
#12120=CARTESIAN_POINT ( 'NONE',  ( -16.20072894238734307, 0.5024448614660336210, -230.4554067149722130 ) ) ;
#12121=CARTESIAN_POINT ( 'NONE',  ( 18.55298002304457228, -12.22359628793950570, -216.9137843736221782 ) ) ;
#12122=CARTESIAN_POINT ( 'NONE',  ( -15.82069055112642353, 8.315535108674763976, -217.2800172218543935 ) ) ;
#12123=CARTESIAN_POINT ( 'NONE',  ( -20.43618815875133521, 1.403378831510147196, -232.9646741665398224 ) ) ;
#12125=CARTESIAN_POINT ( 'NONE',  ( -1.380908993000753648, -20.21092959135559752, -218.0995018783601438 ) ) ;
#12128=CARTESIAN_POINT ( 'NONE',  ( -22.11084984981285118, 10.96048252433489623, -216.6117774006995376 ) ) ;
#12129=CARTESIAN_POINT ( 'NONE',  ( 15.76600796393256410, -24.40864267010898558, -225.5036181134576907 ) ) ;
#12130=CARTESIAN_POINT ( 'NONE',  ( 13.36754297251702717, -1.844478585726079256, -222.6328387543338181 ) ) ;
#12132=CARTESIAN_POINT ( 'NONE',  ( 20.92326490933994876, 18.00580109995737033, -222.6060933800056034 ) ) ;
#12133=CARTESIAN_POINT ( 'NONE',  ( -10.98447002683091256, 8.146786682930290624, -230.8316952156193338 ) ) ;
#12134=CARTESIAN_POINT ( 'NONE',  ( 13.96918721733258195, 14.12724320058294403, -230.4946432816737172 ) ) ;
#12135=CARTESIAN_POINT ( 'NONE',  ( -1.494569538902034145, -28.29191435206508487, -228.8702894339512852 ) ) ;
#12136=CARTESIAN_POINT ( 'NONE',  ( 30.29962988386644085, -7.724198041227372080, -225.2151988352147782 ) ) ;
#12138=CARTESIAN_POINT ( 'NONE',  ( -16.07193224038526580, 12.24477688577882439, -232.1409653212175499 ) ) ;
#12139=CARTESIAN_POINT ( 'NONE',  ( -23.52458685063474420, 4.195399146287285497, -230.7490123595086970 ) ) ;
#12140=CARTESIAN_POINT ( 'NONE',  ( -17.17981675979428147, 1.478343374046288128, -216.2419730925687418 ) ) ;
#12141=CARTESIAN_POINT ( 'NONE',  ( -4.572289063834428013, -16.67516242687949557, -229.9678395161569142 ) ) ;
#12144=CARTESIAN_POINT ( 'NONE',  ( 22.42095341476093040, 9.457779162868732215, -232.6339572190428555 ) ) ;
#12145=CARTESIAN_POINT ( 'NONE',  ( 11.63667859525082093, -10.90089931597979600, -224.9413544669828013 ) ) ;
#12146=CARTESIAN_POINT ( 'NONE',  ( 3.763426558366607111, 28.60172112197566818, -230.1816715025297526 ) ) ;
#12147=CARTESIAN_POINT ( 'NONE',  ( -8.172572110426221670, 16.86653848210977813, -233.4220330256369493 ) ) ;
#12148=CARTESIAN_POINT ( 'NONE',  ( 13.21888801141564151, 2.135177519634172238, -228.0426311217386797 ) ) ;
#12150=CARTESIAN_POINT ( 'NONE',  ( 8.496844655769807630, 14.66037471857024599, -219.1631158796573118 ) ) ;
#12152=CARTESIAN_POINT ( 'NONE',  ( -7.460068573003235670, -29.58770008691625364, -228.1902472473001637 ) ) ;
#12153=CARTESIAN_POINT ( 'NONE',  ( 18.00123703865980218, -15.82960056198189491, -233.0014896689109776 ) ) ;
#12156=CARTESIAN_POINT ( 'NONE',  ( -9.924247690135956645, 7.079756654796299564, -222.1205998075789694 ) ) ;
#12157=CARTESIAN_POINT ( 'NONE',  ( -17.33275459786259276, -4.423804729537573088, -220.8440611986277418 ) ) ;
#12159=CARTESIAN_POINT ( 'NONE',  ( 14.19979467405507556, 6.351366891014061267, -230.8614099669030679 ) ) ;
#12160=CARTESIAN_POINT ( 'NONE',  ( 3.192353461299334061, 22.13718518159985393, -217.1103300728619843 ) ) ;
#12161=CARTESIAN_POINT ( 'NONE',  ( 3.100794261777709782, 20.70580715608724276, -231.8781843337728219 ) ) ;
#12163=CARTESIAN_POINT ( 'NONE',  ( -27.92538795710911259, -2.661554249663629079, -224.6264721727631581 ) ) ;
#12164=CARTESIAN_POINT ( 'NONE',  ( 16.54345861550681107, 19.37554510112122230, -218.2240151908141002 ) ) ;
#12165=CARTESIAN_POINT ( 'NONE',  ( -8.329232059016652201, 11.81357365351366617, -230.1839637212758021 ) ) ;
#12166=CARTESIAN_POINT ( 'NONE',  ( -13.43384090552117271, 6.057765724406720231, -225.7182623230366119 ) ) ;
#12167=CARTESIAN_POINT ( 'NONE',  ( -19.18273340400098448, -14.85130345181434741, -232.7114379411565039 ) ) ;
#12168=CARTESIAN_POINT ( 'NONE',  ( -15.15434969228324924, 4.423874646950748613, -230.6144467931089821 ) ) ;
#12172=CARTESIAN_POINT ( 'NONE',  ( 17.91327661571172314, 1.545939370248587075, -216.9938266089438912 ) ) ;
#12173=CARTESIAN_POINT ( 'NONE',  ( -10.45265333418718612, 16.71118685480038479, -231.7490466715443631 ) ) ;
#12175=CARTESIAN_POINT ( 'NONE',  ( 11.50837930502119733, 10.86662242793286381, -233.1728506169798436 ) ) ;
#12176=CARTESIAN_POINT ( 'NONE',  ( 20.88210880980788531, 0.9259446317980322139, -218.6312544800709929 ) ) ;
#12177=CARTESIAN_POINT ( 'NONE',  ( -22.42461747750134293, -16.81348984091923171, -233.1118345967658172 ) ) ;
#12178=CARTESIAN_POINT ( 'NONE',  ( -28.74911369566071784, -10.37195270599671737, -225.4617258471509729 ) ) ;
#12180=CARTESIAN_POINT ( 'NONE',  ( -13.58389614404818069, 15.11490620317918676, -215.3922994348461941 ) ) ;
#12181=CARTESIAN_POINT ( 'NONE',  ( 0.04660897052267574947, -31.13860575300111577, -224.7746869833732717 ) ) ;
#12182=CARTESIAN_POINT ( 'NONE',  ( -3.368164009525018265, 19.03203264544105622, -233.5986411977714567 ) ) ;
#12183=CARTESIAN_POINT ( 'NONE',  ( 27.24384134789437439, -15.00887433271272364, -228.9543321217944083 ) ) ;
#12184=CARTESIAN_POINT ( 'NONE',  ( 13.80743592543072396, -3.637675435010108906E-12, -228.0000000000000568 ) ) ;
#12185=CARTESIAN_POINT ( 'NONE',  ( 18.30177952310522471, 1.918278963380847468, -233.8574151782075887 ) ) ;
#12187=CARTESIAN_POINT ( 'NONE',  ( 0.04449911090679885967, 16.51968908208873899, -222.9067194156212111 ) ) ;
#12188=CARTESIAN_POINT ( 'NONE',  ( -21.28183200535960040, 1.085030287403131233, -217.0000000015322712 ) ) ;
#12189=CARTESIAN_POINT ( 'NONE',  ( 18.60971343765040942, 2.368090295052050820, -218.6871071987073094 ) ) ;
#12190=CARTESIAN_POINT ( 'NONE',  ( 13.25330606581809789, 10.40242132629824034, -230.9170765704288044 ) ) ;
#12191=CARTESIAN_POINT ( 'NONE',  ( -2.619247311076123630, -29.90652300472198988, -220.3405913430138128 ) ) ;
#12192=CARTESIAN_POINT ( 'NONE',  ( 7.283976506941576723, 24.82246917020504284, -234.3244871078919402 ) ) ;
#12194=CARTESIAN_POINT ( 'NONE',  ( -3.739406429132753562, -13.42303118918103344, -219.1969888661882635 ) ) ;
#12195=CARTESIAN_POINT ( 'NONE',  ( -17.14223598032838325, 23.31797360549976261, -226.5771676936548431 ) ) ;
#12196=CARTESIAN_POINT ( 'NONE',  ( 16.64575860537911112, 25.12688477742292648, -227.5050599151411745 ) ) ;
#12197=CARTESIAN_POINT ( 'NONE',  ( -22.20848920810297855, -2.028924892417935055, -232.4401719831211039 ) ) ;
#12198=CARTESIAN_POINT ( 'NONE',  ( -18.42638600874552424, 7.060399206045774534, -230.3991437614443214 ) ) ;
#12199=CARTESIAN_POINT ( 'NONE',  ( -12.26337789213896201, 9.274758280606999250, -219.9806108963443876 ) ) ;
#12200=CARTESIAN_POINT ( 'NONE',  ( 17.66865342763861690, 2.849170916951684784, -230.9175656266857004 ) ) ;
#12202=CARTESIAN_POINT ( 'NONE',  ( 10.78187269046063435, 10.73871010366167944, -221.9206544238666368 ) ) ;
#12203=CARTESIAN_POINT ( 'NONE',  ( 13.77063830053042892, -24.19668776886549821, -225.6207953771408086 ) ) ;
#12205=CARTESIAN_POINT ( 'NONE',  ( 13.39541376241636783, -3.462025909069690321, -228.4300562622815391 ) ) ;
#12206=CARTESIAN_POINT ( 'NONE',  ( 1.296323513242173542, 20.09034598902932345, -230.5712631353794961 ) ) ;
#12209=CARTESIAN_POINT ( 'NONE',  ( 8.689059922489732912, 15.18271246186214363, -218.7354841152034908 ) ) ;
#12210=CARTESIAN_POINT ( 'NONE',  ( -14.30218759248275084, -10.01744029472290620, -234.2423117832250341 ) ) ;
#12211=CARTESIAN_POINT ( 'NONE',  ( -5.804961988600464196, -12.67915086496026511, -228.7923277404792088 ) ) ;
#12212=CARTESIAN_POINT ( 'NONE',  ( 1.541778504653760429, -23.48174737203985529, -233.9922866444541967 ) ) ;
#12213=CARTESIAN_POINT ( 'NONE',  ( -9.060146982536336324, 27.14942986116457746, -225.6568961786626062 ) ) ;
#12215=CARTESIAN_POINT ( 'NONE',  ( 20.92326490933994876, 18.00580109995737033, -222.6060933800056034 ) ) ;
#12217=CARTESIAN_POINT ( 'NONE',  ( -13.65925618638770800, 3.289586759644148817, -222.1579143493116533 ) ) ;
#12218=CARTESIAN_POINT ( 'NONE',  ( -9.403561938624596550, 12.70246821120386471, -220.7484614495429582 ) ) ;
#12219=CARTESIAN_POINT ( 'NONE',  ( 9.527502190795640757, 23.55559004943647139, -217.4101659741468211 ) ) ;
#12220=CARTESIAN_POINT ( 'NONE',  ( 18.40125535140034430, 0.01434342441762339639, -233.2485400239426099 ) ) ;
#12221=CARTESIAN_POINT ( 'NONE',  ( 13.34963947135311102, 7.416462695144936390, -217.9359469527792044 ) ) ;
#12222=CARTESIAN_POINT ( 'NONE',  ( 7.739744183733028748, -12.54214339878522999, -227.5419174737939159 ) ) ;
#12225=CARTESIAN_POINT ( 'NONE',  ( -2.808235066048971440, 30.42019778760651150, -222.6481917607299295 ) ) ;
#12226=CARTESIAN_POINT ( 'NONE',  ( 22.78751929883380356, -1.647884454956899836, -231.3901500139513416 ) ) ;
#12227=CARTESIAN_POINT ( 'NONE',  ( 24.21331552874348958, 0.07051084380047288602, -231.7986140076958463 ) ) ;
#12228=CARTESIAN_POINT ( 'NONE',  ( 15.42212722119060864, 5.401662248084913465, -220.8333402320903645 ) ) ;
#12229=CARTESIAN_POINT ( 'NONE',  ( -28.17543631911187063, 3.557555778861649642, -230.1980773687482156 ) ) ;
#12230=CARTESIAN_POINT ( 'NONE',  ( 5.434900225474387447, -11.93567727083262042, -224.7511004068755369 ) ) ;
#12232=CARTESIAN_POINT ( 'NONE',  ( -7.913358619554302642, 16.16796202616373890, -233.0981776325470491 ) ) ;
#12234=CARTESIAN_POINT ( 'NONE',  ( -13.10651848559790444, 3.262242204071156948, -224.3513854875720597 ) ) ;
#12235=CARTESIAN_POINT ( 'NONE',  ( -18.96646980336054611, -22.16549408654085696, -227.7928771762007329 ) ) ;
#12238=CARTESIAN_POINT ( 'NONE',  ( -26.58771759052039485, 5.114955214121561511, -218.2823714869195442 ) ) ;
#12239=CARTESIAN_POINT ( 'NONE',  ( 13.24102317311734112, -10.11186274821533715, -227.6843928184991057 ) ) ;
#12240=CARTESIAN_POINT ( 'NONE',  ( -22.20848920810297855, -2.028924892417935055, -232.4401719831211039 ) ) ;
#12243=CARTESIAN_POINT ( 'NONE',  ( 20.59763700141659015, 7.383112456150029423, -232.0722244125682039 ) ) ;
#12244=CARTESIAN_POINT ( 'NONE',  ( -7.694246740028670928, 10.31295298368923063, -221.9989544301487001 ) ) ;
#12245=CARTESIAN_POINT ( 'NONE',  ( 24.93482953594869755, 13.13888391581411241, -222.4369546851285691 ) ) ;
#12246=CARTESIAN_POINT ( 'NONE',  ( -0.7782973328492528431, -21.73504563028646075, -232.5926793935175283 ) ) ;
#12247=CARTESIAN_POINT ( 'NONE',  ( 17.72923050078999907, -1.936365952008033853, -232.4832991314195567 ) ) ;
#12249=CARTESIAN_POINT ( 'NONE',  ( 2.485733319737138736, 14.76073968410796056, -221.5245536174130905 ) ) ;
#12250=CARTESIAN_POINT ( 'NONE',  ( -14.01525440049806193, 8.239250543314939890, -226.5804714421811070 ) ) ;
#12251=CARTESIAN_POINT ( 'NONE',  ( 22.24262848503957812, 2.205713500382371794, -232.7243927205662430 ) ) ;
#12252=CARTESIAN_POINT ( 'NONE',  ( -23.09090074015852778, -15.52172445179926896, -222.9863534629544972 ) ) ;
#12255=CARTESIAN_POINT ( 'NONE',  ( 26.53121369294028042, 10.74560293343441586, -229.2288136770759195 ) ) ;
#12256=CARTESIAN_POINT ( 'NONE',  ( 3.050495372378628112, -23.18092737088175781, -231.5841725462776992 ) ) ;
#12257=CARTESIAN_POINT ( 'NONE',  ( 12.99034161053428349, 11.71468708507361889, -230.9043293568357740 ) ) ;
#12258=CARTESIAN_POINT ( 'NONE',  ( -10.45786516112131892, 23.61456281964591852, -233.2869923610001592 ) ) ;
#12259=CARTESIAN_POINT ( 'NONE',  ( 11.21112214669106777, 5.418350954422431975, -227.6539796508718325 ) ) ;
#12260=CARTESIAN_POINT ( 'NONE',  ( 4.730976410881341465, 17.65764351829336931, -217.6025626048331674 ) ) ;
#12262=CARTESIAN_POINT ( 'NONE',  ( 1.623338700557370951, -21.82196275546919040, -234.1129525514646730 ) ) ;
#12263=CARTESIAN_POINT ( 'NONE',  ( 19.88636028791461641, -20.85574262981397453, -219.9907771812986823 ) ) ;
#12266=CARTESIAN_POINT ( 'NONE',  ( -12.61443312487471324, 8.399394471292156439, -217.5740162615319093 ) ) ;
#12267=CARTESIAN_POINT ( 'NONE',  ( -26.25663555152313222, -8.728475094464092976, -226.4697227271102236 ) ) ;
#12268=CARTESIAN_POINT ( 'NONE',  ( -14.58575946311604277, 2.190332613129932327, -228.6717927865686590 ) ) ;
#12269=CARTESIAN_POINT ( 'NONE',  ( 6.771176146757415637, 15.60014285904435027, -218.3493856697694753 ) ) ;
#12270=CARTESIAN_POINT ( 'NONE',  ( -1.243734262319729389, 14.23902626181890518, -226.4313640849764795 ) ) ;
#12272=CARTESIAN_POINT ( 'NONE',  ( 18.12061937846576853, -10.14999073105125227, -235.3098052193838612 ) ) ;
#12274=CARTESIAN_POINT ( 'NONE',  ( 18.76922974182421555, 13.12635134380198210, -217.8010375391909008 ) ) ;
#12276=CARTESIAN_POINT ( 'NONE',  ( -20.95553895916151177, 12.88782924195037438, -232.2493899712447956 ) ) ;
#12277=CARTESIAN_POINT ( 'NONE',  ( -14.30096418567650041, 6.974026439069829664, -228.7941652905285537 ) ) ;
#12278=CARTESIAN_POINT ( 'NONE',  ( -10.73077095140340376, -23.14408218571897891, -231.4559151628563995 ) ) ;
#12279=CARTESIAN_POINT ( 'NONE',  ( -10.51143808951550085, 11.41308718311005066, -231.3573069600382439 ) ) ;
#12284=CARTESIAN_POINT ( 'NONE',  ( -15.07599795178976443, 12.40109266655585429, -218.9921934537110815 ) ) ;
#12285=CARTESIAN_POINT ( 'NONE',  ( 10.90540179105271967, 5.382827416078996841, -224.1493061458977820 ) ) ;
#12286=CARTESIAN_POINT ( 'NONE',  ( -14.10849459794400751, -0.2436790717799666162, -223.1085195285415921 ) ) ;
#12287=CARTESIAN_POINT ( 'NONE',  ( -30.94549479715584539, -0.2777009447058255143, -220.3105931650466118 ) ) ;
#12289=CARTESIAN_POINT ( 'NONE',  ( -16.30907414568449454, -3.310091733494833655, -231.8954501777161283 ) ) ;
#12290=CARTESIAN_POINT ( 'NONE',  ( -10.59650102373989533, 7.849913810122476576, -230.0486530042683171 ) ) ;
#12291=CARTESIAN_POINT ( 'NONE',  ( -15.48425879135615446, -25.29886615046042309, -220.6886037686364261 ) ) ;
#12292=CARTESIAN_POINT ( 'NONE',  ( 10.85888002857596923, 15.81835858589122878, -232.3913150909872627 ) ) ;
#12293=CARTESIAN_POINT ( 'NONE',  ( 4.210909054564462295, -12.48022235161367988, -220.2789660014272215 ) ) ;
#12294=CARTESIAN_POINT ( 'NONE',  ( 14.87928902430193467, -0.2810696969786992683, -227.9872538617268276 ) ) ;
#12295=CARTESIAN_POINT ( 'NONE',  ( -24.79507334250576278, 6.844873424762779379, -218.1074956078844878 ) ) ;
#12297=CARTESIAN_POINT ( 'NONE',  ( 0.4762409465891800919, 16.20008108839776284, -225.9988706007428050 ) ) ;
#12298=CARTESIAN_POINT ( 'NONE',  ( 22.16968511661519869, 1.542591969257184337, -234.6098499860488573 ) ) ;
#12300=CARTESIAN_POINT ( 'NONE',  ( 21.60524407607017849, 3.028118258437591415, -217.8361640396714449 ) ) ;
#12301=CARTESIAN_POINT ( 'NONE',  ( 12.49127101283658803, 6.474961340449192804, -221.2149164507559078 ) ) ;
#12302=CARTESIAN_POINT ( 'NONE',  ( 7.141633727147962851, -29.98958059360777639, -229.8804610602846594 ) ) ;
#12303=CARTESIAN_POINT ( 'NONE',  ( 14.82579616070250417, 22.96152595385638762, -233.8920860146931489 ) ) ;
#12305=CARTESIAN_POINT ( 'NONE',  ( 0.6837842112036801590, -24.48318360891119028, -216.1006322475167281 ) ) ;
#12306=CARTESIAN_POINT ( 'NONE',  ( -8.611121136347097860, 17.46802294375265419, -231.5575697815534113 ) ) ;
#12307=CARTESIAN_POINT ( 'NONE',  ( 7.450672702945051462, 17.42371045663376705, -217.2894981592719432 ) ) ;
#12309=CARTESIAN_POINT ( 'NONE',  ( -24.76115377241536208, -2.015397159694146456, -231.8500816169410825 ) ) ;
#12310=CARTESIAN_POINT ( 'NONE',  ( -15.50322565568834321, 9.749075856218723857, -229.6019304695566916 ) ) ;
#12312=CARTESIAN_POINT ( 'NONE',  ( -9.578110717394128670, 23.64032677849093034, -215.7669555765890550 ) ) ;
#12313=CARTESIAN_POINT ( 'NONE',  ( 24.32561047128371001, 1.769413244618101011, -218.8629106451077462 ) ) ;
#12315=CARTESIAN_POINT ( 'NONE',  ( 6.726326701167932853, -14.50135447204537087, -224.8733857281379755 ) ) ;
#12317=CARTESIAN_POINT ( 'NONE',  ( 12.75766869239441803, -12.84633107758633663, -232.0853690516983079 ) ) ;
#12318=CARTESIAN_POINT ( 'NONE',  ( -6.208492967940078877, 16.71913201805454463, -230.4912298573936766 ) ) ;
#12320=CARTESIAN_POINT ( 'NONE',  ( 11.87982377808925527, 10.85265283465803421, -229.5027252913499183 ) ) ;
#12321=CARTESIAN_POINT ( 'NONE',  ( 27.92729748684602598, -8.572309054117944527, -222.6487661343338686 ) ) ;
#12322=CARTESIAN_POINT ( 'NONE',  ( -20.76924187596804217, -21.50248317380421170, -228.3679492147379335 ) ) ;
#12323=CARTESIAN_POINT ( 'NONE',  ( -1.177898122437396333, -26.14463525305933445, -216.8677949074964033 ) ) ;
#12324=CARTESIAN_POINT ( 'NONE',  ( -3.389634396460917465, 16.42708991135657115, -221.9057377485790994 ) ) ;
#12326=CARTESIAN_POINT ( 'NONE',  ( 16.23850682336481199, 8.051046992137072422, -219.2473483181185827 ) ) ;
#12327=CARTESIAN_POINT ( 'NONE',  ( -9.740348021262962064, 16.12529029871877384, -216.4361617420699702 ) ) ;
#12328=CARTESIAN_POINT ( 'NONE',  ( -8.791002657293931932, 17.82034842365333205, -218.5247019341474584 ) ) ;
#12330=( BOUNDED_SURFACE ( )  B_SPLINE_SURFACE ( 3, 3, ( 
 ( #7062, #3554, #1657, #5460, #3773, #3443, #7173, #8637, #14038, #18868, #10210, #12120, #5347, #17292, #3327, #8531, #17078, #19195, #15395, #12229, #10323, #10432, #8862, #6834, #22243, #1981, #13702, #1868, #20765, #19081, #5127, #17186, #12008, #8749, #303, #1763, #15611, #75, #6946, #10540, #13817, #20656, #3657, #5239, #15726, #20874, #12342, #13930, #18975, #4004, #21217, #9531, #4227, #17868, #11324, #12684, #10880, #5803, #19855, #13008, #4119, #2756, #17757, #14603, #12576, #4329, #16499, #14489, #2430, #10998, #6028, #12796, #21325, #11212, #14383, #18193, #9313, #16174, #6135, #5919, #2320, #17974, #9206, #4441, #2650, #16069, #639, #7515, #19532, #744, #2538, #7620, #16391, #7950, #9637, #5696, #21544, #19642, #11106, #1076, #9415, #16280, #21111, #19419, #855, #7733, #21438, #969, #18079, #12902, #7843, #19749, #14709, #27, #5081, #10491, #5300, #17357, #12074, #1934, #20490, #16917, #8486, #19970, #6897, #1719, #22084, #10277, #13767, #13881, #19036, #14814, #4557, #7009, #18715, #21659, #3613, #141, #11433, #17033, #20606, #4975, #6250, #3279, #22198, #5192, #11850, #18931, #6674, #13124, #12182, #3506, #18302, #15350, #10164, #20719, #2861, #10054, #1608, #1491, #15455, #11962, #8369, #15239, #13546, #20381, #6786, #13655, #18823, #3395, #17143, #8594, #10385, #17246, #1817, #8695, #15561, #7564, #12739, #5409, #3839, #8924, #17809, #17694, #4173, #16007, #21158, #4061, #17586, #8814, #476, #19472, #14105, #11051, #12517, #9257, #19259, #10606, #13992, #17917, #2152, #19367, #15790, #7350, #5746, #3948, #14432, #16116, #9032, #15677, #15896, #689, #10824, #21265, #2263, #19584, #7125, #5858, #369, #10936, #14216, #5529, #257, #7236, #20828, #20942, #12292, #19144, #12408, #3724, #17475, #9146, #2046, #14326, #10720, #21051, #5641, #583, #7458, #12626, #2374, #8006, #18024, #21827, #6080, #14656, #9801, #9586, #21383, #21599, #7677, #16666, #6307, #5973, #14547, #12850, #19692, #21489, #6190, #11268, #20025, #11595, #14986, #9363, #2916, #16449, #1022, #1247, #14759, #13069, #8121, #6416, #2591, #16222, #797, #4612, #14874, #4278, #21715, #19799, #13286, #9691, #19913, #20128, #4716, #2481, #13182, #11158, #7899, #9474, #18137, #16334, #2812, #4502, #1130, #910, #7790, #16552, #11487, #18354, #12955, #4383, #2703, #11381, #18250, #6761, #9918, #17005, #1696, #22173, #20698, #16782, #5275, #17222, #6986, #20466, #6527, #4949, #8568, #3031, #18469, #10251, #13858, #6646, #1584, #8459, #20578, #1357, #117, #11712, #13631, #12049, #10028, #8671, #15432, #20355 ),
 ( #8230, #3482, #2, #21936, #15100, #13396, #20242, #15211, #15327, #11825, #13742, #4836, #15534, #18583, #18906, #3254, #10138, #10359, #5057, #11934, #1795, #3145, #16891, #1465, #8341, #5167, #6870, #22057, #13516, #18691, #18799, #3369, #17117, #7541, #2350, #14411, #9118, #21243, #17561, #13966, #5503, #17330, #12497, #19234, #10801, #19447, #9235, #3926, #17667, #19344, #5723, #7212, #1907, #19013, #15652, #449, #16095, #8791, #14078, #12266, #21136, #21031, #12156, #2237, #15982, #7435, #20916, #3590, #3814, #559, #17451, #10467, #15871, #12603, #344, #20805, #232, #7102, #12384, #7324, #19119, #10697, #14303, #14194, #17785, #4034, #2130, #5382, #3696, #10581, #666, #10910, #2020, #9007, #5619, #8900, #15766, #2892, #2566, #13155, #6164, #18112, #11028, #9775, #8096, #4256, #4586, #16310, #11462, #12826, #19561, #4358, #11356, #9562, #14963, #4148, #5835, #18331, #16640, #7874, #16200, #14633, #18225, #12713, #17895, #19887, #1221, #886, #11241, #2680, #7981, #2458, #9341, #21357, #999, #21689, #19669, #771, #2785, #7763, #7651, #14522, #9450, #9668, #21465, #6057, #12931, #5949, #21576, #20001, #16424, #19777, #11134, #14736, #13041, #4476, #18002, #16527, #1106, #14846, #6281, #21913, #4810, #18882, #5141, #13715, #13606, #1775, #4694, #20329, #15076, #6738, #13489, #10112, #10336, #22254, #16867, #11569, #5032, #20215, #6502, #11686, #8649, #13373, #15299, #3229, #10224, #18558, #21803, #17200, #22149, #15185, #20443, #8432, #3124, #16978, #11909, #20555, #3457, #6390, #18443, #12023, #10004, #13262, #20106, #6847, #3006, #1443, #18774, #8315, #9889, #22029, #6620, #3341, #4925, #17092, #16755, #11801, #1557, #1333, #8205, #18668, #1670, #8545, #15409, #21006, #5254, #5596, #10557, #19423, #426, #5478, #10885, #5702, #17761, #12477, #2325, #20891, #17306, #8878, #20670, #15850, #321, #14171, #534, #12580, #7301, #19323, #3903, #9094, #17427, #12134, #92, #18990, #3792, #4009, #3569, #1997, #15626, #2212, #2107, #15510, #10778, #17646, #15961, #15742, #6963, #7189, #7411, #20780, #13834, #19211, #14281, #3673, #1882, #10446, #8765, #14055, #10676, #206, #12361, #21115, #17540, #7076, #13945, #8987, #5361, #12245, #19096, #4333, #1080, #12906, #13129, #7520, #7954, #9318, #19860, #14607, #5923, #21664, #749, #14388, #16178, #14819, #6254, #14494, #19974, #5808, #2654, #643, #14714, #4561, #2542, #12800, #21329, #16395, #859, #9421, #21549, #2434, #11437, #19646, #4231, #16502, #16285, #12689, #6032, #21221, #18306, #13014, #19536, #4123, #11004, #17872, #11111, #19753 ),
 ( #7625, #11217, #17979, #9210, #4446, #7737, #21442, #18085, #9535, #974, #7848, #6140, #11328, #16073, #18197, #2760, #9641, #9977, #16838, #17065, #15155, #13461, #1642, #15382, #2979, #9749, #1194, #5005, #8405, #14936, #15272, #20186, #6820, #10085, #21997, #20523, #22229, #5112, #22122, #11994, #8286, #4669, #18528, #8071, #3203, #1414, #1526, #10197, #13686, #16950, #6709, #13580, #18745, #4782, #21776, #16612, #6364, #20301, #2865, #13236, #11657, #9863, #11882, #11776, #20082, #20416, #3312, #8519, #3094, #11542, #6592, #18416, #8180, #16728, #4896, #1305, #13344, #15045, #21886, #6475, #18640, #7160, #3540, #10526, #15822, #14026, #2184, #3872, #12218, #5673, #19070, #10752, #20863, #17618, #291, #509, #17173, #9065, #18963, #7271, #1970, #15599, #15932, #10419, #1750, #17280, #7385, #14253, #1854, #21086, #15485, #12328, #10309, #2078, #18854, #3645, #178, #8732, #3759, #17396, #8848, #8958, #12108, #3429, #7047, #13919, #8624, #58, #5446, #6932, #13803, #20754, #5335, #5567, #19183, #20642, #10644, #398, #14140, #15714, #5227, #17511, #20979, #12445, #19295, #16253, #12982, #720, #14360, #17729, #21631, #5893, #828, #19505, #4203, #9505, #7708, #18170, #19829, #12770, #12551, #19618, #4415, #14577, #11299, #21413, #16476, #10855, #2734, #12659, #943, #17949, #9287, #9614, #4095, #2297, #10971, #1053, #7926, #17841, #14789, #9181, #6003, #3981, #18053, #19398, #11082, #16148, #2406, #19725, #2513, #9391, #2622, #5778, #16044, #7594, #14463, #616, #12875, #7491, #4305, #21193, #21296, #16366, #11187, #7820, #14685, #21519, #6111, #3064, #15018, #1499, #15359, #18723, #13099, #6683, #13317, #20158, #20390, #18503, #16812, #4983, #3288, #6338, #19945, #4534, #8378, #11750, #18279, #18616, #1279, #10172, #13434, #9953, #1617, #17041, #8495, #3177, #6223, #11630, #8040, #21858, #11410, #6562, #4751, #4871, #13555, #2840, #20276, #10061, #16925, #22093, #8153, #9722, #16584, #15247, #18386, #1165, #9836, #1388, #11858, #2949, #14908, #13211, #21748, #20056, #4643, #11516, #6447, #8263, #16698, #15130, #21969, #18939, #7244, #264, #12190, #5089, #3848, #2160, #20614, #20950, #10394, #5538, #6906, #13663, #20728, #5418, #3621, #9040, #20499, #22206, #12416, #10728, #1941, #10286, #8703, #12301, #6795, #11969, #14000, #17593, #17254, #5308, #19045, #2053, #18831, #3405, #15463, #17365, #15798, #13775, #19268, #19154, #1826, #17151, #1728, #3514, #3732, #15569, #149, #7017, #8602, #15686, #14114, #10500, #13891, #36, #8821, #7134, #20836, #5200, #10614, #17485, #12083, #8931 ),
 ( #376, #7877, #4480, #4697, #16643, #11244, #21360, #21693, #14636, #16314, #6060, #18446, #890, #9671, #19891, #4589, #21468, #15906, #11572, #16530, #9565, #7984, #2788, #7766, #11359, #14849, #14966, #20109, #3009, #5952, #8099, #19780, #774, #7654, #1225, #12829, #18116, #9453, #1109, #14739, #18228, #14526, #21806, #2683, #19672, #6284, #12934, #4361, #16427, #4259, #1002, #13158, #20004, #11465, #21579, #11137, #18005, #18334, #6167, #2895, #9778, #13044, #6394, #13265, #2569, #13838, #5258, #21916, #1778, #13495, #12138, #20676, #17204, #15080, #11805, #1675, #22033, #18993, #20333, #16982, #8549, #6624, #15413, #16870, #9894, #96, #17097, #16758, #10117, #4929, #15514, #1337, #6966, #18672, #8653, #10228, #22153, #6506, #8208, #13376, #8319, #20218, #3233, #4814, #1447, #11692, #8435, #22257, #13610, #18562, #3127, #10007, #15189, #1561, #11913, #15305, #6742, #6852, #20447, #5036, #13720, #18779, #3345, #20559, #5146, #12027, #18888, #3462, #10340, #21009, #19428, #17431, #16076, #537, #5481, #9214, #12692, #7193, #9097, #20895, #12364, #19214, #20784, #19327, #17764, #8990, #3796, #5365, #429, #10680, #10782, #7081, #325, #7415, #5812, #8883, #3677, #15747, #646, #7523, #2328, #17650, #3573, #8769, #2111, #15853, #19100, #2215, #17543, #14174, #14392, #4012, #7304, #15631, #15964, #2001, #10561, #14060, #10450, #5599, #3906, #12480, #14284, #21118, #17311, #21224, #5706, #12583, #10888, #1886, #212, #13949, #12249, #18310, #1198, #14940, #9321, #11441, #863, #21781, #8075, #4566, #2437, #21446, #11332, #9425, #6368, #7740, #4336, #18203, #16288, #2764, #4234, #19539, #9752, #4450, #4127, #19756, #14612, #2870, #11008, #16616, #6035, #17875, #19864, #9539, #16181, #752, #7628, #17982, #14498, #12909, #21332, #11114, #5926, #18088, #9645, #977, #12805, #19649, #2544, #11220, #2657, #21553, #16400, #7852, #16507, #14718, #6144, #1084, #13018, #7958, #14823, #21668, #6258, #13133, #19979, #6479, #8409, #6824, #4786, #3433, #10201, #15159, #18858, #63, #16842, #18748, #8291, #22002, #6597, #8183, #6714, #5117, #18644, #13465, #15049, #10089, #20304, #20420, #16731, #9981, #17068, #15488, #18531, #13348, #3099, #10314, #17177, #11999, #5009, #13240, #18419, #20085, #4901, #1647, #1418, #4672, #16954, #13690, #11780, #21890, #2983, #11547, #3207, #1531, #20191, #15277, #8522, #22126, #1753, #20528, #13584, #9866, #11886, #8628, #3318, #1309, #15386, #11661, #22233, #21090, #7051, #17621, #12333, #3647, #19401, #20756, #12111, #13921, #5676, #12554, #12220, #10859, #3544, #401 ),
 ( #16047, #10531, #12447, #1972, #8850, #15717, #1858, #7275, #3984, #19186, #294, #8737, #3762, #7162, #14145, #10422, #17398, #3875, #9184, #19072, #5337, #14029, #17735, #2300, #6937, #20982, #13807, #18967, #5450, #181, #5570, #20865, #17514, #20647, #7388, #10647, #17283, #19298, #2082, #8960, #15824, #5230, #10756, #2187, #9068, #15937, #512, #15603, #14257, #16370, #16257, #14688, #9509, #7599, #18057, #21522, #21634, #4537, #18282, #12663, #14792, #4207, #2843, #11413, #7929, #5784, #2517, #6114, #12774, #9725, #11086, #7712, #12985, #19622, #19832, #14582, #19511, #19729, #4098, #6228, #4420, #10976, #17846, #2410, #9292, #17953, #4309, #9395, #18173, #618, #13102, #7494, #1056, #21417, #6007, #19948, #12879, #11191, #14363, #21196, #724, #16153, #14467, #2737, #11302, #21301, #9617, #833, #5898, #7823, #2628, #947, #16479, #18834, #13557, #11971, #21971, #18389, #9955, #21751, #16927, #1390, #15249, #1619, #13665, #8380, #22096, #1501, #10174, #11634, #6341, #1168, #20059, #4873, #20501, #13214, #18505, #16702, #3290, #3179, #3408, #6685, #20392, #11860, #3067, #16587, #8265, #4985, #21861, #8045, #20278, #17044, #4754, #2953, #4646, #14911, #16814, #11752, #1282, #15132, #18725, #18618, #22208, #8497, #6564, #11519, #13438, #15361, #10063, #6797, #5091, #9841, #8156, #15021, #6450, #13320, #20160, #7021, #486, #1828, #15465, #10396, #9042, #2162, #15571, #14229, #6908, #3734, #1730, #15800, #5652, #3623, #13893, #151, #17487, #1943, #10502, #378, #3516, #7360, #20730, #5310, #17595, #12192, #7246, #12529, #19048, #17256, #17367, #21064, #15908, #19377, #2055, #10288, #38, #8823, #8705, #8933, #15688, #20838, #17153, #10730, #266, #13777, #14117, #7136, #14002, #5421, #8604, #12303, #10618, #19156, #20952, #5540, #20617, #5202, #12420, #19271, #3850, #12085, #18941, #21393, #2603, #2714, #7908, #21610, #16019, #18147, #7575, #6202, #14771, #11278, #9156, #5867, #18034, #16126, #13079, #14441, #11060, #9484, #699, #16345, #10947, #3958, #16459, #11167, #10833, #4184, #21276, #9596, #17706, #1034, #12748, #2272, #4288, #16232, #594, #7467, #14336, #2384, #21169, #19597, #5756, #17821, #12636, #2492, #921, #7687, #19484, #4071, #9268, #17929, #9372, #5985, #808, #14556, #7801, #12859, #19703, #14666, #21500, #6090, #12965, #19809, #4394, #18259, #1595, #13191, #15111, #13531, #11497, #10151, #16903, #21837, #3267, #6774, #1256, #3158, #14998, #6427, #13297, #14883, #13411, #11839, #3042, #20138, #21724, #16792, #4729, #4849, #1142, #2926, #22186, #1367, #20369, #8132 ),
 ( #18704, #11608, #17020, #4623, #11391, #18480, #10042, #8243, #19923, #2823, #4511, #8472, #15339, #21948, #8019, #9930, #1479, #9703, #16563, #11727, #6317, #6540, #20253, #18595, #22070, #20035, #18366, #9814, #8355, #4960, #16676, #15226, #6660, #15548, #19245, #460, #17234, #19129, #8682, #127, #6995, #8580, #7111, #5515, #19022, #13867, #15444, #10476, #20708, #20815, #17130, #10370, #10592, #15882, #18918, #13753, #3494, #10707, #3825, #12394, #5392, #13643, #18810, #12166, #6884, #12277, #5286, #1919, #2140, #14088, #3600, #3381, #3709, #12060, #20592, #1805, #20479, #5178, #13975, #17341, #2031, #8800, #5070, #9017, #17461, #15661, #8910, #242, #15776, #355, #7223, #17571, #11946, #10262, #1706, #14, #20928, #2690, #18123, #14644, #12507, #9244, #21367, #19457, #16434, #10922, #14419, #5959, #4045, #12836, #14313, #7337, #19786, #14533, #21040, #5844, #19680, #11038, #9572, #5630, #14204, #6069, #19354, #9350, #17678, #16104, #4266, #3936, #10811, #11144, #2250, #17794, #12723, #19570, #9461, #9130, #11253, #569, #2468, #897, #21145, #4369, #18012, #676, #12941, #15993, #2360, #2578, #7551, #21252, #4157, #7445, #782, #21475, #17904, #16210, #5733, #7663, #16321, #7774, #12612, #1117, #6403, #15088, #9679, #18236, #16538, #1345, #9903, #3018, #8107, #21924, #14746, #20011, #11367, #1233, #13166, #18341, #8216, #18455, #7993, #21587, #21814, #2796, #14858, #21701, #1009, #6292, #14973, #2902, #20115, #4597, #7884, #6176, #13273, #11473, #4704, #11581, #9787, #16766, #13055, #19900, #4488, #16652, #9440, #990, #2341, #658, #7754, #1096, #16088, #14514, #19553, #6155, #6047, #14837, #4348, #9553, #14729, #5940, #19440, #11126, #7864, #2450, #21680, #878, #19879, #7641, #21235, #9227, #6271, #12818, #14626, #4141, #17994, #16415, #21458, #2776, #4465, #19661, #4026, #16518, #11232, #18103, #19768, #2557, #16302, #21566, #7535, #14404, #12922, #7969, #5827, #21346, #11020, #13031, #2670, #10903, #11345, #18216, #9659, #4246, #17777, #12706, #17887, #9333, #16193, #765, #13597, #1325, #14955, #18323, #22246, #6492, #1433, #20097, #4801, #10103, #8306, #18762, #20434, #13362, #13146, #20206, #5023, #15173, #11899, #16857, #17082, #11454, #3331, #13252, #1545, #18548, #9881, #10214, #4686, #2883, #11559, #1660, #8535, #18434, #15399, #9764, #6611, #4578, #18660, #19991, #11677, #16745, #2997, #20319, #3115, #9995, #3220, #6380, #16630, #8196, #15064, #1213, #22018, #8088, #13480, #21794, #21904, #16967, #4917, #11793, #8423, #15290, #22139, #6729, #15615, #2095, #15949, #19312 ),
 ( #20769, #17416, #17634, #7289, #1871, #12014, #12349, #5242, #6951, #18979, #9082, #13823, #308, #10546, #17528, #12123, #6838, #2201, #7179, #195, #20880, #15731, #20660, #1986, #5586, #13706, #8866, #17189, #7065, #19201, #20543, #5130, #5466, #18872, #17296, #12234, #19085, #8975, #3446, #10768, #80, #14044, #415, #3558, #3890, #3781, #8754, #12466, #10327, #10436, #10663, #13934, #5351, #3661, #1766, #15839, #20996, #14160, #8640, #15501, #19635, #737, #7725, #3997, #19525, #19742, #2749, #5796, #633, #12677, #19847, #6127, #14702, #14596, #9630, #5689, #21315, #16063, #21431, #14481, #11099, #11316, #962, #17860, #12568, #6021, #21210, #7509, #4112, #524, #14376, #16272, #4219, #11205, #10991, #7402, #18186, #847, #16167, #12894, #9408, #2423, #17967, #4322, #21536, #4434, #19413, #9306, #7613, #5912, #14272, #21104, #7836, #10873, #12789, #18071, #2531, #17749, #2643, #9523, #16383, #13001, #2313, #9198, #16492, #6697, #1403, #11870, #16717, #11531, #22110, #4994, #13569, #13225, #1515, #16825, #6464, #21650, #20405, #18734, #14924, #15261, #4658, #3300, #1181, #7943, #15034, #21986, #20175, #1069, #14807, #6243, #20290, #13117, #19963, #4769, #4550, #11426, #18404, #16600, #3191, #3083, #18295, #8275, #6579, #11765, #2966, #2854, #8168, #4885, #21764, #9738, #11645, #16939, #9852, #8059, #6353, #20071, #1294, #18516, #21875, #13333, #13449, #9966, #15144, #8393, #18629, #10074, #3526, #2370, #5321, #9252, #13905, #14428, #8508, #16112, #10298, #21154, #15584, #6920, #685, #1739, #15371, #17162, #7559, #21261, #15474, #5852, #6809, #3944, #1630, #16003, #12735, #10405, #13789, #47, #17689, #1839, #17267, #578, #3418, #19579, #20627, #5213, #17803, #8717, #13675, #7032, #22218, #10184, #14321, #20512, #5102, #11982, #18843, #12095, #20740, #18950, #5742, #17053, #8613, #162, #10932, #12202, #19363, #10820, #2258, #9141, #7453, #12621, #19466, #4055, #2477, #6301, #9686, #16218, #16546, #21483, #8116, #11376, #16443, #21821, #16659, #6411, #1124, #13281, #9580, #5969, #19794, #9358, #4497, #11261, #19688, #21594, #2806, #2910, #14981, #792, #18019, #4167, #11046, #2586, #9795, #14651, #1242, #11153, #17912, #2698, #8001, #7892, #7671, #14542, #21378, #12845, #4274, #6185, #9468, #12950, #14866, #16329, #905, #18244, #7785, #6076, #1016, #14753, #13174, #4377, #18131, #13062, #19908, #20019, #21709, #4606, #11481, #18348, #3476, #6980, #1460, #3363, #15206, #22051, #6641, #15095, #13626, #12043, #3248, #13511, #21932, #17000, #20349, #5052, #1352, #16885, #17112, #112 ) ),
 .UNSPECIFIED., .T., .F., .F. ) 
 B_SPLINE_SURFACE_WITH_KNOTS ( ( 4, 3, 4 ),
 ( 4, 2, 2, 2, 2, 2, 2, 2, 2, 2, 2, 2, 2, 2, 2, 2, 2, 2, 2, 2, 2, 2, 2, 2, 2, 2, 2, 2, 2, 2, 2, 2, 2, 2, 2, 2, 2, 2, 2, 2, 2, 2, 2, 2, 2, 2, 2, 2, 2, 2, 2, 2, 2, 2, 2, 2, 2, 2, 2, 2, 2, 2, 2, 2, 2, 2, 2, 2, 2, 2, 2, 2, 2, 2, 2, 2, 2, 2, 2, 2, 2, 2, 2, 2, 2, 2, 2, 2, 2, 2, 2, 2, 2, 2, 2, 2, 2, 2, 2, 2, 2, 2, 2, 2, 2, 2, 2, 2, 2, 2, 2, 2, 2, 2, 2, 2, 2, 2, 2, 2, 2, 2, 2, 2, 2, 2, 2, 2, 2, 2, 2, 2, 2, 2, 2, 2, 2, 2, 2, 2, 2, 2, 2, 2, 2, 2, 2, 2, 2, 2, 2, 2, 2, 2, 2, 2, 2, 2, 2, 2, 2, 2, 2, 2, 2, 2, 2, 4 ),
 ( 0.000000000000000000, 0.5000000000000000000, 1.000000000000000000 ),
 ( 0.000000000000000000, 0.001952908952989333875, 0.003905817905978667751, 0.007323408573709997045, 0.01074099924144132634, 0.01415858990917265650, 0.01586738524303832332, 0.01757618057690398666, 0.02099377124463531682, 0.02441136191236664699, 0.02782895258009797368, 0.03124654324782930384, 0.03466413391556063400, 0.03808172458329196070, 0.04149931525102329433, 0.04491690591875462102, 0.04662570125262028436, 0.04833449658648594771, 0.05175208725421727440, 0.05346088258808293775, 0.05516967792194860110, 0.05858726858967993473, 0.06200485925741126836, 0.06542244992514259505, 0.06884004059287393562, 0.07225763126060526231, 0.07567522192833658901, 0.07909281259606792958, 0.08251040326379925627, 0.08421919859766491268, 0.08592799393153058296, 0.08934558459926195129, 0.09276317526699331961, 0.09447197060085900377, 0.09618076593472468794, 0.09959835660245604239, 0.1030159472701873968, 0.1064335379379187652, 0.1098511286056501335, 0.1132687192733815018, 0.1166863099411127869, 0.1201039006088440858, 0.1235214912765753847, 0.1252302866104410273, 0.1269390819443066698, 0.1303566726120379826, 0.1320654679459036251, 0.1337742632797692677, 0.1371918539475005527, 0.1406094446152318378, 0.1440270352829631784, 0.1474446259506944912, 0.1508622166184258040, 0.1542798072861571446, 0.1576973979538884851, 0.1611149886216198257, 0.1645325792893511663, 0.1679501699570824791, 0.1713677606248137919, 0.1747853512925451325, 0.1764941466264108028, 0.1782029419602764730, 0.1816205326280078136, 0.1850381232957391542, 0.1884557139634704670, 0.1918733046312017798, 0.1952908952989331204, 0.1987084859666644610, 0.2021260766343957738, 0.2055436673021270866, 0.2072524626359927569, 0.2089612579698584272, 0.2123788486375897677, 0.2140876439714554380, 0.2157964393053211083, 0.2192140299730524489, 0.2226316206407837617, 0.2260492113085151300, 0.2294668019762464706, 0.2328843926439778111, 0.2363019833117091517, 0.2397195739794404923, 0.2431371646471718329, 0.2465547553149031734, 0.2499723459826345140, 0.2533899366503657991, 0.2568075273180971396, 0.2602251179858284802, 0.2636427086535597653, 0.2670602993212910503, 0.2704778899890223909, 0.2738954806567537315, 0.2773130713244850165, 0.2807306619922163571, 0.2841482526599476977, 0.2858570479938133957, 0.2875658433276790382, 0.2909834339954103788, 0.2926922293292760768, 0.2944010246631417194, 0.2978186153308730599, 0.3012362059986043450, 0.3046537966663356856, 0.3080713873340670261, 0.3114889780017983112, 0.3149065686695296518, 0.3183241593372609923, 0.3217417500049923329, 0.3234505453388579754, 0.3251593406727236735, 0.3285769313404549585, 0.3319945220081862991, 0.3354121126759176397, 0.3388297033436489247, 0.3422472940113802653, 0.3456648846791116059, 0.3490824753468429464, 0.3525000660145742870, 0.3559176566823056276, 0.3593352473500369682, 0.3627528380177683087, 0.3661704286854996493, 0.3695880193532309343, 0.3730056100209622749, 0.3747144053548279174, 0.3764232006886936155, 0.3798407913564249005, 0.3832583820241562411, 0.3866759726918875817, 0.3900935633596189223, 0.3935111540273502628, 0.3969287446950816034, 0.4003463353628129440, 0.4037639260305442845, 0.4054727213644099271, 0.4071815166982756251, 0.4105991073660069102, 0.4140166980337382507, 0.4157254933676038933, 0.4174342887014695913, 0.4208518793692008764, 0.4242694700369322169, 0.4276870607046635575, 0.4311046513723948981, 0.4345222420401262386, 0.4379398327078575237, 0.4413574233755888643, 0.4447750140433202048, 0.4464838093771859029, 0.4481926047110515454, 0.4516101953787828860, 0.4533189907126485840, 0.4550277860465142266, 0.4584453767142455671, 0.4618629673819769077, 0.4652805580497082483, 0.4686981487174395888, 0.4721157393851709294, 0.4755333300529022145, 0.4789509207206335550, 0.4823685113883648956, 0.4840773067222305381, 0.4857861020560961807, 0.4892036927238275212, 0.4926212833915588618, 0.4960388740592901469, 0.4979917830122794764, 0.4999446919652688059 ),
 .UNSPECIFIED. ) 
 GEOMETRIC_REPRESENTATION_ITEM ( )  RATIONAL_B_SPLINE_SURFACE ( (
 ( 1.000000000000000000, 1.000000000000000000, 1.000000000000000000, 1.000000000000000000, 1.000000000000000000, 1.000000000000000000, 1.000000000000000000, 1.000000000000000000, 1.000000000000000000, 1.000000000000000000, 1.000000000000000000, 1.000000000000000000, 1.000000000000000000, 1.000000000000000000, 1.000000000000000000, 1.000000000000000000, 1.000000000000000000, 1.000000000000000000, 1.000000000000000000, 1.000000000000000000, 1.000000000000000000, 1.000000000000000000, 1.000000000000000000, 1.000000000000000000, 1.000000000000000000, 1.000000000000000000, 1.000000000000000000, 1.000000000000000000, 1.000000000000000000, 1.000000000000000000, 1.000000000000000000, 1.000000000000000000, 1.000000000000000000, 1.000000000000000000, 1.000000000000000000, 1.000000000000000000, 1.000000000000000000, 1.000000000000000000, 1.000000000000000000, 1.000000000000000000, 1.000000000000000000, 1.000000000000000000, 1.000000000000000000, 1.000000000000000000, 1.000000000000000000, 1.000000000000000000, 1.000000000000000000, 1.000000000000000000, 1.000000000000000000, 1.000000000000000000, 1.000000000000000000, 1.000000000000000000, 1.000000000000000000, 1.000000000000000000, 1.000000000000000000, 1.000000000000000000, 1.000000000000000000, 1.000000000000000000, 1.000000000000000000, 1.000000000000000000, 1.000000000000000000, 1.000000000000000000, 1.000000000000000000, 1.000000000000000000, 1.000000000000000000, 1.000000000000000000, 1.000000000000000000, 1.000000000000000000, 1.000000000000000000, 1.000000000000000000, 1.000000000000000000, 1.000000000000000000, 1.000000000000000000, 1.000000000000000000, 1.000000000000000000, 1.000000000000000000, 1.000000000000000000, 1.000000000000000000, 1.000000000000000000, 1.000000000000000000, 1.000000000000000000, 1.000000000000000000, 1.000000000000000000, 1.000000000000000000, 1.000000000000000000, 1.000000000000000000, 1.000000000000000000, 1.000000000000000000, 1.000000000000000000, 1.000000000000000000, 1.000000000000000000, 1.000000000000000000, 1.000000000000000000, 1.000000000000000000, 1.000000000000000000, 1.000000000000000000, 1.000000000000000000, 1.000000000000000000, 1.000000000000000000, 1.000000000000000000, 1.000000000000000000, 1.000000000000000000, 1.000000000000000000, 1.000000000000000000, 1.000000000000000000, 1.000000000000000000, 1.000000000000000000, 1.000000000000000000, 1.000000000000000000, 1.000000000000000000, 1.000000000000000000, 1.000000000000000000, 1.000000000000000000, 1.000000000000000000, 1.000000000000000000, 1.000000000000000000, 1.000000000000000000, 1.000000000000000000, 1.000000000000000000, 1.000000000000000000, 1.000000000000000000, 1.000000000000000000, 1.000000000000000000, 1.000000000000000000, 1.000000000000000000, 1.000000000000000000, 1.000000000000000000, 1.000000000000000000, 1.000000000000000000, 1.000000000000000000, 1.000000000000000000, 1.000000000000000000, 1.000000000000000000, 1.000000000000000000, 1.000000000000000000, 1.000000000000000000, 1.000000000000000000, 1.000000000000000000, 1.000000000000000000, 1.000000000000000000, 1.000000000000000000, 1.000000000000000000, 1.000000000000000000, 1.000000000000000000, 1.000000000000000000, 1.000000000000000000, 1.000000000000000000, 1.000000000000000000, 1.000000000000000000, 1.000000000000000000, 1.000000000000000000, 1.000000000000000000, 1.000000000000000000, 1.000000000000000000, 1.000000000000000000, 1.000000000000000000, 1.000000000000000000, 1.000000000000000000, 1.000000000000000000, 1.000000000000000000, 1.000000000000000000, 1.000000000000000000, 1.000000000000000000, 1.000000000000000000, 1.000000000000000000, 1.000000000000000000, 1.000000000000000000, 1.000000000000000000, 1.000000000000000000, 1.000000000000000000, 1.000000000000000000, 1.000000000000000000, 1.000000000000000000, 1.000000000000000000, 1.000000000000000000, 1.000000000000000000, 1.000000000000000000, 1.000000000000000000, 1.000000000000000000, 1.000000000000000000, 1.000000000000000000, 1.000000000000000000, 1.000000000000000000, 1.000000000000000000, 1.000000000000000000, 1.000000000000000000, 1.000000000000000000, 1.000000000000000000, 1.000000000000000000, 1.000000000000000000, 1.000000000000000000, 1.000000000000000000, 1.000000000000000000, 1.000000000000000000, 1.000000000000000000, 1.000000000000000000, 1.000000000000000000, 1.000000000000000000, 1.000000000000000000, 1.000000000000000000, 1.000000000000000000, 1.000000000000000000, 1.000000000000000000, 1.000000000000000000, 1.000000000000000000, 1.000000000000000000, 1.000000000000000000, 1.000000000000000000, 1.000000000000000000, 1.000000000000000000, 1.000000000000000000, 1.000000000000000000, 1.000000000000000000, 1.000000000000000000, 1.000000000000000000, 1.000000000000000000, 1.000000000000000000, 1.000000000000000000, 1.000000000000000000, 1.000000000000000000, 1.000000000000000000, 1.000000000000000000, 1.000000000000000000, 1.000000000000000000, 1.000000000000000000, 1.000000000000000000, 1.000000000000000000, 1.000000000000000000, 1.000000000000000000, 1.000000000000000000, 1.000000000000000000, 1.000000000000000000, 1.000000000000000000, 1.000000000000000000, 1.000000000000000000, 1.000000000000000000, 1.000000000000000000, 1.000000000000000000, 1.000000000000000000, 1.000000000000000000, 1.000000000000000000, 1.000000000000000000, 1.000000000000000000, 1.000000000000000000, 1.000000000000000000, 1.000000000000000000, 1.000000000000000000, 1.000000000000000000, 1.000000000000000000, 1.000000000000000000, 1.000000000000000000, 1.000000000000000000, 1.000000000000000000, 1.000000000000000000, 1.000000000000000000, 1.000000000000000000, 1.000000000000000000, 1.000000000000000000, 1.000000000000000000, 1.000000000000000000, 1.000000000000000000, 1.000000000000000000, 1.000000000000000000, 1.000000000000000000, 1.000000000000000000, 1.000000000000000000, 1.000000000000000000, 1.000000000000000000, 1.000000000000000000, 1.000000000000000000, 1.000000000000000000, 1.000000000000000000, 1.000000000000000000, 1.000000000000000000, 1.000000000000000000, 1.000000000000000000, 1.000000000000000000, 1.000000000000000000, 1.000000000000000000, 1.000000000000000000, 1.000000000000000000, 1.000000000000000000, 1.000000000000000000, 1.000000000000000000, 1.000000000000000000, 1.000000000000000000, 1.000000000000000000, 1.000000000000000000, 1.000000000000000000, 1.000000000000000000, 1.000000000000000000, 1.000000000000000000, 1.000000000000000000, 1.000000000000000000, 1.000000000000000000, 1.000000000000000000, 1.000000000000000000, 1.000000000000000000, 1.000000000000000000, 1.000000000000000000, 1.000000000000000000, 1.000000000000000000, 1.000000000000000000, 1.000000000000000000, 1.000000000000000000, 1.000000000000000000, 1.000000000000000000, 1.000000000000000000, 1.000000000000000000, 1.000000000000000000, 1.000000000000000000, 1.000000000000000000, 1.000000000000000000, 1.000000000000000000, 1.000000000000000000, 1.000000000000000000, 1.000000000000000000, 1.000000000000000000, 1.000000000000000000, 1.000000000000000000, 1.000000000000000000, 1.000000000000000000, 1.000000000000000000, 1.000000000000000000, 1.000000000000000000, 1.000000000000000000, 1.000000000000000000, 1.000000000000000000, 1.000000000000000000, 1.000000000000000000, 1.000000000000000000, 1.000000000000000000, 1.000000000000000000, 1.000000000000000000, 1.000000000000000000, 1.000000000000000000),
 ( 0.3333333333333333703, 0.3333333333333333703, 0.3333333333333333703, 0.3333333333333333703, 0.3333333333333333703, 0.3333333333333333703, 0.3333333333333333703, 0.3333333333333333703, 0.3333333333333333703, 0.3333333333333333703, 0.3333333333333333703, 0.3333333333333333703, 0.3333333333333333703, 0.3333333333333333703, 0.3333333333333333703, 0.3333333333333333703, 0.3333333333333333703, 0.3333333333333333703, 0.3333333333333333703, 0.3333333333333333703, 0.3333333333333333703, 0.3333333333333333703, 0.3333333333333333703, 0.3333333333333333703, 0.3333333333333333703, 0.3333333333333333703, 0.3333333333333333703, 0.3333333333333333703, 0.3333333333333333703, 0.3333333333333333703, 0.3333333333333333703, 0.3333333333333333703, 0.3333333333333333703, 0.3333333333333333703, 0.3333333333333333703, 0.3333333333333333703, 0.3333333333333333703, 0.3333333333333333703, 0.3333333333333333703, 0.3333333333333333703, 0.3333333333333333703, 0.3333333333333333703, 0.3333333333333333703, 0.3333333333333333703, 0.3333333333333333703, 0.3333333333333333703, 0.3333333333333333703, 0.3333333333333333703, 0.3333333333333333703, 0.3333333333333333703, 0.3333333333333333703, 0.3333333333333333703, 0.3333333333333333703, 0.3333333333333333703, 0.3333333333333333703, 0.3333333333333333703, 0.3333333333333333703, 0.3333333333333333703, 0.3333333333333333703, 0.3333333333333333703, 0.3333333333333333703, 0.3333333333333333703, 0.3333333333333333703, 0.3333333333333333703, 0.3333333333333333703, 0.3333333333333333703, 0.3333333333333333703, 0.3333333333333333703, 0.3333333333333333703, 0.3333333333333333703, 0.3333333333333333703, 0.3333333333333333703, 0.3333333333333333703, 0.3333333333333333703, 0.3333333333333333703, 0.3333333333333333703, 0.3333333333333333703, 0.3333333333333333703, 0.3333333333333333703, 0.3333333333333333703, 0.3333333333333333703, 0.3333333333333333703, 0.3333333333333333703, 0.3333333333333333703, 0.3333333333333333703, 0.3333333333333333703, 0.3333333333333333703, 0.3333333333333333703, 0.3333333333333333703, 0.3333333333333333703, 0.3333333333333333703, 0.3333333333333333703, 0.3333333333333333703, 0.3333333333333333703, 0.3333333333333333703, 0.3333333333333333703, 0.3333333333333333703, 0.3333333333333333703, 0.3333333333333333703, 0.3333333333333333703, 0.3333333333333333703, 0.3333333333333333703, 0.3333333333333333703, 0.3333333333333333703, 0.3333333333333333703, 0.3333333333333333703, 0.3333333333333333703, 0.3333333333333333703, 0.3333333333333333703, 0.3333333333333333703, 0.3333333333333333703, 0.3333333333333333703, 0.3333333333333333703, 0.3333333333333333703, 0.3333333333333333703, 0.3333333333333333703, 0.3333333333333333703, 0.3333333333333333703, 0.3333333333333333703, 0.3333333333333333703, 0.3333333333333333703, 0.3333333333333333703, 0.3333333333333333703, 0.3333333333333333703, 0.3333333333333333703, 0.3333333333333333703, 0.3333333333333333703, 0.3333333333333333703, 0.3333333333333333703, 0.3333333333333333703, 0.3333333333333333703, 0.3333333333333333703, 0.3333333333333333703, 0.3333333333333333703, 0.3333333333333333703, 0.3333333333333333703, 0.3333333333333333703, 0.3333333333333333703, 0.3333333333333333703, 0.3333333333333333703, 0.3333333333333333703, 0.3333333333333333703, 0.3333333333333333703, 0.3333333333333333703, 0.3333333333333333703, 0.3333333333333333703, 0.3333333333333333703, 0.3333333333333333703, 0.3333333333333333703, 0.3333333333333333703, 0.3333333333333333703, 0.3333333333333333703, 0.3333333333333333703, 0.3333333333333333703, 0.3333333333333333703, 0.3333333333333333703, 0.3333333333333333703, 0.3333333333333333703, 0.3333333333333333703, 0.3333333333333333703, 0.3333333333333333703, 0.3333333333333333703, 0.3333333333333333703, 0.3333333333333333703, 0.3333333333333333703, 0.3333333333333333703, 0.3333333333333333703, 0.3333333333333333703, 0.3333333333333333703, 0.3333333333333333703, 0.3333333333333333703, 0.3333333333333333703, 0.3333333333333333703, 0.3333333333333333703, 0.3333333333333333703, 0.3333333333333333703, 0.3333333333333333703, 0.3333333333333333703, 0.3333333333333333703, 0.3333333333333333703, 0.3333333333333333703, 0.3333333333333333703, 0.3333333333333333703, 0.3333333333333333703, 0.3333333333333333703, 0.3333333333333333703, 0.3333333333333333703, 0.3333333333333333703, 0.3333333333333333703, 0.3333333333333333703, 0.3333333333333333703, 0.3333333333333333703, 0.3333333333333333703, 0.3333333333333333703, 0.3333333333333333703, 0.3333333333333333703, 0.3333333333333333703, 0.3333333333333333703, 0.3333333333333333703, 0.3333333333333333703, 0.3333333333333333703, 0.3333333333333333703, 0.3333333333333333703, 0.3333333333333333703, 0.3333333333333333703, 0.3333333333333333703, 0.3333333333333333703, 0.3333333333333333703, 0.3333333333333333703, 0.3333333333333333703, 0.3333333333333333703, 0.3333333333333333703, 0.3333333333333333703, 0.3333333333333333703, 0.3333333333333333703, 0.3333333333333333703, 0.3333333333333333703, 0.3333333333333333703, 0.3333333333333333703, 0.3333333333333333703, 0.3333333333333333703, 0.3333333333333333703, 0.3333333333333333703, 0.3333333333333333703, 0.3333333333333333703, 0.3333333333333333703, 0.3333333333333333703, 0.3333333333333333703, 0.3333333333333333703, 0.3333333333333333703, 0.3333333333333333703, 0.3333333333333333703, 0.3333333333333333703, 0.3333333333333333703, 0.3333333333333333703, 0.3333333333333333703, 0.3333333333333333703, 0.3333333333333333703, 0.3333333333333333703, 0.3333333333333333703, 0.3333333333333333703, 0.3333333333333333703, 0.3333333333333333703, 0.3333333333333333703, 0.3333333333333333703, 0.3333333333333333703, 0.3333333333333333703, 0.3333333333333333703, 0.3333333333333333703, 0.3333333333333333703, 0.3333333333333333703, 0.3333333333333333703, 0.3333333333333333703, 0.3333333333333333703, 0.3333333333333333703, 0.3333333333333333703, 0.3333333333333333703, 0.3333333333333333703, 0.3333333333333333703, 0.3333333333333333703, 0.3333333333333333703, 0.3333333333333333703, 0.3333333333333333703, 0.3333333333333333703, 0.3333333333333333703, 0.3333333333333333703, 0.3333333333333333703, 0.3333333333333333703, 0.3333333333333333703, 0.3333333333333333703, 0.3333333333333333703, 0.3333333333333333703, 0.3333333333333333703, 0.3333333333333333703, 0.3333333333333333703, 0.3333333333333333703, 0.3333333333333333703, 0.3333333333333333703, 0.3333333333333333703, 0.3333333333333333703, 0.3333333333333333703, 0.3333333333333333703, 0.3333333333333333703, 0.3333333333333333703, 0.3333333333333333703, 0.3333333333333333703, 0.3333333333333333703, 0.3333333333333333703, 0.3333333333333333703, 0.3333333333333333703, 0.3333333333333333703, 0.3333333333333333703, 0.3333333333333333703, 0.3333333333333333703, 0.3333333333333333703, 0.3333333333333333703, 0.3333333333333333703, 0.3333333333333333703, 0.3333333333333333703, 0.3333333333333333703, 0.3333333333333333703, 0.3333333333333333703, 0.3333333333333333703, 0.3333333333333333703, 0.3333333333333333703, 0.3333333333333333703, 0.3333333333333333703, 0.3333333333333333703, 0.3333333333333333703, 0.3333333333333333703, 0.3333333333333333703, 0.3333333333333333703, 0.3333333333333333703, 0.3333333333333333703, 0.3333333333333333703, 0.3333333333333333703, 0.3333333333333333703, 0.3333333333333333703, 0.3333333333333333703, 0.3333333333333333703, 0.3333333333333333703, 0.3333333333333333703, 0.3333333333333333703, 0.3333333333333333703, 0.3333333333333333703, 0.3333333333333333703, 0.3333333333333333703, 0.3333333333333333703, 0.3333333333333333703, 0.3333333333333333703, 0.3333333333333333703, 0.3333333333333333703, 0.3333333333333333703, 0.3333333333333333703, 0.3333333333333333703, 0.3333333333333333703),
 ( 0.3333333333333333703, 0.3333333333333333703, 0.3333333333333333703, 0.3333333333333333703, 0.3333333333333333703, 0.3333333333333333703, 0.3333333333333333703, 0.3333333333333333703, 0.3333333333333333703, 0.3333333333333333703, 0.3333333333333333703, 0.3333333333333333703, 0.3333333333333333703, 0.3333333333333333703, 0.3333333333333333703, 0.3333333333333333703, 0.3333333333333333703, 0.3333333333333333703, 0.3333333333333333703, 0.3333333333333333703, 0.3333333333333333703, 0.3333333333333333703, 0.3333333333333333703, 0.3333333333333333703, 0.3333333333333333703, 0.3333333333333333703, 0.3333333333333333703, 0.3333333333333333703, 0.3333333333333333703, 0.3333333333333333703, 0.3333333333333333703, 0.3333333333333333703, 0.3333333333333333703, 0.3333333333333333703, 0.3333333333333333703, 0.3333333333333333703, 0.3333333333333333703, 0.3333333333333333703, 0.3333333333333333703, 0.3333333333333333703, 0.3333333333333333703, 0.3333333333333333703, 0.3333333333333333703, 0.3333333333333333703, 0.3333333333333333703, 0.3333333333333333703, 0.3333333333333333703, 0.3333333333333333703, 0.3333333333333333703, 0.3333333333333333703, 0.3333333333333333703, 0.3333333333333333703, 0.3333333333333333703, 0.3333333333333333703, 0.3333333333333333703, 0.3333333333333333703, 0.3333333333333333703, 0.3333333333333333703, 0.3333333333333333703, 0.3333333333333333703, 0.3333333333333333703, 0.3333333333333333703, 0.3333333333333333703, 0.3333333333333333703, 0.3333333333333333703, 0.3333333333333333703, 0.3333333333333333703, 0.3333333333333333703, 0.3333333333333333703, 0.3333333333333333703, 0.3333333333333333703, 0.3333333333333333703, 0.3333333333333333703, 0.3333333333333333703, 0.3333333333333333703, 0.3333333333333333703, 0.3333333333333333703, 0.3333333333333333703, 0.3333333333333333703, 0.3333333333333333703, 0.3333333333333333703, 0.3333333333333333703, 0.3333333333333333703, 0.3333333333333333703, 0.3333333333333333703, 0.3333333333333333703, 0.3333333333333333703, 0.3333333333333333703, 0.3333333333333333703, 0.3333333333333333703, 0.3333333333333333703, 0.3333333333333333703, 0.3333333333333333703, 0.3333333333333333703, 0.3333333333333333703, 0.3333333333333333703, 0.3333333333333333703, 0.3333333333333333703, 0.3333333333333333703, 0.3333333333333333703, 0.3333333333333333703, 0.3333333333333333703, 0.3333333333333333703, 0.3333333333333333703, 0.3333333333333333703, 0.3333333333333333703, 0.3333333333333333703, 0.3333333333333333703, 0.3333333333333333703, 0.3333333333333333703, 0.3333333333333333703, 0.3333333333333333703, 0.3333333333333333703, 0.3333333333333333703, 0.3333333333333333703, 0.3333333333333333703, 0.3333333333333333703, 0.3333333333333333703, 0.3333333333333333703, 0.3333333333333333703, 0.3333333333333333703, 0.3333333333333333703, 0.3333333333333333703, 0.3333333333333333703, 0.3333333333333333703, 0.3333333333333333703, 0.3333333333333333703, 0.3333333333333333703, 0.3333333333333333703, 0.3333333333333333703, 0.3333333333333333703, 0.3333333333333333703, 0.3333333333333333703, 0.3333333333333333703, 0.3333333333333333703, 0.3333333333333333703, 0.3333333333333333703, 0.3333333333333333703, 0.3333333333333333703, 0.3333333333333333703, 0.3333333333333333703, 0.3333333333333333703, 0.3333333333333333703, 0.3333333333333333703, 0.3333333333333333703, 0.3333333333333333703, 0.3333333333333333703, 0.3333333333333333703, 0.3333333333333333703, 0.3333333333333333703, 0.3333333333333333703, 0.3333333333333333703, 0.3333333333333333703, 0.3333333333333333703, 0.3333333333333333703, 0.3333333333333333703, 0.3333333333333333703, 0.3333333333333333703, 0.3333333333333333703, 0.3333333333333333703, 0.3333333333333333703, 0.3333333333333333703, 0.3333333333333333703, 0.3333333333333333703, 0.3333333333333333703, 0.3333333333333333703, 0.3333333333333333703, 0.3333333333333333703, 0.3333333333333333703, 0.3333333333333333703, 0.3333333333333333703, 0.3333333333333333703, 0.3333333333333333703, 0.3333333333333333703, 0.3333333333333333703, 0.3333333333333333703, 0.3333333333333333703, 0.3333333333333333703, 0.3333333333333333703, 0.3333333333333333703, 0.3333333333333333703, 0.3333333333333333703, 0.3333333333333333703, 0.3333333333333333703, 0.3333333333333333703, 0.3333333333333333703, 0.3333333333333333703, 0.3333333333333333703, 0.3333333333333333703, 0.3333333333333333703, 0.3333333333333333703, 0.3333333333333333703, 0.3333333333333333703, 0.3333333333333333703, 0.3333333333333333703, 0.3333333333333333703, 0.3333333333333333703, 0.3333333333333333703, 0.3333333333333333703, 0.3333333333333333703, 0.3333333333333333703, 0.3333333333333333703, 0.3333333333333333703, 0.3333333333333333703, 0.3333333333333333703, 0.3333333333333333703, 0.3333333333333333703, 0.3333333333333333703, 0.3333333333333333703, 0.3333333333333333703, 0.3333333333333333703, 0.3333333333333333703, 0.3333333333333333703, 0.3333333333333333703, 0.3333333333333333703, 0.3333333333333333703, 0.3333333333333333703, 0.3333333333333333703, 0.3333333333333333703, 0.3333333333333333703, 0.3333333333333333703, 0.3333333333333333703, 0.3333333333333333703, 0.3333333333333333703, 0.3333333333333333703, 0.3333333333333333703, 0.3333333333333333703, 0.3333333333333333703, 0.3333333333333333703, 0.3333333333333333703, 0.3333333333333333703, 0.3333333333333333703, 0.3333333333333333703, 0.3333333333333333703, 0.3333333333333333703, 0.3333333333333333703, 0.3333333333333333703, 0.3333333333333333703, 0.3333333333333333703, 0.3333333333333333703, 0.3333333333333333703, 0.3333333333333333703, 0.3333333333333333703, 0.3333333333333333703, 0.3333333333333333703, 0.3333333333333333703, 0.3333333333333333703, 0.3333333333333333703, 0.3333333333333333703, 0.3333333333333333703, 0.3333333333333333703, 0.3333333333333333703, 0.3333333333333333703, 0.3333333333333333703, 0.3333333333333333703, 0.3333333333333333703, 0.3333333333333333703, 0.3333333333333333703, 0.3333333333333333703, 0.3333333333333333703, 0.3333333333333333703, 0.3333333333333333703, 0.3333333333333333703, 0.3333333333333333703, 0.3333333333333333703, 0.3333333333333333703, 0.3333333333333333703, 0.3333333333333333703, 0.3333333333333333703, 0.3333333333333333703, 0.3333333333333333703, 0.3333333333333333703, 0.3333333333333333703, 0.3333333333333333703, 0.3333333333333333703, 0.3333333333333333703, 0.3333333333333333703, 0.3333333333333333703, 0.3333333333333333703, 0.3333333333333333703, 0.3333333333333333703, 0.3333333333333333703, 0.3333333333333333703, 0.3333333333333333703, 0.3333333333333333703, 0.3333333333333333703, 0.3333333333333333703, 0.3333333333333333703, 0.3333333333333333703, 0.3333333333333333703, 0.3333333333333333703, 0.3333333333333333703, 0.3333333333333333703, 0.3333333333333333703, 0.3333333333333333703, 0.3333333333333333703, 0.3333333333333333703, 0.3333333333333333703, 0.3333333333333333703, 0.3333333333333333703, 0.3333333333333333703, 0.3333333333333333703, 0.3333333333333333703, 0.3333333333333333703, 0.3333333333333333703, 0.3333333333333333703, 0.3333333333333333703, 0.3333333333333333703, 0.3333333333333333703, 0.3333333333333333703, 0.3333333333333333703, 0.3333333333333333703, 0.3333333333333333703, 0.3333333333333333703, 0.3333333333333333703, 0.3333333333333333703, 0.3333333333333333703, 0.3333333333333333703, 0.3333333333333333703, 0.3333333333333333703, 0.3333333333333333703, 0.3333333333333333703, 0.3333333333333333703, 0.3333333333333333703, 0.3333333333333333703, 0.3333333333333333703, 0.3333333333333333703, 0.3333333333333333703, 0.3333333333333333703, 0.3333333333333333703, 0.3333333333333333703, 0.3333333333333333703, 0.3333333333333333703, 0.3333333333333333703, 0.3333333333333333703, 0.3333333333333333703),
 ( 1.000000000000000000, 1.000000000000000000, 1.000000000000000000, 1.000000000000000000, 1.000000000000000000, 1.000000000000000000, 1.000000000000000000, 1.000000000000000000, 1.000000000000000000, 1.000000000000000000, 1.000000000000000000, 1.000000000000000000, 1.000000000000000000, 1.000000000000000000, 1.000000000000000000, 1.000000000000000000, 1.000000000000000000, 1.000000000000000000, 1.000000000000000000, 1.000000000000000000, 1.000000000000000000, 1.000000000000000000, 1.000000000000000000, 1.000000000000000000, 1.000000000000000000, 1.000000000000000000, 1.000000000000000000, 1.000000000000000000, 1.000000000000000000, 1.000000000000000000, 1.000000000000000000, 1.000000000000000000, 1.000000000000000000, 1.000000000000000000, 1.000000000000000000, 1.000000000000000000, 1.000000000000000000, 1.000000000000000000, 1.000000000000000000, 1.000000000000000000, 1.000000000000000000, 1.000000000000000000, 1.000000000000000000, 1.000000000000000000, 1.000000000000000000, 1.000000000000000000, 1.000000000000000000, 1.000000000000000000, 1.000000000000000000, 1.000000000000000000, 1.000000000000000000, 1.000000000000000000, 1.000000000000000000, 1.000000000000000000, 1.000000000000000000, 1.000000000000000000, 1.000000000000000000, 1.000000000000000000, 1.000000000000000000, 1.000000000000000000, 1.000000000000000000, 1.000000000000000000, 1.000000000000000000, 1.000000000000000000, 1.000000000000000000, 1.000000000000000000, 1.000000000000000000, 1.000000000000000000, 1.000000000000000000, 1.000000000000000000, 1.000000000000000000, 1.000000000000000000, 1.000000000000000000, 1.000000000000000000, 1.000000000000000000, 1.000000000000000000, 1.000000000000000000, 1.000000000000000000, 1.000000000000000000, 1.000000000000000000, 1.000000000000000000, 1.000000000000000000, 1.000000000000000000, 1.000000000000000000, 1.000000000000000000, 1.000000000000000000, 1.000000000000000000, 1.000000000000000000, 1.000000000000000000, 1.000000000000000000, 1.000000000000000000, 1.000000000000000000, 1.000000000000000000, 1.000000000000000000, 1.000000000000000000, 1.000000000000000000, 1.000000000000000000, 1.000000000000000000, 1.000000000000000000, 1.000000000000000000, 1.000000000000000000, 1.000000000000000000, 1.000000000000000000, 1.000000000000000000, 1.000000000000000000, 1.000000000000000000, 1.000000000000000000, 1.000000000000000000, 1.000000000000000000, 1.000000000000000000, 1.000000000000000000, 1.000000000000000000, 1.000000000000000000, 1.000000000000000000, 1.000000000000000000, 1.000000000000000000, 1.000000000000000000, 1.000000000000000000, 1.000000000000000000, 1.000000000000000000, 1.000000000000000000, 1.000000000000000000, 1.000000000000000000, 1.000000000000000000, 1.000000000000000000, 1.000000000000000000, 1.000000000000000000, 1.000000000000000000, 1.000000000000000000, 1.000000000000000000, 1.000000000000000000, 1.000000000000000000, 1.000000000000000000, 1.000000000000000000, 1.000000000000000000, 1.000000000000000000, 1.000000000000000000, 1.000000000000000000, 1.000000000000000000, 1.000000000000000000, 1.000000000000000000, 1.000000000000000000, 1.000000000000000000, 1.000000000000000000, 1.000000000000000000, 1.000000000000000000, 1.000000000000000000, 1.000000000000000000, 1.000000000000000000, 1.000000000000000000, 1.000000000000000000, 1.000000000000000000, 1.000000000000000000, 1.000000000000000000, 1.000000000000000000, 1.000000000000000000, 1.000000000000000000, 1.000000000000000000, 1.000000000000000000, 1.000000000000000000, 1.000000000000000000, 1.000000000000000000, 1.000000000000000000, 1.000000000000000000, 1.000000000000000000, 1.000000000000000000, 1.000000000000000000, 1.000000000000000000, 1.000000000000000000, 1.000000000000000000, 1.000000000000000000, 1.000000000000000000, 1.000000000000000000, 1.000000000000000000, 1.000000000000000000, 1.000000000000000000, 1.000000000000000000, 1.000000000000000000, 1.000000000000000000, 1.000000000000000000, 1.000000000000000000, 1.000000000000000000, 1.000000000000000000, 1.000000000000000000, 1.000000000000000000, 1.000000000000000000, 1.000000000000000000, 1.000000000000000000, 1.000000000000000000, 1.000000000000000000, 1.000000000000000000, 1.000000000000000000, 1.000000000000000000, 1.000000000000000000, 1.000000000000000000, 1.000000000000000000, 1.000000000000000000, 1.000000000000000000, 1.000000000000000000, 1.000000000000000000, 1.000000000000000000, 1.000000000000000000, 1.000000000000000000, 1.000000000000000000, 1.000000000000000000, 1.000000000000000000, 1.000000000000000000, 1.000000000000000000, 1.000000000000000000, 1.000000000000000000, 1.000000000000000000, 1.000000000000000000, 1.000000000000000000, 1.000000000000000000, 1.000000000000000000, 1.000000000000000000, 1.000000000000000000, 1.000000000000000000, 1.000000000000000000, 1.000000000000000000, 1.000000000000000000, 1.000000000000000000, 1.000000000000000000, 1.000000000000000000, 1.000000000000000000, 1.000000000000000000, 1.000000000000000000, 1.000000000000000000, 1.000000000000000000, 1.000000000000000000, 1.000000000000000000, 1.000000000000000000, 1.000000000000000000, 1.000000000000000000, 1.000000000000000000, 1.000000000000000000, 1.000000000000000000, 1.000000000000000000, 1.000000000000000000, 1.000000000000000000, 1.000000000000000000, 1.000000000000000000, 1.000000000000000000, 1.000000000000000000, 1.000000000000000000, 1.000000000000000000, 1.000000000000000000, 1.000000000000000000, 1.000000000000000000, 1.000000000000000000, 1.000000000000000000, 1.000000000000000000, 1.000000000000000000, 1.000000000000000000, 1.000000000000000000, 1.000000000000000000, 1.000000000000000000, 1.000000000000000000, 1.000000000000000000, 1.000000000000000000, 1.000000000000000000, 1.000000000000000000, 1.000000000000000000, 1.000000000000000000, 1.000000000000000000, 1.000000000000000000, 1.000000000000000000, 1.000000000000000000, 1.000000000000000000, 1.000000000000000000, 1.000000000000000000, 1.000000000000000000, 1.000000000000000000, 1.000000000000000000, 1.000000000000000000, 1.000000000000000000, 1.000000000000000000, 1.000000000000000000, 1.000000000000000000, 1.000000000000000000, 1.000000000000000000, 1.000000000000000000, 1.000000000000000000, 1.000000000000000000, 1.000000000000000000, 1.000000000000000000, 1.000000000000000000, 1.000000000000000000, 1.000000000000000000, 1.000000000000000000, 1.000000000000000000, 1.000000000000000000, 1.000000000000000000, 1.000000000000000000, 1.000000000000000000, 1.000000000000000000, 1.000000000000000000, 1.000000000000000000, 1.000000000000000000, 1.000000000000000000, 1.000000000000000000, 1.000000000000000000, 1.000000000000000000, 1.000000000000000000, 1.000000000000000000, 1.000000000000000000, 1.000000000000000000, 1.000000000000000000, 1.000000000000000000, 1.000000000000000000, 1.000000000000000000, 1.000000000000000000, 1.000000000000000000, 1.000000000000000000, 1.000000000000000000, 1.000000000000000000, 1.000000000000000000, 1.000000000000000000, 1.000000000000000000, 1.000000000000000000, 1.000000000000000000, 1.000000000000000000, 1.000000000000000000, 1.000000000000000000, 1.000000000000000000, 1.000000000000000000, 1.000000000000000000, 1.000000000000000000, 1.000000000000000000, 1.000000000000000000, 1.000000000000000000, 1.000000000000000000, 1.000000000000000000, 1.000000000000000000, 1.000000000000000000, 1.000000000000000000),
 ( 0.3333333333333333703, 0.3333333333333333703, 0.3333333333333333703, 0.3333333333333333703, 0.3333333333333333703, 0.3333333333333333703, 0.3333333333333333703, 0.3333333333333333703, 0.3333333333333333703, 0.3333333333333333703, 0.3333333333333333703, 0.3333333333333333703, 0.3333333333333333703, 0.3333333333333333703, 0.3333333333333333703, 0.3333333333333333703, 0.3333333333333333703, 0.3333333333333333703, 0.3333333333333333703, 0.3333333333333333703, 0.3333333333333333703, 0.3333333333333333703, 0.3333333333333333703, 0.3333333333333333703, 0.3333333333333333703, 0.3333333333333333703, 0.3333333333333333703, 0.3333333333333333703, 0.3333333333333333703, 0.3333333333333333703, 0.3333333333333333703, 0.3333333333333333703, 0.3333333333333333703, 0.3333333333333333703, 0.3333333333333333703, 0.3333333333333333703, 0.3333333333333333703, 0.3333333333333333703, 0.3333333333333333703, 0.3333333333333333703, 0.3333333333333333703, 0.3333333333333333703, 0.3333333333333333703, 0.3333333333333333703, 0.3333333333333333703, 0.3333333333333333703, 0.3333333333333333703, 0.3333333333333333703, 0.3333333333333333703, 0.3333333333333333703, 0.3333333333333333703, 0.3333333333333333703, 0.3333333333333333703, 0.3333333333333333703, 0.3333333333333333703, 0.3333333333333333703, 0.3333333333333333703, 0.3333333333333333703, 0.3333333333333333703, 0.3333333333333333703, 0.3333333333333333703, 0.3333333333333333703, 0.3333333333333333703, 0.3333333333333333703, 0.3333333333333333703, 0.3333333333333333703, 0.3333333333333333703, 0.3333333333333333703, 0.3333333333333333703, 0.3333333333333333703, 0.3333333333333333703, 0.3333333333333333703, 0.3333333333333333703, 0.3333333333333333703, 0.3333333333333333703, 0.3333333333333333703, 0.3333333333333333703, 0.3333333333333333703, 0.3333333333333333703, 0.3333333333333333703, 0.3333333333333333703, 0.3333333333333333703, 0.3333333333333333703, 0.3333333333333333703, 0.3333333333333333703, 0.3333333333333333703, 0.3333333333333333703, 0.3333333333333333703, 0.3333333333333333703, 0.3333333333333333703, 0.3333333333333333703, 0.3333333333333333703, 0.3333333333333333703, 0.3333333333333333703, 0.3333333333333333703, 0.3333333333333333703, 0.3333333333333333703, 0.3333333333333333703, 0.3333333333333333703, 0.3333333333333333703, 0.3333333333333333703, 0.3333333333333333703, 0.3333333333333333703, 0.3333333333333333703, 0.3333333333333333703, 0.3333333333333333703, 0.3333333333333333703, 0.3333333333333333703, 0.3333333333333333703, 0.3333333333333333703, 0.3333333333333333703, 0.3333333333333333703, 0.3333333333333333703, 0.3333333333333333703, 0.3333333333333333703, 0.3333333333333333703, 0.3333333333333333703, 0.3333333333333333703, 0.3333333333333333703, 0.3333333333333333703, 0.3333333333333333703, 0.3333333333333333703, 0.3333333333333333703, 0.3333333333333333703, 0.3333333333333333703, 0.3333333333333333703, 0.3333333333333333703, 0.3333333333333333703, 0.3333333333333333703, 0.3333333333333333703, 0.3333333333333333703, 0.3333333333333333703, 0.3333333333333333703, 0.3333333333333333703, 0.3333333333333333703, 0.3333333333333333703, 0.3333333333333333703, 0.3333333333333333703, 0.3333333333333333703, 0.3333333333333333703, 0.3333333333333333703, 0.3333333333333333703, 0.3333333333333333703, 0.3333333333333333703, 0.3333333333333333703, 0.3333333333333333703, 0.3333333333333333703, 0.3333333333333333703, 0.3333333333333333703, 0.3333333333333333703, 0.3333333333333333703, 0.3333333333333333703, 0.3333333333333333703, 0.3333333333333333703, 0.3333333333333333703, 0.3333333333333333703, 0.3333333333333333703, 0.3333333333333333703, 0.3333333333333333703, 0.3333333333333333703, 0.3333333333333333703, 0.3333333333333333703, 0.3333333333333333703, 0.3333333333333333703, 0.3333333333333333703, 0.3333333333333333703, 0.3333333333333333703, 0.3333333333333333703, 0.3333333333333333703, 0.3333333333333333703, 0.3333333333333333703, 0.3333333333333333703, 0.3333333333333333703, 0.3333333333333333703, 0.3333333333333333703, 0.3333333333333333703, 0.3333333333333333703, 0.3333333333333333703, 0.3333333333333333703, 0.3333333333333333703, 0.3333333333333333703, 0.3333333333333333703, 0.3333333333333333703, 0.3333333333333333703, 0.3333333333333333703, 0.3333333333333333703, 0.3333333333333333703, 0.3333333333333333703, 0.3333333333333333703, 0.3333333333333333703, 0.3333333333333333703, 0.3333333333333333703, 0.3333333333333333703, 0.3333333333333333703, 0.3333333333333333703, 0.3333333333333333703, 0.3333333333333333703, 0.3333333333333333703, 0.3333333333333333703, 0.3333333333333333703, 0.3333333333333333703, 0.3333333333333333703, 0.3333333333333333703, 0.3333333333333333703, 0.3333333333333333703, 0.3333333333333333703, 0.3333333333333333703, 0.3333333333333333703, 0.3333333333333333703, 0.3333333333333333703, 0.3333333333333333703, 0.3333333333333333703, 0.3333333333333333703, 0.3333333333333333703, 0.3333333333333333703, 0.3333333333333333703, 0.3333333333333333703, 0.3333333333333333703, 0.3333333333333333703, 0.3333333333333333703, 0.3333333333333333703, 0.3333333333333333703, 0.3333333333333333703, 0.3333333333333333703, 0.3333333333333333703, 0.3333333333333333703, 0.3333333333333333703, 0.3333333333333333703, 0.3333333333333333703, 0.3333333333333333703, 0.3333333333333333703, 0.3333333333333333703, 0.3333333333333333703, 0.3333333333333333703, 0.3333333333333333703, 0.3333333333333333703, 0.3333333333333333703, 0.3333333333333333703, 0.3333333333333333703, 0.3333333333333333703, 0.3333333333333333703, 0.3333333333333333703, 0.3333333333333333703, 0.3333333333333333703, 0.3333333333333333703, 0.3333333333333333703, 0.3333333333333333703, 0.3333333333333333703, 0.3333333333333333703, 0.3333333333333333703, 0.3333333333333333703, 0.3333333333333333703, 0.3333333333333333703, 0.3333333333333333703, 0.3333333333333333703, 0.3333333333333333703, 0.3333333333333333703, 0.3333333333333333703, 0.3333333333333333703, 0.3333333333333333703, 0.3333333333333333703, 0.3333333333333333703, 0.3333333333333333703, 0.3333333333333333703, 0.3333333333333333703, 0.3333333333333333703, 0.3333333333333333703, 0.3333333333333333703, 0.3333333333333333703, 0.3333333333333333703, 0.3333333333333333703, 0.3333333333333333703, 0.3333333333333333703, 0.3333333333333333703, 0.3333333333333333703, 0.3333333333333333703, 0.3333333333333333703, 0.3333333333333333703, 0.3333333333333333703, 0.3333333333333333703, 0.3333333333333333703, 0.3333333333333333703, 0.3333333333333333703, 0.3333333333333333703, 0.3333333333333333703, 0.3333333333333333703, 0.3333333333333333703, 0.3333333333333333703, 0.3333333333333333703, 0.3333333333333333703, 0.3333333333333333703, 0.3333333333333333703, 0.3333333333333333703, 0.3333333333333333703, 0.3333333333333333703, 0.3333333333333333703, 0.3333333333333333703, 0.3333333333333333703, 0.3333333333333333703, 0.3333333333333333703, 0.3333333333333333703, 0.3333333333333333703, 0.3333333333333333703, 0.3333333333333333703, 0.3333333333333333703, 0.3333333333333333703, 0.3333333333333333703, 0.3333333333333333703, 0.3333333333333333703, 0.3333333333333333703, 0.3333333333333333703, 0.3333333333333333703, 0.3333333333333333703, 0.3333333333333333703, 0.3333333333333333703, 0.3333333333333333703, 0.3333333333333333703, 0.3333333333333333703, 0.3333333333333333703, 0.3333333333333333703, 0.3333333333333333703, 0.3333333333333333703, 0.3333333333333333703, 0.3333333333333333703, 0.3333333333333333703, 0.3333333333333333703, 0.3333333333333333703, 0.3333333333333333703, 0.3333333333333333703, 0.3333333333333333703, 0.3333333333333333703, 0.3333333333333333703, 0.3333333333333333703, 0.3333333333333333703, 0.3333333333333333703, 0.3333333333333333703),
 ( 0.3333333333333333703, 0.3333333333333333703, 0.3333333333333333703, 0.3333333333333333703, 0.3333333333333333703, 0.3333333333333333703, 0.3333333333333333703, 0.3333333333333333703, 0.3333333333333333703, 0.3333333333333333703, 0.3333333333333333703, 0.3333333333333333703, 0.3333333333333333703, 0.3333333333333333703, 0.3333333333333333703, 0.3333333333333333703, 0.3333333333333333703, 0.3333333333333333703, 0.3333333333333333703, 0.3333333333333333703, 0.3333333333333333703, 0.3333333333333333703, 0.3333333333333333703, 0.3333333333333333703, 0.3333333333333333703, 0.3333333333333333703, 0.3333333333333333703, 0.3333333333333333703, 0.3333333333333333703, 0.3333333333333333703, 0.3333333333333333703, 0.3333333333333333703, 0.3333333333333333703, 0.3333333333333333703, 0.3333333333333333703, 0.3333333333333333703, 0.3333333333333333703, 0.3333333333333333703, 0.3333333333333333703, 0.3333333333333333703, 0.3333333333333333703, 0.3333333333333333703, 0.3333333333333333703, 0.3333333333333333703, 0.3333333333333333703, 0.3333333333333333703, 0.3333333333333333703, 0.3333333333333333703, 0.3333333333333333703, 0.3333333333333333703, 0.3333333333333333703, 0.3333333333333333703, 0.3333333333333333703, 0.3333333333333333703, 0.3333333333333333703, 0.3333333333333333703, 0.3333333333333333703, 0.3333333333333333703, 0.3333333333333333703, 0.3333333333333333703, 0.3333333333333333703, 0.3333333333333333703, 0.3333333333333333703, 0.3333333333333333703, 0.3333333333333333703, 0.3333333333333333703, 0.3333333333333333703, 0.3333333333333333703, 0.3333333333333333703, 0.3333333333333333703, 0.3333333333333333703, 0.3333333333333333703, 0.3333333333333333703, 0.3333333333333333703, 0.3333333333333333703, 0.3333333333333333703, 0.3333333333333333703, 0.3333333333333333703, 0.3333333333333333703, 0.3333333333333333703, 0.3333333333333333703, 0.3333333333333333703, 0.3333333333333333703, 0.3333333333333333703, 0.3333333333333333703, 0.3333333333333333703, 0.3333333333333333703, 0.3333333333333333703, 0.3333333333333333703, 0.3333333333333333703, 0.3333333333333333703, 0.3333333333333333703, 0.3333333333333333703, 0.3333333333333333703, 0.3333333333333333703, 0.3333333333333333703, 0.3333333333333333703, 0.3333333333333333703, 0.3333333333333333703, 0.3333333333333333703, 0.3333333333333333703, 0.3333333333333333703, 0.3333333333333333703, 0.3333333333333333703, 0.3333333333333333703, 0.3333333333333333703, 0.3333333333333333703, 0.3333333333333333703, 0.3333333333333333703, 0.3333333333333333703, 0.3333333333333333703, 0.3333333333333333703, 0.3333333333333333703, 0.3333333333333333703, 0.3333333333333333703, 0.3333333333333333703, 0.3333333333333333703, 0.3333333333333333703, 0.3333333333333333703, 0.3333333333333333703, 0.3333333333333333703, 0.3333333333333333703, 0.3333333333333333703, 0.3333333333333333703, 0.3333333333333333703, 0.3333333333333333703, 0.3333333333333333703, 0.3333333333333333703, 0.3333333333333333703, 0.3333333333333333703, 0.3333333333333333703, 0.3333333333333333703, 0.3333333333333333703, 0.3333333333333333703, 0.3333333333333333703, 0.3333333333333333703, 0.3333333333333333703, 0.3333333333333333703, 0.3333333333333333703, 0.3333333333333333703, 0.3333333333333333703, 0.3333333333333333703, 0.3333333333333333703, 0.3333333333333333703, 0.3333333333333333703, 0.3333333333333333703, 0.3333333333333333703, 0.3333333333333333703, 0.3333333333333333703, 0.3333333333333333703, 0.3333333333333333703, 0.3333333333333333703, 0.3333333333333333703, 0.3333333333333333703, 0.3333333333333333703, 0.3333333333333333703, 0.3333333333333333703, 0.3333333333333333703, 0.3333333333333333703, 0.3333333333333333703, 0.3333333333333333703, 0.3333333333333333703, 0.3333333333333333703, 0.3333333333333333703, 0.3333333333333333703, 0.3333333333333333703, 0.3333333333333333703, 0.3333333333333333703, 0.3333333333333333703, 0.3333333333333333703, 0.3333333333333333703, 0.3333333333333333703, 0.3333333333333333703, 0.3333333333333333703, 0.3333333333333333703, 0.3333333333333333703, 0.3333333333333333703, 0.3333333333333333703, 0.3333333333333333703, 0.3333333333333333703, 0.3333333333333333703, 0.3333333333333333703, 0.3333333333333333703, 0.3333333333333333703, 0.3333333333333333703, 0.3333333333333333703, 0.3333333333333333703, 0.3333333333333333703, 0.3333333333333333703, 0.3333333333333333703, 0.3333333333333333703, 0.3333333333333333703, 0.3333333333333333703, 0.3333333333333333703, 0.3333333333333333703, 0.3333333333333333703, 0.3333333333333333703, 0.3333333333333333703, 0.3333333333333333703, 0.3333333333333333703, 0.3333333333333333703, 0.3333333333333333703, 0.3333333333333333703, 0.3333333333333333703, 0.3333333333333333703, 0.3333333333333333703, 0.3333333333333333703, 0.3333333333333333703, 0.3333333333333333703, 0.3333333333333333703, 0.3333333333333333703, 0.3333333333333333703, 0.3333333333333333703, 0.3333333333333333703, 0.3333333333333333703, 0.3333333333333333703, 0.3333333333333333703, 0.3333333333333333703, 0.3333333333333333703, 0.3333333333333333703, 0.3333333333333333703, 0.3333333333333333703, 0.3333333333333333703, 0.3333333333333333703, 0.3333333333333333703, 0.3333333333333333703, 0.3333333333333333703, 0.3333333333333333703, 0.3333333333333333703, 0.3333333333333333703, 0.3333333333333333703, 0.3333333333333333703, 0.3333333333333333703, 0.3333333333333333703, 0.3333333333333333703, 0.3333333333333333703, 0.3333333333333333703, 0.3333333333333333703, 0.3333333333333333703, 0.3333333333333333703, 0.3333333333333333703, 0.3333333333333333703, 0.3333333333333333703, 0.3333333333333333703, 0.3333333333333333703, 0.3333333333333333703, 0.3333333333333333703, 0.3333333333333333703, 0.3333333333333333703, 0.3333333333333333703, 0.3333333333333333703, 0.3333333333333333703, 0.3333333333333333703, 0.3333333333333333703, 0.3333333333333333703, 0.3333333333333333703, 0.3333333333333333703, 0.3333333333333333703, 0.3333333333333333703, 0.3333333333333333703, 0.3333333333333333703, 0.3333333333333333703, 0.3333333333333333703, 0.3333333333333333703, 0.3333333333333333703, 0.3333333333333333703, 0.3333333333333333703, 0.3333333333333333703, 0.3333333333333333703, 0.3333333333333333703, 0.3333333333333333703, 0.3333333333333333703, 0.3333333333333333703, 0.3333333333333333703, 0.3333333333333333703, 0.3333333333333333703, 0.3333333333333333703, 0.3333333333333333703, 0.3333333333333333703, 0.3333333333333333703, 0.3333333333333333703, 0.3333333333333333703, 0.3333333333333333703, 0.3333333333333333703, 0.3333333333333333703, 0.3333333333333333703, 0.3333333333333333703, 0.3333333333333333703, 0.3333333333333333703, 0.3333333333333333703, 0.3333333333333333703, 0.3333333333333333703, 0.3333333333333333703, 0.3333333333333333703, 0.3333333333333333703, 0.3333333333333333703, 0.3333333333333333703, 0.3333333333333333703, 0.3333333333333333703, 0.3333333333333333703, 0.3333333333333333703, 0.3333333333333333703, 0.3333333333333333703, 0.3333333333333333703, 0.3333333333333333703, 0.3333333333333333703, 0.3333333333333333703, 0.3333333333333333703, 0.3333333333333333703, 0.3333333333333333703, 0.3333333333333333703, 0.3333333333333333703, 0.3333333333333333703, 0.3333333333333333703, 0.3333333333333333703, 0.3333333333333333703, 0.3333333333333333703, 0.3333333333333333703, 0.3333333333333333703, 0.3333333333333333703, 0.3333333333333333703, 0.3333333333333333703, 0.3333333333333333703, 0.3333333333333333703, 0.3333333333333333703, 0.3333333333333333703, 0.3333333333333333703, 0.3333333333333333703, 0.3333333333333333703, 0.3333333333333333703, 0.3333333333333333703, 0.3333333333333333703, 0.3333333333333333703, 0.3333333333333333703, 0.3333333333333333703, 0.3333333333333333703),
 ( 1.000000000000000000, 1.000000000000000000, 1.000000000000000000, 1.000000000000000000, 1.000000000000000000, 1.000000000000000000, 1.000000000000000000, 1.000000000000000000, 1.000000000000000000, 1.000000000000000000, 1.000000000000000000, 1.000000000000000000, 1.000000000000000000, 1.000000000000000000, 1.000000000000000000, 1.000000000000000000, 1.000000000000000000, 1.000000000000000000, 1.000000000000000000, 1.000000000000000000, 1.000000000000000000, 1.000000000000000000, 1.000000000000000000, 1.000000000000000000, 1.000000000000000000, 1.000000000000000000, 1.000000000000000000, 1.000000000000000000, 1.000000000000000000, 1.000000000000000000, 1.000000000000000000, 1.000000000000000000, 1.000000000000000000, 1.000000000000000000, 1.000000000000000000, 1.000000000000000000, 1.000000000000000000, 1.000000000000000000, 1.000000000000000000, 1.000000000000000000, 1.000000000000000000, 1.000000000000000000, 1.000000000000000000, 1.000000000000000000, 1.000000000000000000, 1.000000000000000000, 1.000000000000000000, 1.000000000000000000, 1.000000000000000000, 1.000000000000000000, 1.000000000000000000, 1.000000000000000000, 1.000000000000000000, 1.000000000000000000, 1.000000000000000000, 1.000000000000000000, 1.000000000000000000, 1.000000000000000000, 1.000000000000000000, 1.000000000000000000, 1.000000000000000000, 1.000000000000000000, 1.000000000000000000, 1.000000000000000000, 1.000000000000000000, 1.000000000000000000, 1.000000000000000000, 1.000000000000000000, 1.000000000000000000, 1.000000000000000000, 1.000000000000000000, 1.000000000000000000, 1.000000000000000000, 1.000000000000000000, 1.000000000000000000, 1.000000000000000000, 1.000000000000000000, 1.000000000000000000, 1.000000000000000000, 1.000000000000000000, 1.000000000000000000, 1.000000000000000000, 1.000000000000000000, 1.000000000000000000, 1.000000000000000000, 1.000000000000000000, 1.000000000000000000, 1.000000000000000000, 1.000000000000000000, 1.000000000000000000, 1.000000000000000000, 1.000000000000000000, 1.000000000000000000, 1.000000000000000000, 1.000000000000000000, 1.000000000000000000, 1.000000000000000000, 1.000000000000000000, 1.000000000000000000, 1.000000000000000000, 1.000000000000000000, 1.000000000000000000, 1.000000000000000000, 1.000000000000000000, 1.000000000000000000, 1.000000000000000000, 1.000000000000000000, 1.000000000000000000, 1.000000000000000000, 1.000000000000000000, 1.000000000000000000, 1.000000000000000000, 1.000000000000000000, 1.000000000000000000, 1.000000000000000000, 1.000000000000000000, 1.000000000000000000, 1.000000000000000000, 1.000000000000000000, 1.000000000000000000, 1.000000000000000000, 1.000000000000000000, 1.000000000000000000, 1.000000000000000000, 1.000000000000000000, 1.000000000000000000, 1.000000000000000000, 1.000000000000000000, 1.000000000000000000, 1.000000000000000000, 1.000000000000000000, 1.000000000000000000, 1.000000000000000000, 1.000000000000000000, 1.000000000000000000, 1.000000000000000000, 1.000000000000000000, 1.000000000000000000, 1.000000000000000000, 1.000000000000000000, 1.000000000000000000, 1.000000000000000000, 1.000000000000000000, 1.000000000000000000, 1.000000000000000000, 1.000000000000000000, 1.000000000000000000, 1.000000000000000000, 1.000000000000000000, 1.000000000000000000, 1.000000000000000000, 1.000000000000000000, 1.000000000000000000, 1.000000000000000000, 1.000000000000000000, 1.000000000000000000, 1.000000000000000000, 1.000000000000000000, 1.000000000000000000, 1.000000000000000000, 1.000000000000000000, 1.000000000000000000, 1.000000000000000000, 1.000000000000000000, 1.000000000000000000, 1.000000000000000000, 1.000000000000000000, 1.000000000000000000, 1.000000000000000000, 1.000000000000000000, 1.000000000000000000, 1.000000000000000000, 1.000000000000000000, 1.000000000000000000, 1.000000000000000000, 1.000000000000000000, 1.000000000000000000, 1.000000000000000000, 1.000000000000000000, 1.000000000000000000, 1.000000000000000000, 1.000000000000000000, 1.000000000000000000, 1.000000000000000000, 1.000000000000000000, 1.000000000000000000, 1.000000000000000000, 1.000000000000000000, 1.000000000000000000, 1.000000000000000000, 1.000000000000000000, 1.000000000000000000, 1.000000000000000000, 1.000000000000000000, 1.000000000000000000, 1.000000000000000000, 1.000000000000000000, 1.000000000000000000, 1.000000000000000000, 1.000000000000000000, 1.000000000000000000, 1.000000000000000000, 1.000000000000000000, 1.000000000000000000, 1.000000000000000000, 1.000000000000000000, 1.000000000000000000, 1.000000000000000000, 1.000000000000000000, 1.000000000000000000, 1.000000000000000000, 1.000000000000000000, 1.000000000000000000, 1.000000000000000000, 1.000000000000000000, 1.000000000000000000, 1.000000000000000000, 1.000000000000000000, 1.000000000000000000, 1.000000000000000000, 1.000000000000000000, 1.000000000000000000, 1.000000000000000000, 1.000000000000000000, 1.000000000000000000, 1.000000000000000000, 1.000000000000000000, 1.000000000000000000, 1.000000000000000000, 1.000000000000000000, 1.000000000000000000, 1.000000000000000000, 1.000000000000000000, 1.000000000000000000, 1.000000000000000000, 1.000000000000000000, 1.000000000000000000, 1.000000000000000000, 1.000000000000000000, 1.000000000000000000, 1.000000000000000000, 1.000000000000000000, 1.000000000000000000, 1.000000000000000000, 1.000000000000000000, 1.000000000000000000, 1.000000000000000000, 1.000000000000000000, 1.000000000000000000, 1.000000000000000000, 1.000000000000000000, 1.000000000000000000, 1.000000000000000000, 1.000000000000000000, 1.000000000000000000, 1.000000000000000000, 1.000000000000000000, 1.000000000000000000, 1.000000000000000000, 1.000000000000000000, 1.000000000000000000, 1.000000000000000000, 1.000000000000000000, 1.000000000000000000, 1.000000000000000000, 1.000000000000000000, 1.000000000000000000, 1.000000000000000000, 1.000000000000000000, 1.000000000000000000, 1.000000000000000000, 1.000000000000000000, 1.000000000000000000, 1.000000000000000000, 1.000000000000000000, 1.000000000000000000, 1.000000000000000000, 1.000000000000000000, 1.000000000000000000, 1.000000000000000000, 1.000000000000000000, 1.000000000000000000, 1.000000000000000000, 1.000000000000000000, 1.000000000000000000, 1.000000000000000000, 1.000000000000000000, 1.000000000000000000, 1.000000000000000000, 1.000000000000000000, 1.000000000000000000, 1.000000000000000000, 1.000000000000000000, 1.000000000000000000, 1.000000000000000000, 1.000000000000000000, 1.000000000000000000, 1.000000000000000000, 1.000000000000000000, 1.000000000000000000, 1.000000000000000000, 1.000000000000000000, 1.000000000000000000, 1.000000000000000000, 1.000000000000000000, 1.000000000000000000, 1.000000000000000000, 1.000000000000000000, 1.000000000000000000, 1.000000000000000000, 1.000000000000000000, 1.000000000000000000, 1.000000000000000000, 1.000000000000000000, 1.000000000000000000, 1.000000000000000000, 1.000000000000000000, 1.000000000000000000, 1.000000000000000000, 1.000000000000000000, 1.000000000000000000, 1.000000000000000000, 1.000000000000000000, 1.000000000000000000, 1.000000000000000000, 1.000000000000000000, 1.000000000000000000, 1.000000000000000000, 1.000000000000000000, 1.000000000000000000, 1.000000000000000000, 1.000000000000000000, 1.000000000000000000, 1.000000000000000000, 1.000000000000000000, 1.000000000000000000) ) ) 
 REPRESENTATION_ITEM ( '' )  SURFACE ( )  );
#12332=CARTESIAN_POINT ( 'NONE',  ( 10.03842945413050458, 28.43460431997513638, -225.8374938385031214 ) ) ;
#12333=CARTESIAN_POINT ( 'NONE',  ( 15.39025625686376841, 1.044190007782545226, -218.9203249718910911 ) ) ;
#12334=CARTESIAN_POINT ( 'NONE',  ( 11.75404126451729070, 5.688294280104953415, -229.3533586468489602 ) ) ;
#12335=CARTESIAN_POINT ( 'NONE',  ( 16.43596176044053081, -17.06621466254232544, -232.8418678805942648 ) ) ;
#12338=CARTESIAN_POINT ( 'NONE',  ( -6.855867220396999251, 12.17758473459128332, -220.6375607554995213 ) ) ;
#12339=CARTESIAN_POINT ( 'NONE',  ( 23.20431681157275605, -3.694239143335118492, -219.1264243754107781 ) ) ;
#12340=CARTESIAN_POINT ( 'NONE',  ( 14.96415947227435339, -1.927366939720012606, -222.7010313878448358 ) ) ;
#12341=CARTESIAN_POINT ( 'NONE',  ( 20.89184612657454920, 5.404957034965973683, -232.0952743654565609 ) ) ;
#12342=CARTESIAN_POINT ( 'NONE',  ( -25.61997837663875188, 10.01664178086244483, -231.6711741719404074 ) ) ;
#12343=CARTESIAN_POINT ( 'NONE',  ( 1.904360901363437275, -12.77109371939166138, -224.5066922355585177 ) ) ;
#12345=CARTESIAN_POINT ( 'NONE',  ( -23.98802705797876200, 19.46654170242919690, -223.5293093576406989 ) ) ;
#12347=CARTESIAN_POINT ( 'NONE',  ( -22.57859951143173660, 16.82392524473188899, -219.5628058978911383 ) ) ;
#12349=CARTESIAN_POINT ( 'NONE',  ( -15.23434562258889891, -0.4010941804143903222, -220.4743703065900036 ) ) ;
#12350=CARTESIAN_POINT ( 'NONE',  ( -19.18273340400098448, -14.85130345181434741, -232.7114379411565039 ) ) ;
#12354=CARTESIAN_POINT ( 'NONE',  ( -13.55591840520136770, 8.363404288414606924, -231.2690188357804857 ) ) ;
#12355=CARTESIAN_POINT ( 'NONE',  ( 0.6837842112036801590, -24.48318360891119028, -216.1006322475167281 ) ) ;
#12358=CARTESIAN_POINT ( 'NONE',  ( 24.52860916307685457, 12.75391509163817361, -221.3604763108436941 ) ) ;
#12359=CARTESIAN_POINT ( 'NONE',  ( -4.591517861330576267, 12.55780501983563191, -223.5932882008353033 ) ) ;
#12361=CARTESIAN_POINT ( 'NONE',  ( 18.51425713624010427, 11.82474821235740592, -231.3645840199355632 ) ) ;
#12362=CARTESIAN_POINT ( 'NONE',  ( 3.520698644836853131, -14.14291361662535884, -221.2714412251625618 ) ) ;
#12364=CARTESIAN_POINT ( 'NONE',  ( -4.742143146070755932, 15.01230778631049567, -221.4832709320255049 ) ) ;
#12366=CARTESIAN_POINT ( 'NONE',  ( -15.82036597035495795, 4.920771916499852239, -223.0095317795067160 ) ) ;
#12367=CARTESIAN_POINT ( 'NONE',  ( -27.05172747931452903, 14.36075930490012276, -228.5082213655825853 ) ) ;
#12368=CARTESIAN_POINT ( 'NONE',  ( -12.19937816677273013, -10.70901586236097636, -226.3808855409166370 ) ) ;
#12372=CARTESIAN_POINT ( 'NONE',  ( 21.14328650935969023, 6.072767611243683916, -217.6422864096696514 ) ) ;
#12373=CARTESIAN_POINT ( 'NONE',  ( 1.672997396509183110, -28.78979777605457713, -223.2908548649682814 ) ) ;
#12374=CARTESIAN_POINT ( 'NONE',  ( 17.43816562714825125, 15.15720016074785903, -232.3748236813696906 ) ) ;
#12375=CARTESIAN_POINT ( 'NONE',  ( -11.26857159993117996, 28.96895336474501192, -225.6039696848669678 ) ) ;
#12376=CARTESIAN_POINT ( 'NONE',  ( 14.96462366732929716, 7.179279272144128754, -233.2042342402542374 ) ) ;
#12377=CARTESIAN_POINT ( 'NONE',  ( 10.66614775643814994, 26.29080367171353672, -230.0818785118670178 ) ) ;
#12379=CARTESIAN_POINT ( 'NONE',  ( -15.17658589853145479, -26.64966442869902252, -226.8090782225333442 ) ) ;
#12380=CARTESIAN_POINT ( 'NONE',  ( 10.24538335401965661, -11.82980241027587276, -219.3753974371782363 ) ) ;
#12384=CARTESIAN_POINT ( 'NONE',  ( -23.16143087541734502, 21.36835206473086046, -221.8715256527013651 ) ) ;
#12385=CARTESIAN_POINT ( 'NONE',  ( -25.18517655442826353, -3.313270981248286340, -229.9274946033256697 ) ) ;
#12386=CARTESIAN_POINT ( 'NONE',  ( 22.16327814861754675, 7.634676377199016706, -234.0520676664821735 ) ) ;
#12387=CARTESIAN_POINT ( 'NONE',  ( 2.893760225568064115, 14.39521026618305477, -227.6654023557511550 ) ) ;
#12388=CARTESIAN_POINT ( 'NONE',  ( 5.079647427451626562, 16.77877517420371234, -220.7769382327915366 ) ) ;
#12390=CARTESIAN_POINT ( 'NONE',  ( 8.477993572791891808, -8.340333012420144243, -224.9486226631276793 ) ) ;
#12392=CARTESIAN_POINT ( 'NONE',  ( 21.39553407250273054, 8.453402029343234148, -217.9531594780983141 ) ) ;
#12393=CARTESIAN_POINT ( 'NONE',  ( -10.33514150881494942, 13.62639309082336503, -216.9544063991933172 ) ) ;
#12394=CARTESIAN_POINT ( 'NONE',  ( -15.54392142943450317, 6.670312097614393920, -219.6934017696036676 ) ) ;
#12395=CARTESIAN_POINT ( 'NONE',  ( -17.66047203424674450, -3.377913611064220056, -232.7782090104293786 ) ) ;
#12396=CARTESIAN_POINT ( 'NONE',  ( -20.18153419852512442, 14.25141268122526483, -233.5059133483111964 ) ) ;
#12400=CARTESIAN_POINT ( 'NONE',  ( -11.79656379827575918, 10.43402410864828589, -226.0519616335988076 ) ) ;
#12401=CARTESIAN_POINT ( 'NONE',  ( 9.616550234602936342, 9.263684773868845923, -230.4827401731016607 ) ) ;
#12402=CARTESIAN_POINT ( 'NONE',  ( 27.50364976068844669, 3.973406265104437729, -228.8805639113908228 ) ) ;
#12404=CARTESIAN_POINT ( 'NONE',  ( -26.63259355655987548, -7.256793811979244779, -216.2488627322786101 ) ) ;
#12405=CARTESIAN_POINT ( 'NONE',  ( -21.14773328851117995, -13.15959238732831693, -217.2646803791660943 ) ) ;
#12406=CARTESIAN_POINT ( 'NONE',  ( -10.49339404011726984, 12.66576824096800991, -217.2681947942554643 ) ) ;
#12407=CARTESIAN_POINT ( 'NONE',  ( -1.308474130992312023, -24.58654860180777391, -216.2430112183533026 ) ) ;
#12408=CARTESIAN_POINT ( 'NONE',  ( 13.43170911749896490, 19.07691563292472026, -232.7497845103644636 ) ) ;
#12409=CARTESIAN_POINT ( 'NONE',  ( 4.772350409791505932, -16.13531085440822466, -233.6884202312745344 ) ) ;
#12411=CARTESIAN_POINT ( 'NONE',  ( -14.94640692938030746, 5.382918922058764544, -220.5478552936960455 ) ) ;
#12413=CARTESIAN_POINT ( 'NONE',  ( -2.543684969149407227, 16.28137730373167713, -227.6987697727321915 ) ) ;
#12414=CARTESIAN_POINT ( 'NONE',  ( -26.02492405343843984, 6.940268742526972900, -218.8798307745116460 ) ) ;
#12415=CARTESIAN_POINT ( 'NONE',  ( 27.75679124201660741, 4.911524026080384075, -221.4430403652340829 ) ) ;
#12416=CARTESIAN_POINT ( 'NONE',  ( 19.13999328532042910, 9.776920959053244431, -216.1190985676915375 ) ) ;
#12417=CARTESIAN_POINT ( 'NONE',  ( -10.64756522805915395, -11.91724881161430361, -221.7317784521105750 ) ) ;
#12420=CARTESIAN_POINT ( 'NONE',  ( 18.15173157547545557, 23.32481284044927961, -217.8532150843729482 ) ) ;
#12422=CARTESIAN_POINT ( 'NONE',  ( -10.19343904566850867, -16.03376756945627335, -215.1857286610140250 ) ) ;
#12423=CARTESIAN_POINT ( 'NONE',  ( -7.250603130619442283, 20.89725557392719324, -217.7893896917081520 ) ) ;
#12424=CARTESIAN_POINT ( 'NONE',  ( 9.774133712851615030, 11.09751083462123766, -229.6876724410067823 ) ) ;
#12425=CARTESIAN_POINT ( 'NONE',  ( -20.21481434941064848, 7.972326285609216967, -230.8475376972877484 ) ) ;
#12426=CARTESIAN_POINT ( 'NONE',  ( -13.31245686955614005, 26.96290519511623174, -230.1796856776773836 ) ) ;
#12427=CARTESIAN_POINT ( 'NONE',  ( 15.21408433160105034, 3.021350230896802103, -222.3056493717910769 ) ) ;
#12430=CARTESIAN_POINT ( 'NONE',  ( 9.379155480182538085, -13.23755613463586300, -225.9392943819708250 ) ) ;
#12433=CARTESIAN_POINT ( 'NONE',  ( 7.045253012492558753, -17.38872841331140862, -218.3726031779064556 ) ) ;
#12434=CARTESIAN_POINT ( 'NONE',  ( -1.158668551263366986, 23.31492692626720853, -219.2372600964201865 ) ) ;
#12436=CARTESIAN_POINT ( 'NONE',  ( 8.496844655769807630, 14.66037471857024599, -219.1631158796573118 ) ) ;
#12437=CARTESIAN_POINT ( 'NONE',  ( 24.59129902578158067, -8.191391589517788674, -218.4338547727923299 ) ) ;
#12438=CARTESIAN_POINT ( 'NONE',  ( -20.83683780809167629, -19.66850649927503625, -219.7460615899071570 ) ) ;
#12439=CARTESIAN_POINT ( 'NONE',  ( -5.178973235464019886, -24.35492185057628944, -233.6431870320687381 ) ) ;
#12441=CARTESIAN_POINT ( 'NONE',  ( -2.618694198633108261, 15.69630225547860825, -226.1451761977223498 ) ) ;
#12443=CARTESIAN_POINT ( 'NONE',  ( 24.38255093784924199, 7.851200578213498815, -231.2687759850219607 ) ) ;
#12444=CARTESIAN_POINT ( 'NONE',  ( -16.39453490553961856, 20.24836633112041184, -233.1722131570092245 ) ) ;
#12445=CARTESIAN_POINT ( 'NONE',  ( -2.723069588102707606, 15.58614045890443833, -225.0254611642426141 ) ) ;
#12446=CARTESIAN_POINT ( 'NONE',  ( 0.1556102272723409452, 19.71550568250159685, -232.1993058477363547 ) ) ;
#12447=CARTESIAN_POINT ( 'NONE',  ( -20.86570240061152148, 1.122719768445835875, -219.0984131021933763 ) ) ;
#12448=CARTESIAN_POINT ( 'NONE',  ( 13.21888801141564151, 2.135177519634172238, -228.0426311217386797 ) ) ;
#12450=CARTESIAN_POINT ( 'NONE',  ( 7.074707374710634156, -26.72731565888815553, -229.5909540767539738 ) ) ;
#12455=CARTESIAN_POINT ( 'NONE',  ( 5.069241901512100412, 14.34986542013820632, -229.6420000777802954 ) ) ;
#12456=CARTESIAN_POINT ( 'NONE',  ( 24.99579664921074240, -7.791002435033769657, -229.1824765006467715 ) ) ;
#12458=CARTESIAN_POINT ( 'NONE',  ( 16.91879448796214191, 0.8271603773820436212, -230.0510230802265710 ) ) ;
#12460=CARTESIAN_POINT ( 'NONE',  ( 6.053458391837899910, -12.85229775019162268, -220.9645494416007523 ) ) ;
#12462=CARTESIAN_POINT ( 'NONE',  ( -6.101488798441174310, 11.33371047077072369, -225.3616985956418546 ) ) ;
#12464=CARTESIAN_POINT ( 'NONE',  ( -10.30034651166687887, 25.05454868506992838, -216.5587736482213188 ) ) ;
#12466=CARTESIAN_POINT ( 'NONE',  ( -27.29953305526601426, 11.21644211419729054, -229.3676346105362995 ) ) ;
#12467=CARTESIAN_POINT ( 'NONE',  ( -9.776740361816679936, -16.43846667899986258, -218.0739489017842061 ) ) ;
#12469=CARTESIAN_POINT ( 'NONE',  ( 22.03647168421188596, 0.3315607655626346961, -232.0572713672587213 ) ) ;
#12470=CARTESIAN_POINT ( 'NONE',  ( -15.20262116893801974, 8.038155052917188570, -217.6767387945475036 ) ) ;
#12471=CARTESIAN_POINT ( 'NONE',  ( 4.894111852004805030, -16.26971588820515890, -218.1545738548100530 ) ) ;
#12474=CARTESIAN_POINT ( 'NONE',  ( 21.91535456744164279, 7.573568724377624406, -232.0371228855588868 ) ) ;
#12475=CARTESIAN_POINT ( 'NONE',  ( -7.352050649209116884, 10.05454564170545417, -223.7370967983176229 ) ) ;
#12477=CARTESIAN_POINT ( 'NONE',  ( 16.29563576379945999, 21.41235115595959826, -221.8114656550040991 ) ) ;
#12478=CARTESIAN_POINT ( 'NONE',  ( -2.076897692258683925, -29.27639190819841275, -225.1343076284445601 ) ) ;
#12480=CARTESIAN_POINT ( 'NONE',  ( 3.080453011304693511, 29.32691491905673331, -222.8956499783474499 ) ) ;
#12481=CARTESIAN_POINT ( 'NONE',  ( -18.02718827071834085, 20.33515877052379395, -229.5060669840136143 ) ) ;
#12482=CARTESIAN_POINT ( 'NONE',  ( -19.26845014167239611, 9.481468541508135672, -234.4856117705182328 ) ) ;
#12483=CARTESIAN_POINT ( 'NONE',  ( -10.44804907229818980, -15.26164834479392240, -220.3887109030195859 ) ) ;
#12486=CARTESIAN_POINT ( 'NONE',  ( -18.71530386740073126, -0.6857509888707814527, -217.6195632122020527 ) ) ;
#12487=CARTESIAN_POINT ( 'NONE',  ( 8.192339082998598698, -27.06056373437490947, -224.5174968915583236 ) ) ;
#12488=CARTESIAN_POINT ( 'NONE',  ( 10.57926812561479757, 10.00910231482511215, -225.8341706491384286 ) ) ;
#12489=CARTESIAN_POINT ( 'NONE',  ( -18.47334320050258327, 24.79293862780133040, -226.9986786077537317 ) ) ;
#12490=CARTESIAN_POINT ( 'NONE',  ( 26.75877786246624623, 11.80320999550499117, -231.5572967531201414 ) ) ;
#12491=CARTESIAN_POINT ( 'NONE',  ( 9.586902571418640662, 24.43292817174309661, -231.9968623198229807 ) ) ;
#12492=CARTESIAN_POINT ( 'NONE',  ( 13.47875474198669821, 0.7946461602593113405, -222.1045510852317761 ) ) ;
#12493=CARTESIAN_POINT ( 'NONE',  ( -8.803769170443210612, -17.82266517633203406, -233.6972128408098683 ) ) ;
#12494=CARTESIAN_POINT ( 'NONE',  ( 19.68037530048075112, -17.97179847169212508, -231.8517058357153076 ) ) ;
#12497=CARTESIAN_POINT ( 'NONE',  ( -16.85225081326727903, 6.237400186851330020, -234.5847093771173206 ) ) ;
#12498=CARTESIAN_POINT ( 'NONE',  ( -16.25683815890624473, -3.869351682469674980, -222.5551530127839044 ) ) ;
#12499=CARTESIAN_POINT ( 'NONE',  ( -25.64868633208605786, 12.30364128039660798, -229.0020209687957049 ) ) ;
#12500=CARTESIAN_POINT ( 'NONE',  ( 15.37089934297015503, 20.64239674606488961, -217.2018742121147170 ) ) ;
#12501=CARTESIAN_POINT ( 'NONE',  ( 5.791579991237209235, 15.48299465423324861, -228.0203551130359472 ) ) ;
#12503=CARTESIAN_POINT ( 'NONE',  ( 8.679960083554519201, -14.04048791834972398, -217.5462328905347249 ) ) ;
#12505=CARTESIAN_POINT ( 'NONE',  ( 15.87442104186276381, 8.674488492264579520, -230.9702037640878416 ) ) ;
#12506=CARTESIAN_POINT ( 'NONE',  ( -19.90771709537278156, 23.83218599423810602, -225.0439263757368735 ) ) ;
#12507=CARTESIAN_POINT ( 'NONE',  ( -17.94782256308196366, 19.07396065564992682, -232.7143578890335220 ) ) ;
#12508=CARTESIAN_POINT ( 'NONE',  ( -25.34460520202507539, -7.988444519707189606, -217.6292756219348234 ) ) ;
#12509=CARTESIAN_POINT ( 'NONE',  ( -26.74045434827795020, 12.41518252455047744, -220.4617428697642652 ) ) ;
#12510=CARTESIAN_POINT ( 'NONE',  ( 15.96089671440110713, 1.143943728337336374, -218.3532651118343892 ) ) ;
#12511=CARTESIAN_POINT ( 'NONE',  ( -10.65640919150578192, 23.79238421564942740, -218.1088542024188826 ) ) ;
#12512=CARTESIAN_POINT ( 'NONE',  ( 24.61409543538958289, 19.88121288930873476, -228.5015986536257344 ) ) ;
#12513=CARTESIAN_POINT ( 'NONE',  ( 19.29259174080182504, 0.5828707127177102931, -219.2781652733668807 ) ) ;
#12514=CARTESIAN_POINT ( 'NONE',  ( -17.83852468596024110, -8.357198216422425219, -233.0481596892792879 ) ) ;
#12515=CARTESIAN_POINT ( 'NONE',  ( 5.646952844456516019, 23.06006924884521325, -218.8221376988549878 ) ) ;
#12516=CARTESIAN_POINT ( 'NONE',  ( -0.1947256686167265494, -30.94043057420685727, -223.1178397439027492 ) ) ;
#12517=CARTESIAN_POINT ( 'NONE',  ( 4.343013938751969505, 13.02036404005131587, -224.7825435359082178 ) ) ;
#12518=CARTESIAN_POINT ( 'NONE',  ( 15.81704710165450756, -18.55181613945514840, -214.8869746720286287 ) ) ;
#12519=CARTESIAN_POINT ( 'NONE',  ( 22.00000000000000711, 0.000000000000000000, -233.0000000000000284 ) ) ;
#12521=CARTESIAN_POINT ( 'NONE',  ( -20.57288920227272655, 16.51351902378409520, -230.8484733908063333 ) ) ;
#12523=CARTESIAN_POINT ( 'NONE',  ( 19.75516891782859474, -3.344025276999063934, -216.3638920815759263 ) ) ;
#12524=CARTESIAN_POINT ( 'NONE',  ( 2.445562843591592372, 25.89340784564244657, -229.2671352353737859 ) ) ;
#12525=CARTESIAN_POINT ( 'NONE',  ( 19.55931020704464274, 3.833820734573247346, -215.4549349108404783 ) ) ;
#12526=CARTESIAN_POINT ( 'NONE',  ( 17.00168025137501004, 6.212099629982537508, -219.0548246536471595 ) ) ;
#12528=CARTESIAN_POINT ( 'NONE',  ( -15.95469971785872332, -24.72796590591627464, -225.3946449442874211 ) ) ;
#12529=CARTESIAN_POINT ( 'NONE',  ( 9.400341091271927851, 28.64465517894215196, -231.0823126271420165 ) ) ;
#12531=CARTESIAN_POINT ( 'NONE',  ( 0.3555517721839966394, -12.99484957898737569, -222.7951259809431974 ) ) ;
#12532=CARTESIAN_POINT ( 'NONE',  ( -14.22255565734842619, 21.32307452572284134, -218.8849463683180261 ) ) ;
#12533=CARTESIAN_POINT ( 'NONE',  ( 16.10596270516584028, 24.75152718569329835, -228.9330127594856492 ) ) ;
#12534=CARTESIAN_POINT ( 'NONE',  ( -21.99356461413155728, 5.827088221545293045, -219.1725956997024127 ) ) ;
#12536=CARTESIAN_POINT ( 'NONE',  ( -10.83439284573031536, 18.36737820296253432, -234.3014274143859836 ) ) ;
#12537=CARTESIAN_POINT ( 'NONE',  ( 20.88210880980788531, 0.9259446317980322139, -218.6312544800709929 ) ) ;
#12538=CARTESIAN_POINT ( 'NONE',  ( 7.436546160899932367, -15.25288503996851475, -221.8354696069030467 ) ) ;
#12540=CARTESIAN_POINT ( 'NONE',  ( 12.70013114424463296, -16.94540864491495924, -217.3462533088837745 ) ) ;
#12541=CARTESIAN_POINT ( 'NONE',  ( 0.4762409465891800919, 16.20008108839776284, -225.9988706007428050 ) ) ;
#12543=CARTESIAN_POINT ( 'NONE',  ( 15.76910524310159900, 5.601482066865847820, -220.3440822020379528 ) ) ;
#12544=CARTESIAN_POINT ( 'NONE',  ( -22.24434812881145618, 2.221346625544017961, -216.9231029185778254 ) ) ;
#12545=CARTESIAN_POINT ( 'NONE',  ( -11.20272313682045073, -7.956653478762055087, -225.3025344850567819 ) ) ;
#12546=CARTESIAN_POINT ( 'NONE',  ( 7.437838793555467731, -20.85539581353325289, -233.9154700400843865 ) ) ;
#12547=CARTESIAN_POINT ( 'NONE',  ( -6.067446494494625142, 16.28408815813367028, -230.0786439517394513 ) ) ;
#12549=CARTESIAN_POINT ( 'NONE',  ( 20.64430047260004031, 12.67811357335941480, -231.0449411089858813 ) ) ;
#12550=CARTESIAN_POINT ( 'NONE',  ( -10.45786516112131892, 23.61456281964591852, -233.2869923610001592 ) ) ;
#12551=CARTESIAN_POINT ( 'NONE',  ( -1.796846813493219619, 26.08418332695505271, -220.7262848173578504 ) ) ;
#12553=CARTESIAN_POINT ( 'NONE',  ( 2.485733319737138736, 14.76073968410796056, -221.5245536174130905 ) ) ;
#12554=CARTESIAN_POINT ( 'NONE',  ( 17.57135037026572277, 0.09191994211922807634, -232.8447871904542410 ) ) ;
#12555=CARTESIAN_POINT ( 'NONE',  ( 17.96045420455031305, -0.3746358454349600908, -217.9627609769914613 ) ) ;
#12556=CARTESIAN_POINT ( 'NONE',  ( 17.47229821656412341, -21.26691171910925249, -219.4940788861217413 ) ) ;
#12560=CARTESIAN_POINT ( 'NONE',  ( 5.248230734842167955, 23.54336384919183445, -216.8914391693808739 ) ) ;
#12561=CARTESIAN_POINT ( 'NONE',  ( 19.53765964318905546, -5.556987368099968627, -230.7409885362571345 ) ) ;
#12563=CARTESIAN_POINT ( 'NONE',  ( 15.10937218716165020, -26.44221868192832758, -222.7999243300199907 ) ) ;
#12565=CARTESIAN_POINT ( 'NONE',  ( -10.45786516112131892, 23.61456281964591852, -233.2869923610001592 ) ) ;
#12566=CARTESIAN_POINT ( 'NONE',  ( -8.123851230256436295, 20.56863949923577550, -215.0796075421103239 ) ) ;
#12568=CARTESIAN_POINT ( 'NONE',  ( -13.58874046263339608, 12.73011668665171392, -216.5659449791897941 ) ) ;
#12569=CARTESIAN_POINT ( 'NONE',  ( -11.57846532275044460, -10.37575015818511304, -229.3776965522603462 ) ) ;
#12573=CARTESIAN_POINT ( 'NONE',  ( -18.08305592660031991, 4.022743421239192152, -217.2335041149100050 ) ) ;
#12574=CARTESIAN_POINT ( 'NONE',  ( 8.479858146824877707, -14.20649975585062563, -220.0175458633526091 ) ) ;
#12576=CARTESIAN_POINT ( 'NONE',  ( -11.67631226053870996, 6.737291529340801333, -227.3110382950315227 ) ) ;
#12577=CARTESIAN_POINT ( 'NONE',  ( 19.79854089336508594, 4.557290221971136646, -217.3342919181881143 ) ) ;
#12578=CARTESIAN_POINT ( 'NONE',  ( -22.56222084847001597, 18.89892770556097901, -231.8972396388394088 ) ) ;
#12580=CARTESIAN_POINT ( 'NONE',  ( 10.79895562092076844, 12.01490073542734116, -225.7380208924852809 ) ) ;
#12581=CARTESIAN_POINT ( 'NONE',  ( -0.6720842648862578317, -17.90033647106004011, -231.4757128331908973 ) ) ;
#12582=ORIENTED_EDGE ( 'NONE', *, *, #10591, .F. ) ;
#12583=CARTESIAN_POINT ( 'NONE',  ( 2.951582164238582440, 19.39026647431845873, -217.4356918981242472 ) ) ;
#12584=CARTESIAN_POINT ( 'NONE',  ( -9.969679877803788060, 12.84542071557917176, -220.4758784541224657 ) ) ;
#12585=CARTESIAN_POINT ( 'NONE',  ( -10.94147694953847250, 13.90730769817462864, -218.7797619932150042 ) ) ;
#12586=CARTESIAN_POINT ( 'NONE',  ( -13.63268120803286720, -13.08481847960132249, -219.9337478264210404 ) ) ;
#12589=CARTESIAN_POINT ( 'NONE',  ( -13.93333636822611155, 3.327141996558931947, -221.4468162587888287 ) ) ;
#12590=CARTESIAN_POINT ( 'NONE',  ( 7.754512012237808172, -26.66010948812077430, -222.3649102068104924 ) ) ;
#12591=CARTESIAN_POINT ( 'NONE',  ( 26.48990917286906921, 12.16675355942207659, -225.0153622588060216 ) ) ;
#12592=CARTESIAN_POINT ( 'NONE',  ( -3.082945806077231676, 30.69897765966285874, -224.2387254578930822 ) ) ;
#12594=CARTESIAN_POINT ( 'NONE',  ( -27.32994399549947673, 3.379920396491164603, -227.9326384921875217 ) ) ;
#12596=CARTESIAN_POINT ( 'NONE',  ( 5.017623471397871349, 29.83561274492976878, -222.9769172135417250 ) ) ;
#12597=CARTESIAN_POINT ( 'NONE',  ( 13.51280905378919606, 1.666897247961874884, -222.5030422686260465 ) ) ;
#12598=CARTESIAN_POINT ( 'NONE',  ( -17.42499862437977853, -18.98713029041037004, -232.7811807006768845 ) ) ;
#12599=CARTESIAN_POINT ( 'NONE',  ( 15.84759643368428428, -7.142586963752317608, -231.1761396821659673 ) ) ;
#12603=CARTESIAN_POINT ( 'NONE',  ( -21.64120863631820413, 17.87363223393748868, -233.1390268986752119 ) ) ;
#12604=CARTESIAN_POINT ( 'NONE',  ( -16.74998343472315199, -3.152285961911668988, -228.0274629056708022 ) ) ;
#12605=CARTESIAN_POINT ( 'NONE',  ( -20.57288920227272655, 16.51351902378409520, -230.8484733908063333 ) ) ;
#12606=CARTESIAN_POINT ( 'NONE',  ( 27.79746884017060538, 13.63637251724950339, -226.5788410723774575 ) ) ;
#12607=CARTESIAN_POINT ( 'NONE',  ( 0.3355639943343493026, 23.87279439325363128, -218.0067922387550823 ) ) ;
#12609=CARTESIAN_POINT ( 'NONE',  ( 10.18197402670511842, -10.22146582328408115, -231.5691222609812598 ) ) ;
#12610=CARTESIAN_POINT ( 'NONE',  ( 28.51464931495100785, 5.422321182929326966, -223.8116416110474347 ) ) ;
#12611=CARTESIAN_POINT ( 'NONE',  ( -0.04850409037381671340, 14.20520396026658716, -231.8092226852533031 ) ) ;
#12612=CARTESIAN_POINT ( 'NONE',  ( -3.309130212696198559, 28.80211350556483296, -217.4284252357080334 ) ) ;
#12613=CARTESIAN_POINT ( 'NONE',  ( -11.96453848309674228, -6.796862595549911568, -223.8262896469332759 ) ) ;
#12614=CARTESIAN_POINT ( 'NONE',  ( -13.83274569775339202, 16.20364235096346661, -234.0851861771356539 ) ) ;
#12617=CARTESIAN_POINT ( 'NONE',  ( 24.56541673123750158, -5.996287403333383281, -231.6940117905984664 ) ) ;
#12618=CARTESIAN_POINT ( 'NONE',  ( 1.867752180833619713, 31.25122076096762669, -227.4007918511463231 ) ) ;
#12619=CARTESIAN_POINT ( 'NONE',  ( 26.50744623559791435, 1.694095366541529923, -217.6968951254705473 ) ) ;
#12620=CARTESIAN_POINT ( 'NONE',  ( 28.56567312134318826, 3.451746495494312672, -224.1550573921799412 ) ) ;
#12621=CARTESIAN_POINT ( 'NONE',  ( 12.58590500897257947, 11.38573988265384607, -230.4867078522624695 ) ) ;
#12622=CARTESIAN_POINT ( 'NONE',  ( -17.60306105620566441, -10.62493847279374926, -216.8163279515337649 ) ) ;
#12624=CARTESIAN_POINT ( 'NONE',  ( 4.936777854427027989, 27.97379167488809060, -227.0886654730259124 ) ) ;
#12625=CARTESIAN_POINT ( 'NONE',  ( -1.542335193334551491, -19.71915426430242135, -216.1352730594569209 ) ) ;
#12626=CARTESIAN_POINT ( 'NONE',  ( 14.39473142419577023, 15.98257177912839389, -217.4557725731239373 ) ) ;
#12627=CARTESIAN_POINT ( 'NONE',  ( 7.141633727147962851, -29.98958059360777639, -229.8804610602846594 ) ) ;
#12629=CARTESIAN_POINT ( 'NONE',  ( -12.87285471141929172, 9.485162256560764504, -229.1865421006261840 ) ) ;
#12631=CARTESIAN_POINT ( 'NONE',  ( -22.94312929380076937, -2.351969141711130806, -217.0768970835230505 ) ) ;
#12632=CARTESIAN_POINT ( 'NONE',  ( 12.83388873239664996, 22.07510045760132655, -230.4740059944613222 ) ) ;
#12633=CARTESIAN_POINT ( 'NONE',  ( -12.05423124486310904, 12.38527783110887803, -219.7419643105747014 ) ) ;
#12634=CARTESIAN_POINT ( 'NONE',  ( -17.92628912275201003, -0.6090139417824500523, -215.7724435048976943 ) ) ;
#12635=CARTESIAN_POINT ( 'NONE',  ( -8.288471666609035893, -17.31860360376325403, -217.6655967056599366 ) ) ;
#12636=CARTESIAN_POINT ( 'NONE',  ( 27.79290571682592770, 12.05347838982552666, -230.1298045326732051 ) ) ;
#12638=CARTESIAN_POINT ( 'NONE',  ( -10.91546170668013005, -7.896971223757457636, -230.5866998909293102 ) ) ;
#12639=CARTESIAN_POINT ( 'NONE',  ( 7.772443558932104146, 25.24620711463332157, -231.7813173736589931 ) ) ;
#12640=CARTESIAN_POINT ( 'NONE',  ( 11.43247012502872728, 12.44034019618676190, -231.9336559008378629 ) ) ;
#12642=CARTESIAN_POINT ( 'NONE',  ( -15.15469129103955304, 15.56563882170958024, -231.6314069158229643 ) ) ;
#12644=CARTESIAN_POINT ( 'NONE',  ( 3.044038000507106378, 30.22621415828681180, -231.1553244844465382 ) ) ;
#12645=CARTESIAN_POINT ( 'NONE',  ( 15.18181359483165949, 6.369295616116027681, -230.7949408486033462 ) ) ;
#12647=CARTESIAN_POINT ( 'NONE',  ( 15.70595326690115634, -18.65841243762358559, -219.6423885132037981 ) ) ;
#12648=CARTESIAN_POINT ( 'NONE',  ( 5.452943511046377090, -14.64908918772281865, -221.6090591728701611 ) ) ;
#12651=CARTESIAN_POINT ( 'NONE',  ( 21.31262902390056624, 0.4111834581965390645, -232.0572713672585792 ) ) ;
#12652=CARTESIAN_POINT ( 'NONE',  ( 14.62702828724412285, -1.994068170757606673, -224.0552340365271959 ) ) ;
#12653=CARTESIAN_POINT ( 'NONE',  ( -12.13177435108894642, -8.392035797555511323, -228.8392847287196332 ) ) ;
#12654=CARTESIAN_POINT ( 'NONE',  ( 1.292981098121811279, -26.53499626907933262, -232.9055005154886828 ) ) ;
#12655=CARTESIAN_POINT ( 'NONE',  ( 6.295505112925526170, 15.36201163567862693, -221.5772643759389098 ) ) ;
#12657=CARTESIAN_POINT ( 'NONE',  ( -11.30246491834384770, 5.534029070539333794, -225.8243940897388597 ) ) ;
#12658=CARTESIAN_POINT ( 'NONE',  ( -7.825349071214003693, 24.14595706726266755, -216.5959661901539732 ) ) ;
#12659=CARTESIAN_POINT ( 'NONE',  ( 0.4762409465891800919, 16.20008108839776284, -225.9988706007428050 ) ) ;
#12660=CARTESIAN_POINT ( 'NONE',  ( -24.25245498015852874, 0.2109992039763788352, -218.1398602137601301 ) ) ;
#12662=CARTESIAN_POINT ( 'NONE',  ( 14.60728983664449387, 19.38727400458104455, -216.6381802409380555 ) ) ;
#12663=CARTESIAN_POINT ( 'NONE',  ( -15.82068653568960137, 8.372322471091806051, -220.7139663195713979 ) ) ;
#12664=CARTESIAN_POINT ( 'NONE',  ( 12.66989206167516357, 2.082990619159506007, -225.6419847029432901 ) ) ;
#12665=CARTESIAN_POINT ( 'NONE',  ( 2.283233934795953601, -16.37150177406293849, -220.5471140349473842 ) ) ;
#12669=CARTESIAN_POINT ( 'NONE',  ( 13.43170911749896490, 19.07691563292472026, -232.7497845103644636 ) ) ;
#12670=CARTESIAN_POINT ( 'NONE',  ( -17.01570095888788003, -2.024181990473361115, -234.1256067144893791 ) ) ;
#12671=CARTESIAN_POINT ( 'NONE',  ( -15.30864812529618391, 1.596444765892653717, -220.3859421844601627 ) ) ;
#12672=CARTESIAN_POINT ( 'NONE',  ( -1.177898122437396333, -26.14463525305933445, -216.8677949074964033 ) ) ;
#12674=CARTESIAN_POINT ( 'NONE',  ( -11.26857159993117996, 28.96895336474501192, -225.6039696848669678 ) ) ;
#12675=CARTESIAN_POINT ( 'NONE',  ( -21.66801938871533650, 16.28801167444048659, -218.5240035253498547 ) ) ;
#12677=CARTESIAN_POINT ( 'NONE',  ( -15.48255455842386219, 10.01793346089237069, -233.1197357361336913 ) ) ;
#12678=CARTESIAN_POINT ( 'NONE',  ( -10.06927776881013514, -17.00317020600589402, -217.8513858272130790 ) ) ;
#12681=CARTESIAN_POINT ( 'NONE',  ( -10.30050448363967419, 10.07750059423401190, -220.1837019037183723 ) ) ;
#12682=CARTESIAN_POINT ( 'NONE',  ( 7.813662449283098610, -13.08401493520405445, -221.9442578939891177 ) ) ;
#12684=CARTESIAN_POINT ( 'NONE',  ( -19.25929423112888017, 9.818144317380269825, -216.1837936240308409 ) ) ;
#12686=CARTESIAN_POINT ( 'NONE',  ( -13.63442241228529994, 1.608023091903783008, -219.2326980015357094 ) ) ;
#12687=CARTESIAN_POINT ( 'NONE',  ( -1.336753021691559962, 16.04398320409420720, -230.2310715620304507 ) ) ;
#12689=CARTESIAN_POINT ( 'NONE',  ( 14.65309016725241698, 3.424799466898550637, -221.5217808432381048 ) ) ;
#12690=CARTESIAN_POINT ( 'NONE',  ( -14.13544422886439911, -23.73189729233824252, -223.0800202563271171 ) ) ;
#12692=CARTESIAN_POINT ( 'NONE',  ( -6.720912670637915198, 19.69156892798266512, -217.8848069150180891 ) ) ;
#12693=CARTESIAN_POINT ( 'NONE',  ( -10.07004052286948337, 22.64471483900350179, -217.4645417110143626 ) ) ;
#12694=CARTESIAN_POINT ( 'NONE',  ( -10.52776196018457711, 13.57482816453351937, -219.2327734183297423 ) ) ;
#12696=CARTESIAN_POINT ( 'NONE',  ( -9.770823421170108602, -12.84821564276127503, -225.3905567659999178 ) ) ;
#12699=CARTESIAN_POINT ( 'NONE',  ( -14.87984907657228639, 0.2138881189739126887, -228.7773920408832282 ) ) ;
#12700=CARTESIAN_POINT ( 'NONE',  ( -1.243024450407066439, -19.42038079238686876, -231.9048276842376595 ) ) ;
#12701=CARTESIAN_POINT ( 'NONE',  ( 18.29617186523616468, 23.20920553663278341, -223.4372550713720216 ) ) ;
#12702=CARTESIAN_POINT ( 'NONE',  ( 0.9908753270255351575, 13.79205759140780430, -228.0165926715089881 ) ) ;
#12705=CARTESIAN_POINT ( 'NONE',  ( -23.30382222616342247, 9.914163031146200566, -218.5285240371296425 ) ) ;
#12706=CARTESIAN_POINT ( 'NONE',  ( 21.14441169763230732, 12.98245189690719315, -217.0976687089155064 ) ) ;
#12707=CARTESIAN_POINT ( 'NONE',  ( 18.76922974182421555, 13.12635134380198210, -217.8010375391909008 ) ) ;
#12709=CARTESIAN_POINT ( 'NONE',  ( -13.05629324012484282, -10.24599397043673221, -218.7452066004821347 ) ) ;
#12710=CARTESIAN_POINT ( 'NONE',  ( 1.623338700557370951, -21.82196275546919040, -234.1129525514646730 ) ) ;
#12713=CARTESIAN_POINT ( 'NONE',  ( -7.099035520468861549, 19.73710792467281649, -233.8745459908100770 ) ) ;
#12714=CARTESIAN_POINT ( 'NONE',  ( 13.85225051576513700, -1.547701942753643145, -218.6451083988944788 ) ) ;
#12717=CARTESIAN_POINT ( 'NONE',  ( 10.95881707662767290, 12.06788758096456782, -231.4359029166177208 ) ) ;
#12718=CARTESIAN_POINT ( 'NONE',  ( 10.32480721127626033, 15.84468581819879773, -230.0799086455579072 ) ) ;
#12720=CARTESIAN_POINT ( 'NONE',  ( 11.84677440217253341, -6.023754617643652054, -230.4469913264703962 ) ) ;
#12721=CARTESIAN_POINT ( 'NONE',  ( 16.00819137755116373, 4.595691552992191120, -229.5669508871464757 ) ) ;
#12722=CARTESIAN_POINT ( 'NONE',  ( -1.584125552723561592, 20.48724127025963782, -214.7515060525244621 ) ) ;
#12723=CARTESIAN_POINT ( 'NONE',  ( -11.59874896804548250, 27.28969409813203484, -218.8626241359735332 ) ) ;
#12724=CARTESIAN_POINT ( 'NONE',  ( -24.65069530437947876, -0.7989515219415058711, -216.4419420286324112 ) ) ;
#12726=CARTESIAN_POINT ( 'NONE',  ( -17.65835845419170624, 22.55329142274348442, -231.2673511165784532 ) ) ;
#12729=CARTESIAN_POINT ( 'NONE',  ( 25.69761320619099720, -8.403105518750903613, -219.2599777650661110 ) ) ;
#12731=CARTESIAN_POINT ( 'NONE',  ( -1.585416880194127520, 15.28258783379090424, -231.0852564988603319 ) ) ;
#12732=CARTESIAN_POINT ( 'NONE',  ( 27.08260752785270853, 4.114838227474355570, -232.2882281786467331 ) ) ;
#12733=CARTESIAN_POINT ( 'NONE',  ( -22.04257564474043818, 18.72061943465525857, -219.1781831295219263 ) ) ;
#12735=CARTESIAN_POINT ( 'NONE',  ( 11.33210854356620523, 22.81476816607802149, -217.8536224460118262 ) ) ;
#12737=CARTESIAN_POINT ( 'NONE',  ( -1.336753021691559962, 16.04398320409420720, -230.2310715620304507 ) ) ;
#12738=CARTESIAN_POINT ( 'NONE',  ( -14.40111287326894640, -6.123720356435734757, -220.5571602876142094 ) ) ;
#12739=CARTESIAN_POINT ( 'NONE',  ( 3.763426558366607111, 28.60172112197566818, -230.1816715025297526 ) ) ;
#12740=CARTESIAN_POINT ( 'NONE',  ( 9.191046577198441980, -13.34937224525895161, -233.4761082295262611 ) ) ;
#12742=CARTESIAN_POINT ( 'NONE',  ( -21.23733589435050817, 17.25275849955597351, -229.9547908233139708 ) ) ;
#12743=CARTESIAN_POINT ( 'NONE',  ( 12.90474009670415967, -3.145873754258878385, -224.5449843457338375 ) ) ;
#12744=CARTESIAN_POINT ( 'NONE',  ( 6.729623925010410623, 16.84721552001897038, -219.9221131804260381 ) ) ;
#12745=CARTESIAN_POINT ( 'NONE',  ( -22.07068341299880743, 18.38202870573248049, -227.7785760498121306 ) ) ;
#12746=CARTESIAN_POINT ( 'NONE',  ( -11.80036766549451599, 3.629178540272184783, -221.4826559383200220 ) ) ;
#12747=CARTESIAN_POINT ( 'NONE',  ( -8.537495277687638051, -14.12518193842558212, -230.5589415009361858 ) ) ;
#12748=CARTESIAN_POINT ( 'NONE',  ( 10.90540179105271967, 5.382827416078996841, -224.1493061458977820 ) ) ;
#12751=CARTESIAN_POINT ( 'NONE',  ( -20.52308621596579030, -13.62600152083235905, -234.9101091540371442 ) ) ;
#12752=CARTESIAN_POINT ( 'NONE',  ( -0.1881941282075867139, 17.37563936270229092, -230.9177995227891813 ) ) ;
#12753=CARTESIAN_POINT ( 'NONE',  ( 13.16746181015946959, 0.3897807143096829741, -227.1676274388083243 ) ) ;
#12754=CARTESIAN_POINT ( 'NONE',  ( -6.255852670334142829, 13.96671599789818252, -220.4426911866496823 ) ) ;
#12755=CARTESIAN_POINT ( 'NONE',  ( 13.09827881591457022, 28.40264942367575784, -221.1045935444571455 ) ) ;
#12756=CARTESIAN_POINT ( 'NONE',  ( 19.30248206944178335, -1.297331563427565726, -230.8957665284791290 ) ) ;
#12757=CARTESIAN_POINT ( 'NONE',  ( -3.917974041549708630, -18.23196399112299559, -217.4080104222929606 ) ) ;
#12758=CARTESIAN_POINT ( 'NONE',  ( 2.936803900436826709, -18.74190719154852758, -218.5197582523356061 ) ) ;
#12760=CARTESIAN_POINT ( 'NONE',  ( 24.58316096239279602, 5.861425670879941485, -231.3104446318280623 ) ) ;
#12761=CARTESIAN_POINT ( 'NONE',  ( 11.31395536621571019, -8.070181239749643964, -225.0898076798974614 ) ) ;
#12762=CARTESIAN_POINT ( 'NONE',  ( -11.07688804854283049, -12.81333559660784971, -232.1241261852632363 ) ) ;
#12764=CARTESIAN_POINT ( 'NONE',  ( -6.052919920376759855, -15.38051382379660836, -218.0337201863237624 ) ) ;
#12766=CARTESIAN_POINT ( 'NONE',  ( 3.325336547283623378, 18.92213121405483633, -219.7480163085221818 ) ) ;
#12768=CARTESIAN_POINT ( 'NONE',  ( -16.36835685385702988, 8.002698209344293545, -233.7585018083067894 ) ) ;
#12769=CARTESIAN_POINT ( 'NONE',  ( -5.807479211365208727, 19.77444019604324410, -216.0778658752277863 ) ) ;
#12770=CARTESIAN_POINT ( 'NONE',  ( -2.015708574708954259, 26.78900769828807782, -221.5371848586876808 ) ) ;
#12771=CARTESIAN_POINT ( 'NONE',  ( 27.20328812258980378, -0.4806365347271125965, -218.3128023695579998 ) ) ;
#12773=CARTESIAN_POINT ( 'NONE',  ( 14.20064147608437821, 14.63411858269657806, -233.6150408276221242 ) ) ;
#12774=CARTESIAN_POINT ( 'NONE',  ( -15.50322565568834321, 9.749075856218723857, -229.6019304695566916 ) ) ;
#12775=CARTESIAN_POINT ( 'NONE',  ( 13.12946830070648652, 6.370976456471619365, -231.5124810213676483 ) ) ;
#12776=CARTESIAN_POINT ( 'NONE',  ( 1.102456202203287550, -23.13885590315818064, -232.0370787247644557 ) ) ;
#12778=DIRECTION ( 'NONE',  ( -0.9940043559354330149, -0.1093404791528966163, -6.737719923507020479E-14 ) ) ;
#12779=CARTESIAN_POINT ( 'NONE',  ( 18.23324537670537993, 23.47692953258263771, -224.8333321331434433 ) ) ;
#12780=CARTESIAN_POINT ( 'NONE',  ( 20.53618124091710939, -19.36892006637360097, -226.5121684596580849 ) ) ;
#12784=CARTESIAN_POINT ( 'NONE',  ( -15.48425879135615446, -25.29886615046042309, -220.6886037686364261 ) ) ;
#12786=CARTESIAN_POINT ( 'NONE',  ( 4.484811161826725900, 15.38298568785217313, -219.4617573400562662 ) ) ;
#12787=CARTESIAN_POINT ( 'NONE',  ( -4.334570222994868161, 11.62786715207288601, -222.6396919303362267 ) ) ;
#12789=CARTESIAN_POINT ( 'NONE',  ( -6.855867220396999251, 12.17758473459128332, -220.6375607554995213 ) ) ;
#12790=CARTESIAN_POINT ( 'NONE',  ( 28.44445586451508845, -4.662230540760189612, -220.9797193573593290 ) ) ;
#12793=CARTESIAN_POINT ( 'NONE',  ( -2.698926868850080041, 12.89339462271858316, -226.7595176699009585 ) ) ;
#12794=CARTESIAN_POINT ( 'NONE',  ( 7.829076659910394476, -15.59360078984655651, -230.7142312655459762 ) ) ;
#12796=CARTESIAN_POINT ( 'NONE',  ( -19.00318367631585659, 13.14621133775862916, -233.8403879275295765 ) ) ;
#12797=CARTESIAN_POINT ( 'NONE',  ( -21.39667546302236900, 3.687493526428279100, -235.1435990565495047 ) ) ;
#12798=CARTESIAN_POINT ( 'NONE',  ( -6.702936938788568888, 25.88675107068059944, -218.1129661040884287 ) ) ;
#12800=CARTESIAN_POINT ( 'NONE',  ( 28.52435124311170966, 7.611291969169514005, -224.8315247833735384 ) ) ;
#12801=CARTESIAN_POINT ( 'NONE',  ( -7.205518813659622879, -14.37210213534873482, -226.5338589405291998 ) ) ;
#12805=CARTESIAN_POINT ( 'NONE',  ( 14.60728983664449387, 19.38727400458104455, -216.6381802409380555 ) ) ;
#12806=CARTESIAN_POINT ( 'NONE',  ( -12.96364545172611571, 10.77137376900670063, -221.1208843751685720 ) ) ;
#12807=CARTESIAN_POINT ( 'NONE',  ( -13.96653539523557619, 20.94398119165846239, -231.8597527081015528 ) ) ;
#12808=CARTESIAN_POINT ( 'NONE',  ( -20.80379704402785990, -7.385557752804055909, -217.9407440132496845 ) ) ;
#12811=CARTESIAN_POINT ( 'NONE',  ( -14.29986196492902550, 0.06805469746732484282, -227.4167624117703213 ) ) ;
#12812=CARTESIAN_POINT ( 'NONE',  ( -6.241914139598351952, -12.26321662989467320, -220.9276712261616353 ) ) ;
#12813=CARTESIAN_POINT ( 'NONE',  ( 20.34032485158648029, 2.741617426884598530, -217.9827731991294968 ) ) ;
#12814=CARTESIAN_POINT ( 'NONE',  ( -7.825349071214003693, 24.14595706726266755, -216.5959661901539732 ) ) ;
#12817=CARTESIAN_POINT ( 'NONE',  ( -15.51814470728089645, 2.949994979016113739, -222.8331727603033130 ) ) ;
#12818=CARTESIAN_POINT ( 'NONE',  ( 18.69149182921226782, 24.00661454656289706, -229.8257469855424517 ) ) ;
#12819=CARTESIAN_POINT ( 'NONE',  ( 17.68508104102419409, 23.41266195669770767, -227.5327139115408954 ) ) ;
#12821=CARTESIAN_POINT ( 'NONE',  ( -12.37311134093142506, -6.729359123088276995, -218.5215259163429380 ) ) ;
#12822=CARTESIAN_POINT ( 'NONE',  ( -11.40116373163465369, -15.95513543764466213, -216.7841692646331353 ) ) ;
#12823=CARTESIAN_POINT ( 'NONE',  ( 7.021536848793814123, -14.49751826649810482, -218.4909385705359455 ) ) ;
#12826=CARTESIAN_POINT ( 'NONE',  ( -11.19105919052231179, 21.17456633634251872, -216.2128528132037957 ) ) ;
#12827=CARTESIAN_POINT ( 'NONE',  ( 13.86864723624500328, -7.301706307425273046, -233.2436966314882909 ) ) ;
#12828=CARTESIAN_POINT ( 'NONE',  ( 25.54997870115619207, -2.097555195297153841, -218.7002440566220400 ) ) ;
#12829=CARTESIAN_POINT ( 'NONE',  ( -13.37045227479810094, 5.250293981428504786, -224.2914120185227205 ) ) ;
#12830=CARTESIAN_POINT ( 'NONE',  ( 7.018811797190238622, 13.93862807232938472, -230.2855929063610176 ) ) ;
#12831=CARTESIAN_POINT ( 'NONE',  ( 9.653903571287008489, 19.16609876806546353, -219.1149796918802792 ) ) ;
#12833=CARTESIAN_POINT ( 'NONE',  ( 7.462112298232926655, -14.04285870004232528, -232.2430251799377174 ) ) ;
#12835=CARTESIAN_POINT ( 'NONE',  ( -9.578110717394128670, 23.64032677849093034, -215.7669555765890550 ) ) ;
#12836=CARTESIAN_POINT ( 'NONE',  ( -14.30586181932858914, 18.69563132175512266, -215.8217153853723573 ) ) ;
#12837=CARTESIAN_POINT ( 'NONE',  ( -12.18037021406049547, -6.685450889859271051, -226.7642181357440734 ) ) ;
#12838=CARTESIAN_POINT ( 'NONE',  ( -11.02345917017863464, 29.02019856777526741, -223.9475008740665771 ) ) ;
#12839=CARTESIAN_POINT ( 'NONE',  ( -21.08008464085897060, -0.9048411197481797119, -217.0000000010748522 ) ) ;
#12841=CARTESIAN_POINT ( 'NONE',  ( 28.36095019830170472, -8.296631283839911220, -225.2861439608085448 ) ) ;
#12842=CARTESIAN_POINT ( 'NONE',  ( -2.121548062149551495, 13.26065194155116345, -221.8830439064491884 ) ) ;
#12843=CARTESIAN_POINT ( 'NONE',  ( -20.67624351032310059, -0.8683020119106035217, -219.0957770725675005 ) ) ;
#12844=CARTESIAN_POINT ( 'NONE',  ( -28.13472254077564116, 12.33996625515159629, -224.9141344439281909 ) ) ;
#12845=CARTESIAN_POINT ( 'NONE',  ( 18.04365516558436866, 6.721233635139160612, -218.4376093631473168 ) ) ;
#12848=CARTESIAN_POINT ( 'NONE',  ( -9.290933312444883185, 29.15551353946876745, -225.8551562993724247 ) ) ;
#12849=CARTESIAN_POINT ( 'NONE',  ( -23.54665576872953636, -14.78900941482413067, -230.7594827126482073 ) ) ;
#12850=CARTESIAN_POINT ( 'NONE',  ( 20.41153371889344825, 17.18812948447019551, -230.7531656956970778 ) ) ;
#12851=CARTESIAN_POINT ( 'NONE',  ( -7.913663017152074097, -13.07021161337726944, -228.8713148165744258 ) ) ;
#12853=CARTESIAN_POINT ( 'NONE',  ( -26.38808873681881906, 13.30696350521622939, -225.1492950792419663 ) ) ;
#12854=CARTESIAN_POINT ( 'NONE',  ( 15.69671663880151868, -19.77919342852767315, -217.9503656454650411 ) ) ;
#12855=CARTESIAN_POINT ( 'NONE',  ( 5.688640247940316641, 20.34961083808282822, -230.9155060479073711 ) ) ;
#12856=CARTESIAN_POINT ( 'NONE',  ( -17.49393085256189906, 10.63366922396483361, -217.7502683347138657 ) ) ;
#12857=CARTESIAN_POINT ( 'NONE',  ( -21.73153953336191790, 8.758376218440917071, -235.2971293019126051 ) ) ;
#12858=CARTESIAN_POINT ( 'NONE',  ( -5.234434610370643171, -17.78654814248861626, -233.1081320952062867 ) ) ;
#12859=CARTESIAN_POINT ( 'NONE',  ( 13.72784977962315267, 2.687686193488206143, -220.8507880271885995 ) ) ;
#12861=CARTESIAN_POINT ( 'NONE',  ( -12.06899374386015644, -4.263779665926158202, -221.6855044605631520 ) ) ;
#12862=CARTESIAN_POINT ( 'NONE',  ( -0.9249541874382023465, 14.55235618511626328, -223.7321818898853962 ) ) ;
#12863=CARTESIAN_POINT ( 'NONE',  ( 20.05202556141620107, 8.012988804822112954, -215.8722494878839200 ) ) ;
#12864=CARTESIAN_POINT ( 'NONE',  ( -12.66290653391502907, 23.44312233264792411, -230.9359094203250606 ) ) ;
#12865=CARTESIAN_POINT ( 'NONE',  ( 6.839751633953758514, 19.11639828585652623, -235.1218211620789873 ) ) ;
#12866=CARTESIAN_POINT ( 'NONE',  ( -2.821634405314548566, -24.60373223977012458, -232.0829149086248435 ) ) ;
#12867=CARTESIAN_POINT ( 'NONE',  ( 1.366658787427950772, -15.59113167952139456, -228.2894046839634257 ) ) ;
#12868=CARTESIAN_POINT ( 'NONE',  ( 18.06016678184731461, 2.257982981100609354, -218.9983079406065940 ) ) ;
#12869=CARTESIAN_POINT ( 'NONE',  ( 18.55298002304457228, -12.22359628793950570, -216.9137843736221782 ) ) ;
#12870=CARTESIAN_POINT ( 'NONE',  ( -15.51091956967506391, -1.782849713491490018, -228.8089183834494520 ) ) ;
#12871=CARTESIAN_POINT ( 'NONE',  ( -9.078153229956912540, -10.71731945587431056, -228.5228069477245469 ) ) ;
#12872=CARTESIAN_POINT ( 'NONE',  ( 15.03112630398312177, 24.11065413595933293, -226.8236212149936080 ) ) ;
#12873=CARTESIAN_POINT ( 'NONE',  ( -23.49520248890869212, 11.82830312093803649, -233.3871405502527807 ) ) ;
#12874=CARTESIAN_POINT ( 'NONE',  ( 4.883314309504700468, 19.06839645569368358, -217.0171359871271193 ) ) ;
#12875=CARTESIAN_POINT ( 'NONE',  ( 4.152856881432678726, 16.71326706899027670, -228.3712188091315909 ) ) ;
#12876=CARTESIAN_POINT ( 'NONE',  ( 30.21546680466445167, 0.1681144524405517038, -223.7059097242262737 ) ) ;
#12878=CARTESIAN_POINT ( 'NONE',  ( 17.29648694364601980, 10.20782262162153842, -233.8400727604031317 ) ) ;
#12879=CARTESIAN_POINT ( 'NONE',  ( -13.23768812067001477, 12.78288831771969569, -230.4179793829127902 ) ) ;
#12880=CARTESIAN_POINT ( 'NONE',  ( -28.00010259152825398, 3.831607968041374157, -225.8381323513402208 ) ) ;
#12881=CARTESIAN_POINT ( 'NONE',  ( -5.139154528335864391, -14.05392405596956529, -226.2842807754188641 ) ) ;
#12884=CARTESIAN_POINT ( 'NONE',  ( 2.008896548638861024, 20.64812324442097591, -233.5818019448501843 ) ) ;
#12885=CARTESIAN_POINT ( 'NONE',  ( 14.64841443880303373, -15.14843974207636101, -218.3573740752273125 ) ) ;
#12888=CARTESIAN_POINT ( 'NONE',  ( -13.60146639818222702, -25.11808310587244009, -230.9974232610874196 ) ) ;
#12891=CARTESIAN_POINT ( 'NONE',  ( 5.141746912158045468, 22.01688500372448232, -216.6678693612369386 ) ) ;
#12892=CARTESIAN_POINT ( 'NONE',  ( 1.920320557106582893, 25.99317453242502296, -234.5637964893073217 ) ) ;
#12894=CARTESIAN_POINT ( 'NONE',  ( -15.58461825850822180, 18.91734573546571951, -233.7691177939990723 ) ) ;
#12895=CARTESIAN_POINT ( 'NONE',  ( -30.71739798481564421, -2.702902032605977389, -225.9472362185736642 ) ) ;
#12896=CARTESIAN_POINT ( 'NONE',  ( 28.19769730429874599, -1.268543021275377658, -231.5188709829604363 ) ) ;
#12899=CARTESIAN_POINT ( 'NONE',  ( -11.42613629117093765, 28.09170287990588832, -228.7150250545069241 ) ) ;
#12900=CARTESIAN_POINT ( 'NONE',  ( -20.50691009226094863, -22.90269851828495007, -230.6242067303112435 ) ) ;
#12901=CARTESIAN_POINT ( 'NONE',  ( 13.82188917133564132, -5.740199443570373816, -227.9076376976435654 ) ) ;
#12902=CARTESIAN_POINT ( 'NONE',  ( -12.74846050492543625, 19.93509882904884734, -216.0172840992881049 ) ) ;
#12903=CARTESIAN_POINT ( 'NONE',  ( -13.84508897751235246, 5.904954704487344941, -218.7722818424232401 ) ) ;
#12904=CARTESIAN_POINT ( 'NONE',  ( 0.3355639943343493026, 23.87279439325363128, -218.0067922387550823 ) ) ;
#12906=CARTESIAN_POINT ( 'NONE',  ( 20.41968681625622040, 10.18377600976054076, -218.1989382652844256 ) ) ;
#12907=CARTESIAN_POINT ( 'NONE',  ( -16.83358080157556103, -19.16169236771116857, -229.6922051654298116 ) ) ;
#12909=CARTESIAN_POINT ( 'NONE',  ( 16.10596270516584028, 24.75152718569329835, -228.9330127594856492 ) ) ;
#12910=CARTESIAN_POINT ( 'NONE',  ( -14.46024998630872282, 14.54669730493860946, -231.4156670963686508 ) ) ;
#12911=CARTESIAN_POINT ( 'NONE',  ( -15.57505478537380306, 24.84242291948262249, -225.5907943047649837 ) ) ;
#12913=CARTESIAN_POINT ( 'NONE',  ( 27.12528000378512871, -1.050705938820645224, -232.4139529590446784 ) ) ;
#12916=CARTESIAN_POINT ( 'NONE',  ( -13.98136146596813845, 3.850743984385103680, -228.7620665878280590 ) ) ;
#12917=CARTESIAN_POINT ( 'NONE',  ( -12.16163208632051784, -17.84934472108236747, -234.2417547270719638 ) ) ;
#12918=CARTESIAN_POINT ( 'NONE',  ( 14.22574309452842733, 4.476723532073429546, -225.5862451792618231 ) ) ;
#12919=CARTESIAN_POINT ( 'NONE',  ( -2.208416658185406334, 29.10348627872611615, -219.8480645685746424 ) ) ;
#12921=CARTESIAN_POINT ( 'NONE',  ( -17.65933056022148762, 0.7424667221540405260, -229.0964312085266386 ) ) ;
#12922=CARTESIAN_POINT ( 'NONE',  ( 13.06625079052675531, 10.14096931681969238, -232.1435240729728093 ) ) ;
#12924=ADVANCED_FACE ( 'NONE', ( #8091 ), #13779, .F. ) ;
#12925=CARTESIAN_POINT ( 'NONE',  ( 17.43816562714825125, 15.15720016074785903, -232.3748236813696906 ) ) ;
#12927=CARTESIAN_POINT ( 'NONE',  ( 22.78751929883380356, -1.647884454956899836, -231.3901500139513416 ) ) ;
#12928=CARTESIAN_POINT ( 'NONE',  ( -18.75993824683981970, -9.028840681436806292, -217.1556094966459227 ) ) ;
#12931=CARTESIAN_POINT ( 'NONE',  ( -1.268862717067444024, 15.25222216985846480, -229.0661283592426116 ) ) ;
#12932=CARTESIAN_POINT ( 'NONE',  ( 28.41126862162173694, -7.739794849403359933, -232.1728475156252500 ) ) ;
#12933=CARTESIAN_POINT ( 'NONE',  ( 19.06212547406409641, -9.287000003594721775, -232.7453815625877667 ) ) ;
#12934=CARTESIAN_POINT ( 'NONE',  ( -24.18895665211001500, 11.26087434487096139, -231.0040666710689550 ) ) ;
#12935=CARTESIAN_POINT ( 'NONE',  ( 11.96568375430165254, 8.504117401580989721, -219.8633768076029753 ) ) ;
#12936=CARTESIAN_POINT ( 'NONE',  ( 13.55451907249704213, 16.71566520821242818, -219.1474322952048226 ) ) ;
#12938=CARTESIAN_POINT ( 'NONE',  ( 1.038689920556553847, -18.98022482494055652, -217.9213632692622866 ) ) ;
#12940=CARTESIAN_POINT ( 'NONE',  ( 4.719925043692215993, 22.16918918211828782, -214.6883144083888908 ) ) ;
#12941=CARTESIAN_POINT ( 'NONE',  ( -4.154119475380428916, 11.54776298361823095, -227.0876712548254943 ) ) ;
#12942=CARTESIAN_POINT ( 'NONE',  ( 20.08508968036338871, -9.819972662663129626, -218.2881406113160381 ) ) ;
#12943=CARTESIAN_POINT ( 'NONE',  ( -2.808235066048971440, 30.42019778760651150, -222.6481917607299295 ) ) ;
#12946=CARTESIAN_POINT ( 'NONE',  ( -3.712761995161701911, 23.50704853188985766, -216.1220552374512067 ) ) ;
#12947=CARTESIAN_POINT ( 'NONE',  ( -17.59913672443795463, -0.5356773789333074687, -220.7342471185320960 ) ) ;
#12949=CARTESIAN_POINT ( 'NONE',  ( -9.250876228778270871, 9.538614635316015722, -227.1332118982684563 ) ) ;
#12950=CARTESIAN_POINT ( 'NONE',  ( 14.85123888640019452, 5.067529763532427012, -221.9058491819374979 ) ) ;
#12951=CARTESIAN_POINT ( 'NONE',  ( -5.589224416770360193, 14.13652937339764115, -225.1481999119820330 ) ) ;
#12953=CARTESIAN_POINT ( 'NONE',  ( 2.085064686336211892, 14.99578618537741548, -226.0985834012817861 ) ) ;
#12954=CARTESIAN_POINT ( 'NONE',  ( -25.10035252441274167, -15.33546242866430198, -228.3913311683031964 ) ) ;
#12955=CARTESIAN_POINT ( 'NONE',  ( 14.22574309452842733, 4.476723532073429546, -225.5862451792618231 ) ) ;
#12956=CARTESIAN_POINT ( 'NONE',  ( -5.646690751453034451, -19.25001164140187981, -233.5706237494638913 ) ) ;
#12959=CARTESIAN_POINT ( 'NONE',  ( -17.99720854823001659, 13.97888873227035056, -232.2992184661552244 ) ) ;
#12960=CARTESIAN_POINT ( 'NONE',  ( 19.78534257568999166, -22.00365353819481840, -227.2618024355658974 ) ) ;
#12961=CARTESIAN_POINT ( 'NONE',  ( 6.295505112925526170, 15.36201163567862693, -221.5772643759389098 ) ) ;
#12962=CARTESIAN_POINT ( 'NONE',  ( -9.988594796049140356, 11.34066464990972811, -226.6453149279956563 ) ) ;
#12963=CARTESIAN_POINT ( 'NONE',  ( -14.74212732455322161, 0.2624230007780231633, -231.8143822214177874 ) ) ;
#12964=CARTESIAN_POINT ( 'NONE',  ( -17.58891219272264905, -6.833323493373833379, -229.9407564095759540 ) ) ;
#12965=CARTESIAN_POINT ( 'NONE',  ( 13.49694890958685711, 2.186465430673721677, -228.8273158381700512 ) ) ;
#12967=CARTESIAN_POINT ( 'NONE',  ( -14.64285150619984677, -17.93374633926643824, -235.3168067477300838 ) ) ;
#12968=CARTESIAN_POINT ( 'NONE',  ( 0.1556102272723409452, 19.71550568250159685, -232.1993058477363547 ) ) ;
#12969=CARTESIAN_POINT ( 'NONE',  ( 13.10956039622986324, 4.581323766968698585, -221.0328522389722252 ) ) ;
#12970=CARTESIAN_POINT ( 'NONE',  ( -16.45414350258782221, 17.57852913985137988, -231.3969631806205598 ) ) ;
#12971=CARTESIAN_POINT ( 'NONE',  ( 18.69149182921226782, 24.00661454656289706, -229.8257469855424517 ) ) ;
#12972=CARTESIAN_POINT ( 'NONE',  ( 3.608972370552595343, -15.05750810295313435, -224.7555151483228713 ) ) ;
#12973=CARTESIAN_POINT ( 'NONE',  ( -2.609511328024065602, -16.97143768612226822, -230.2205646068415490 ) ) ;
#12974=CARTESIAN_POINT ( 'NONE',  ( 28.57344184061583192, 5.631897254180425527, -225.1192013637692355 ) ) ;
#12975=CARTESIAN_POINT ( 'NONE',  ( 22.44368505003003378, -11.72633196808685163, -232.1179326287041533 ) ) ;
#12976=CARTESIAN_POINT ( 'NONE',  ( -28.18501077041064562, -8.523171531337160545, -227.0531053546762337 ) ) ;
#12977=CARTESIAN_POINT ( 'NONE',  ( -11.88525712185471050, -8.925198460467992589, -221.0951487055306472 ) ) ;
#12978=CARTESIAN_POINT ( 'NONE',  ( 15.28499842775873319, 22.98894588155567931, -221.0942409093412095 ) ) ;
#12980=CARTESIAN_POINT ( 'NONE',  ( -17.18633058961025029, 6.481319267413964802, -216.1357216783315494 ) ) ;
#12981=CARTESIAN_POINT ( 'NONE',  ( -3.855805549595750392, 26.68244055262801950, -232.4569730455296508 ) ) ;
#12982=CARTESIAN_POINT ( 'NONE',  ( -2.532302712337851425, 16.54370602006230939, -228.1940632970506613 ) ) ;
#12983=CARTESIAN_POINT ( 'NONE',  ( 21.68440970896747544, -13.87065835575754846, -215.6285083892243790 ) ) ;
#12984=CARTESIAN_POINT ( 'NONE',  ( 21.38922145650625239, 17.10616209967719215, -217.8354246241890451 ) ) ;
#12985=CARTESIAN_POINT ( 'NONE',  ( -19.72392517715239535, 13.50888179936880107, -230.7714862421596251 ) ) ;
#12986=CARTESIAN_POINT ( 'NONE',  ( -15.10945752141584464, 6.470132813599071220, -220.1568141593501764 ) ) ;
#12987=CARTESIAN_POINT ( 'NONE',  ( -1.827935560680505445, -14.81092009092713369, -225.7372845858837707 ) ) ;
#12990=CARTESIAN_POINT ( 'NONE',  ( 19.19288224840068935, 10.13059690604263174, -232.1906135022504998 ) ) ;
#12991=CARTESIAN_POINT ( 'NONE',  ( 16.16137015560671131, -6.751010448487875237, -221.3181884246570519 ) ) ;
#12992=CARTESIAN_POINT ( 'NONE',  ( -21.43408368508570305, 3.680162304907783621, -233.1134812316964542 ) ) ;
#12994=CARTESIAN_POINT ( 'NONE',  ( -14.34280792637948743, -22.10828917559366147, -217.4172704053049756 ) ) ;
#12997=CARTESIAN_POINT ( 'NONE',  ( 3.763426558366607111, 28.60172112197566818, -230.1816715025297526 ) ) ;
#12999=CARTESIAN_POINT ( 'NONE',  ( -5.568057711815838751, 28.69723585065299076, -232.1518503103610271 ) ) ;
#13001=CARTESIAN_POINT ( 'NONE',  ( -7.913358619554302642, 16.16796202616373890, -233.0981776325470491 ) ) ;
#13002=CARTESIAN_POINT ( 'NONE',  ( -13.63272521699743756, -3.226083955879493814, -228.1383267723209656 ) ) ;
#13005=CARTESIAN_POINT ( 'NONE',  ( -6.571166997218196748, 12.74865329367398736, -229.9840124400968762 ) ) ;
#13006=CARTESIAN_POINT ( 'NONE',  ( -7.625346832407194242, -11.41809035428902064, -218.7189489878062716 ) ) ;
#13007=CARTESIAN_POINT ( 'NONE',  ( 13.62757736989142465, -5.584028114184929947, -227.2616851496390211 ) ) ;
#13008=CARTESIAN_POINT ( 'NONE',  ( -14.07917727715460821, 7.534853284453274291, -218.6337090155677458 ) ) ;
#13010=CARTESIAN_POINT ( 'NONE',  ( -14.83095329101371540, 1.580869236763225549, -217.8331819987577660 ) ) ;
#13012=CARTESIAN_POINT ( 'NONE',  ( 2.601379523478754674, 17.36677895276155681, -230.4357129074444117 ) ) ;
#13014=CARTESIAN_POINT ( 'NONE',  ( 15.58465056415575312, 2.812367138262562349, -229.5090343034091234 ) ) ;
#13015=CARTESIAN_POINT ( 'NONE',  ( -7.719684133369767665, -19.28933804209621528, -218.9187502689394478 ) ) ;
#13017=CARTESIAN_POINT ( 'NONE',  ( -12.05423124486310904, 12.38527783110887803, -219.7419643105747014 ) ) ;
#13018=CARTESIAN_POINT ( 'NONE',  ( 11.43247012502872728, 12.44034019618676190, -231.9336559008378629 ) ) ;
#13019=CARTESIAN_POINT ( 'NONE',  ( 5.030854775705693172, 19.94152319263364603, -234.9034581965229336 ) ) ;
#13021=CARTESIAN_POINT ( 'NONE',  ( 30.05917755080113096, -2.930701380670650114, -221.3976229872638726 ) ) ;
#13024=CARTESIAN_POINT ( 'NONE',  ( -11.98736441306973077, 11.45674391201457176, -217.8252237716743025 ) ) ;
#13025=CARTESIAN_POINT ( 'NONE',  ( -16.91104737563547644, -22.20641354538343748, -232.3619262256263482 ) ) ;
#13026=CARTESIAN_POINT ( 'NONE',  ( 28.02123297569005089, 5.903198806000402143, -227.5759114383273811 ) ) ;
#13027=CARTESIAN_POINT ( 'NONE',  ( 9.107417252317809186, 16.30291009569977234, -218.0131178633739921 ) ) ;
#13028=CARTESIAN_POINT ( 'NONE',  ( 14.87721638700776694, -2.584478279266595013, -226.5265678059390666 ) ) ;
#13029=UNCERTAINTY_MEASURE_WITH_UNIT (LENGTH_MEASURE( 1.000000000000000082E-05 ), #16011, 'distance_accuracy_value', 'NONE');
#13030=CARTESIAN_POINT ( 'NONE',  ( -21.93223149637851677, 1.726402211042445067, -231.1052103444381203 ) ) ;
#13031=CARTESIAN_POINT ( 'NONE',  ( 21.92281339924938877, 16.67475415235398017, -231.9828670874568957 ) ) ;
#13032=( NAMED_UNIT ( * ) PLANE_ANGLE_UNIT ( ) SI_UNIT ( $, .RADIAN. ) );
#13035=CARTESIAN_POINT ( 'NONE',  ( 18.04365516558436866, 6.721233635139160612, -218.4376093631473168 ) ) ;
#13036=CARTESIAN_POINT ( 'NONE',  ( 18.57039993684838564, -7.499893981036622748, -219.4816775992414080 ) ) ;
#13037=CARTESIAN_POINT ( 'NONE',  ( -11.36971918743327237, -8.287084598727400220, -223.1364763414170227 ) ) ;
#13041=CARTESIAN_POINT ( 'NONE',  ( -2.117958212721558375, 27.20243410318316535, -230.7086725634165418 ) ) ;
#13042=CARTESIAN_POINT ( 'NONE',  ( 31.06375291838557118, -1.327124779900562768, -220.7315133954257647 ) ) ;
#13043=CARTESIAN_POINT ( 'NONE',  ( 25.69672030403964769, -15.30292110028031338, -224.0206579222720791 ) ) ;
#13044=CARTESIAN_POINT ( 'NONE',  ( -12.82737030338386219, 8.595865151885988098, -221.6735325378515142 ) ) ;
#13045=CARTESIAN_POINT ( 'NONE',  ( 12.25122766587143630, 4.035812653434439845, -225.7709573147497224 ) ) ;
#13046=CARTESIAN_POINT ( 'NONE',  ( 12.00334754111224100, 12.62951371569041115, -228.5814949098771649 ) ) ;
#13048=CARTESIAN_POINT ( 'NONE',  ( 3.610394173775429039, -14.27701378914486874, -220.9234757326916281 ) ) ;
#13051=CARTESIAN_POINT ( 'NONE',  ( -28.76901170826145560, 13.32870333992657663, -228.6722616467874616 ) ) ;
#13054=CARTESIAN_POINT ( 'NONE',  ( -12.98662328632235585, 28.83726371277012035, -223.5970274767108776 ) ) ;
#13055=CARTESIAN_POINT ( 'NONE',  ( 5.501756899793208255, 15.97909684020861043, -233.9380718515096191 ) ) ;
#13056=CARTESIAN_POINT ( 'NONE',  ( 14.02135871364020936, -4.809710560857269002, -224.5109434094503911 ) ) ;
#13057=CARTESIAN_POINT ( 'NONE',  ( -11.33137429837660193, 27.25022425932026238, -230.1650924901870212 ) ) ;
#13059=CARTESIAN_POINT ( 'NONE',  ( 2.276720224425493821, 13.44951395023989171, -229.9230017221896105 ) ) ;
#13060=CARTESIAN_POINT ( 'NONE',  ( 26.56239871811266440, 9.439457669498057868, -217.7226690415261885 ) ) ;
#13061=CARTESIAN_POINT ( 'NONE',  ( -11.98736441306973077, 11.45674391201457176, -217.8252237716743025 ) ) ;
#13062=CARTESIAN_POINT ( 'NONE',  ( 24.58316096239279602, 5.861425670879941485, -231.3104446318280623 ) ) ;
#13064=CARTESIAN_POINT ( 'NONE',  ( 6.173705828530630768, 14.85108299334794957, -222.6284669816953112 ) ) ;
#13067=CARTESIAN_POINT ( 'NONE',  ( 16.01130065545721592, 20.79417322911648114, -220.9619135886794652 ) ) ;
#13068=CARTESIAN_POINT ( 'NONE',  ( -25.82802808205240552, -14.78441951539553401, -222.6940535085979604 ) ) ;
#13069=CARTESIAN_POINT ( 'NONE',  ( 13.69275646168278371, 8.674223198772375909, -220.8699857572541987 ) ) ;
#13070=CARTESIAN_POINT ( 'NONE',  ( -3.168869516962652622, -26.26615012824360207, -217.0152745877844040 ) ) ;
#13073=CARTESIAN_POINT ( 'NONE',  ( -7.250603130619442283, 20.89725557392719324, -217.7893896917081520 ) ) ;
#13074=CARTESIAN_POINT ( 'NONE',  ( 24.14841045621385263, -15.62485098017456586, -229.9279278555176518 ) ) ;
#13075=CARTESIAN_POINT ( 'NONE',  ( 25.85827166240959940, 13.84420748389600675, -220.2831452073696425 ) ) ;
#13076=CARTESIAN_POINT ( 'NONE',  ( -12.82737030338386219, 8.595865151885988098, -221.6735325378515142 ) ) ;
#13077=CARTESIAN_POINT ( 'NONE',  ( -16.95112677453439431, 10.32962960657076934, -214.9445123409346650 ) ) ;
#13078=CARTESIAN_POINT ( 'NONE',  ( -24.64494147011371084, -8.645298684267959999, -229.1812397229770113 ) ) ;
#13079=CARTESIAN_POINT ( 'NONE',  ( 22.92330650806121639, 19.11387742755395180, -231.6463539987045976 ) ) ;
#13082=CARTESIAN_POINT ( 'NONE',  ( -19.82723516873631908, -6.367811336401608457, -234.7370909334860869 ) ) ;
#13083=CARTESIAN_POINT ( 'NONE',  ( 1.939863782649466017, 28.20584428268631783, -229.4487744520996273 ) ) ;
#13084=CARTESIAN_POINT ( 'NONE',  ( 27.69955354773053458, 12.81264626165819287, -221.7750850138309602 ) ) ;
#13085=CARTESIAN_POINT ( 'NONE',  ( -11.83954511762131112, 10.58068896997146346, -226.6171226499791089 ) ) ;
#13086=CARTESIAN_POINT ( 'NONE',  ( 3.714886539878811789, 12.88803176524806560, -219.5889136906770034 ) ) ;
#13088=CARTESIAN_POINT ( 'NONE',  ( 0.7938325546108213615, -23.90362011959725663, -218.0438616059182380 ) ) ;
#13089=CARTESIAN_POINT ( 'NONE',  ( 1.874647746501092893, -15.20125101474619633, -222.7462710229423521 ) ) ;
#13090=CARTESIAN_POINT ( 'NONE',  ( -12.36382104905844592, -0.1264132474004772688, -228.0034406263598896 ) ) ;
#13091=CARTESIAN_POINT ( 'NONE',  ( 24.80560757033128993, -15.22139526172250079, -221.3338856610240271 ) ) ;
#13092=CARTESIAN_POINT ( 'NONE',  ( -25.95884575339096401, -1.972114683626720044, -231.2145524501483749 ) ) ;
#13093=CARTESIAN_POINT ( 'NONE',  ( -12.42894476027428929, -17.97759322220185396, -216.3110355466728834 ) ) ;
#13094=CARTESIAN_POINT ( 'NONE',  ( 3.182992543297812560, 16.68308636702302650, -221.9272281984358415 ) ) ;
#13096=CARTESIAN_POINT ( 'NONE',  ( -30.35034897870229287, 7.696526532841741819, -221.5749790623549416 ) ) ;
#13098=CARTESIAN_POINT ( 'NONE',  ( 8.979547488457603421, 23.24376652602565230, -232.6628827740196357 ) ) ;
#13099=CARTESIAN_POINT ( 'NONE',  ( 7.804112641607792611, 19.76858558208418515, -218.6463059509973164 ) ) ;
#13100=CARTESIAN_POINT ( 'NONE',  ( 9.734612854996214537, -6.789898087979761243, -225.0934417779699004 ) ) ;
#13101=CARTESIAN_POINT ( 'NONE',  ( 17.31940731551425827, 24.90170669671083914, -222.9868986272316533 ) ) ;
#13102=CARTESIAN_POINT ( 'NONE',  ( -11.82020046940938407, 10.16362659047642758, -224.3364193436540575 ) ) ;
#13103=CARTESIAN_POINT ( 'NONE',  ( -16.29666348338687953, 2.994680995215331709, -221.2421885839926006 ) ) ;
#13104=CARTESIAN_POINT ( 'NONE',  ( 4.002939343642331949, -22.37368820207002429, -217.8631878264377804 ) ) ;
#13107=CARTESIAN_POINT ( 'NONE',  ( 18.76922974182421555, 13.12635134380198210, -217.8010375391909008 ) ) ;
#13108=CARTESIAN_POINT ( 'NONE',  ( 10.54788747927062964, -11.30141756528536412, -223.8337882627521651 ) ) ;
#13109=CARTESIAN_POINT ( 'NONE',  ( -14.07336028695978314, 1.752429266630609828, -222.9750305084206161 ) ) ;
#13111=CARTESIAN_POINT ( 'NONE',  ( -8.491902988188710921, -10.37035003683405066, -223.9502466269643435 ) ) ;
#13113=CARTESIAN_POINT ( 'NONE',  ( 4.343013938751969505, 13.02036404005131587, -224.7825435359082178 ) ) ;
#13115=CARTESIAN_POINT ( 'NONE',  ( -5.467362224022371819, 23.92882567691090046, -234.7811165710531611 ) ) ;
#13117=CARTESIAN_POINT ( 'NONE',  ( -3.855805549595750392, 26.68244055262801950, -232.4569730455296508 ) ) ;
#13118=CARTESIAN_POINT ( 'NONE',  ( -14.84457943406284208, -4.054717634150219574, -219.4128920803699430 ) ) ;
#13121=CARTESIAN_POINT ( 'NONE',  ( -13.58874046263339608, 12.73011668665171392, -216.5659449791897941 ) ) ;
#13122=CARTESIAN_POINT ( 'NONE',  ( -13.27281469842883688, -16.60017218729922561, -235.3541344917538254 ) ) ;
#13123=CARTESIAN_POINT ( 'NONE',  ( 25.69672030403964769, -15.30292110028031338, -224.0206579222720791 ) ) ;
#13124=CARTESIAN_POINT ( 'NONE',  ( -3.205260335674071648, 17.52234722004434531, -232.9754319808710363 ) ) ;
#13125=CARTESIAN_POINT ( 'NONE',  ( -17.18633058961025029, 6.481319267413964802, -216.1357216783315494 ) ) ;
#13127=CARTESIAN_POINT ( 'NONE',  ( -1.470815287892122125, 29.54293232078718745, -224.5855911371830302 ) ) ;
#13129=CARTESIAN_POINT ( 'NONE',  ( 19.31922195716811430, 9.600631919686000160, -218.1359845693048101 ) ) ;
#13130=CARTESIAN_POINT ( 'NONE',  ( -8.126933673790581736, -26.89509779614531126, -227.4795931708183048 ) ) ;
#13132=CARTESIAN_POINT ( 'NONE',  ( -12.87285471141929172, 9.485162256560764504, -229.1865421006261840 ) ) ;
#13133=CARTESIAN_POINT ( 'NONE',  ( 20.26651059498356844, 18.95255124124090074, -231.7206897233655525 ) ) ;
#13134=CARTESIAN_POINT ( 'NONE',  ( 2.469769522101480597, 18.85781121334172639, -215.5372409425634430 ) ) ;
#13135=CARTESIAN_POINT ( 'NONE',  ( -20.79829908948044448, -4.820361304162784855, -232.2223801333801703 ) ) ;
#13136=EDGE_CURVE ( 'NONE', #2027, #7856, #13741, .T. ) ;
#13140=CARTESIAN_POINT ( 'NONE',  ( -12.44873260470819787, 7.411970124596155785, -229.4214091473984070 ) ) ;
#13141=CARTESIAN_POINT ( 'NONE',  ( -3.368184987477955694, -15.91886893360235078, -219.1066823976216256 ) ) ;
#13143=CARTESIAN_POINT ( 'NONE',  ( 11.13678936984666912, 26.95732789089726111, -228.8350761760834757 ) ) ;
#13145=CARTESIAN_POINT ( 'NONE',  ( -14.58084844870496966, 13.85720943031455832, -233.3219724312919254 ) ) ;
#13146=CARTESIAN_POINT ( 'NONE',  ( 23.64727379217503866, 9.907944788639682088, -232.0643337313508709 ) ) ;
#13148=CARTESIAN_POINT ( 'NONE',  ( 16.64225601860865211, 1.926018578292457928, -220.2177910260893725 ) ) ;
#13150=CARTESIAN_POINT ( 'NONE',  ( 25.46431111394153390, -2.048831322092446783, -230.3135391428295975 ) ) ;
#13151=CARTESIAN_POINT ( 'NONE',  ( -23.10791503177032880, -5.282985115830100220, -217.6364121950018671 ) ) ;
#13155=CARTESIAN_POINT ( 'NONE',  ( -14.00980274651940682, 20.05588230486321066, -234.2453272803952586 ) ) ;
#13156=CARTESIAN_POINT ( 'NONE',  ( 25.79180107113126397, -16.09695083256378112, -231.0225534820104656 ) ) ;
#13157=CARTESIAN_POINT ( 'NONE',  ( 24.80560757033128993, -15.22139526172250079, -221.3338856610240271 ) ) ;
#13158=CARTESIAN_POINT ( 'NONE',  ( -25.19248792833826300, 13.40115236862232528, -221.2817950683888455 ) ) ;
#13159=CARTESIAN_POINT ( 'NONE',  ( -19.67797246974518544, 1.229961341702398681, -219.4743747885323160 ) ) ;
#13160=CARTESIAN_POINT ( 'NONE',  ( 12.91443243054181700, 13.28840485332751875, -229.6651346406987955 ) ) ;
#13162=CARTESIAN_POINT ( 'NONE',  ( -0.6720842648862578317, -17.90033647106004011, -231.4757128331908973 ) ) ;
#13164=CARTESIAN_POINT ( 'NONE',  ( -15.57331739480619248, 4.297375044201914740, -216.4079605712025511 ) ) ;
#13165=CARTESIAN_POINT ( 'NONE',  ( 12.65306858828212810, 29.42930486385247590, -226.3758484992818012 ) ) ;
#13166=CARTESIAN_POINT ( 'NONE',  ( 1.920320557106582893, 25.99317453242502296, -234.5637964893073217 ) ) ;
#13167=CARTESIAN_POINT ( 'NONE',  ( 14.09645999499448088, -9.025099991742237648, -228.8994629750086744 ) ) ;
#13168=CARTESIAN_POINT ( 'NONE',  ( -12.74846050492543625, 19.93509882904884734, -216.0172840992881049 ) ) ;
#13169=CARTESIAN_POINT ( 'NONE',  ( -29.95012366401462955, 4.746560250930182967, -224.6954343660969471 ) ) ;
#13171=CARTESIAN_POINT ( 'NONE',  ( 15.89102655998366664, 24.10108298038447572, -232.7733025413564008 ) ) ;
#13172=CARTESIAN_POINT ( 'NONE',  ( -17.65933056022148762, 0.7424667221540405260, -229.0964312085266386 ) ) ;
#13173=CARTESIAN_POINT ( 'NONE',  ( -21.02719846458807851, 18.12262440796364871, -218.0220709499931502 ) ) ;
#13174=CARTESIAN_POINT ( 'NONE',  ( 18.46552355142154411, 5.019711608606525211, -231.5099115070375433 ) ) ;
#13176=CARTESIAN_POINT ( 'NONE',  ( 7.017641603801325623, 14.96204511409594673, -228.1064041248110073 ) ) ;
#13180=CARTESIAN_POINT ( 'NONE',  ( 8.961491954973460849, 17.27041174997091844, -219.7661252763212474 ) ) ;
#13181=CARTESIAN_POINT ( 'NONE',  ( -17.42499862437977853, -18.98713029041037004, -232.7811807006768845 ) ) ;
#13182=CARTESIAN_POINT ( 'NONE',  ( 26.48990917286906921, 12.16675355942207659, -225.0153622588060216 ) ) ;
#13183=CARTESIAN_POINT ( 'NONE',  ( -9.481788909210624894, -22.96916533494018253, -217.3969400264330716 ) ) ;
#13185=CARTESIAN_POINT ( 'NONE',  ( -16.50467377682197423, 21.56569464670658220, -229.9175202103629374 ) ) ;
#13186=CARTESIAN_POINT ( 'NONE',  ( 11.97732832373273126, -6.576952149368169742, -223.6031523087739572 ) ) ;
#13187=CARTESIAN_POINT ( 'NONE',  ( 12.23475091788960434, 6.342242864926500800, -221.9572581868331156 ) ) ;
#13188=CARTESIAN_POINT ( 'NONE',  ( -9.233762381136051189, 19.18161952504991419, -232.0796851897838451 ) ) ;
#13189=CARTESIAN_POINT ( 'NONE',  ( -13.06407726305387307, 3.888674610242962348, -219.0371145420960204 ) ) ;
#13190=CARTESIAN_POINT ( 'NONE',  ( -19.94082127283490280, -7.534429669270808816, -230.8553971038493557 ) ) ;
#13191=CARTESIAN_POINT ( 'NONE',  ( 21.06229272850552547, 3.434461253538921621, -234.1452885155528918 ) ) ;
#13193=CARTESIAN_POINT ( 'NONE',  ( -16.32911940539174367, -0.4850290419235887551, -232.0399150213553412 ) ) ;
#13194=CARTESIAN_POINT ( 'NONE',  ( 14.69879291197755222, 10.86005690695417236, -216.7815908316746913 ) ) ;
#13195=CARTESIAN_POINT ( 'NONE',  ( 17.22423229049764970, 1.395540479540137380, -217.3898520248025363 ) ) ;
#13196=CARTESIAN_POINT ( 'NONE',  ( -1.585416880194127520, 15.28258783379090424, -231.0852564988603319 ) ) ;
#13197=CARTESIAN_POINT ( 'NONE',  ( 9.533850545951205291, 16.09136358716069637, -215.9093469876620475 ) ) ;
#13198=CARTESIAN_POINT ( 'NONE',  ( 3.191506000329551007, -19.56356538597602679, -231.2193641236077326 ) ) ;
#13201=CARTESIAN_POINT ( 'NONE',  ( -5.322766963623397629, -16.65786661440869665, -219.3972027188067671 ) ) ;
#13202=CARTESIAN_POINT ( 'NONE',  ( -12.13319425917249283, 4.024026700415168634, -229.5243363405849095 ) ) ;
#13203=CARTESIAN_POINT ( 'NONE',  ( 15.05686526350529775, -5.555778903407086133, -220.1433349335996468 ) ) ;
#13204=CARTESIAN_POINT ( 'NONE',  ( -14.37894460687751597, -1.926260335694933268, -225.0161641904981593 ) ) ;
#13205=CARTESIAN_POINT ( 'NONE',  ( -12.13177435108894642, -8.392035797555511323, -228.8392847287196332 ) ) ;
#13206=CARTESIAN_POINT ( 'NONE',  ( 21.24820809707834357, 20.59746639607275398, -225.8540969741923732 ) ) ;
#13208=CARTESIAN_POINT ( 'NONE',  ( -15.33438615632468149, 23.56248205204123991, -229.2747191038674544 ) ) ;
#13209=CARTESIAN_POINT ( 'NONE',  ( 25.85827166240959940, 13.84420748389600675, -220.2831452073696425 ) ) ;
#13210=CARTESIAN_POINT ( 'NONE',  ( 11.33210854356620523, 22.81476816607802149, -217.8536224460118262 ) ) ;
#13211=CARTESIAN_POINT ( 'NONE',  ( 17.98704291748025952, 16.14142602298251461, -217.3684083235702644 ) ) ;
#13212=CARTESIAN_POINT ( 'NONE',  ( 10.30964016151751750, -15.48526446506176413, -234.8200832677974859 ) ) ;
#13213=CARTESIAN_POINT ( 'NONE',  ( 13.86383614057800884, 4.939477956453596441, -219.6543243356308324 ) ) ;
#13214=CARTESIAN_POINT ( 'NONE',  ( -8.900302563431933933, 20.17395648083808268, -216.9116515890487733 ) ) ;
#13215=CARTESIAN_POINT ( 'NONE',  ( -10.03082531488024109, -22.09229706162428286, -231.9736132431984572 ) ) ;
#13216=CARTESIAN_POINT ( 'NONE',  ( -16.74550766701807447, 3.787526820511904813, -217.9802846976114381 ) ) ;
#13218=CARTESIAN_POINT ( 'NONE',  ( 21.39553407250273054, 8.453402029343234148, -217.9531594780983141 ) ) ;
#13219=CARTESIAN_POINT ( 'NONE',  ( 15.01754996320599744, -10.17932250226635738, -220.3401326760229040 ) ) ;
#13220=CARTESIAN_POINT ( 'NONE',  ( -13.96147744945181124, 5.260363697127891314, -222.3342733685200301 ) ) ;
#13221=CARTESIAN_POINT ( 'NONE',  ( -7.800954605602409053, -29.95157606033723496, -226.5906573908930000 ) ) ;
#13222=CARTESIAN_POINT ( 'NONE',  ( -18.94009481283715957, 3.115208415279245191, -230.3622730452590588 ) ) ;
#13223=CARTESIAN_POINT ( 'NONE',  ( 1.557078628722260438, 24.20011951319323273, -235.1441088220640268 ) ) ;
#13224=ORIENTED_EDGE ( 'NONE', *, *, #4161, .F. ) ;
#13225=CARTESIAN_POINT ( 'NONE',  ( -8.501641725227710111, 25.47064987787527102, -217.3358698761548737 ) ) ;
#13226=CARTESIAN_POINT ( 'NONE',  ( -17.83852468596024110, -8.357198216422425219, -233.0481596892792879 ) ) ;
#13227=CARTESIAN_POINT ( 'NONE',  ( 30.87761267810551757, -2.376991648450896388, -225.4116222034606949 ) ) ;
#13229=CARTESIAN_POINT ( 'NONE',  ( 5.623554730548537606, 15.65270319720736225, -231.3185741195121068 ) ) ;
#13230=CARTESIAN_POINT ( 'NONE',  ( -7.108809775916832940, -10.55228017211132929, -220.3225562754048212 ) ) ;
#13231=CARTESIAN_POINT ( 'NONE',  ( 10.30328786010431052, -20.08430705480546408, -216.1847100135515802 ) ) ;
#13232=CARTESIAN_POINT ( 'NONE',  ( 13.96958060839473958, -9.488587112651741151, -218.7731372952745232 ) ) ;
#13233=CARTESIAN_POINT ( 'NONE',  ( -8.221702953833418093, 11.87876791566348800, -223.9138461338794741 ) ) ;
#13234=CARTESIAN_POINT ( 'NONE',  ( 11.27486163995310164, 25.12851252939060487, -222.6718455410222930 ) ) ;
#13235=CARTESIAN_POINT ( 'NONE',  ( -28.99926036811508467, 3.909990568804979194, -228.9613767892386988 ) ) ;
#13236=CARTESIAN_POINT ( 'NONE',  ( -12.89119823113977503, 10.10140484475961564, -218.5945808114896636 ) ) ;
#13237=CARTESIAN_POINT ( 'NONE',  ( -26.75342641616541783, -10.60804028525731546, -225.2137697103424898 ) ) ;
#13239=CARTESIAN_POINT ( 'NONE',  ( -22.24722865165759345, 18.77558306771206986, -226.5077042908023941 ) ) ;
#13240=CARTESIAN_POINT ( 'NONE',  ( 21.52074627118099315, 8.791036694007010155, -215.9547738671300294 ) ) ;
#13241=CARTESIAN_POINT ( 'NONE',  ( 1.898427734299754421, 12.47096978853034521, -227.5043976727869506 ) ) ;
#13243=CARTESIAN_POINT ( 'NONE',  ( -26.24201160508392761, -9.884581200937399004, -221.6903139798603206 ) ) ;
#13245=CARTESIAN_POINT ( 'NONE',  ( -17.65835845419170624, 22.55329142274348442, -231.2673511165784532 ) ) ;
#13246=CARTESIAN_POINT ( 'NONE',  ( -4.782174899302804150, -29.09898918907212817, -227.3916599557566940 ) ) ;
#13247=CARTESIAN_POINT ( 'NONE',  ( 28.57344184061583192, 5.631897254180425527, -225.1192013637692355 ) ) ;
#13248=CARTESIAN_POINT ( 'NONE',  ( 8.979547488457603421, 23.24376652602565230, -232.6628827740196357 ) ) ;
#13251=CARTESIAN_POINT ( 'NONE',  ( -11.94727018630768178, 9.025563988971828877, -220.6148682757971358 ) ) ;
#13252=CARTESIAN_POINT ( 'NONE',  ( 22.37138132874926910, 6.723028048925958622, -217.7073806909121743 ) ) ;
#13254=CARTESIAN_POINT ( 'NONE',  ( 15.54590875671327233, 1.102094689760376056, -222.2065310083714849 ) ) ;
#13255=CARTESIAN_POINT ( 'NONE',  ( 18.60971343765040942, 2.368090295052050820, -218.6871071987073094 ) ) ;
#13258=CARTESIAN_POINT ( 'NONE',  ( 16.24842259479558848, -3.494976385286828080, -222.6392560871376816 ) ) ;
#13259=CARTESIAN_POINT ( 'NONE',  ( -17.58118739749173898, -8.238107657346720458, -217.5252134542318458 ) ) ;
#13262=CARTESIAN_POINT ( 'NONE',  ( 8.858651440950676914, 22.47383302477780376, -230.7859943773311215 ) ) ;
#13263=CARTESIAN_POINT ( 'NONE',  ( 13.44856294975069488, -28.16358066815265460, -226.3235907536142406 ) ) ;
#13264=CARTESIAN_POINT ( 'NONE',  ( 13.91151814069282722, -15.58123622716646572, -216.5183035683795367 ) ) ;
#13265=CARTESIAN_POINT ( 'NONE',  ( -11.94782396647286049, 8.456988817430419303, -225.5094493096559063 ) ) ;
#13266=CARTESIAN_POINT ( 'NONE',  ( 21.52074627118099315, 8.791036694007010155, -215.9547738671300294 ) ) ;
#13267=CARTESIAN_POINT ( 'NONE',  ( 25.53003411612920459, 7.940385729200389875, -230.5495695598654322 ) ) ;
#13269=CARTESIAN_POINT ( 'NONE',  ( 13.50228739682142454, -27.74890714798514679, -227.9743917065363519 ) ) ;
#13271=CARTESIAN_POINT ( 'NONE',  ( -16.81617677814535128, 0.6259372974186930838, -233.5115673467681745 ) ) ;
#13272=CARTESIAN_POINT ( 'NONE',  ( 10.81638188557560731, 14.98959006186633403, -234.2424515599453514 ) ) ;
#13273=CARTESIAN_POINT ( 'NONE',  ( 3.490345297502855715, 11.17751288514984331, -224.7799703251421022 ) ) ;
#13274=CARTESIAN_POINT ( 'NONE',  ( 23.21483485987735307, -16.21330837850192097, -225.6840547952056397 ) ) ;
#13275=CARTESIAN_POINT ( 'NONE',  ( -6.282398543089500187, 12.01615879894893801, -228.5121145169883903 ) ) ;
#13276=CARTESIAN_POINT ( 'NONE',  ( -13.10651848559790444, 3.262242204071156948, -224.3513854875720597 ) ) ;
#13278=CARTESIAN_POINT ( 'NONE',  ( 14.82579616070250417, 22.96152595385638762, -233.8920860146931489 ) ) ;
#13279=CARTESIAN_POINT ( 'NONE',  ( -19.92987771446595957, 11.92619342620000999, -232.5382020162021206 ) ) ;
#13280=CARTESIAN_POINT ( 'NONE',  ( -2.934221234790329369, 15.07857928364152222, -230.9558365497803720 ) ) ;
#13281=CARTESIAN_POINT ( 'NONE',  ( 16.84848658399567611, 11.39632653812981644, -217.9589513831453473 ) ) ;
#13282=CARTESIAN_POINT ( 'NONE',  ( 6.295505112925526170, 15.36201163567862693, -221.5772643759389098 ) ) ;
#13283=CARTESIAN_POINT ( 'NONE',  ( 26.54225689383817866, -6.924125931238839016, -230.1506921200174247 ) ) ;
#13285=CARTESIAN_POINT ( 'NONE',  ( -29.22168435891936156, -1.352755938724206519, -225.9547066689444250 ) ) ;
#13286=CARTESIAN_POINT ( 'NONE',  ( 19.19288224840068935, 10.13059690604263174, -232.1906135022504998 ) ) ;
#13287=CARTESIAN_POINT ( 'NONE',  ( -3.878264816061211651, -12.95777722686681344, -227.3767537598947683 ) ) ;
#13289=CARTESIAN_POINT ( 'NONE',  ( -10.84440549681320221, 27.00404139634608214, -224.0969657459751261 ) ) ;
#13291=CARTESIAN_POINT ( 'NONE',  ( 13.20312407767240614, -7.650902547765872086, -230.0578600405493717 ) ) ;
#13292=CARTESIAN_POINT ( 'NONE',  ( 15.74259730902452858, 17.40808440793174583, -232.1327802909178786 ) ) ;
#13293=CARTESIAN_POINT ( 'NONE',  ( -4.067324790461362305, 15.10342260507846746, -228.2464404076259257 ) ) ;
#13294=CARTESIAN_POINT ( 'NONE',  ( -7.099035520468861549, 19.73710792467281649, -233.8745459908100770 ) ) ;
#13296=CARTESIAN_POINT ( 'NONE',  ( -26.25663555152313222, -8.728475094464092976, -226.4697227271102236 ) ) ;
#13297=CARTESIAN_POINT ( 'NONE',  ( 20.64287812348744566, 0.2024751443801864337, -216.7518974727033481 ) ) ;
#13299=CARTESIAN_POINT ( 'NONE',  ( -25.32359575169976296, -0.6821277435459325300, -233.2512658769913969 ) ) ;
#13300=CARTESIAN_POINT ( 'NONE',  ( 6.771176146757415637, 15.60014285904435027, -218.3493856697694753 ) ) ;
#13301=CARTESIAN_POINT ( 'NONE',  ( -17.00819119081011266, 8.904695857470725784, -219.7915043529501133 ) ) ;
#13302=CARTESIAN_POINT ( 'NONE',  ( 10.86206282953156510, 30.27427353967719981, -226.0953027964478110 ) ) ;
#13303=CARTESIAN_POINT ( 'NONE',  ( 27.79670308438203108, 10.67628923451848877, -225.2981230784098727 ) ) ;
#13304=CARTESIAN_POINT ( 'NONE',  ( -2.927465716848487887, -13.57531311500885352, -224.4053031992201852 ) ) ;
#13306=CARTESIAN_POINT ( 'NONE',  ( -13.53581065110708970, -26.13331550560631555, -224.9773145811678887 ) ) ;
#13307=CARTESIAN_POINT ( 'NONE',  ( -13.56011990957801139, -0.3895158544032599202, -219.3211261236655218 ) ) ;
#13308=CARTESIAN_POINT ( 'NONE',  ( 13.99926435381047618, -21.11851526759364006, -232.9234173943665951 ) ) ;
#13309=CARTESIAN_POINT ( 'NONE',  ( 29.83024462204712179, 0.7507192471929857724, -227.4186229137179396 ) ) ;
#13310=CARTESIAN_POINT ( 'NONE',  ( -15.22366728182010043, -5.552021002219007961, -230.2511309519622671 ) ) ;
#13311=CARTESIAN_POINT ( 'NONE',  ( 18.75523091462765990, 19.46592657336209697, -230.4909883316157391 ) ) ;
#13314=CARTESIAN_POINT ( 'NONE',  ( -8.137644474477026435, 12.10064032984799098, -226.6735072060122036 ) ) ;
#13315=CARTESIAN_POINT ( 'NONE',  ( 8.812670488384366507, 12.21486833790445914, -225.9961634525829197 ) ) ;
#13316=CARTESIAN_POINT ( 'NONE',  ( -3.082945806077231676, 30.69897765966285874, -224.2387254578930822 ) ) ;
#13317=CARTESIAN_POINT ( 'NONE',  ( 7.067550969709256670, 17.75197616922148569, -219.3387126207321955 ) ) ;
#13318=CARTESIAN_POINT ( 'NONE',  ( 14.59690920037431638, -12.12875852167710988, -234.7370354398910877 ) ) ;
#13319=CARTESIAN_POINT ( 'NONE',  ( -11.07173923371951574, 9.938770595667456575, -229.9381419817434562 ) ) ;
#13320=CARTESIAN_POINT ( 'NONE',  ( -0.1452471002967452851, 24.29564289358754081, -234.0861481044164805 ) ) ;
#13321=CARTESIAN_POINT ( 'NONE',  ( -11.82217545354207644, -11.78227988727524966, -219.0934395369134506 ) ) ;
#13322=CARTESIAN_POINT ( 'NONE',  ( -14.68037037322036475, 3.441677802729143920, -220.1396515630443389 ) ) ;
#13324=CARTESIAN_POINT ( 'NONE',  ( 14.63113973005795643, 4.926264598692385199, -222.4866305912601945 ) ) ;
#13325=CARTESIAN_POINT ( 'NONE',  ( 12.33825063215758888, -15.78239559842968909, -231.3245247598261471 ) ) ;
#13326=CARTESIAN_POINT ( 'NONE',  ( -17.49393085256189906, 10.63366922396483361, -217.7502683347138657 ) ) ;
#13327=CARTESIAN_POINT ( 'NONE',  ( 2.785859284650920031, 14.19821255961969619, -226.9946081512528906 ) ) ;
#13328=CARTESIAN_POINT ( 'NONE',  ( -23.54665576872953636, -14.78900941482413067, -230.7594827126482073 ) ) ;
#13330=CARTESIAN_POINT ( 'NONE',  ( 16.21758812354607215, 4.665393561625732488, -232.5634757513959983 ) ) ;
#13331=CARTESIAN_POINT ( 'NONE',  ( 9.253342549662157523, 15.33540844142859605, -216.2601104504267937 ) ) ;
#13333=CARTESIAN_POINT ( 'NONE',  ( 5.017623471397871349, 29.83561274492976878, -222.9769172135417250 ) ) ;
#13334=CARTESIAN_POINT ( 'NONE',  ( 16.69326964758149856, -4.763004462669847783, -219.2590076381798951 ) ) ;
#13337=CARTESIAN_POINT ( 'NONE',  ( 4.730976410881341465, 17.65764351829336931, -217.6025626048331674 ) ) ;
#13338=CARTESIAN_POINT ( 'NONE',  ( -4.051702682916754839, -14.52120462818199798, -217.8402208339018671 ) ) ;
#13339=CARTESIAN_POINT ( 'NONE',  ( 1.729916699924999746, -18.64927252049523432, -233.5000329212076906 ) ) ;
#13340=CARTESIAN_POINT ( 'NONE',  ( 17.95694455891925756, -3.510678534943489026, -231.2643001502910067 ) ) ;
#13341=CARTESIAN_POINT ( 'NONE',  ( -12.89119823113977503, 10.10140484475961564, -218.5945808114896636 ) ) ;
#13342=CARTESIAN_POINT ( 'NONE',  ( 10.79895562092076844, 12.01490073542734116, -225.7380208924852809 ) ) ;
#13344=CARTESIAN_POINT ( 'NONE',  ( -21.95649697515285581, 20.70968357470995258, -226.9638023349746447 ) ) ;
#13345=CARTESIAN_POINT ( 'NONE',  ( -15.02851318684991000, -5.270497739200964205, -221.5518599052197146 ) ) ;
#13347=CARTESIAN_POINT ( 'NONE',  ( -10.23029362138610843, 26.44342627367518617, -221.6879936327511871 ) ) ;
#13348=CARTESIAN_POINT ( 'NONE',  ( 27.79746884017060538, 13.63637251724950339, -226.5788410723774575 ) ) ;
#13349=CARTESIAN_POINT ( 'NONE',  ( 8.036750260989780514, 26.29729070384984624, -233.5018314387838529 ) ) ;
#13350=CARTESIAN_POINT ( 'NONE',  ( 12.90505172109588194, -11.18139282378177768, -218.7382941517081747 ) ) ;
#13353=CARTESIAN_POINT ( 'NONE',  ( -15.48255455842386219, 10.01793346089237069, -233.1197357361336913 ) ) ;
#13354=CARTESIAN_POINT ( 'NONE',  ( -11.58651333402397476, -12.19597367159924595, -216.5418320517508448 ) ) ;
#13355=CARTESIAN_POINT ( 'NONE',  ( 12.23063869552301242, 12.84118223717021934, -218.8273164334868284 ) ) ;
#13357=CARTESIAN_POINT ( 'NONE',  ( 8.785770181087007913, -10.38731345016515917, -223.4272116603623317 ) ) ;
#13358=CARTESIAN_POINT ( 'NONE',  ( -24.68906941503829700, 2.445024713909649705, -232.6803430500543755 ) ) ;
#13360=CARTESIAN_POINT ( 'NONE',  ( -18.70090456008720992, 23.36146401084868884, -220.3989740370807056 ) ) ;
#13362=CARTESIAN_POINT ( 'NONE',  ( 22.42095341476093040, 9.457779162868732215, -232.6339572190428555 ) ) ;
#13363=SURFACE_SIDE_STYLE ('',( #9660 ) ) ;
#13365=CARTESIAN_POINT ( 'NONE',  ( -3.400000000000003908, 0.000000000000000000, -224.9999999999999716 ) ) ;
#13366=CARTESIAN_POINT ( 'NONE',  ( 15.01439307471096463, 1.118969480519667048, -226.7488225241675366 ) ) ;
#13368=CARTESIAN_POINT ( 'NONE',  ( 14.80019294276752007, -6.608272808847591051, -224.1005182637183566 ) ) ;
#13369=CARTESIAN_POINT ( 'NONE',  ( -26.43144772945995413, -6.745116643720071359, -219.5134289301136050 ) ) ;
#13373=CARTESIAN_POINT ( 'NONE',  ( 5.711092584709906106, 26.13380667269736790, -220.5232813324456629 ) ) ;
#13374=CARTESIAN_POINT ( 'NONE',  ( 10.74287257054252720, -16.14773823008032849, -215.8883494958819824 ) ) ;
#13375=CARTESIAN_POINT ( 'NONE',  ( 21.39922646226391478, -21.53954253117021977, -224.1701659532164967 ) ) ;
#13376=CARTESIAN_POINT ( 'NONE',  ( -14.87932799058895128, 18.71706570923887369, -231.8731726670167745 ) ) ;
#13377=CARTESIAN_POINT ( 'NONE',  ( 12.88374853655145458, 4.106359831454843068, -228.1016120772327440 ) ) ;
#13378=CARTESIAN_POINT ( 'NONE',  ( 12.56556766396551872, 9.776144415819011613, -223.4791766911294815 ) ) ;
#13380=CARTESIAN_POINT ( 'NONE',  ( -8.507271545618831254, -16.45592803179997787, -230.0780227380557790 ) ) ;
#13382=CARTESIAN_POINT ( 'NONE',  ( -12.13692969104051400, -0.3108940857385004697, -222.6170402347994184 ) ) ;
#13383=CARTESIAN_POINT ( 'NONE',  ( 14.28815361401014172, 13.86049093364188778, -216.0585456615740156 ) ) ;
#13384=CARTESIAN_POINT ( 'NONE',  ( 27.38348740615853316, -3.050674415727137045, -231.0934891209028876 ) ) ;
#13385=CARTESIAN_POINT ( 'NONE',  ( 4.907833106823921376, 13.98151846258800290, -229.0190609869640923 ) ) ;
#13386=CARTESIAN_POINT ( 'NONE',  ( -12.31207293045244988, 6.732038552366256923, -221.0952066824360713 ) ) ;
#13388=CARTESIAN_POINT ( 'NONE',  ( 9.616550234602936342, 9.263684773868845923, -230.4827401731016607 ) ) ;
#13390=CARTESIAN_POINT ( 'NONE',  ( -17.91769793922991028, 3.277678596821882007, -219.5526088240203819 ) ) ;
#13391=CARTESIAN_POINT ( 'NONE',  ( -17.75316132689678383, 25.03468689048078843, -222.1645193425721061 ) ) ;
#13393=CARTESIAN_POINT ( 'NONE',  ( 14.02816775221371337, 20.58276248714641810, -218.7180790146936999 ) ) ;
#13395=CARTESIAN_POINT ( 'NONE',  ( -22.05223281125446633, 0.4748437386657422543, -217.8785187290425256 ) ) ;
#13396=CARTESIAN_POINT ( 'NONE',  ( -14.70339349403010942, -0.4153334646997780544, -217.8790668391084466 ) ) ;
#13397=CARTESIAN_POINT ( 'NONE',  ( -13.13215111221786024, -8.938624195428067409, -226.3235457059856515 ) ) ;
#13401=CARTESIAN_POINT ( 'NONE',  ( -4.130417896617784912, 16.21758012034559826, -229.8171973319304584 ) ) ;
#13402=CARTESIAN_POINT ( 'NONE',  ( 2.936803900436826709, -18.74190719154852758, -218.5197582523356061 ) ) ;
#13404=CARTESIAN_POINT ( 'NONE',  ( 12.55473222622303986, 11.30320364856893001, -218.8964119182764989 ) ) ;
#13405=CARTESIAN_POINT ( 'NONE',  ( -4.691002462566371101, 21.98518063340150164, -232.2516024630330094 ) ) ;
#13406=CARTESIAN_POINT ( 'NONE',  ( -10.14083745617744547, 19.87482866967577877, -216.0596634563153486 ) ) ;
#13407=VERTEX_POINT ( 'NONE', #851 ) ;
#13408=CARTESIAN_POINT ( 'NONE',  ( -18.57671526409105667, -15.84599122335686161, -218.9973662248357300 ) ) ;
#13409=CARTESIAN_POINT ( 'NONE',  ( 11.13678936984666912, 26.95732789089726111, -228.8350761760834757 ) ) ;
#13411=CARTESIAN_POINT ( 'NONE',  ( 17.96045420455031305, -0.3746358454349600908, -217.9627609769914613 ) ) ;
#13414=CARTESIAN_POINT ( 'NONE',  ( 24.21331552874348958, 0.07051084380047288602, -231.7986140076958463 ) ) ;
#13415=CARTESIAN_POINT ( 'NONE',  ( 12.74913679152205148, 9.185760885856177893, -218.6542381594888980 ) ) ;
#13417=CARTESIAN_POINT ( 'NONE',  ( -21.99356461413155728, 5.827088221545293045, -219.1725956997024127 ) ) ;
#13419=CARTESIAN_POINT ( 'NONE',  ( -2.328291070394212792, 14.80737693666302945, -219.0291440940735868 ) ) ;
#13420=CARTESIAN_POINT ( 'NONE',  ( 14.92135368508905202, 7.451356898669101447, -219.1823315336843621 ) ) ;
#13422=CARTESIAN_POINT ( 'NONE',  ( -6.651864601267788224, -12.12497212411570580, -228.9083653044881714 ) ) ;
#13424=CARTESIAN_POINT ( 'NONE',  ( -14.34029329777712469, -14.57793623142476669, -217.2545494607695389 ) ) ;
#13425=CARTESIAN_POINT ( 'NONE',  ( -22.04004491965229207, 12.41871177236473578, -215.2165492276571115 ) ) ;
#13426=CARTESIAN_POINT ( 'NONE',  ( 7.080148886126969465, -28.65852557119563926, -219.9679292432588227 ) ) ;
#13427=CARTESIAN_POINT ( 'NONE',  ( 21.26068545928058384, -3.181857413669367141, -233.8217025890263585 ) ) ;
#13428=CARTESIAN_POINT ( 'NONE',  ( -24.76115377241536208, -2.015397159694146456, -231.8500816169410825 ) ) ;
#13429=CARTESIAN_POINT ( 'NONE',  ( 8.812670488384366507, 12.21486833790445914, -225.9961634525829197 ) ) ;
#13431=CARTESIAN_POINT ( 'NONE',  ( -14.60180519431160917, 24.46340507526420893, -221.8423643191928534 ) ) ;
#13432=CARTESIAN_POINT ( 'NONE',  ( 10.14297843322460402, 14.69845403004500639, -219.2805000163441207 ) ) ;
#13433=CARTESIAN_POINT ( 'NONE',  ( 22.46220731426537043, 18.23201731183003460, -227.5436199598787539 ) ) ;
#13434=CARTESIAN_POINT ( 'NONE',  ( 15.03112630398312177, 24.11065413595933293, -226.8236212149936080 ) ) ;
#13435=CARTESIAN_POINT ( 'NONE',  ( 17.14704237169575052, -19.77033640698606121, -215.4809218419665342 ) ) ;
#13438=CARTESIAN_POINT ( 'NONE',  ( -2.328291070394212792, 14.80737693666302945, -219.0291440940735868 ) ) ;
#13441=CARTESIAN_POINT ( 'NONE',  ( 10.57926812561479757, 10.00910231482511215, -225.8341706491384286 ) ) ;
#13442=CARTESIAN_POINT ( 'NONE',  ( 8.222674095483935020, -17.25680718911290512, -231.8150392270642612 ) ) ;
#13443=CARTESIAN_POINT ( 'NONE',  ( -22.07068341299880743, 18.38202870573248049, -227.7785760498121306 ) ) ;
#13444=CARTESIAN_POINT ( 'NONE',  ( -4.855966894080006035, 26.75753167227873064, -230.1547293463117114 ) ) ;
#13445=CARTESIAN_POINT ( 'NONE',  ( -16.05483997570105714, -7.226811045751038165, -218.5819178105544438 ) ) ;
#13446=CARTESIAN_POINT ( 'NONE',  ( -26.64664107080812627, 5.256684826493772000, -228.0533579629717735 ) ) ;
#13448=CARTESIAN_POINT ( 'NONE',  ( 8.343316395906509086, 11.57404413652245800, -231.1403332574589911 ) ) ;
#13449=CARTESIAN_POINT ( 'NONE',  ( 5.169766346882679997, 29.28517558595074988, -221.5178724947562614 ) ) ;
#13450=CARTESIAN_POINT ( 'NONE',  ( 12.14783608763084644, -10.95966212275308571, -222.8518398773795184 ) ) ;
#13451=CARTESIAN_POINT ( 'NONE',  ( 23.27685575300125720, -16.81362096763192326, -220.1650456318757563 ) ) ;
#13454=CARTESIAN_POINT ( 'NONE',  ( 7.168644370073567806, 19.32044210858112265, -233.1278450877711634 ) ) ;
#13455=CARTESIAN_POINT ( 'NONE',  ( -12.17842630902860712, -4.030040138803427929, -228.6515579410213661 ) ) ;
#13456=CARTESIAN_POINT ( 'NONE',  ( -5.525229149912007642, -13.32411127922494742, -220.4018445532201440 ) ) ;
#13457=CARTESIAN_POINT ( 'NONE',  ( 13.91151814069282722, -15.58123622716646572, -216.5183035683795367 ) ) ;
#13458=CARTESIAN_POINT ( 'NONE',  ( -27.40681729237160269, 15.04232492504307572, -225.3323746796125704 ) ) ;
#13459=CARTESIAN_POINT ( 'NONE',  ( 9.322595869360968734, 23.38184458253662967, -230.2763482547081821 ) ) ;
#13460=CARTESIAN_POINT ( 'NONE',  ( -22.11084984981285118, 10.96048252433489623, -216.6117774006995376 ) ) ;
#13461=CARTESIAN_POINT ( 'NONE',  ( -31.04267853410473421, 7.029517189377418873, -226.8060334161593516 ) ) ;
#13462=CARTESIAN_POINT ( 'NONE',  ( -15.65746202990257174, -5.535581341804817868, -220.4933418326074559 ) ) ;
#13464=CARTESIAN_POINT ( 'NONE',  ( -7.250603130619442283, 20.89725557392719324, -217.7893896917081520 ) ) ;
#13465=CARTESIAN_POINT ( 'NONE',  ( 12.96449997971774870, 8.285709878278680662, -230.9518598506670628 ) ) ;
#13466=CARTESIAN_POINT ( 'NONE',  ( -5.974114889119001681, 17.52937113675171332, -232.3862906442651592 ) ) ;
#13467=CARTESIAN_POINT ( 'NONE',  ( 14.49023023880111083, -12.14520762395643061, -217.6171285705176501 ) ) ;
#13470=CARTESIAN_POINT ( 'NONE',  ( -12.74846050492543625, 19.93509882904884734, -216.0172840992881049 ) ) ;
#13471=CARTESIAN_POINT ( 'NONE',  ( -30.53557093151922430, -9.496448454471346778, -222.0905184547210638 ) ) ;
#13474=CARTESIAN_POINT ( 'NONE',  ( 5.623554730548537606, 15.65270319720736225, -231.3185741195121068 ) ) ;
#13476=( GEOMETRIC_REPRESENTATION_CONTEXT ( 3 ) GLOBAL_UNCERTAINTY_ASSIGNED_CONTEXT ( ( #21344 ) ) GLOBAL_UNIT_ASSIGNED_CONTEXT ( ( #11346, #6493, #21905 ) ) REPRESENTATION_CONTEXT ( 'NONE', 'WORKASPACE' ) );
#13477=CARTESIAN_POINT ( 'NONE',  ( 20.98776729843937972, -13.55153944770713359, -217.5092423276211946 ) ) ;
#13478=CARTESIAN_POINT ( 'NONE',  ( -29.30406754532526037, 5.063969254119831120, -221.8212091093853076 ) ) ;
#13479=CARTESIAN_POINT ( 'NONE',  ( -13.43384090552117271, 6.057765724406720231, -225.7182623230366119 ) ) ;
#13480=CARTESIAN_POINT ( 'NONE',  ( 18.79638869589749461, 0.4878066561304963966, -219.5712168927955759 ) ) ;
#13481=CARTESIAN_POINT ( 'NONE',  ( -10.03082531488024109, -22.09229706162428286, -231.9736132431984572 ) ) ;
#13483=CARTESIAN_POINT ( 'NONE',  ( 27.40550551777678123, 5.967061366481472895, -228.7463788799179554 ) ) ;
#13485=CARTESIAN_POINT ( 'NONE',  ( 20.53618124091710939, -19.36892006637360097, -226.5121684596580849 ) ) ;
#13486=CARTESIAN_POINT ( 'NONE',  ( 13.10740018641116400, -2.248054146740232184, -226.9883072097889567 ) ) ;
#13489=CARTESIAN_POINT ( 'NONE',  ( 2.601379523478754674, 17.36677895276155681, -230.4357129074444117 ) ) ;
#13490=CARTESIAN_POINT ( 'NONE',  ( 6.114261689233397412, -11.26162238963769369, -223.0577857700231164 ) ) ;
#13492=CARTESIAN_POINT ( 'NONE',  ( 15.11994912051959972, -12.48385213956034079, -232.8079920308188377 ) ) ;
#13493=EDGE_LOOP ( 'NONE', ( #13224, #15607, #5510, #21117 ) ) ;
#13495=CARTESIAN_POINT ( 'NONE',  ( -15.11329978779464689, 11.41628732213579411, -231.7124318929555500 ) ) ;
#13496=CARTESIAN_POINT ( 'NONE',  ( 15.91624278015930649, 5.932232821383347954, -217.3600859879243217 ) ) ;
#13497=CARTESIAN_POINT ( 'NONE',  ( 13.71585692689473213, 6.523039003617190801, -224.4540437369149402 ) ) ;
#13499=CARTESIAN_POINT ( 'NONE',  ( -8.398697845537501649, -22.62202615048447640, -219.0766901614751703 ) ) ;
#13501=CARTESIAN_POINT ( 'NONE',  ( -13.56011990957801139, -0.3895158544032599202, -219.3211261236655218 ) ) ;
#13503=CARTESIAN_POINT ( 'NONE',  ( 4.914880347045685660, 14.54749271951947698, -232.8668677254037789 ) ) ;
#13504=CARTESIAN_POINT ( 'NONE',  ( 10.07328213880649592, -15.27579949576245966, -229.4560222226588451 ) ) ;
#13505=CARTESIAN_POINT ( 'NONE',  ( 8.689059922489732912, 15.18271246186214363, -218.7354841152034908 ) ) ;
#13506=CARTESIAN_POINT ( 'NONE',  ( -26.74045434827795020, 12.41518252455047744, -220.4617428697642652 ) ) ;
#13507=CARTESIAN_POINT ( 'NONE',  ( 3.711349367426693746, 16.84755988915346236, -233.7359972593521888 ) ) ;
#13509=CARTESIAN_POINT ( 'NONE',  ( -26.70018640714903668, 3.110792036746048428, -228.8761207540193823 ) ) ;
#13510=CARTESIAN_POINT ( 'NONE',  ( -2.735889804569492600, 12.71735652435744512, -225.1194195722198117 ) ) ;
#13511=CARTESIAN_POINT ( 'NONE',  ( 14.80394259695730064, 1.224172658189580432, -225.4564070658925061 ) ) ;
#13512=CARTESIAN_POINT ( 'NONE',  ( -1.643553855084622928, -13.05119293000219294, -222.7191902239112551 ) ) ;
#13513=CARTESIAN_POINT ( 'NONE',  ( 23.12216041205843453, 0.2121350054995089496, -232.0572713672589202 ) ) ;
#13515=CARTESIAN_POINT ( 'NONE',  ( -21.80830016239255897, -4.781675611938959847, -217.4666014280278148 ) ) ;
#13516=CARTESIAN_POINT ( 'NONE',  ( -20.73319232323294514, 5.144688277016327582, -214.6391322078443977 ) ) ;
#13517=CARTESIAN_POINT ( 'NONE',  ( -14.92584319327083442, -9.764953932613968490, -229.6443584147421006 ) ) ;
#13519=CARTESIAN_POINT ( 'NONE',  ( 10.46316887740464985, -17.92901728017801233, -232.6108895528913081 ) ) ;
#13520=CARTESIAN_POINT ( 'NONE',  ( 20.40268796714816801, 18.65534563792085621, -219.5587498978784993 ) ) ;
#13521=CARTESIAN_POINT ( 'NONE',  ( -10.40174557315337900, 22.75579539577861965, -231.4492192189165962 ) ) ;
#13522=CARTESIAN_POINT ( 'NONE',  ( -14.84124724799726991, 21.42277200659090042, -233.6300684249849553 ) ) ;
#13524=CARTESIAN_POINT ( 'NONE',  ( 13.95860357795928941, -2.197645239214564672, -231.3209047126647988 ) ) ;
#13527=CARTESIAN_POINT ( 'NONE',  ( 6.093530912645064745, 16.79941505724243811, -232.1766444656230419 ) ) ;
#13530=CARTESIAN_POINT ( 'NONE',  ( -21.89065952084834166, -0.9940043559354216907, -218.9999999999999716 ) ) ;
#13531=CARTESIAN_POINT ( 'NONE',  ( 25.70350299105564318, 4.008313962570879241, -233.1578316763087173 ) ) ;
#13533=CARTESIAN_POINT ( 'NONE',  ( -15.95680269303277221, -1.471987722620473615, -218.5035227479738751 ) ) ;
#13535=CARTESIAN_POINT ( 'NONE',  ( 23.22505041959077232, 19.39625294115234055, -221.5972645870541555 ) ) ;
#13536=CARTESIAN_POINT ( 'NONE',  ( -23.67953786836281083, 9.946055673977088674, -229.5560005648173671 ) ) ;
#13537=CARTESIAN_POINT ( 'NONE',  ( 1.984991703947643904, 14.51738422979996912, -218.4500278854917781 ) ) ;
#13539=CARTESIAN_POINT ( 'NONE',  ( 16.77055746703809191, 7.081497542956901370, -232.0295235404293521 ) ) ;
#13541=CARTESIAN_POINT ( 'NONE',  ( -9.654146510541638193, -9.431978497097317060, -229.7352898675592314 ) ) ;
#13543=CARTESIAN_POINT ( 'NONE',  ( -18.38002254392888446, -21.81807606669838506, -229.0374583293157968 ) ) ;
#13544=CARTESIAN_POINT ( 'NONE',  ( -26.42613204384124259, 13.88327151024443395, -218.2510073314678323 ) ) ;
#13545=CARTESIAN_POINT ( 'NONE',  ( 15.34510829589250491, -24.56813251781886009, -230.1307231235174982 ) ) ;
#13546=CARTESIAN_POINT ( 'NONE',  ( -0.1571923090946999446, 19.34188126963334398, -216.6893131123363787 ) ) ;
#13547=CARTESIAN_POINT ( 'NONE',  ( 14.51690190576628048, -4.522004643715366257, -218.3468014590714859 ) ) ;
#13548=CARTESIAN_POINT ( 'NONE',  ( -24.15031621174628285, -13.05338392360020627, -219.0842748323915714 ) ) ;
#13549=CARTESIAN_POINT ( 'NONE',  ( 12.55473222622303986, 11.30320364856893001, -218.8964119182764989 ) ) ;
#13552=CARTESIAN_POINT ( 'NONE',  ( -10.30040261405712698, 19.75576125044891285, -218.0811964201226658 ) ) ;
#13553=CARTESIAN_POINT ( 'NONE',  ( 9.125049424194871861, 12.37796447639467523, -227.2539065556229332 ) ) ;
#13554=CARTESIAN_POINT ( 'NONE',  ( 23.04897566969193079, 17.95862962700741861, -223.6438515760422661 ) ) ;
#13555=CARTESIAN_POINT ( 'NONE',  ( 9.125049424194871861, 12.37796447639467523, -227.2539065556229332 ) ) ;
#13556=CARTESIAN_POINT ( 'NONE',  ( 0.5573677079071300833, -14.80782849724859496, -218.9269569601107719 ) ) ;
#13557=CARTESIAN_POINT ( 'NONE',  ( -9.523248388595575875, 12.31121908620753125, -221.6288572946744182 ) ) ;
#13561=CARTESIAN_POINT ( 'NONE',  ( 24.03642272140365677, 3.646960756862087205, -218.2320643939070806 ) ) ;
#13562=CARTESIAN_POINT ( 'NONE',  ( 3.692943796146577196, -17.43777048755501724, -232.3481250940208156 ) ) ;
#13563=CARTESIAN_POINT ( 'NONE',  ( -13.75208518020500748, 5.661250135068270239, -227.6647651141479685 ) ) ;
#13564=CARTESIAN_POINT ( 'NONE',  ( -0.7041916573665241152, 14.60214745152014437, -226.3818583194645555 ) ) ;
#13565=CARTESIAN_POINT ( 'NONE',  ( -11.20272313682045073, -7.956653478762055087, -225.3025344850567819 ) ) ;
#13566=CARTESIAN_POINT ( 'NONE',  ( -20.41147829968989313, 3.432784889297933795, -230.9611049257633510 ) ) ;
#13567=CARTESIAN_POINT ( 'NONE',  ( 24.81668481317358399, 17.11438712655213124, -222.1096362285750274 ) ) ;
#13569=CARTESIAN_POINT ( 'NONE',  ( -9.716674560061926869, 27.56227806819028103, -219.4917914922789919 ) ) ;
#13570=CARTESIAN_POINT ( 'NONE',  ( 14.06411491198613462, -8.094314315948059502, -222.2253600114596566 ) ) ;
#13571=CARTESIAN_POINT ( 'NONE',  ( 12.90505172109588194, -11.18139282378177768, -218.7382941517081747 ) ) ;
#13573=CARTESIAN_POINT ( 'NONE',  ( 11.13678936984666912, 26.95732789089726111, -228.8350761760834757 ) ) ;
#13574=CARTESIAN_POINT ( 'NONE',  ( -9.690988788510356500, -7.266623515821958534, -222.7221403394456445 ) ) ;
#13575=CARTESIAN_POINT ( 'NONE',  ( -6.052919920376759855, -15.38051382379660836, -218.0337201863237624 ) ) ;
#13576=CARTESIAN_POINT ( 'NONE',  ( 15.34510829589250491, -24.56813251781886009, -230.1307231235174982 ) ) ;
#13577=CARTESIAN_POINT ( 'NONE',  ( -18.17591565587962776, 16.23604867791855355, -233.2845329962925121 ) ) ;
#13578=CARTESIAN_POINT ( 'NONE',  ( 12.84032013659066251, 19.10303921738740485, -230.8110334357214128 ) ) ;
#13579=CARTESIAN_POINT ( 'NONE',  ( -27.82842955277035202, 11.70195273568964112, -227.9294339757464911 ) ) ;
#13580=CARTESIAN_POINT ( 'NONE',  ( -25.98311979368102342, 15.13734258059737670, -220.6162231662327429 ) ) ;
#13581=CARTESIAN_POINT ( 'NONE',  ( -15.57180599510074437, -4.609960555941468918, -228.7341395176208323 ) ) ;
#13583=CARTESIAN_POINT ( 'NONE',  ( -4.715783688792956063, 28.29821729825949816, -228.0423900005874600 ) ) ;
#13584=CARTESIAN_POINT ( 'NONE',  ( 29.89309326230132058, 6.052383583152112223, -228.3539431708548477 ) ) ;
#13585=CARTESIAN_POINT ( 'NONE',  ( 5.264801124131998300, 10.54092478143144795, -226.4890466082630098 ) ) ;
#13586=CARTESIAN_POINT ( 'NONE',  ( 22.55746627616819566, -14.21542447219996852, -231.9819121152456205 ) ) ;
#13589=CARTESIAN_POINT ( 'NONE',  ( -6.571166997218196748, 12.74865329367398736, -229.9840124400968762 ) ) ;
#13590=CARTESIAN_POINT ( 'NONE',  ( -14.38198375515248273, -6.747285987484331393, -233.1569015480179985 ) ) ;
#13592=CARTESIAN_POINT ( 'NONE',  ( 14.95414693437772868, 8.262206471704862665, -230.1862972580043163 ) ) ;
#13594=CARTESIAN_POINT ( 'NONE',  ( 14.18709644517307922, -11.45356969546147496, -232.2178450427173004 ) ) ;
#13595=CARTESIAN_POINT ( 'NONE',  ( -19.25929423112888017, 9.818144317380269825, -216.1837936240308409 ) ) ;
#13597=CARTESIAN_POINT ( 'NONE',  ( 14.92135368508905202, 7.451356898669101447, -219.1823315336843621 ) ) ;
#13598=CARTESIAN_POINT ( 'NONE',  ( -13.01444359484612079, -23.32256785062423887, -219.1545357706015693 ) ) ;
#13600=CARTESIAN_POINT ( 'NONE',  ( 22.03647168420945590, 0.3315607655625663064, -232.0572713672586644 ) ) ;
#13601=CARTESIAN_POINT ( 'NONE',  ( -16.71711190488355570, 0.6105529133557690002, -230.9511258789794681 ) ) ;
#13602=CARTESIAN_POINT ( 'NONE',  ( 12.33825063215758888, -15.78239559842968909, -231.3245247598261471 ) ) ;
#13603=CARTESIAN_POINT ( 'NONE',  ( -29.27492217116574480, -1.185422171198730501, -224.8132346143397342 ) ) ;
#13605=CARTESIAN_POINT ( 'NONE',  ( 12.00334754111224100, 12.62951371569041115, -228.5814949098771649 ) ) ;
#13606=CARTESIAN_POINT ( 'NONE',  ( 1.430961520682887400, 16.89318350835024063, -220.3256763723340157 ) ) ;
#13607=CARTESIAN_POINT ( 'NONE',  ( 10.59985392024617745, -10.68425835910226418, -232.2123170752960277 ) ) ;
#13608=CARTESIAN_POINT ( 'NONE',  ( 14.65870393774896030, -26.09170264574407838, -221.2973805112574723 ) ) ;
#13610=CARTESIAN_POINT ( 'NONE',  ( -14.22255565734842619, 21.32307452572284134, -218.8849463683180261 ) ) ;
#13611=CARTESIAN_POINT ( 'NONE',  ( -15.37153448429513602, 5.014568651886798456, -224.5085656291724945 ) ) ;
#13612=CARTESIAN_POINT ( 'NONE',  ( 26.92457506054779515, 6.538608665672222209, -219.8654465082432807 ) ) ;
#13614=CARTESIAN_POINT ( 'NONE',  ( -11.76273268715550913, -21.77324546118368787, -230.3967548854103313 ) ) ;
#13617=CARTESIAN_POINT ( 'NONE',  ( 11.20580770355584299, 27.81589616365139150, -231.3138133330081132 ) ) ;
#13618=CARTESIAN_POINT ( 'NONE',  ( 13.95302107590712737, -11.87212821339389812, -220.3052895324516385 ) ) ;
#13619=CARTESIAN_POINT ( 'NONE',  ( 4.730976410881341465, 17.65764351829336931, -217.6025626048331674 ) ) ;
#13620=CARTESIAN_POINT ( 'NONE',  ( -21.89482327431018760, 1.733733432562314158, -233.1353281693111796 ) ) ;
#13623=CARTESIAN_POINT ( 'NONE',  ( 23.07558131619435571, 16.33594519118144817, -217.0553921114837124 ) ) ;
#13624=CARTESIAN_POINT ( 'NONE',  ( -15.46752262371512820, 15.15798787883389487, -233.5981584775992701 ) ) ;
#13625=CARTESIAN_POINT ( 'NONE',  ( -2.817219543927646175, 14.13981714106644993, -229.6779615865167443 ) ) ;
#13626=CARTESIAN_POINT ( 'NONE',  ( 16.64225601860865211, 1.926018578292457928, -220.2177910260893725 ) ) ;
#13627=CARTESIAN_POINT ( 'NONE',  ( 6.131461862964278531, -15.14974102410872625, -231.6805438559109973 ) ) ;
#13628=CARTESIAN_POINT ( 'NONE',  ( 26.48152825632016061, -2.044474411990439666, -219.3412966555575565 ) ) ;
#13629=DIRECTION ( 'NONE',  ( 0.000000000000000000, 0.000000000000000000, -1.000000000000000000 ) ) ;
#13631=CARTESIAN_POINT ( 'NONE',  ( 16.91879448796214191, 0.8271603773820436212, -230.0510230802265710 ) ) ;
#13632=CARTESIAN_POINT ( 'NONE',  ( -15.89829452305285606, -16.08449805557013335, -231.9408725418336701 ) ) ;
#13634=CARTESIAN_POINT ( 'NONE',  ( 6.679827377097204533, -23.59744646493245668, -231.8618301756397670 ) ) ;
#13635=CARTESIAN_POINT ( 'NONE',  ( -13.81390866287826746, 1.832988708064121175, -224.4361041349432639 ) ) ;
#13636=CARTESIAN_POINT ( 'NONE',  ( -0.1881941282075867139, 17.37563936270229092, -230.9177995227891813 ) ) ;
#13637=CARTESIAN_POINT ( 'NONE',  ( -16.58369694688956741, 24.75758513462668375, -230.3405478298966784 ) ) ;
#13639=CARTESIAN_POINT ( 'NONE',  ( -16.74998343472315199, -3.152285961911668988, -228.0274629056708022 ) ) ;
#13641=CARTESIAN_POINT ( 'NONE',  ( 10.78187269046063435, 10.73871010366167944, -221.9206544238666368 ) ) ;
#13642=CARTESIAN_POINT ( 'NONE',  ( -23.30382222616342247, 9.914163031146200566, -218.5285240371296425 ) ) ;
#13643=CARTESIAN_POINT ( 'NONE',  ( -14.08236938285573636, 6.062428076406559008, -221.7923619418395447 ) ) ;
#13645=CARTESIAN_POINT ( 'NONE',  ( 22.73582563804385970, 20.20868311426415431, -227.8513184012435886 ) ) ;
#13646=CARTESIAN_POINT ( 'NONE',  ( -16.04492519386327487, 1.819644280589142626, -223.4665098021627614 ) ) ;
#13647=CARTESIAN_POINT ( 'NONE',  ( 2.276720224425493821, 13.44951395023989171, -229.9230017221896105 ) ) ;
#13648=CARTESIAN_POINT ( 'NONE',  ( 22.42095341476093040, 9.457779162868732215, -232.6339572190428555 ) ) ;
#13650=CARTESIAN_POINT ( 'NONE',  ( -11.54310632260721903, -10.65784888458977697, -232.4489430773787149 ) ) ;
#13652=CARTESIAN_POINT ( 'NONE',  ( -14.26331330459994540, -11.99770975811722451, -232.1846756268951708 ) ) ;
#13653=CARTESIAN_POINT ( 'NONE',  ( -7.329856113536736828, 10.17606210583481818, -226.3085553030691415 ) ) ;
#13654=CARTESIAN_POINT ( 'NONE',  ( 5.434900225474387447, -11.93567727083262042, -224.7511004068755369 ) ) ;
#13655=CARTESIAN_POINT ( 'NONE',  ( 0.6364901924797052857, 13.89978473517355617, -221.8840706290426397 ) ) ;
#13656=CARTESIAN_POINT ( 'NONE',  ( 11.97659261343968851, -3.740017786417877854, -223.6042415182018033 ) ) ;
#13657=CARTESIAN_POINT ( 'NONE',  ( -28.55814054826834791, -1.660722980825670048, -228.2640858091212408 ) ) ;
#13658=CARTESIAN_POINT ( 'NONE',  ( 12.79953165872901266, 10.20044330008568778, -230.3912386799665626 ) ) ;
#13660=CARTESIAN_POINT ( 'NONE',  ( -0.3589900283600636066, 18.35437183075527656, -220.3960288481451357 ) ) ;
#13661=CARTESIAN_POINT ( 'NONE',  ( 12.63974878616558328, 15.03448928898568759, -231.7036488814491406 ) ) ;
#13662=CARTESIAN_POINT ( 'NONE',  ( 12.71450444683213021, 7.595266944807587350, -224.4213778964231665 ) ) ;
#13663=CARTESIAN_POINT ( 'NONE',  ( 26.51393280883522863, 15.12455065102723495, -226.1955201378414415 ) ) ;
#13664=CARTESIAN_POINT ( 'NONE',  ( 6.679393088666140343, -31.31585170264869689, -224.7195491891107793 ) ) ;
#13665=CARTESIAN_POINT ( 'NONE',  ( -11.55316006017064012, 19.79513644261079719, -232.3088878043970453 ) ) ;
#13666=CARTESIAN_POINT ( 'NONE',  ( 24.58316096239279602, 5.861425670879941485, -231.3104446318280623 ) ) ;
#13668=CARTESIAN_POINT ( 'NONE',  ( 14.02967383842077709, -23.07461891086659378, -219.7428183145782725 ) ) ;
#13669=CARTESIAN_POINT ( 'NONE',  ( -11.05032764129755840, 11.65053160594169945, -221.1796278216217218 ) ) ;
#13670=CARTESIAN_POINT ( 'NONE',  ( 10.31623634631035991, 26.83927646318382898, -220.2315638557092541 ) ) ;
#13671=CARTESIAN_POINT ( 'NONE',  ( -14.76273180397945772, -6.370707202906876532, -220.0066229284273334 ) ) ;
#13672=CARTESIAN_POINT ( 'NONE',  ( -16.37512411505367282, 2.406627362596846620, -227.7341547288202719 ) ) ;
#13673=CARTESIAN_POINT ( 'NONE',  ( 9.851209273476317918, 25.48401176094959553, -233.7173763849377792 ) ) ;
#13675=CARTESIAN_POINT ( 'NONE',  ( 10.85888002857596923, 15.81835858589122878, -232.3913150909872627 ) ) ;
#13676=CARTESIAN_POINT ( 'NONE',  ( 15.93530172229541364, -10.24337635388110890, -230.8272463582829630 ) ) ;
#13677=CARTESIAN_POINT ( 'NONE',  ( 24.57161139520042781, -7.530326316930160857, -232.9949629211864419 ) ) ;
#13679=CARTESIAN_POINT ( 'NONE',  ( 3.449504654906655254, 27.59247159270940841, -231.3461799890608859 ) ) ;
#13680=CARTESIAN_POINT ( 'NONE',  ( -30.26911233660276679, -7.575179034252494503, -222.6017624672529109 ) ) ;
#13681=CARTESIAN_POINT ( 'NONE',  ( -5.519971913460887336, -12.21762732219001713, -227.2962593638428359 ) ) ;
#13682=CARTESIAN_POINT ( 'NONE',  ( 5.953549895739506326, -12.70069413479034104, -221.3143591192976203 ) ) ;
#13683=CARTESIAN_POINT ( 'NONE',  ( -21.72273972318264867, 21.08396222359856864, -224.0477214759881690 ) ) ;
#13684=CARTESIAN_POINT ( 'NONE',  ( 5.066530254613678785, 15.76189963344335254, -222.1234037505291781 ) ) ;
#13685=CARTESIAN_POINT ( 'NONE',  ( -16.65698539163286540, 11.03290537638306112, -233.6474915129378758 ) ) ;
#13686=CARTESIAN_POINT ( 'NONE',  ( -27.05172747931452903, 14.36075930490012276, -228.5082213655825853 ) ) ;
#13687=CARTESIAN_POINT ( 'NONE',  ( -17.67448836398429890, -11.08962652971676199, -218.7915233441472367 ) ) ;
#13689=CARTESIAN_POINT ( 'NONE',  ( -4.855966894080006035, 26.75753167227873064, -230.1547293463117114 ) ) ;
#13690=CARTESIAN_POINT ( 'NONE',  ( 12.23284375931666013, 4.108221165122169616, -224.0993108960438462 ) ) ;
#13691=CARTESIAN_POINT ( 'NONE',  ( 5.434119414999338815, 11.18343085245738777, -221.0450680983404936 ) ) ;
#13693=CARTESIAN_POINT ( 'NONE',  ( 24.05238142633148968, -17.07083877791421500, -221.4615098029387070 ) ) ;
#13697=CARTESIAN_POINT ( 'NONE',  ( -4.620781219515533778, 16.99182040716223696, -217.1278208835672672 ) ) ;
#13699=CARTESIAN_POINT ( 'NONE',  ( -17.45568254742804370, -7.678338623619185732, -234.9220303918225738 ) ) ;
#13701=CARTESIAN_POINT ( 'NONE',  ( 15.61962121506769385, 4.525360868525488911, -229.0684696061408090 ) ) ;
#13702=CARTESIAN_POINT ( 'NONE',  ( -25.29098058636142810, 5.014641116111857144, -217.4658967307323110 ) ) ;
#13703=CARTESIAN_POINT ( 'NONE',  ( 10.10435529162921853, -13.32996982371095918, -231.5224098423250894 ) ) ;
#13705=CARTESIAN_POINT ( 'NONE',  ( -14.10849459794400751, -0.2436790717799666162, -223.1085195285415921 ) ) ;
#13706=CARTESIAN_POINT ( 'NONE',  ( -26.58771759052039485, 5.114955214121561511, -218.2823714869195442 ) ) ;
#13707=CARTESIAN_POINT ( 'NONE',  ( -0.6703493356118243041, -28.01673786290986712, -221.2203946787553548 ) ) ;
#13711=CARTESIAN_POINT ( 'NONE',  ( 18.46162736253148395, -12.23454570505295358, -218.9425382959138062 ) ) ;
#13712=CARTESIAN_POINT ( 'NONE',  ( 14.66528321205121976, -2.062017816318827190, -227.1804948401301374 ) ) ;
#13714=CARTESIAN_POINT ( 'NONE',  ( 16.48099188159542194, 16.04875567542346815, -230.8408106201084706 ) ) ;
#13715=CARTESIAN_POINT ( 'NONE',  ( 1.313727069624702981, 17.80710275190598324, -219.4197901500037062 ) ) ;
#13716=CARTESIAN_POINT ( 'NONE',  ( 20.77649313750695370, -15.65279155457156435, -215.5859610257211898 ) ) ;
#13718=CARTESIAN_POINT ( 'NONE',  ( 8.649266908999912573, -10.50942778440553482, -226.4415026780416440 ) ) ;
#13720=CARTESIAN_POINT ( 'NONE',  ( -8.030397104878142400, 15.90963402996711373, -230.6518438502475590 ) ) ;
#13721=CARTESIAN_POINT ( 'NONE',  ( -23.99493126334580850, 6.052326449358573335, -219.7958990219547672 ) ) ;
#13722=CARTESIAN_POINT ( 'NONE',  ( 15.88536911906737181, 12.85343532334862893, -218.9532478288372204 ) ) ;
#13723=CARTESIAN_POINT ( 'NONE',  ( -9.501265986711061373, -18.16888683615402300, -230.9326763462221948 ) ) ;
#13726=CARTESIAN_POINT ( 'NONE',  ( 22.44730228620155899, 3.608729811217749717, -232.0798239124179645 ) ) ;
#13727=CARTESIAN_POINT ( 'NONE',  ( 12.24130115618514125, -19.65891960071846967, -230.7381047918825914 ) ) ;
#13728=CARTESIAN_POINT ( 'NONE',  ( 5.169766346882679997, 29.28517558595074988, -221.5178724947562614 ) ) ;
#13729=CARTESIAN_POINT ( 'NONE',  ( -15.58461825850822180, 18.91734573546571951, -233.7691177939990723 ) ) ;
#13731=CARTESIAN_POINT ( 'NONE',  ( 26.50744623559791435, 1.694095366541529923, -217.6968951254705473 ) ) ;
#13734=CARTESIAN_POINT ( 'NONE',  ( -6.571166997218196748, 12.74865329367398736, -229.9840124400968762 ) ) ;
#13735=CARTESIAN_POINT ( 'NONE',  ( -3.400000000000003908, 0.000000000000000000, -224.9999999999999716 ) ) ;
#13736=CARTESIAN_POINT ( 'NONE',  ( -3.734153817218577309, -19.72686645808614614, -233.9207428641194610 ) ) ;
#13738=FACE_OUTER_BOUND ( 'NONE', #20511, .T. ) ;
#13740=CARTESIAN_POINT ( 'NONE',  ( -23.84209965496292227, -7.976777114481962805, -232.1458837748831456 ) ) ;
#13741=B_SPLINE_CURVE_WITH_KNOTS ( 'NONE', 3,
 ( #8758, #20883, #18982, #15953, #10439, #13937, #5469, #17532, #7068, #12469 ),
 .UNSPECIFIED., .F., .F.,
 ( 4, 2, 2, 2, 4 ),
 ( 0.4925451859516016828, 0.4926212833915588618, 0.4960388740592901469, 0.4979917830122794764, 0.4999446919652688059 ),
 .UNSPECIFIED. ) ;
#13742=CARTESIAN_POINT ( 'NONE',  ( -13.09048442463468120, -0.002406630494250819839, -229.7150300986316438 ) ) ;
#13743=CARTESIAN_POINT ( 'NONE',  ( -15.00281653375496127, -15.21317112889928858, -231.9690514080965613 ) ) ;
#13746=CARTESIAN_POINT ( 'NONE',  ( 13.60960062514055657, -26.18013421850907108, -225.9721930653775246 ) ) ;
#13747=CARTESIAN_POINT ( 'NONE',  ( 22.16968511661519869, 1.542591969257184337, -234.6098499860488573 ) ) ;
#13748=CARTESIAN_POINT ( 'NONE',  ( -1.772400894765090662, 19.49811434610897010, -217.8797837662441168 ) ) ;
#13749=CARTESIAN_POINT ( 'NONE',  ( -9.439286754415764591, 28.32957437491962338, -228.7842975624562598 ) ) ;
#13750=CARTESIAN_POINT ( 'NONE',  ( 22.56961104628404868, -1.854966590244772950, -214.8717168148014025 ) ) ;
#13751=CARTESIAN_POINT ( 'NONE',  ( 15.91295838535984331, 21.88410254487826379, -230.9583961155862823 ) ) ;
#13752=CARTESIAN_POINT ( 'NONE',  ( -16.88427011841620029, 9.219900108593305887, -231.9155403335099948 ) ) ;
#13753=CARTESIAN_POINT ( 'NONE',  ( -19.84402263676350131, 8.565754689849573111, -217.6561116767911983 ) ) ;
#13754=CARTESIAN_POINT ( 'NONE',  ( -15.95714424191699266, -19.90201571590360885, -231.7641511196865451 ) ) ;
#13757=CARTESIAN_POINT ( 'NONE',  ( 30.52813181070726856, 5.438803974502569361, -223.5441926215666513 ) ) ;
#13758=CARTESIAN_POINT ( 'NONE',  ( -16.54465188417290022, 6.134005835925411709, -228.8256222654843270 ) ) ;
#13759=CARTESIAN_POINT ( 'NONE',  ( 13.79814099039094089, 16.09927043668092850, -214.6489469124405502 ) ) ;
#13760=CARTESIAN_POINT ( 'NONE',  ( 13.06625079052675531, 10.14096931681969238, -232.1435240729728093 ) ) ;
#13761=CARTESIAN_POINT ( 'NONE',  ( -5.974374721719333259, -11.49502099717533454, -225.7652523315031488 ) ) ;
#13764=CARTESIAN_POINT ( 'NONE',  ( -4.994543945659216000, -15.01629888130124435, -221.3392717856295633 ) ) ;
#13765=CARTESIAN_POINT ( 'NONE',  ( -6.079211283031130897, 16.94466709905296753, -232.9163774423793711 ) ) ;
#13766=CARTESIAN_POINT ( 'NONE',  ( 6.741123954526870854, -14.00899218320067341, -219.0418835583997179 ) ) ;
#13767=CARTESIAN_POINT ( 'NONE',  ( -11.42613629117093765, 28.09170287990588832, -228.7150250545069241 ) ) ;
#13768=CARTESIAN_POINT ( 'NONE',  ( 23.46500920064399409, -11.67104692860896620, -233.8722294412333724 ) ) ;
#13769=CARTESIAN_POINT ( 'NONE',  ( -17.58118739749173898, -8.238107657346720458, -217.5252134542318458 ) ) ;
#13770=CARTESIAN_POINT ( 'NONE',  ( -24.15814485343234352, 4.373587128574028426, -232.6698675874553430 ) ) ;
#13772=CARTESIAN_POINT ( 'NONE',  ( -5.560972518124746244, 14.60655266358653215, -227.5460946431043681 ) ) ;
#13773=CARTESIAN_POINT ( 'NONE',  ( 21.17011458613547248, 1.652544727609948527, -234.6098499860487152 ) ) ;
#13774=CARTESIAN_POINT ( 'NONE',  ( 17.99029889091409018, 9.613712288440757092, -232.0298403238024036 ) ) ;
#13775=CARTESIAN_POINT ( 'NONE',  ( 29.01678366425524658, 8.126504218505314014, -229.6975090854573125 ) ) ;
#13776=CARTESIAN_POINT ( 'NONE',  ( -0.07228948136920625156, -12.49432715273631445, -224.3346527204968766 ) ) ;
#13777=CARTESIAN_POINT ( 'NONE',  ( 5.964915545484365644, 11.50358694729900577, -229.9646467236423462 ) ) ;
#13779=( BOUNDED_SURFACE ( )  B_SPLINE_SURFACE ( 3, 3, ( 
 ( #20100, #4689, #11563, #16972, #18438, #3336, #10218, #9884, #12018, #16748, #8539, #8427, #13601, #15403, #17087, #15070, #21908, #7406, #17300, #1770, #15505, #19316, #419, #6956, #7293, #12238, #21108, #2099, #7183, #12573, #14276, #19417, #14165, #4001, #312, #20773, #7069, #8979, #8871, #17420, #21000, #10440, #5693, #5355, #13938, #2205, #1989, #13828, #14048, #85, #9085, #5590, #20664, #5246, #12128, #17193, #15735, #18983, #12470, #3895, #8644, #3562, #1875, #17638, #20884, #5470, #15954, #12354, #19204, #528, #8759, #15619, #200, #19089, #10772, #3665, #10551, #3785, #10667, #17533, #15843, #852, #6247, #1073, #13121, #7840, #19967, #16276, #12681, #4224, #16066, #9412, #2753, #19639, #14706, #7947, #2647, #9528, #11209, #7729, #14600, #21541, #637, #14380, #21435, #14811, #7513, #5916, #10995, #19851, #19746, #10876, #18075, #966, #6131, #11103, #17754, #2535, #13005, #16171, #2317, #6025, #11321, #21320, #19530, #21214, #9203, #17971, #12899, #17865, #4326, #4438, #16387, #16496, #18190, #9634, #5800, #21654, #4116, #2427, #9310, #741, #7617, #14485, #12793, #4662, #15265, #9970, #1298, #17058, #18408, #9742, #11535, #3305, #18738, #9856, #8512, #1185, #20294, #18299, #10078, #22222, #20179, #21990, #10188, #8279, #15375, #2858, #1635, #2970, #22115, #16829, #8172, #6813, #16721, #16604, #15038, #13679, #4554, #21879, #11430, #8064, #4889, #14929, #16943, #21768, #4773, #6468, #13337, #11769, #18521, #11650, #1519, #20075, #6357, #3087, #1407, #11874, #15148, #13229, #6583, #13454, #18633, #8397, #3195, #6702, #13573, #20409, #4998, #10302, #17503, #15814, #7377, #10744, #5105, #20970, #5327, #12209, #12436, #10518, #8840, #19287, #17610, #20634, #11986, #18847, #391, #3751, #17165, #10636, #15589, #2176, #5438, #17386, #15923, #9057, #501, #2070, #20515, #3637, #51, #13911, #3422, #19062, #3864, #7039, #8950, #1743, #12320, #19174, #20854, #1962, #15706, #7262, #8617, #15477, #283, #6924, #13793, #170, #5219, #14132, #7152, #12100, #5558, #18955, #3531, #20746, #10411, #14018, #17272, #1846, #8724, #17941, #14677, #2397, #16036, #19390, #1045, #7586, #2505, #21184, #5884, #11179, #9383, #19822, #21511, #14455, #14245, #21288, #6102, #9280, #19610, #4195, #16356, #12543, #18160, #7483, #16245, #7812, #5770, #4407, #18046, #16140, #11289, #21078, #17833, #19716, #712, #12760, #11073, #9173, #7699, #12974, #820, #14568, #608, #21405, #5995, #2725, #9496, #2615, #12868, #16468, #19497, #14352, #4085, #9606, #5665, #3973, #4297, #10847, #17721, #934, #12651, #2287 ),
 ( #10962, #3277, #20379, #10162, #4862, #17031, #13307, #9714, #1268, #13090, #6438, #22082, #16688, #11739, #4973, #21960, #6553, #8254, #20149, #4742, #18607, #19936, #11402, #18493, #11848, #4524, #2940, #8032, #16915, #16803, #7918, #15121, #20266, #3169, #8144, #14781, #21849, #10052, #13202, #21623, #11621, #8367, #18376, #16575, #18271, #6215, #15009, #3053, #14898, #9943, #1489, #1378, #13544, #15237, #13425, #2832, #6672, #18713, #1156, #21737, #6329, #20047, #4634, #11508, #9827, #12290, #7007, #20604, #14103, #15453, #6784, #1717, #367, #15788, #19142, #10718, #20940, #8484, #2044, #8693, #15559, #7234, #13879, #12180, #5527, #12406, #8592, #15348, #22196, #3722, #7123, #13653, #13990, #18929, #19257, #8812, #20717, #3837, #1606, #20488, #20826, #5079, #5298, #3393, #17244, #11960, #139, #18821, #10383, #5407, #10275, #15675, #255, #1932, #19034, #3611, #10604, #17141, #25, #10489, #6895, #13765, #3504, #5190, #17473, #17355, #12072, #8922, #1815, #12848, #4059, #17584, #9255, #5971, #581, #19797, #21263, #18022, #5744, #19365, #474, #4381, #10934, #5856, #2261, #16114, #14545, #12737, #908, #2589, #17807, #2150, #2372, #9472, #19582, #16332, #4171, #21487, #15894, #7788, #17692, #19690, #687, #14324, #14654, #9144, #7348, #16005, #6078, #12953, #7456, #9030, #14214, #11049, #21049, #795, #5639, #7562, #21156, #12624, #2479, #14430, #17915, #7675, #10822, #12515, #19470, #9361, #3946, #16220, #21381, #4276, #11156, #18881, #15407, #14757, #16447, #21597, #20668, #3228, #1020, #8544, #2701, #4500, #6737, #10223, #10335, #15509, #7897, #2810, #21713, #18352, #6960, #90, #3456, #6188, #13180, #3340, #1128, #11266, #14872, #10111, #17091, #8004, #1669, #18248, #18135, #1774, #18772, #13832, #11485, #6305, #17198, #9584, #8648, #20023, #13067, #11907, #1556, #19911, #11379, #9689, #16550, #4610, #16976, #8431, #15298, #22148, #13605, #22253, #20442, #5031, #6846, #13714, #20552, #5140, #12022, #15623, #14052, #17643, #12132, #14384, #19319, #640, #15739, #10672, #17537, #7408, #3567, #9207, #20777, #423, #21112, #19093, #17758, #2209, #7186, #10882, #5252, #8875, #10775, #317, #20888, #5475, #204, #21003, #19420, #2103, #12358, #7074, #8984, #19208, #16070, #531, #9091, #15847, #7516, #10554, #5359, #17424, #2322, #18987, #4006, #3899, #10444, #17304, #3789, #12243, #12474, #7298, #14168, #1880, #5697, #5593, #8763, #15958, #3670, #1993, #14278, #13943, #12577, #14710, #2651, #9638, #4228, #21218, #16609, #21545, #4558, #19857, #1191, #19643, #19971, #9417, #11434, #5920 ),
 ( #9314, #7734, #11325, #5805, #8068, #13010, #12686, #16282, #4330, #11214, #1077, #19533, #2862, #14491, #16392, #14816, #12797, #18303, #18194, #856, #9746, #4120, #2539, #4442, #14604, #21439, #6029, #16175, #6136, #13125, #18081, #12903, #745, #9532, #19750, #11001, #16500, #2757, #970, #17869, #11107, #21326, #17975, #2431, #7622, #7844, #7951, #21661, #6251, #13458, #8176, #22119, #6589, #3199, #3426, #15379, #9974, #20079, #20413, #13341, #15042, #4779, #17169, #21883, #8402, #18637, #3309, #20183, #14933, #10306, #15269, #20519, #13577, #6361, #6472, #10082, #5002, #13683, #18851, #4666, #11654, #3091, #21994, #1747, #21772, #22226, #11539, #16834, #6706, #18525, #13233, #1411, #20298, #11878, #8283, #18742, #15152, #18413, #5109, #10194, #2976, #4893, #11773, #11991, #9860, #16725, #16947, #6817, #17062, #1523, #1302, #1639, #8516, #3977, #19066, #14022, #20858, #10748, #6928, #12547, #1850, #3755, #2180, #174, #21082, #5563, #10522, #14249, #17725, #12213, #14136, #3641, #17392, #1966, #3535, #2074, #505, #5442, #8844, #10415, #12324, #15710, #19394, #3868, #12441, #19179, #10851, #13915, #8728, #20750, #5669, #8621, #7381, #395, #15482, #13799, #7156, #15595, #15818, #287, #10640, #55, #9061, #17507, #20638, #20975, #7043, #5331, #8954, #5223, #7266, #19291, #17614, #15927, #12104, #18959, #17276, #18050, #7922, #938, #16040, #17837, #19721, #7816, #1049, #6219, #14356, #16144, #12766, #9387, #19942, #13094, #9610, #7487, #4199, #16362, #14459, #11406, #5888, #16249, #14681, #21292, #21515, #9284, #2292, #14786, #9500, #4529, #2509, #19614, #21627, #9177, #612, #11078, #16472, #2619, #14573, #21189, #5774, #12655, #716, #19501, #17945, #4090, #7590, #10967, #824, #6107, #5999, #2402, #7703, #21409, #12872, #4301, #11183, #12978, #19826, #4411, #11294, #18166, #2729, #20385, #16579, #22201, #11512, #13429, #11853, #9831, #8490, #15242, #20153, #1611, #5084, #21853, #1494, #13311, #4746, #11625, #13206, #11744, #10167, #1383, #18497, #20051, #15125, #3059, #6790, #13549, #22087, #8258, #20494, #1274, #18381, #8148, #15354, #13658, #17036, #10057, #18275, #1160, #16807, #2944, #3173, #9947, #6557, #2836, #18718, #21964, #8036, #8372, #16692, #15013, #6442, #9718, #20270, #18611, #4867, #6678, #16920, #14902, #21743, #4978, #6333, #3282, #4638, #5195, #7128, #10609, #10723, #15899, #1723, #3509, #144, #19040, #7353, #479, #19263, #17146, #13886, #3727, #1821, #21056, #15564, #3616, #17480, #8698, #2049, #18934, #11965, #2155, #19149, #14220, #12185, #7012, #17589, #18826 ),
 ( #3843, #5303, #3398, #10495, #9035, #13995, #10281, #15682, #8597, #15459, #31, #12078, #372, #17360, #20722, #6900, #10389, #13770, #17249, #20609, #1937, #8817, #8927, #260, #20831, #5413, #12295, #15793, #7239, #14108, #20945, #5533, #12411, #19695, #4282, #5977, #4177, #17921, #9477, #10826, #9149, #16225, #9590, #2265, #692, #5749, #14659, #14550, #1025, #12853, #18027, #913, #14435, #5644, #19587, #16337, #10939, #7902, #9366, #6083, #16119, #7461, #17697, #14762, #21269, #801, #12629, #11054, #2595, #7680, #11271, #12959, #5861, #12521, #12742, #19802, #21386, #4387, #11161, #16452, #3951, #18140, #19475, #7794, #2485, #2377, #2706, #4064, #16010, #17812, #19370, #587, #9261, #14329, #21162, #21492, #7568, #1360, #15216, #9806, #20028, #13185, #3035, #8124, #16670, #8233, #1134, #1468, #4615, #11490, #18586, #1250, #11384, #6419, #19916, #3148, #15103, #18253, #4504, #2815, #6649, #14989, #9694, #21939, #6531, #21603, #8345, #6195, #10032, #21830, #13289, #16894, #20130, #11600, #22060, #13073, #2920, #8012, #14877, #16555, #21718, #18357, #6310, #4719, #18472, #9921, #16785, #13401, #20245, #4839, #11716, #5206, #6691, #10179, #13444, #18511, #3294, #18945, #11640, #10069, #15138, #1734, #1624, #10400, #22212, #5096, #10293, #1508, #15029, #13564, #3412, #20284, #17260, #18729, #15469, #3185, #16820, #20169, #1833, #8388, #17048, #21979, #20399, #11977, #8502, #20623, #42, #15256, #21869, #22103, #6913, #15366, #13784, #6803, #3520, #13327, #12090, #6573, #17158, #4989, #11759, #6458, #4880, #4763, #18624, #3075, #9961, #16933, #1398, #8271, #13670, #11864, #20505, #18838, #8608, #12307, #20842, #15913, #382, #8937, #14234, #1948, #5760, #19163, #5425, #16023, #15804, #5314, #5546, #13898, #599, #12533, #12196, #20734, #19052, #17825, #7250, #3627, #5656, #3962, #8710, #21173, #15577, #9161, #14121, #20957, #7471, #12424, #19276, #14340, #12640, #8827, #156, #7025, #10837, #21068, #10507, #19381, #3738, #19489, #492, #3854, #4077, #10952, #17373, #17711, #15693, #10734, #270, #2059, #7140, #17599, #14006, #17492, #2278, #10622, #7365, #2166, #9046, #11283, #20040, #9601, #14775, #19929, #11171, #2387, #16351, #13084, #7693, #4627, #6094, #2827, #12863, #4188, #7579, #11501, #18039, #12969, #9376, #926, #21615, #19814, #8024, #9707, #2608, #9272, #9489, #16567, #4399, #1147, #18153, #6321, #703, #14890, #2496, #4515, #7805, #21397, #21730, #16236, #14445, #813, #13195, #16130, #14562, #21280, #5874, #2718, #12753, #7912, #19601, #14670, #5989, #19707, #16463, #21504 ),
 ( #11064, #1038, #6207, #17934, #11395, #18263, #4292, #13646, #15341, #1483, #20596, #1371, #18485, #8247, #15448, #1710, #10269, #10155, #5183, #1261, #16907, #11612, #3270, #10046, #6665, #6888, #18815, #13417, #8136, #1600, #16796, #3047, #15115, #18370, #9934, #11842, #22076, #6777, #21953, #2931, #13758, #18707, #8585, #17024, #9819, #6545, #13536, #8478, #17135, #18, #15002, #16682, #20373, #22189, #21840, #6432, #3387, #13301, #20258, #20482, #20142, #4735, #4854, #11731, #4965, #5073, #18599, #3162, #8360, #15230, #11951, #3831, #1926, #21151, #15669, #19135, #10713, #8806, #17578, #19028, #12066, #2255, #19252, #7450, #12284, #7117, #17686, #575, #9137, #248, #19360, #12400, #2039, #17238, #15999, #14318, #10482, #10817, #13983, #18923, #3605, #3498, #10598, #2145, #15783, #10375, #1809, #8686, #15552, #132, #14096, #7001, #20821, #9025, #13873, #20712, #15888, #5293, #5399, #17468, #8916, #14210, #12173, #17347, #3716, #7229, #5635, #361, #20934, #466, #5522, #7343, #21045, #12511, #3941, #789, #7668, #14538, #682, #21480, #19904, #11150, #21374, #7556, #2583, #5966, #9683, #1013, #2695, #18016, #7998, #11043, #5849, #17909, #2803, #11373, #4493, #19791, #14863, #10928, #4271, #21258, #12946, #19685, #16325, #16543, #6182, #12842, #17800, #11258, #4164, #12731, #2474, #5739, #19576, #6073, #9465, #16440, #9355, #12618, #1121, #4374, #18241, #18127, #19463, #16215, #902, #9577, #7889, #4052, #2367, #9249, #16109, #7782, #14750, #14425, #14648, #13059, #21591, #1349, #13507, #11587, #8560, #3022, #6519, #20345, #18459, #4941, #6408, #21705, #11924, #6637, #17107, #21929, #16771, #5048, #10241, #18792, #9909, #6753, #22047, #11703, #4603, #3359, #1687, #20120, #20459, #8221, #6297, #13278, #13171, #20232, #11817, #3137, #20016, #11478, #18345, #2907, #9792, #1457, #16656, #15092, #18683, #1238, #8112, #3245, #14978, #13388, #4826, #18575, #1576, #21818, #4708, #10019, #16882, #15318, #8331, #15202, #10129, #16996, #8448, #22165, #13623, #20908, #10460, #17322, #1900, #10352, #8893, #7316, #20797, #8782, #17215, #12259, #15643, #19337, #10690, #12376, #5376, #17660, #20688, #15526, #5268, #12490, #21022, #14185, #7204, #2229, #20571, #13959, #8664, #337, #7093, #3689, #3917, #15863, #224, #5158, #5495, #13849, #109, #12148, #15425, #6978, #15758, #19111, #3807, #19006, #8882, #10794, #14071, #5611, #19227, #6863, #3583, #10573, #17442, #13731, #17554, #2122, #2012, #12039, #9000, #441, #18899, #3473, #1788, #988, #877, #11344, #14296, #7640, #2340, #16301, #764, #19660 ),
 ( #21565, #18215, #6046, #4464, #14513, #10901, #2449, #21129, #21345, #7863, #17886, #12921, #6154, #7753, #14624, #9439, #13030, #5938, #4245, #7534, #12594, #11125, #19878, #5716, #4140, #9226, #18102, #17993, #9111, #21457, #19767, #4347, #9332, #15975, #12817, #11231, #14403, #549, #2556, #9552, #19551, #17776, #19439, #7428, #16192, #2669, #16087, #16414, #14728, #4025, #657, #21234, #5826, #12705, #11019, #17264, #20204, #1836, #6491, #7028, #1095, #8714, #2882, #13479, #8195, #21793, #15581, #16628, #7968, #9763, #159, #13902, #8087, #20737, #21679, #18547, #16517, #8305, #5318, #18431, #6379, #14954, #9994, #16744, #2996, #15172, #18321, #12199, #13251, #20096, #10403, #9880, #6270, #21903, #14835, #2775, #6610, #13145, #19990, #9657, #1324, #4577, #15063, #11453, #4800, #1212, #13360, #4684, #11558, #11676, #3114, #20318, #16856, #1432, #22015, #4916, #11792, #18659, #3219, #10954, #2062, #706, #15696, #12536, #10511, #2280, #14448, #12426, #384, #8942, #3965, #10737, #19279, #9163, #12312, #16133, #7252, #15807, #4079, #3856, #274, #15916, #1952, #17827, #601, #7144, #8830, #14009, #5877, #17602, #20846, #16026, #14344, #19055, #9274, #3631, #19492, #2169, #9048, #2390, #494, #7368, #7581, #21283, #19166, #17376, #5428, #21177, #7473, #3741, #5763, #14124, #10626, #10840, #14236, #17495, #20960, #5548, #12644, #21070, #5659, #19383, #17714, #17937, #11285, #4629, #21507, #9709, #9823, #4517, #11397, #13086, #2934, #4403, #7914, #11173, #16238, #1040, #16684, #9379, #7807, #12865, #21732, #21618, #8139, #19931, #2829, #8027, #6097, #12755, #18155, #1151, #18042, #15004, #16465, #13197, #816, #6323, #7695, #20042, #18265, #2720, #2498, #1263, #21842, #2611, #6210, #19603, #16569, #14892, #11504, #12971, #4190, #9603, #18372, #9491, #11067, #14778, #14564, #21399, #5991, #19711, #4294, #19817, #16353, #928, #14672, #3389, #1602, #12068, #13760, #22078, #15554, #6667, #20599, #8480, #5186, #10157, #10377, #4737, #18925, #6547, #17137, #11844, #3164, #3500, #20260, #11615, #13420, #17240, #1811, #11733, #8688, #3049, #22192, #20144, #11953, #6434, #13539, #10048, #18601, #13648, #20375, #4967, #18817, #21955, #13303, #16909, #1485, #18488, #18709, #9936, #3272, #16798, #1373, #10271, #8249, #15117, #4857, #8362, #17027, #15233, #1712, #8588, #15343, #6779, #20484, #6890, #5075, #15450, #20, #12402, #10715, #14320, #12620, #251, #7003, #20714, #2257, #5637, #12176, #12513, #17470, #4054, #7345, #19254, #17802, #19465, #2369, #19362, #9251, #5524, #1928, #15785, #5295, #20936 ),
 ( #468, #135, #10930, #7452, #19030, #2041, #14212, #12286, #13876, #3607, #577, #8919, #10484, #3943, #20823, #7119, #19137, #17349, #13985, #15890, #3833, #10819, #5401, #8808, #15671, #21047, #5741, #17688, #3718, #10601, #17581, #9139, #21153, #363, #7231, #14098, #2147, #16002, #9027, #4605, #1123, #21260, #18018, #7891, #5968, #2909, #19687, #904, #14752, #12844, #21593, #791, #16111, #6300, #1015, #11480, #16327, #11152, #2697, #4166, #2805, #11045, #8000, #16442, #6075, #5851, #20018, #18347, #14540, #14865, #4273, #21707, #7670, #7558, #14650, #6184, #19793, #684, #14427, #12733, #13173, #19578, #18129, #17911, #2585, #13061, #2476, #9357, #19907, #16217, #9467, #21482, #12949, #18243, #21377, #7784, #4376, #11260, #9685, #9579, #4496, #11375, #16545, #15426, #18900, #13391, #15321, #4829, #11706, #18577, #4710, #3247, #1689, #15205, #3139, #11589, #6639, #10022, #13734, #5051, #6755, #22050, #12041, #15094, #9912, #21931, #6864, #6700, #8562, #1578, #9794, #14980, #8334, #3024, #16999, #1459, #20348, #20572, #20234, #6521, #17111, #16884, #6410, #13510, #21820, #5159, #13625, #13280, #20122, #18461, #16658, #4943, #16775, #20461, #11927, #1240, #8115, #1351, #10243, #11819, #18685, #8223, #10132, #8451, #22167, #18794, #3362, #10353, #1789, #5613, #9001, #15528, #15865, #20799, #7429, #10691, #15759, #21130, #15976, #5717, #443, #12596, #8894, #5269, #19113, #8665, #2014, #17661, #12260, #7317, #551, #17555, #2123, #3808, #14297, #17444, #20910, #1901, #6979, #14072, #3475, #111, #5377, #3584, #12491, #12377, #17216, #14187, #21023, #19338, #3690, #13850, #338, #3919, #8784, #20691, #7206, #10795, #12150, #19228, #5497, #2232, #10574, #9112, #10461, #19007, #17324, #15644, #226, #7095, #13960, #6274, #12819, #11349, #14627, #18219, #879, #1099, #17778, #2778, #19554, #7867, #2558, #16194, #9662, #11021, #2342, #4142, #16521, #7974, #2451, #14840, #16089, #12925, #10904, #2673, #21683, #19662, #766, #9334, #4350, #11127, #4248, #9555, #12707, #659, #9229, #7536, #19441, #17995, #14405, #16417, #14731, #4028, #21237, #5829, #19881, #9443, #16304, #17889, #7755, #21459, #7644, #14515, #21347, #5941, #6050, #21570, #993, #19771, #6157, #11235, #18105, #13035, #4468, #8538, #3335, #15402, #10107, #22248, #18551, #14957, #6495, #18325, #11680, #5026, #21907, #16971, #10217, #4920, #11796, #13483, #17086, #4804, #8309, #11562, #16634, #1437, #1663, #9768, #8199, #13255, #22141, #22023, #13148, #20322, #3223, #8426, #13366, #19994, #3118, #1550, #18437, #4580, #16860, #13600 ) ),
 .UNSPECIFIED., .T., .F., .F. ) 
 B_SPLINE_SURFACE_WITH_KNOTS ( ( 4, 3, 4 ),
 ( 4, 2, 2, 2, 2, 2, 2, 2, 2, 2, 2, 2, 2, 2, 2, 2, 2, 2, 2, 2, 2, 2, 2, 2, 2, 2, 2, 2, 2, 2, 2, 2, 2, 2, 2, 2, 2, 2, 2, 2, 2, 2, 2, 2, 2, 2, 2, 2, 2, 2, 2, 2, 2, 2, 2, 2, 2, 2, 2, 2, 2, 2, 2, 2, 2, 2, 2, 2, 2, 2, 2, 2, 2, 2, 2, 2, 2, 2, 2, 2, 2, 2, 2, 2, 2, 2, 2, 2, 2, 2, 2, 2, 2, 2, 2, 2, 2, 2, 2, 2, 2, 2, 2, 2, 2, 2, 2, 2, 2, 2, 2, 2, 2, 2, 2, 2, 2, 2, 2, 2, 2, 2, 2, 2, 2, 2, 2, 2, 2, 2, 2, 2, 2, 2, 2, 2, 2, 2, 2, 2, 2, 2, 2, 2, 2, 2, 2, 2, 2, 2, 2, 2, 2, 2, 2, 2, 2, 2, 2, 2, 2, 2, 2, 2, 2, 2, 2, 4 ),
 ( 0.000000000000000000, 0.5000000000000000000, 1.000000000000000000 ),
 ( 0.000000000000000000, 0.001952908952989333875, 0.003905817905978667751, 0.007323408573709997045, 0.01074099924144132634, 0.01415858990917265650, 0.01586738524303832332, 0.01757618057690398666, 0.02099377124463531682, 0.02441136191236664699, 0.02782895258009797368, 0.03124654324782930384, 0.03466413391556063400, 0.03808172458329196070, 0.04149931525102329433, 0.04491690591875462102, 0.04662570125262028436, 0.04833449658648594771, 0.05175208725421727440, 0.05346088258808293775, 0.05516967792194860110, 0.05858726858967993473, 0.06200485925741126836, 0.06542244992514259505, 0.06884004059287393562, 0.07225763126060526231, 0.07567522192833658901, 0.07909281259606792958, 0.08251040326379925627, 0.08421919859766491268, 0.08592799393153058296, 0.08934558459926195129, 0.09276317526699331961, 0.09447197060085900377, 0.09618076593472468794, 0.09959835660245604239, 0.1030159472701873968, 0.1064335379379187652, 0.1098511286056501335, 0.1132687192733815018, 0.1166863099411127869, 0.1201039006088440858, 0.1235214912765753847, 0.1252302866104410273, 0.1269390819443066698, 0.1303566726120379826, 0.1320654679459036251, 0.1337742632797692677, 0.1371918539475005527, 0.1406094446152318378, 0.1440270352829631784, 0.1474446259506944912, 0.1508622166184258040, 0.1542798072861571446, 0.1576973979538884851, 0.1611149886216198257, 0.1645325792893511663, 0.1679501699570824791, 0.1713677606248137919, 0.1747853512925451325, 0.1764941466264108028, 0.1782029419602764730, 0.1816205326280078136, 0.1850381232957391542, 0.1884557139634704670, 0.1918733046312017798, 0.1952908952989331204, 0.1987084859666644610, 0.2021260766343957738, 0.2055436673021270866, 0.2072524626359927569, 0.2089612579698584272, 0.2123788486375897677, 0.2140876439714554380, 0.2157964393053211083, 0.2192140299730524489, 0.2226316206407837617, 0.2260492113085151300, 0.2294668019762464706, 0.2328843926439778111, 0.2363019833117091517, 0.2397195739794404923, 0.2431371646471718329, 0.2465547553149031734, 0.2499723459826345140, 0.2533899366503657991, 0.2568075273180971396, 0.2602251179858284802, 0.2636427086535597653, 0.2670602993212910503, 0.2704778899890223909, 0.2738954806567537315, 0.2773130713244850165, 0.2807306619922163571, 0.2841482526599476977, 0.2858570479938133957, 0.2875658433276790382, 0.2909834339954103788, 0.2926922293292760768, 0.2944010246631417194, 0.2978186153308730599, 0.3012362059986043450, 0.3046537966663356856, 0.3080713873340670261, 0.3114889780017983112, 0.3149065686695296518, 0.3183241593372609923, 0.3217417500049923329, 0.3234505453388579754, 0.3251593406727236735, 0.3285769313404549585, 0.3319945220081862991, 0.3354121126759176397, 0.3388297033436489247, 0.3422472940113802653, 0.3456648846791116059, 0.3490824753468429464, 0.3525000660145742870, 0.3559176566823056276, 0.3593352473500369682, 0.3627528380177683087, 0.3661704286854996493, 0.3695880193532309343, 0.3730056100209622749, 0.3747144053548279174, 0.3764232006886936155, 0.3798407913564249005, 0.3832583820241562411, 0.3866759726918875817, 0.3900935633596189223, 0.3935111540273502628, 0.3969287446950816034, 0.4003463353628129440, 0.4037639260305442845, 0.4054727213644099271, 0.4071815166982756251, 0.4105991073660069102, 0.4140166980337382507, 0.4157254933676038933, 0.4174342887014695913, 0.4208518793692008764, 0.4242694700369322169, 0.4276870607046635575, 0.4311046513723948981, 0.4345222420401262386, 0.4379398327078575237, 0.4413574233755888643, 0.4447750140433202048, 0.4464838093771859029, 0.4481926047110515454, 0.4516101953787828860, 0.4533189907126485840, 0.4550277860465142266, 0.4584453767142455671, 0.4618629673819769077, 0.4652805580497082483, 0.4686981487174395888, 0.4721157393851709294, 0.4755333300529022145, 0.4789509207206335550, 0.4823685113883648956, 0.4840773067222305381, 0.4857861020560961807, 0.4892036927238275212, 0.4926212833915588618, 0.4960388740592901469, 0.4979917830122794764, 0.4999446919652688059 ),
 .UNSPECIFIED. ) 
 GEOMETRIC_REPRESENTATION_ITEM ( )  RATIONAL_B_SPLINE_SURFACE ( (
 ( 1.000000000000000000, 1.000000000000000000, 1.000000000000000000, 1.000000000000000000, 1.000000000000000000, 1.000000000000000000, 1.000000000000000000, 1.000000000000000000, 1.000000000000000000, 1.000000000000000000, 1.000000000000000000, 1.000000000000000000, 1.000000000000000000, 1.000000000000000000, 1.000000000000000000, 1.000000000000000000, 1.000000000000000000, 1.000000000000000000, 1.000000000000000000, 1.000000000000000000, 1.000000000000000000, 1.000000000000000000, 1.000000000000000000, 1.000000000000000000, 1.000000000000000000, 1.000000000000000000, 1.000000000000000000, 1.000000000000000000, 1.000000000000000000, 1.000000000000000000, 1.000000000000000000, 1.000000000000000000, 1.000000000000000000, 1.000000000000000000, 1.000000000000000000, 1.000000000000000000, 1.000000000000000000, 1.000000000000000000, 1.000000000000000000, 1.000000000000000000, 1.000000000000000000, 1.000000000000000000, 1.000000000000000000, 1.000000000000000000, 1.000000000000000000, 1.000000000000000000, 1.000000000000000000, 1.000000000000000000, 1.000000000000000000, 1.000000000000000000, 1.000000000000000000, 1.000000000000000000, 1.000000000000000000, 1.000000000000000000, 1.000000000000000000, 1.000000000000000000, 1.000000000000000000, 1.000000000000000000, 1.000000000000000000, 1.000000000000000000, 1.000000000000000000, 1.000000000000000000, 1.000000000000000000, 1.000000000000000000, 1.000000000000000000, 1.000000000000000000, 1.000000000000000000, 1.000000000000000000, 1.000000000000000000, 1.000000000000000000, 1.000000000000000000, 1.000000000000000000, 1.000000000000000000, 1.000000000000000000, 1.000000000000000000, 1.000000000000000000, 1.000000000000000000, 1.000000000000000000, 1.000000000000000000, 1.000000000000000000, 1.000000000000000000, 1.000000000000000000, 1.000000000000000000, 1.000000000000000000, 1.000000000000000000, 1.000000000000000000, 1.000000000000000000, 1.000000000000000000, 1.000000000000000000, 1.000000000000000000, 1.000000000000000000, 1.000000000000000000, 1.000000000000000000, 1.000000000000000000, 1.000000000000000000, 1.000000000000000000, 1.000000000000000000, 1.000000000000000000, 1.000000000000000000, 1.000000000000000000, 1.000000000000000000, 1.000000000000000000, 1.000000000000000000, 1.000000000000000000, 1.000000000000000000, 1.000000000000000000, 1.000000000000000000, 1.000000000000000000, 1.000000000000000000, 1.000000000000000000, 1.000000000000000000, 1.000000000000000000, 1.000000000000000000, 1.000000000000000000, 1.000000000000000000, 1.000000000000000000, 1.000000000000000000, 1.000000000000000000, 1.000000000000000000, 1.000000000000000000, 1.000000000000000000, 1.000000000000000000, 1.000000000000000000, 1.000000000000000000, 1.000000000000000000, 1.000000000000000000, 1.000000000000000000, 1.000000000000000000, 1.000000000000000000, 1.000000000000000000, 1.000000000000000000, 1.000000000000000000, 1.000000000000000000, 1.000000000000000000, 1.000000000000000000, 1.000000000000000000, 1.000000000000000000, 1.000000000000000000, 1.000000000000000000, 1.000000000000000000, 1.000000000000000000, 1.000000000000000000, 1.000000000000000000, 1.000000000000000000, 1.000000000000000000, 1.000000000000000000, 1.000000000000000000, 1.000000000000000000, 1.000000000000000000, 1.000000000000000000, 1.000000000000000000, 1.000000000000000000, 1.000000000000000000, 1.000000000000000000, 1.000000000000000000, 1.000000000000000000, 1.000000000000000000, 1.000000000000000000, 1.000000000000000000, 1.000000000000000000, 1.000000000000000000, 1.000000000000000000, 1.000000000000000000, 1.000000000000000000, 1.000000000000000000, 1.000000000000000000, 1.000000000000000000, 1.000000000000000000, 1.000000000000000000, 1.000000000000000000, 1.000000000000000000, 1.000000000000000000, 1.000000000000000000, 1.000000000000000000, 1.000000000000000000, 1.000000000000000000, 1.000000000000000000, 1.000000000000000000, 1.000000000000000000, 1.000000000000000000, 1.000000000000000000, 1.000000000000000000, 1.000000000000000000, 1.000000000000000000, 1.000000000000000000, 1.000000000000000000, 1.000000000000000000, 1.000000000000000000, 1.000000000000000000, 1.000000000000000000, 1.000000000000000000, 1.000000000000000000, 1.000000000000000000, 1.000000000000000000, 1.000000000000000000, 1.000000000000000000, 1.000000000000000000, 1.000000000000000000, 1.000000000000000000, 1.000000000000000000, 1.000000000000000000, 1.000000000000000000, 1.000000000000000000, 1.000000000000000000, 1.000000000000000000, 1.000000000000000000, 1.000000000000000000, 1.000000000000000000, 1.000000000000000000, 1.000000000000000000, 1.000000000000000000, 1.000000000000000000, 1.000000000000000000, 1.000000000000000000, 1.000000000000000000, 1.000000000000000000, 1.000000000000000000, 1.000000000000000000, 1.000000000000000000, 1.000000000000000000, 1.000000000000000000, 1.000000000000000000, 1.000000000000000000, 1.000000000000000000, 1.000000000000000000, 1.000000000000000000, 1.000000000000000000, 1.000000000000000000, 1.000000000000000000, 1.000000000000000000, 1.000000000000000000, 1.000000000000000000, 1.000000000000000000, 1.000000000000000000, 1.000000000000000000, 1.000000000000000000, 1.000000000000000000, 1.000000000000000000, 1.000000000000000000, 1.000000000000000000, 1.000000000000000000, 1.000000000000000000, 1.000000000000000000, 1.000000000000000000, 1.000000000000000000, 1.000000000000000000, 1.000000000000000000, 1.000000000000000000, 1.000000000000000000, 1.000000000000000000, 1.000000000000000000, 1.000000000000000000, 1.000000000000000000, 1.000000000000000000, 1.000000000000000000, 1.000000000000000000, 1.000000000000000000, 1.000000000000000000, 1.000000000000000000, 1.000000000000000000, 1.000000000000000000, 1.000000000000000000, 1.000000000000000000, 1.000000000000000000, 1.000000000000000000, 1.000000000000000000, 1.000000000000000000, 1.000000000000000000, 1.000000000000000000, 1.000000000000000000, 1.000000000000000000, 1.000000000000000000, 1.000000000000000000, 1.000000000000000000, 1.000000000000000000, 1.000000000000000000, 1.000000000000000000, 1.000000000000000000, 1.000000000000000000, 1.000000000000000000, 1.000000000000000000, 1.000000000000000000, 1.000000000000000000, 1.000000000000000000, 1.000000000000000000, 1.000000000000000000, 1.000000000000000000, 1.000000000000000000, 1.000000000000000000, 1.000000000000000000, 1.000000000000000000, 1.000000000000000000, 1.000000000000000000, 1.000000000000000000, 1.000000000000000000, 1.000000000000000000, 1.000000000000000000, 1.000000000000000000, 1.000000000000000000, 1.000000000000000000, 1.000000000000000000, 1.000000000000000000, 1.000000000000000000, 1.000000000000000000, 1.000000000000000000, 1.000000000000000000, 1.000000000000000000, 1.000000000000000000, 1.000000000000000000, 1.000000000000000000, 1.000000000000000000, 1.000000000000000000, 1.000000000000000000, 1.000000000000000000, 1.000000000000000000, 1.000000000000000000, 1.000000000000000000, 1.000000000000000000, 1.000000000000000000, 1.000000000000000000, 1.000000000000000000, 1.000000000000000000, 1.000000000000000000, 1.000000000000000000, 1.000000000000000000, 1.000000000000000000, 1.000000000000000000, 1.000000000000000000, 1.000000000000000000, 1.000000000000000000, 1.000000000000000000, 1.000000000000000000, 1.000000000000000000, 1.000000000000000000, 1.000000000000000000, 1.000000000000000000),
 ( 0.3333333333333333703, 0.3333333333333333703, 0.3333333333333333703, 0.3333333333333333703, 0.3333333333333333703, 0.3333333333333333703, 0.3333333333333333703, 0.3333333333333333703, 0.3333333333333333703, 0.3333333333333333703, 0.3333333333333333703, 0.3333333333333333703, 0.3333333333333333703, 0.3333333333333333703, 0.3333333333333333703, 0.3333333333333333703, 0.3333333333333333703, 0.3333333333333333703, 0.3333333333333333703, 0.3333333333333333703, 0.3333333333333333703, 0.3333333333333333703, 0.3333333333333333703, 0.3333333333333333703, 0.3333333333333333703, 0.3333333333333333703, 0.3333333333333333703, 0.3333333333333333703, 0.3333333333333333703, 0.3333333333333333703, 0.3333333333333333703, 0.3333333333333333703, 0.3333333333333333703, 0.3333333333333333703, 0.3333333333333333703, 0.3333333333333333703, 0.3333333333333333703, 0.3333333333333333703, 0.3333333333333333703, 0.3333333333333333703, 0.3333333333333333703, 0.3333333333333333703, 0.3333333333333333703, 0.3333333333333333703, 0.3333333333333333703, 0.3333333333333333703, 0.3333333333333333703, 0.3333333333333333703, 0.3333333333333333703, 0.3333333333333333703, 0.3333333333333333703, 0.3333333333333333703, 0.3333333333333333703, 0.3333333333333333703, 0.3333333333333333703, 0.3333333333333333703, 0.3333333333333333703, 0.3333333333333333703, 0.3333333333333333703, 0.3333333333333333703, 0.3333333333333333703, 0.3333333333333333703, 0.3333333333333333703, 0.3333333333333333703, 0.3333333333333333703, 0.3333333333333333703, 0.3333333333333333703, 0.3333333333333333703, 0.3333333333333333703, 0.3333333333333333703, 0.3333333333333333703, 0.3333333333333333703, 0.3333333333333333703, 0.3333333333333333703, 0.3333333333333333703, 0.3333333333333333703, 0.3333333333333333703, 0.3333333333333333703, 0.3333333333333333703, 0.3333333333333333703, 0.3333333333333333703, 0.3333333333333333703, 0.3333333333333333703, 0.3333333333333333703, 0.3333333333333333703, 0.3333333333333333703, 0.3333333333333333703, 0.3333333333333333703, 0.3333333333333333703, 0.3333333333333333703, 0.3333333333333333703, 0.3333333333333333703, 0.3333333333333333703, 0.3333333333333333703, 0.3333333333333333703, 0.3333333333333333703, 0.3333333333333333703, 0.3333333333333333703, 0.3333333333333333703, 0.3333333333333333703, 0.3333333333333333703, 0.3333333333333333703, 0.3333333333333333703, 0.3333333333333333703, 0.3333333333333333703, 0.3333333333333333703, 0.3333333333333333703, 0.3333333333333333703, 0.3333333333333333703, 0.3333333333333333703, 0.3333333333333333703, 0.3333333333333333703, 0.3333333333333333703, 0.3333333333333333703, 0.3333333333333333703, 0.3333333333333333703, 0.3333333333333333703, 0.3333333333333333703, 0.3333333333333333703, 0.3333333333333333703, 0.3333333333333333703, 0.3333333333333333703, 0.3333333333333333703, 0.3333333333333333703, 0.3333333333333333703, 0.3333333333333333703, 0.3333333333333333703, 0.3333333333333333703, 0.3333333333333333703, 0.3333333333333333703, 0.3333333333333333703, 0.3333333333333333703, 0.3333333333333333703, 0.3333333333333333703, 0.3333333333333333703, 0.3333333333333333703, 0.3333333333333333703, 0.3333333333333333703, 0.3333333333333333703, 0.3333333333333333703, 0.3333333333333333703, 0.3333333333333333703, 0.3333333333333333703, 0.3333333333333333703, 0.3333333333333333703, 0.3333333333333333703, 0.3333333333333333703, 0.3333333333333333703, 0.3333333333333333703, 0.3333333333333333703, 0.3333333333333333703, 0.3333333333333333703, 0.3333333333333333703, 0.3333333333333333703, 0.3333333333333333703, 0.3333333333333333703, 0.3333333333333333703, 0.3333333333333333703, 0.3333333333333333703, 0.3333333333333333703, 0.3333333333333333703, 0.3333333333333333703, 0.3333333333333333703, 0.3333333333333333703, 0.3333333333333333703, 0.3333333333333333703, 0.3333333333333333703, 0.3333333333333333703, 0.3333333333333333703, 0.3333333333333333703, 0.3333333333333333703, 0.3333333333333333703, 0.3333333333333333703, 0.3333333333333333703, 0.3333333333333333703, 0.3333333333333333703, 0.3333333333333333703, 0.3333333333333333703, 0.3333333333333333703, 0.3333333333333333703, 0.3333333333333333703, 0.3333333333333333703, 0.3333333333333333703, 0.3333333333333333703, 0.3333333333333333703, 0.3333333333333333703, 0.3333333333333333703, 0.3333333333333333703, 0.3333333333333333703, 0.3333333333333333703, 0.3333333333333333703, 0.3333333333333333703, 0.3333333333333333703, 0.3333333333333333703, 0.3333333333333333703, 0.3333333333333333703, 0.3333333333333333703, 0.3333333333333333703, 0.3333333333333333703, 0.3333333333333333703, 0.3333333333333333703, 0.3333333333333333703, 0.3333333333333333703, 0.3333333333333333703, 0.3333333333333333703, 0.3333333333333333703, 0.3333333333333333703, 0.3333333333333333703, 0.3333333333333333703, 0.3333333333333333703, 0.3333333333333333703, 0.3333333333333333703, 0.3333333333333333703, 0.3333333333333333703, 0.3333333333333333703, 0.3333333333333333703, 0.3333333333333333703, 0.3333333333333333703, 0.3333333333333333703, 0.3333333333333333703, 0.3333333333333333703, 0.3333333333333333703, 0.3333333333333333703, 0.3333333333333333703, 0.3333333333333333703, 0.3333333333333333703, 0.3333333333333333703, 0.3333333333333333703, 0.3333333333333333703, 0.3333333333333333703, 0.3333333333333333703, 0.3333333333333333703, 0.3333333333333333703, 0.3333333333333333703, 0.3333333333333333703, 0.3333333333333333703, 0.3333333333333333703, 0.3333333333333333703, 0.3333333333333333703, 0.3333333333333333703, 0.3333333333333333703, 0.3333333333333333703, 0.3333333333333333703, 0.3333333333333333703, 0.3333333333333333703, 0.3333333333333333703, 0.3333333333333333703, 0.3333333333333333703, 0.3333333333333333703, 0.3333333333333333703, 0.3333333333333333703, 0.3333333333333333703, 0.3333333333333333703, 0.3333333333333333703, 0.3333333333333333703, 0.3333333333333333703, 0.3333333333333333703, 0.3333333333333333703, 0.3333333333333333703, 0.3333333333333333703, 0.3333333333333333703, 0.3333333333333333703, 0.3333333333333333703, 0.3333333333333333703, 0.3333333333333333703, 0.3333333333333333703, 0.3333333333333333703, 0.3333333333333333703, 0.3333333333333333703, 0.3333333333333333703, 0.3333333333333333703, 0.3333333333333333703, 0.3333333333333333703, 0.3333333333333333703, 0.3333333333333333703, 0.3333333333333333703, 0.3333333333333333703, 0.3333333333333333703, 0.3333333333333333703, 0.3333333333333333703, 0.3333333333333333703, 0.3333333333333333703, 0.3333333333333333703, 0.3333333333333333703, 0.3333333333333333703, 0.3333333333333333703, 0.3333333333333333703, 0.3333333333333333703, 0.3333333333333333703, 0.3333333333333333703, 0.3333333333333333703, 0.3333333333333333703, 0.3333333333333333703, 0.3333333333333333703, 0.3333333333333333703, 0.3333333333333333703, 0.3333333333333333703, 0.3333333333333333703, 0.3333333333333333703, 0.3333333333333333703, 0.3333333333333333703, 0.3333333333333333703, 0.3333333333333333703, 0.3333333333333333703, 0.3333333333333333703, 0.3333333333333333703, 0.3333333333333333703, 0.3333333333333333703, 0.3333333333333333703, 0.3333333333333333703, 0.3333333333333333703, 0.3333333333333333703, 0.3333333333333333703, 0.3333333333333333703, 0.3333333333333333703, 0.3333333333333333703, 0.3333333333333333703, 0.3333333333333333703, 0.3333333333333333703, 0.3333333333333333703, 0.3333333333333333703, 0.3333333333333333703, 0.3333333333333333703, 0.3333333333333333703, 0.3333333333333333703, 0.3333333333333333703, 0.3333333333333333703, 0.3333333333333333703, 0.3333333333333333703, 0.3333333333333333703, 0.3333333333333333703, 0.3333333333333333703, 0.3333333333333333703, 0.3333333333333333703, 0.3333333333333333703, 0.3333333333333333703),
 ( 0.3333333333333333703, 0.3333333333333333703, 0.3333333333333333703, 0.3333333333333333703, 0.3333333333333333703, 0.3333333333333333703, 0.3333333333333333703, 0.3333333333333333703, 0.3333333333333333703, 0.3333333333333333703, 0.3333333333333333703, 0.3333333333333333703, 0.3333333333333333703, 0.3333333333333333703, 0.3333333333333333703, 0.3333333333333333703, 0.3333333333333333703, 0.3333333333333333703, 0.3333333333333333703, 0.3333333333333333703, 0.3333333333333333703, 0.3333333333333333703, 0.3333333333333333703, 0.3333333333333333703, 0.3333333333333333703, 0.3333333333333333703, 0.3333333333333333703, 0.3333333333333333703, 0.3333333333333333703, 0.3333333333333333703, 0.3333333333333333703, 0.3333333333333333703, 0.3333333333333333703, 0.3333333333333333703, 0.3333333333333333703, 0.3333333333333333703, 0.3333333333333333703, 0.3333333333333333703, 0.3333333333333333703, 0.3333333333333333703, 0.3333333333333333703, 0.3333333333333333703, 0.3333333333333333703, 0.3333333333333333703, 0.3333333333333333703, 0.3333333333333333703, 0.3333333333333333703, 0.3333333333333333703, 0.3333333333333333703, 0.3333333333333333703, 0.3333333333333333703, 0.3333333333333333703, 0.3333333333333333703, 0.3333333333333333703, 0.3333333333333333703, 0.3333333333333333703, 0.3333333333333333703, 0.3333333333333333703, 0.3333333333333333703, 0.3333333333333333703, 0.3333333333333333703, 0.3333333333333333703, 0.3333333333333333703, 0.3333333333333333703, 0.3333333333333333703, 0.3333333333333333703, 0.3333333333333333703, 0.3333333333333333703, 0.3333333333333333703, 0.3333333333333333703, 0.3333333333333333703, 0.3333333333333333703, 0.3333333333333333703, 0.3333333333333333703, 0.3333333333333333703, 0.3333333333333333703, 0.3333333333333333703, 0.3333333333333333703, 0.3333333333333333703, 0.3333333333333333703, 0.3333333333333333703, 0.3333333333333333703, 0.3333333333333333703, 0.3333333333333333703, 0.3333333333333333703, 0.3333333333333333703, 0.3333333333333333703, 0.3333333333333333703, 0.3333333333333333703, 0.3333333333333333703, 0.3333333333333333703, 0.3333333333333333703, 0.3333333333333333703, 0.3333333333333333703, 0.3333333333333333703, 0.3333333333333333703, 0.3333333333333333703, 0.3333333333333333703, 0.3333333333333333703, 0.3333333333333333703, 0.3333333333333333703, 0.3333333333333333703, 0.3333333333333333703, 0.3333333333333333703, 0.3333333333333333703, 0.3333333333333333703, 0.3333333333333333703, 0.3333333333333333703, 0.3333333333333333703, 0.3333333333333333703, 0.3333333333333333703, 0.3333333333333333703, 0.3333333333333333703, 0.3333333333333333703, 0.3333333333333333703, 0.3333333333333333703, 0.3333333333333333703, 0.3333333333333333703, 0.3333333333333333703, 0.3333333333333333703, 0.3333333333333333703, 0.3333333333333333703, 0.3333333333333333703, 0.3333333333333333703, 0.3333333333333333703, 0.3333333333333333703, 0.3333333333333333703, 0.3333333333333333703, 0.3333333333333333703, 0.3333333333333333703, 0.3333333333333333703, 0.3333333333333333703, 0.3333333333333333703, 0.3333333333333333703, 0.3333333333333333703, 0.3333333333333333703, 0.3333333333333333703, 0.3333333333333333703, 0.3333333333333333703, 0.3333333333333333703, 0.3333333333333333703, 0.3333333333333333703, 0.3333333333333333703, 0.3333333333333333703, 0.3333333333333333703, 0.3333333333333333703, 0.3333333333333333703, 0.3333333333333333703, 0.3333333333333333703, 0.3333333333333333703, 0.3333333333333333703, 0.3333333333333333703, 0.3333333333333333703, 0.3333333333333333703, 0.3333333333333333703, 0.3333333333333333703, 0.3333333333333333703, 0.3333333333333333703, 0.3333333333333333703, 0.3333333333333333703, 0.3333333333333333703, 0.3333333333333333703, 0.3333333333333333703, 0.3333333333333333703, 0.3333333333333333703, 0.3333333333333333703, 0.3333333333333333703, 0.3333333333333333703, 0.3333333333333333703, 0.3333333333333333703, 0.3333333333333333703, 0.3333333333333333703, 0.3333333333333333703, 0.3333333333333333703, 0.3333333333333333703, 0.3333333333333333703, 0.3333333333333333703, 0.3333333333333333703, 0.3333333333333333703, 0.3333333333333333703, 0.3333333333333333703, 0.3333333333333333703, 0.3333333333333333703, 0.3333333333333333703, 0.3333333333333333703, 0.3333333333333333703, 0.3333333333333333703, 0.3333333333333333703, 0.3333333333333333703, 0.3333333333333333703, 0.3333333333333333703, 0.3333333333333333703, 0.3333333333333333703, 0.3333333333333333703, 0.3333333333333333703, 0.3333333333333333703, 0.3333333333333333703, 0.3333333333333333703, 0.3333333333333333703, 0.3333333333333333703, 0.3333333333333333703, 0.3333333333333333703, 0.3333333333333333703, 0.3333333333333333703, 0.3333333333333333703, 0.3333333333333333703, 0.3333333333333333703, 0.3333333333333333703, 0.3333333333333333703, 0.3333333333333333703, 0.3333333333333333703, 0.3333333333333333703, 0.3333333333333333703, 0.3333333333333333703, 0.3333333333333333703, 0.3333333333333333703, 0.3333333333333333703, 0.3333333333333333703, 0.3333333333333333703, 0.3333333333333333703, 0.3333333333333333703, 0.3333333333333333703, 0.3333333333333333703, 0.3333333333333333703, 0.3333333333333333703, 0.3333333333333333703, 0.3333333333333333703, 0.3333333333333333703, 0.3333333333333333703, 0.3333333333333333703, 0.3333333333333333703, 0.3333333333333333703, 0.3333333333333333703, 0.3333333333333333703, 0.3333333333333333703, 0.3333333333333333703, 0.3333333333333333703, 0.3333333333333333703, 0.3333333333333333703, 0.3333333333333333703, 0.3333333333333333703, 0.3333333333333333703, 0.3333333333333333703, 0.3333333333333333703, 0.3333333333333333703, 0.3333333333333333703, 0.3333333333333333703, 0.3333333333333333703, 0.3333333333333333703, 0.3333333333333333703, 0.3333333333333333703, 0.3333333333333333703, 0.3333333333333333703, 0.3333333333333333703, 0.3333333333333333703, 0.3333333333333333703, 0.3333333333333333703, 0.3333333333333333703, 0.3333333333333333703, 0.3333333333333333703, 0.3333333333333333703, 0.3333333333333333703, 0.3333333333333333703, 0.3333333333333333703, 0.3333333333333333703, 0.3333333333333333703, 0.3333333333333333703, 0.3333333333333333703, 0.3333333333333333703, 0.3333333333333333703, 0.3333333333333333703, 0.3333333333333333703, 0.3333333333333333703, 0.3333333333333333703, 0.3333333333333333703, 0.3333333333333333703, 0.3333333333333333703, 0.3333333333333333703, 0.3333333333333333703, 0.3333333333333333703, 0.3333333333333333703, 0.3333333333333333703, 0.3333333333333333703, 0.3333333333333333703, 0.3333333333333333703, 0.3333333333333333703, 0.3333333333333333703, 0.3333333333333333703, 0.3333333333333333703, 0.3333333333333333703, 0.3333333333333333703, 0.3333333333333333703, 0.3333333333333333703, 0.3333333333333333703, 0.3333333333333333703, 0.3333333333333333703, 0.3333333333333333703, 0.3333333333333333703, 0.3333333333333333703, 0.3333333333333333703, 0.3333333333333333703, 0.3333333333333333703, 0.3333333333333333703, 0.3333333333333333703, 0.3333333333333333703, 0.3333333333333333703, 0.3333333333333333703, 0.3333333333333333703, 0.3333333333333333703, 0.3333333333333333703, 0.3333333333333333703, 0.3333333333333333703, 0.3333333333333333703, 0.3333333333333333703, 0.3333333333333333703, 0.3333333333333333703, 0.3333333333333333703, 0.3333333333333333703, 0.3333333333333333703, 0.3333333333333333703, 0.3333333333333333703, 0.3333333333333333703, 0.3333333333333333703, 0.3333333333333333703, 0.3333333333333333703, 0.3333333333333333703, 0.3333333333333333703, 0.3333333333333333703, 0.3333333333333333703, 0.3333333333333333703, 0.3333333333333333703, 0.3333333333333333703, 0.3333333333333333703, 0.3333333333333333703, 0.3333333333333333703, 0.3333333333333333703),
 ( 1.000000000000000000, 1.000000000000000000, 1.000000000000000000, 1.000000000000000000, 1.000000000000000000, 1.000000000000000000, 1.000000000000000000, 1.000000000000000000, 1.000000000000000000, 1.000000000000000000, 1.000000000000000000, 1.000000000000000000, 1.000000000000000000, 1.000000000000000000, 1.000000000000000000, 1.000000000000000000, 1.000000000000000000, 1.000000000000000000, 1.000000000000000000, 1.000000000000000000, 1.000000000000000000, 1.000000000000000000, 1.000000000000000000, 1.000000000000000000, 1.000000000000000000, 1.000000000000000000, 1.000000000000000000, 1.000000000000000000, 1.000000000000000000, 1.000000000000000000, 1.000000000000000000, 1.000000000000000000, 1.000000000000000000, 1.000000000000000000, 1.000000000000000000, 1.000000000000000000, 1.000000000000000000, 1.000000000000000000, 1.000000000000000000, 1.000000000000000000, 1.000000000000000000, 1.000000000000000000, 1.000000000000000000, 1.000000000000000000, 1.000000000000000000, 1.000000000000000000, 1.000000000000000000, 1.000000000000000000, 1.000000000000000000, 1.000000000000000000, 1.000000000000000000, 1.000000000000000000, 1.000000000000000000, 1.000000000000000000, 1.000000000000000000, 1.000000000000000000, 1.000000000000000000, 1.000000000000000000, 1.000000000000000000, 1.000000000000000000, 1.000000000000000000, 1.000000000000000000, 1.000000000000000000, 1.000000000000000000, 1.000000000000000000, 1.000000000000000000, 1.000000000000000000, 1.000000000000000000, 1.000000000000000000, 1.000000000000000000, 1.000000000000000000, 1.000000000000000000, 1.000000000000000000, 1.000000000000000000, 1.000000000000000000, 1.000000000000000000, 1.000000000000000000, 1.000000000000000000, 1.000000000000000000, 1.000000000000000000, 1.000000000000000000, 1.000000000000000000, 1.000000000000000000, 1.000000000000000000, 1.000000000000000000, 1.000000000000000000, 1.000000000000000000, 1.000000000000000000, 1.000000000000000000, 1.000000000000000000, 1.000000000000000000, 1.000000000000000000, 1.000000000000000000, 1.000000000000000000, 1.000000000000000000, 1.000000000000000000, 1.000000000000000000, 1.000000000000000000, 1.000000000000000000, 1.000000000000000000, 1.000000000000000000, 1.000000000000000000, 1.000000000000000000, 1.000000000000000000, 1.000000000000000000, 1.000000000000000000, 1.000000000000000000, 1.000000000000000000, 1.000000000000000000, 1.000000000000000000, 1.000000000000000000, 1.000000000000000000, 1.000000000000000000, 1.000000000000000000, 1.000000000000000000, 1.000000000000000000, 1.000000000000000000, 1.000000000000000000, 1.000000000000000000, 1.000000000000000000, 1.000000000000000000, 1.000000000000000000, 1.000000000000000000, 1.000000000000000000, 1.000000000000000000, 1.000000000000000000, 1.000000000000000000, 1.000000000000000000, 1.000000000000000000, 1.000000000000000000, 1.000000000000000000, 1.000000000000000000, 1.000000000000000000, 1.000000000000000000, 1.000000000000000000, 1.000000000000000000, 1.000000000000000000, 1.000000000000000000, 1.000000000000000000, 1.000000000000000000, 1.000000000000000000, 1.000000000000000000, 1.000000000000000000, 1.000000000000000000, 1.000000000000000000, 1.000000000000000000, 1.000000000000000000, 1.000000000000000000, 1.000000000000000000, 1.000000000000000000, 1.000000000000000000, 1.000000000000000000, 1.000000000000000000, 1.000000000000000000, 1.000000000000000000, 1.000000000000000000, 1.000000000000000000, 1.000000000000000000, 1.000000000000000000, 1.000000000000000000, 1.000000000000000000, 1.000000000000000000, 1.000000000000000000, 1.000000000000000000, 1.000000000000000000, 1.000000000000000000, 1.000000000000000000, 1.000000000000000000, 1.000000000000000000, 1.000000000000000000, 1.000000000000000000, 1.000000000000000000, 1.000000000000000000, 1.000000000000000000, 1.000000000000000000, 1.000000000000000000, 1.000000000000000000, 1.000000000000000000, 1.000000000000000000, 1.000000000000000000, 1.000000000000000000, 1.000000000000000000, 1.000000000000000000, 1.000000000000000000, 1.000000000000000000, 1.000000000000000000, 1.000000000000000000, 1.000000000000000000, 1.000000000000000000, 1.000000000000000000, 1.000000000000000000, 1.000000000000000000, 1.000000000000000000, 1.000000000000000000, 1.000000000000000000, 1.000000000000000000, 1.000000000000000000, 1.000000000000000000, 1.000000000000000000, 1.000000000000000000, 1.000000000000000000, 1.000000000000000000, 1.000000000000000000, 1.000000000000000000, 1.000000000000000000, 1.000000000000000000, 1.000000000000000000, 1.000000000000000000, 1.000000000000000000, 1.000000000000000000, 1.000000000000000000, 1.000000000000000000, 1.000000000000000000, 1.000000000000000000, 1.000000000000000000, 1.000000000000000000, 1.000000000000000000, 1.000000000000000000, 1.000000000000000000, 1.000000000000000000, 1.000000000000000000, 1.000000000000000000, 1.000000000000000000, 1.000000000000000000, 1.000000000000000000, 1.000000000000000000, 1.000000000000000000, 1.000000000000000000, 1.000000000000000000, 1.000000000000000000, 1.000000000000000000, 1.000000000000000000, 1.000000000000000000, 1.000000000000000000, 1.000000000000000000, 1.000000000000000000, 1.000000000000000000, 1.000000000000000000, 1.000000000000000000, 1.000000000000000000, 1.000000000000000000, 1.000000000000000000, 1.000000000000000000, 1.000000000000000000, 1.000000000000000000, 1.000000000000000000, 1.000000000000000000, 1.000000000000000000, 1.000000000000000000, 1.000000000000000000, 1.000000000000000000, 1.000000000000000000, 1.000000000000000000, 1.000000000000000000, 1.000000000000000000, 1.000000000000000000, 1.000000000000000000, 1.000000000000000000, 1.000000000000000000, 1.000000000000000000, 1.000000000000000000, 1.000000000000000000, 1.000000000000000000, 1.000000000000000000, 1.000000000000000000, 1.000000000000000000, 1.000000000000000000, 1.000000000000000000, 1.000000000000000000, 1.000000000000000000, 1.000000000000000000, 1.000000000000000000, 1.000000000000000000, 1.000000000000000000, 1.000000000000000000, 1.000000000000000000, 1.000000000000000000, 1.000000000000000000, 1.000000000000000000, 1.000000000000000000, 1.000000000000000000, 1.000000000000000000, 1.000000000000000000, 1.000000000000000000, 1.000000000000000000, 1.000000000000000000, 1.000000000000000000, 1.000000000000000000, 1.000000000000000000, 1.000000000000000000, 1.000000000000000000, 1.000000000000000000, 1.000000000000000000, 1.000000000000000000, 1.000000000000000000, 1.000000000000000000, 1.000000000000000000, 1.000000000000000000, 1.000000000000000000, 1.000000000000000000, 1.000000000000000000, 1.000000000000000000, 1.000000000000000000, 1.000000000000000000, 1.000000000000000000, 1.000000000000000000, 1.000000000000000000, 1.000000000000000000, 1.000000000000000000, 1.000000000000000000, 1.000000000000000000, 1.000000000000000000, 1.000000000000000000, 1.000000000000000000, 1.000000000000000000, 1.000000000000000000, 1.000000000000000000, 1.000000000000000000, 1.000000000000000000, 1.000000000000000000, 1.000000000000000000, 1.000000000000000000, 1.000000000000000000, 1.000000000000000000, 1.000000000000000000, 1.000000000000000000, 1.000000000000000000, 1.000000000000000000, 1.000000000000000000, 1.000000000000000000, 1.000000000000000000, 1.000000000000000000, 1.000000000000000000, 1.000000000000000000, 1.000000000000000000, 1.000000000000000000),
 ( 0.3333333333333333703, 0.3333333333333333703, 0.3333333333333333703, 0.3333333333333333703, 0.3333333333333333703, 0.3333333333333333703, 0.3333333333333333703, 0.3333333333333333703, 0.3333333333333333703, 0.3333333333333333703, 0.3333333333333333703, 0.3333333333333333703, 0.3333333333333333703, 0.3333333333333333703, 0.3333333333333333703, 0.3333333333333333703, 0.3333333333333333703, 0.3333333333333333703, 0.3333333333333333703, 0.3333333333333333703, 0.3333333333333333703, 0.3333333333333333703, 0.3333333333333333703, 0.3333333333333333703, 0.3333333333333333703, 0.3333333333333333703, 0.3333333333333333703, 0.3333333333333333703, 0.3333333333333333703, 0.3333333333333333703, 0.3333333333333333703, 0.3333333333333333703, 0.3333333333333333703, 0.3333333333333333703, 0.3333333333333333703, 0.3333333333333333703, 0.3333333333333333703, 0.3333333333333333703, 0.3333333333333333703, 0.3333333333333333703, 0.3333333333333333703, 0.3333333333333333703, 0.3333333333333333703, 0.3333333333333333703, 0.3333333333333333703, 0.3333333333333333703, 0.3333333333333333703, 0.3333333333333333703, 0.3333333333333333703, 0.3333333333333333703, 0.3333333333333333703, 0.3333333333333333703, 0.3333333333333333703, 0.3333333333333333703, 0.3333333333333333703, 0.3333333333333333703, 0.3333333333333333703, 0.3333333333333333703, 0.3333333333333333703, 0.3333333333333333703, 0.3333333333333333703, 0.3333333333333333703, 0.3333333333333333703, 0.3333333333333333703, 0.3333333333333333703, 0.3333333333333333703, 0.3333333333333333703, 0.3333333333333333703, 0.3333333333333333703, 0.3333333333333333703, 0.3333333333333333703, 0.3333333333333333703, 0.3333333333333333703, 0.3333333333333333703, 0.3333333333333333703, 0.3333333333333333703, 0.3333333333333333703, 0.3333333333333333703, 0.3333333333333333703, 0.3333333333333333703, 0.3333333333333333703, 0.3333333333333333703, 0.3333333333333333703, 0.3333333333333333703, 0.3333333333333333703, 0.3333333333333333703, 0.3333333333333333703, 0.3333333333333333703, 0.3333333333333333703, 0.3333333333333333703, 0.3333333333333333703, 0.3333333333333333703, 0.3333333333333333703, 0.3333333333333333703, 0.3333333333333333703, 0.3333333333333333703, 0.3333333333333333703, 0.3333333333333333703, 0.3333333333333333703, 0.3333333333333333703, 0.3333333333333333703, 0.3333333333333333703, 0.3333333333333333703, 0.3333333333333333703, 0.3333333333333333703, 0.3333333333333333703, 0.3333333333333333703, 0.3333333333333333703, 0.3333333333333333703, 0.3333333333333333703, 0.3333333333333333703, 0.3333333333333333703, 0.3333333333333333703, 0.3333333333333333703, 0.3333333333333333703, 0.3333333333333333703, 0.3333333333333333703, 0.3333333333333333703, 0.3333333333333333703, 0.3333333333333333703, 0.3333333333333333703, 0.3333333333333333703, 0.3333333333333333703, 0.3333333333333333703, 0.3333333333333333703, 0.3333333333333333703, 0.3333333333333333703, 0.3333333333333333703, 0.3333333333333333703, 0.3333333333333333703, 0.3333333333333333703, 0.3333333333333333703, 0.3333333333333333703, 0.3333333333333333703, 0.3333333333333333703, 0.3333333333333333703, 0.3333333333333333703, 0.3333333333333333703, 0.3333333333333333703, 0.3333333333333333703, 0.3333333333333333703, 0.3333333333333333703, 0.3333333333333333703, 0.3333333333333333703, 0.3333333333333333703, 0.3333333333333333703, 0.3333333333333333703, 0.3333333333333333703, 0.3333333333333333703, 0.3333333333333333703, 0.3333333333333333703, 0.3333333333333333703, 0.3333333333333333703, 0.3333333333333333703, 0.3333333333333333703, 0.3333333333333333703, 0.3333333333333333703, 0.3333333333333333703, 0.3333333333333333703, 0.3333333333333333703, 0.3333333333333333703, 0.3333333333333333703, 0.3333333333333333703, 0.3333333333333333703, 0.3333333333333333703, 0.3333333333333333703, 0.3333333333333333703, 0.3333333333333333703, 0.3333333333333333703, 0.3333333333333333703, 0.3333333333333333703, 0.3333333333333333703, 0.3333333333333333703, 0.3333333333333333703, 0.3333333333333333703, 0.3333333333333333703, 0.3333333333333333703, 0.3333333333333333703, 0.3333333333333333703, 0.3333333333333333703, 0.3333333333333333703, 0.3333333333333333703, 0.3333333333333333703, 0.3333333333333333703, 0.3333333333333333703, 0.3333333333333333703, 0.3333333333333333703, 0.3333333333333333703, 0.3333333333333333703, 0.3333333333333333703, 0.3333333333333333703, 0.3333333333333333703, 0.3333333333333333703, 0.3333333333333333703, 0.3333333333333333703, 0.3333333333333333703, 0.3333333333333333703, 0.3333333333333333703, 0.3333333333333333703, 0.3333333333333333703, 0.3333333333333333703, 0.3333333333333333703, 0.3333333333333333703, 0.3333333333333333703, 0.3333333333333333703, 0.3333333333333333703, 0.3333333333333333703, 0.3333333333333333703, 0.3333333333333333703, 0.3333333333333333703, 0.3333333333333333703, 0.3333333333333333703, 0.3333333333333333703, 0.3333333333333333703, 0.3333333333333333703, 0.3333333333333333703, 0.3333333333333333703, 0.3333333333333333703, 0.3333333333333333703, 0.3333333333333333703, 0.3333333333333333703, 0.3333333333333333703, 0.3333333333333333703, 0.3333333333333333703, 0.3333333333333333703, 0.3333333333333333703, 0.3333333333333333703, 0.3333333333333333703, 0.3333333333333333703, 0.3333333333333333703, 0.3333333333333333703, 0.3333333333333333703, 0.3333333333333333703, 0.3333333333333333703, 0.3333333333333333703, 0.3333333333333333703, 0.3333333333333333703, 0.3333333333333333703, 0.3333333333333333703, 0.3333333333333333703, 0.3333333333333333703, 0.3333333333333333703, 0.3333333333333333703, 0.3333333333333333703, 0.3333333333333333703, 0.3333333333333333703, 0.3333333333333333703, 0.3333333333333333703, 0.3333333333333333703, 0.3333333333333333703, 0.3333333333333333703, 0.3333333333333333703, 0.3333333333333333703, 0.3333333333333333703, 0.3333333333333333703, 0.3333333333333333703, 0.3333333333333333703, 0.3333333333333333703, 0.3333333333333333703, 0.3333333333333333703, 0.3333333333333333703, 0.3333333333333333703, 0.3333333333333333703, 0.3333333333333333703, 0.3333333333333333703, 0.3333333333333333703, 0.3333333333333333703, 0.3333333333333333703, 0.3333333333333333703, 0.3333333333333333703, 0.3333333333333333703, 0.3333333333333333703, 0.3333333333333333703, 0.3333333333333333703, 0.3333333333333333703, 0.3333333333333333703, 0.3333333333333333703, 0.3333333333333333703, 0.3333333333333333703, 0.3333333333333333703, 0.3333333333333333703, 0.3333333333333333703, 0.3333333333333333703, 0.3333333333333333703, 0.3333333333333333703, 0.3333333333333333703, 0.3333333333333333703, 0.3333333333333333703, 0.3333333333333333703, 0.3333333333333333703, 0.3333333333333333703, 0.3333333333333333703, 0.3333333333333333703, 0.3333333333333333703, 0.3333333333333333703, 0.3333333333333333703, 0.3333333333333333703, 0.3333333333333333703, 0.3333333333333333703, 0.3333333333333333703, 0.3333333333333333703, 0.3333333333333333703, 0.3333333333333333703, 0.3333333333333333703, 0.3333333333333333703, 0.3333333333333333703, 0.3333333333333333703, 0.3333333333333333703, 0.3333333333333333703, 0.3333333333333333703, 0.3333333333333333703, 0.3333333333333333703, 0.3333333333333333703, 0.3333333333333333703, 0.3333333333333333703, 0.3333333333333333703, 0.3333333333333333703, 0.3333333333333333703, 0.3333333333333333703, 0.3333333333333333703, 0.3333333333333333703, 0.3333333333333333703, 0.3333333333333333703, 0.3333333333333333703, 0.3333333333333333703, 0.3333333333333333703, 0.3333333333333333703, 0.3333333333333333703, 0.3333333333333333703, 0.3333333333333333703, 0.3333333333333333703, 0.3333333333333333703, 0.3333333333333333703, 0.3333333333333333703, 0.3333333333333333703, 0.3333333333333333703),
 ( 0.3333333333333333703, 0.3333333333333333703, 0.3333333333333333703, 0.3333333333333333703, 0.3333333333333333703, 0.3333333333333333703, 0.3333333333333333703, 0.3333333333333333703, 0.3333333333333333703, 0.3333333333333333703, 0.3333333333333333703, 0.3333333333333333703, 0.3333333333333333703, 0.3333333333333333703, 0.3333333333333333703, 0.3333333333333333703, 0.3333333333333333703, 0.3333333333333333703, 0.3333333333333333703, 0.3333333333333333703, 0.3333333333333333703, 0.3333333333333333703, 0.3333333333333333703, 0.3333333333333333703, 0.3333333333333333703, 0.3333333333333333703, 0.3333333333333333703, 0.3333333333333333703, 0.3333333333333333703, 0.3333333333333333703, 0.3333333333333333703, 0.3333333333333333703, 0.3333333333333333703, 0.3333333333333333703, 0.3333333333333333703, 0.3333333333333333703, 0.3333333333333333703, 0.3333333333333333703, 0.3333333333333333703, 0.3333333333333333703, 0.3333333333333333703, 0.3333333333333333703, 0.3333333333333333703, 0.3333333333333333703, 0.3333333333333333703, 0.3333333333333333703, 0.3333333333333333703, 0.3333333333333333703, 0.3333333333333333703, 0.3333333333333333703, 0.3333333333333333703, 0.3333333333333333703, 0.3333333333333333703, 0.3333333333333333703, 0.3333333333333333703, 0.3333333333333333703, 0.3333333333333333703, 0.3333333333333333703, 0.3333333333333333703, 0.3333333333333333703, 0.3333333333333333703, 0.3333333333333333703, 0.3333333333333333703, 0.3333333333333333703, 0.3333333333333333703, 0.3333333333333333703, 0.3333333333333333703, 0.3333333333333333703, 0.3333333333333333703, 0.3333333333333333703, 0.3333333333333333703, 0.3333333333333333703, 0.3333333333333333703, 0.3333333333333333703, 0.3333333333333333703, 0.3333333333333333703, 0.3333333333333333703, 0.3333333333333333703, 0.3333333333333333703, 0.3333333333333333703, 0.3333333333333333703, 0.3333333333333333703, 0.3333333333333333703, 0.3333333333333333703, 0.3333333333333333703, 0.3333333333333333703, 0.3333333333333333703, 0.3333333333333333703, 0.3333333333333333703, 0.3333333333333333703, 0.3333333333333333703, 0.3333333333333333703, 0.3333333333333333703, 0.3333333333333333703, 0.3333333333333333703, 0.3333333333333333703, 0.3333333333333333703, 0.3333333333333333703, 0.3333333333333333703, 0.3333333333333333703, 0.3333333333333333703, 0.3333333333333333703, 0.3333333333333333703, 0.3333333333333333703, 0.3333333333333333703, 0.3333333333333333703, 0.3333333333333333703, 0.3333333333333333703, 0.3333333333333333703, 0.3333333333333333703, 0.3333333333333333703, 0.3333333333333333703, 0.3333333333333333703, 0.3333333333333333703, 0.3333333333333333703, 0.3333333333333333703, 0.3333333333333333703, 0.3333333333333333703, 0.3333333333333333703, 0.3333333333333333703, 0.3333333333333333703, 0.3333333333333333703, 0.3333333333333333703, 0.3333333333333333703, 0.3333333333333333703, 0.3333333333333333703, 0.3333333333333333703, 0.3333333333333333703, 0.3333333333333333703, 0.3333333333333333703, 0.3333333333333333703, 0.3333333333333333703, 0.3333333333333333703, 0.3333333333333333703, 0.3333333333333333703, 0.3333333333333333703, 0.3333333333333333703, 0.3333333333333333703, 0.3333333333333333703, 0.3333333333333333703, 0.3333333333333333703, 0.3333333333333333703, 0.3333333333333333703, 0.3333333333333333703, 0.3333333333333333703, 0.3333333333333333703, 0.3333333333333333703, 0.3333333333333333703, 0.3333333333333333703, 0.3333333333333333703, 0.3333333333333333703, 0.3333333333333333703, 0.3333333333333333703, 0.3333333333333333703, 0.3333333333333333703, 0.3333333333333333703, 0.3333333333333333703, 0.3333333333333333703, 0.3333333333333333703, 0.3333333333333333703, 0.3333333333333333703, 0.3333333333333333703, 0.3333333333333333703, 0.3333333333333333703, 0.3333333333333333703, 0.3333333333333333703, 0.3333333333333333703, 0.3333333333333333703, 0.3333333333333333703, 0.3333333333333333703, 0.3333333333333333703, 0.3333333333333333703, 0.3333333333333333703, 0.3333333333333333703, 0.3333333333333333703, 0.3333333333333333703, 0.3333333333333333703, 0.3333333333333333703, 0.3333333333333333703, 0.3333333333333333703, 0.3333333333333333703, 0.3333333333333333703, 0.3333333333333333703, 0.3333333333333333703, 0.3333333333333333703, 0.3333333333333333703, 0.3333333333333333703, 0.3333333333333333703, 0.3333333333333333703, 0.3333333333333333703, 0.3333333333333333703, 0.3333333333333333703, 0.3333333333333333703, 0.3333333333333333703, 0.3333333333333333703, 0.3333333333333333703, 0.3333333333333333703, 0.3333333333333333703, 0.3333333333333333703, 0.3333333333333333703, 0.3333333333333333703, 0.3333333333333333703, 0.3333333333333333703, 0.3333333333333333703, 0.3333333333333333703, 0.3333333333333333703, 0.3333333333333333703, 0.3333333333333333703, 0.3333333333333333703, 0.3333333333333333703, 0.3333333333333333703, 0.3333333333333333703, 0.3333333333333333703, 0.3333333333333333703, 0.3333333333333333703, 0.3333333333333333703, 0.3333333333333333703, 0.3333333333333333703, 0.3333333333333333703, 0.3333333333333333703, 0.3333333333333333703, 0.3333333333333333703, 0.3333333333333333703, 0.3333333333333333703, 0.3333333333333333703, 0.3333333333333333703, 0.3333333333333333703, 0.3333333333333333703, 0.3333333333333333703, 0.3333333333333333703, 0.3333333333333333703, 0.3333333333333333703, 0.3333333333333333703, 0.3333333333333333703, 0.3333333333333333703, 0.3333333333333333703, 0.3333333333333333703, 0.3333333333333333703, 0.3333333333333333703, 0.3333333333333333703, 0.3333333333333333703, 0.3333333333333333703, 0.3333333333333333703, 0.3333333333333333703, 0.3333333333333333703, 0.3333333333333333703, 0.3333333333333333703, 0.3333333333333333703, 0.3333333333333333703, 0.3333333333333333703, 0.3333333333333333703, 0.3333333333333333703, 0.3333333333333333703, 0.3333333333333333703, 0.3333333333333333703, 0.3333333333333333703, 0.3333333333333333703, 0.3333333333333333703, 0.3333333333333333703, 0.3333333333333333703, 0.3333333333333333703, 0.3333333333333333703, 0.3333333333333333703, 0.3333333333333333703, 0.3333333333333333703, 0.3333333333333333703, 0.3333333333333333703, 0.3333333333333333703, 0.3333333333333333703, 0.3333333333333333703, 0.3333333333333333703, 0.3333333333333333703, 0.3333333333333333703, 0.3333333333333333703, 0.3333333333333333703, 0.3333333333333333703, 0.3333333333333333703, 0.3333333333333333703, 0.3333333333333333703, 0.3333333333333333703, 0.3333333333333333703, 0.3333333333333333703, 0.3333333333333333703, 0.3333333333333333703, 0.3333333333333333703, 0.3333333333333333703, 0.3333333333333333703, 0.3333333333333333703, 0.3333333333333333703, 0.3333333333333333703, 0.3333333333333333703, 0.3333333333333333703, 0.3333333333333333703, 0.3333333333333333703, 0.3333333333333333703, 0.3333333333333333703, 0.3333333333333333703, 0.3333333333333333703, 0.3333333333333333703, 0.3333333333333333703, 0.3333333333333333703, 0.3333333333333333703, 0.3333333333333333703, 0.3333333333333333703, 0.3333333333333333703, 0.3333333333333333703, 0.3333333333333333703, 0.3333333333333333703, 0.3333333333333333703, 0.3333333333333333703, 0.3333333333333333703, 0.3333333333333333703, 0.3333333333333333703, 0.3333333333333333703, 0.3333333333333333703, 0.3333333333333333703, 0.3333333333333333703, 0.3333333333333333703, 0.3333333333333333703, 0.3333333333333333703, 0.3333333333333333703, 0.3333333333333333703, 0.3333333333333333703, 0.3333333333333333703, 0.3333333333333333703, 0.3333333333333333703, 0.3333333333333333703, 0.3333333333333333703, 0.3333333333333333703, 0.3333333333333333703, 0.3333333333333333703, 0.3333333333333333703, 0.3333333333333333703, 0.3333333333333333703, 0.3333333333333333703, 0.3333333333333333703),
 ( 1.000000000000000000, 1.000000000000000000, 1.000000000000000000, 1.000000000000000000, 1.000000000000000000, 1.000000000000000000, 1.000000000000000000, 1.000000000000000000, 1.000000000000000000, 1.000000000000000000, 1.000000000000000000, 1.000000000000000000, 1.000000000000000000, 1.000000000000000000, 1.000000000000000000, 1.000000000000000000, 1.000000000000000000, 1.000000000000000000, 1.000000000000000000, 1.000000000000000000, 1.000000000000000000, 1.000000000000000000, 1.000000000000000000, 1.000000000000000000, 1.000000000000000000, 1.000000000000000000, 1.000000000000000000, 1.000000000000000000, 1.000000000000000000, 1.000000000000000000, 1.000000000000000000, 1.000000000000000000, 1.000000000000000000, 1.000000000000000000, 1.000000000000000000, 1.000000000000000000, 1.000000000000000000, 1.000000000000000000, 1.000000000000000000, 1.000000000000000000, 1.000000000000000000, 1.000000000000000000, 1.000000000000000000, 1.000000000000000000, 1.000000000000000000, 1.000000000000000000, 1.000000000000000000, 1.000000000000000000, 1.000000000000000000, 1.000000000000000000, 1.000000000000000000, 1.000000000000000000, 1.000000000000000000, 1.000000000000000000, 1.000000000000000000, 1.000000000000000000, 1.000000000000000000, 1.000000000000000000, 1.000000000000000000, 1.000000000000000000, 1.000000000000000000, 1.000000000000000000, 1.000000000000000000, 1.000000000000000000, 1.000000000000000000, 1.000000000000000000, 1.000000000000000000, 1.000000000000000000, 1.000000000000000000, 1.000000000000000000, 1.000000000000000000, 1.000000000000000000, 1.000000000000000000, 1.000000000000000000, 1.000000000000000000, 1.000000000000000000, 1.000000000000000000, 1.000000000000000000, 1.000000000000000000, 1.000000000000000000, 1.000000000000000000, 1.000000000000000000, 1.000000000000000000, 1.000000000000000000, 1.000000000000000000, 1.000000000000000000, 1.000000000000000000, 1.000000000000000000, 1.000000000000000000, 1.000000000000000000, 1.000000000000000000, 1.000000000000000000, 1.000000000000000000, 1.000000000000000000, 1.000000000000000000, 1.000000000000000000, 1.000000000000000000, 1.000000000000000000, 1.000000000000000000, 1.000000000000000000, 1.000000000000000000, 1.000000000000000000, 1.000000000000000000, 1.000000000000000000, 1.000000000000000000, 1.000000000000000000, 1.000000000000000000, 1.000000000000000000, 1.000000000000000000, 1.000000000000000000, 1.000000000000000000, 1.000000000000000000, 1.000000000000000000, 1.000000000000000000, 1.000000000000000000, 1.000000000000000000, 1.000000000000000000, 1.000000000000000000, 1.000000000000000000, 1.000000000000000000, 1.000000000000000000, 1.000000000000000000, 1.000000000000000000, 1.000000000000000000, 1.000000000000000000, 1.000000000000000000, 1.000000000000000000, 1.000000000000000000, 1.000000000000000000, 1.000000000000000000, 1.000000000000000000, 1.000000000000000000, 1.000000000000000000, 1.000000000000000000, 1.000000000000000000, 1.000000000000000000, 1.000000000000000000, 1.000000000000000000, 1.000000000000000000, 1.000000000000000000, 1.000000000000000000, 1.000000000000000000, 1.000000000000000000, 1.000000000000000000, 1.000000000000000000, 1.000000000000000000, 1.000000000000000000, 1.000000000000000000, 1.000000000000000000, 1.000000000000000000, 1.000000000000000000, 1.000000000000000000, 1.000000000000000000, 1.000000000000000000, 1.000000000000000000, 1.000000000000000000, 1.000000000000000000, 1.000000000000000000, 1.000000000000000000, 1.000000000000000000, 1.000000000000000000, 1.000000000000000000, 1.000000000000000000, 1.000000000000000000, 1.000000000000000000, 1.000000000000000000, 1.000000000000000000, 1.000000000000000000, 1.000000000000000000, 1.000000000000000000, 1.000000000000000000, 1.000000000000000000, 1.000000000000000000, 1.000000000000000000, 1.000000000000000000, 1.000000000000000000, 1.000000000000000000, 1.000000000000000000, 1.000000000000000000, 1.000000000000000000, 1.000000000000000000, 1.000000000000000000, 1.000000000000000000, 1.000000000000000000, 1.000000000000000000, 1.000000000000000000, 1.000000000000000000, 1.000000000000000000, 1.000000000000000000, 1.000000000000000000, 1.000000000000000000, 1.000000000000000000, 1.000000000000000000, 1.000000000000000000, 1.000000000000000000, 1.000000000000000000, 1.000000000000000000, 1.000000000000000000, 1.000000000000000000, 1.000000000000000000, 1.000000000000000000, 1.000000000000000000, 1.000000000000000000, 1.000000000000000000, 1.000000000000000000, 1.000000000000000000, 1.000000000000000000, 1.000000000000000000, 1.000000000000000000, 1.000000000000000000, 1.000000000000000000, 1.000000000000000000, 1.000000000000000000, 1.000000000000000000, 1.000000000000000000, 1.000000000000000000, 1.000000000000000000, 1.000000000000000000, 1.000000000000000000, 1.000000000000000000, 1.000000000000000000, 1.000000000000000000, 1.000000000000000000, 1.000000000000000000, 1.000000000000000000, 1.000000000000000000, 1.000000000000000000, 1.000000000000000000, 1.000000000000000000, 1.000000000000000000, 1.000000000000000000, 1.000000000000000000, 1.000000000000000000, 1.000000000000000000, 1.000000000000000000, 1.000000000000000000, 1.000000000000000000, 1.000000000000000000, 1.000000000000000000, 1.000000000000000000, 1.000000000000000000, 1.000000000000000000, 1.000000000000000000, 1.000000000000000000, 1.000000000000000000, 1.000000000000000000, 1.000000000000000000, 1.000000000000000000, 1.000000000000000000, 1.000000000000000000, 1.000000000000000000, 1.000000000000000000, 1.000000000000000000, 1.000000000000000000, 1.000000000000000000, 1.000000000000000000, 1.000000000000000000, 1.000000000000000000, 1.000000000000000000, 1.000000000000000000, 1.000000000000000000, 1.000000000000000000, 1.000000000000000000, 1.000000000000000000, 1.000000000000000000, 1.000000000000000000, 1.000000000000000000, 1.000000000000000000, 1.000000000000000000, 1.000000000000000000, 1.000000000000000000, 1.000000000000000000, 1.000000000000000000, 1.000000000000000000, 1.000000000000000000, 1.000000000000000000, 1.000000000000000000, 1.000000000000000000, 1.000000000000000000, 1.000000000000000000, 1.000000000000000000, 1.000000000000000000, 1.000000000000000000, 1.000000000000000000, 1.000000000000000000, 1.000000000000000000, 1.000000000000000000, 1.000000000000000000, 1.000000000000000000, 1.000000000000000000, 1.000000000000000000, 1.000000000000000000, 1.000000000000000000, 1.000000000000000000, 1.000000000000000000, 1.000000000000000000, 1.000000000000000000, 1.000000000000000000, 1.000000000000000000, 1.000000000000000000, 1.000000000000000000, 1.000000000000000000, 1.000000000000000000, 1.000000000000000000, 1.000000000000000000, 1.000000000000000000, 1.000000000000000000, 1.000000000000000000, 1.000000000000000000, 1.000000000000000000, 1.000000000000000000, 1.000000000000000000, 1.000000000000000000, 1.000000000000000000, 1.000000000000000000, 1.000000000000000000, 1.000000000000000000, 1.000000000000000000, 1.000000000000000000, 1.000000000000000000, 1.000000000000000000, 1.000000000000000000, 1.000000000000000000, 1.000000000000000000, 1.000000000000000000, 1.000000000000000000, 1.000000000000000000, 1.000000000000000000, 1.000000000000000000, 1.000000000000000000, 1.000000000000000000, 1.000000000000000000, 1.000000000000000000, 1.000000000000000000, 1.000000000000000000, 1.000000000000000000) ) ) 
 REPRESENTATION_ITEM ( '' )  SURFACE ( )  );
#13782=CARTESIAN_POINT ( 'NONE',  ( 9.678950682101415737, -24.51930918146190663, -231.5088683414745105 ) ) ;
#13783=CARTESIAN_POINT ( 'NONE',  ( -10.23029362138610843, 26.44342627367518617, -221.6879936327511871 ) ) ;
#13784=CARTESIAN_POINT ( 'NONE',  ( 2.485733319737138736, 14.76073968410796056, -221.5245536174130905 ) ) ;
#13785=CARTESIAN_POINT ( 'NONE',  ( -17.58118739749173898, -8.238107657346720458, -217.5252134542318458 ) ) ;
#13786=CARTESIAN_POINT ( 'NONE',  ( -15.82036597035495795, 4.920771916499852239, -223.0095317795067160 ) ) ;
#13787=CARTESIAN_POINT ( 'NONE',  ( 16.11883106748507188, 21.48229216499086291, -233.4985352728212433 ) ) ;
#13789=CARTESIAN_POINT ( 'NONE',  ( 10.02513374692848913, 18.81568788741115128, -217.1505009242214612 ) ) ;
#13790=CARTESIAN_POINT ( 'NONE',  ( 15.22026983281163481, -5.531916908390004828, -229.4891270354009123 ) ) ;
#13791=CARTESIAN_POINT ( 'NONE',  ( 11.97732832373273126, -6.576952149368169742, -223.6031523087739572 ) ) ;
#13793=CARTESIAN_POINT ( 'NONE',  ( 22.84140515590350518, 18.29101041979067332, -226.2334522600520472 ) ) ;
#13794=CARTESIAN_POINT ( 'NONE',  ( -17.75199675706278413, -2.086992369311378326, -216.9839424855219931 ) ) ;
#13795=CARTESIAN_POINT ( 'NONE',  ( -7.460068573003235670, -29.58770008691625364, -228.1902472473001637 ) ) ;
#13797=CARTESIAN_POINT ( 'NONE',  ( 6.131461862964278531, -15.14974102410872625, -231.6805438559109973 ) ) ;
#13799=CARTESIAN_POINT ( 'NONE',  ( -3.015877970456246615, 27.27456613555083464, -227.6995284396757313 ) ) ;
#13801=CARTESIAN_POINT ( 'NONE',  ( 12.98277799799954124, 10.30128574332056779, -221.9415428419440559 ) ) ;
#13802=CARTESIAN_POINT ( 'NONE',  ( -11.98736441306973077, 11.45674391201457176, -217.8252237716743025 ) ) ;
#13803=CARTESIAN_POINT ( 'NONE',  ( -8.881241380679488984, 27.18697625135247975, -224.4474391433207927 ) ) ;
#13804=CARTESIAN_POINT ( 'NONE',  ( 13.92699808111095905, -7.117895771238833547, -219.6066573659836081 ) ) ;
#13806=CARTESIAN_POINT ( 'NONE',  ( -4.130417896617784912, 16.21758012034559826, -229.8171973319304584 ) ) ;
#13807=CARTESIAN_POINT ( 'NONE',  ( -23.99493126334580850, 6.052326449358573335, -219.7958990219547672 ) ) ;
#13808=CARTESIAN_POINT ( 'NONE',  ( 20.82555317450757215, 14.06078233701296476, -215.4201375757437802 ) ) ;
#13809=CARTESIAN_POINT ( 'NONE',  ( 23.17317677245511831, -6.950782331930943414, -233.5406539459643227 ) ) ;
#13813=CARTESIAN_POINT ( 'NONE',  ( 0.9908753270255351575, 13.79205759140780430, -228.0165926715089881 ) ) ;
#13814=CARTESIAN_POINT ( 'NONE',  ( -12.28596215050325924, -1.831058988293407852, -228.6496409048244516 ) ) ;
#13816=CARTESIAN_POINT ( 'NONE',  ( 27.04607490430786854, 4.607450003618843049, -220.3758934308003461 ) ) ;
#13817=CARTESIAN_POINT ( 'NONE',  ( -15.15434969228324924, 4.423874646950748613, -230.6144467931089821 ) ) ;
#13819=CARTESIAN_POINT ( 'NONE',  ( 9.358654279681809740, -11.94480763145079472, -229.8864256833185777 ) ) ;
#13821=CARTESIAN_POINT ( 'NONE',  ( -21.89482327431018760, 1.733733432562314158, -233.1353281693111796 ) ) ;
#13823=CARTESIAN_POINT ( 'NONE',  ( -16.20072894238734307, 0.5024448614660336210, -230.4554067149722130 ) ) ;
#13824=CARTESIAN_POINT ( 'NONE',  ( -5.693514143275418604, -18.22526881224050754, -218.3451910747569968 ) ) ;
#13828=CARTESIAN_POINT ( 'NONE',  ( -27.29953305526601426, 11.21644211419729054, -229.3676346105362995 ) ) ;
#13829=CARTESIAN_POINT ( 'NONE',  ( 12.37559490515920579, -12.83230305503110991, -219.7713711637379106 ) ) ;
#13830=CARTESIAN_POINT ( 'NONE',  ( 13.28800886458158104, -2.093462502527361657, -227.1500392263112929 ) ) ;
#13832=CARTESIAN_POINT ( 'NONE',  ( 14.12692363916921146, 20.59586666873830296, -230.0804552526094540 ) ) ;
#13833=CARTESIAN_POINT ( 'NONE',  ( -17.81561310496929806, 18.25637658208611569, -215.7745954696244439 ) ) ;
#13834=CARTESIAN_POINT ( 'NONE',  ( 12.98277799799954124, 10.30128574332056779, -221.9415428419440559 ) ) ;
#13835=CARTESIAN_POINT ( 'NONE',  ( -3.542274070161974375, -15.57207032904040389, -222.0010230139451437 ) ) ;
#13836=CARTESIAN_POINT ( 'NONE',  ( 25.69249634387097814, -4.932549985819596472, -232.9896235759753438 ) ) ;
#13838=CARTESIAN_POINT ( 'NONE',  ( -12.62195384480319582, 9.244619650382723819, -228.6283004876635516 ) ) ;
#13839=CARTESIAN_POINT ( 'NONE',  ( -15.50322565568834321, 9.749075856218723857, -229.6019304695566916 ) ) ;
#13840=CARTESIAN_POINT ( 'NONE',  ( -12.10258892854866275, 5.599955477755926836, -221.6590149575334010 ) ) ;
#13842=CARTESIAN_POINT ( 'NONE',  ( -2.820113134979321590, -27.38213018110698727, -220.3670599055385821 ) ) ;
#13845=CARTESIAN_POINT ( 'NONE',  ( 15.90795275983908574, 2.546196724714939297, -229.0855319561646297 ) ) ;
#13846=CARTESIAN_POINT ( 'NONE',  ( 10.17740660404977149, -19.92573511251913132, -219.0500883963018737 ) ) ;
#13847=CARTESIAN_POINT ( 'NONE',  ( 5.017623471397871349, 29.83561274492976878, -222.9769172135417250 ) ) ;
#13848=CARTESIAN_POINT ( 'NONE',  ( -12.74846050492543625, 19.93509882904884734, -216.0172840992881049 ) ) ;
#13849=CARTESIAN_POINT ( 'NONE',  ( 12.71499452845021416, 2.172589307656224378, -223.9381607050773084 ) ) ;
#13850=CARTESIAN_POINT ( 'NONE',  ( 11.67669251569587985, 24.04736029062789981, -218.5856804285192254 ) ) ;
#13853=CARTESIAN_POINT ( 'NONE',  ( -6.163092920833200594, -27.00835405423771007, -232.1022292408408987 ) ) ;
#13855=CARTESIAN_POINT ( 'NONE',  ( 14.68556740487494849, -6.365102927765655672, -229.6664356779805587 ) ) ;
#13858=CARTESIAN_POINT ( 'NONE',  ( 18.06016678184731461, 2.257982981100609354, -218.9983079406065940 ) ) ;
#13859=CARTESIAN_POINT ( 'NONE',  ( -18.99425472824626482, -3.261482901149847180, -230.2374083206451871 ) ) ;
#13860=CARTESIAN_POINT ( 'NONE',  ( 30.55431851955342282, 7.682798326916945975, -224.9061577511691610 ) ) ;
#13861=CARTESIAN_POINT ( 'NONE',  ( 2.508382434586714282, 15.09451298870656011, -220.9010239894319625 ) ) ;
#13862=CARTESIAN_POINT ( 'NONE',  ( -3.130305314451475418, 18.08417128930788209, -217.9058652980469333 ) ) ;
#13864=CARTESIAN_POINT ( 'NONE',  ( 25.14972984070899997, 1.185371537549434029, -234.2576837523010909 ) ) ;
#13865=CARTESIAN_POINT ( 'NONE',  ( 10.02513374692848913, 18.81568788741115128, -217.1505009242214612 ) ) ;
#13866=CARTESIAN_POINT ( 'NONE',  ( -19.98042543492610079, 23.51949599776966693, -226.6701036947414138 ) ) ;
#13867=CARTESIAN_POINT ( 'NONE',  ( -24.19163806436329978, 8.131440952769249719, -230.9341214615949127 ) ) ;
#13868=CARTESIAN_POINT ( 'NONE',  ( -10.71823000853037655, -10.52987076429259794, -221.3501620068516331 ) ) ;
#13872=CARTESIAN_POINT ( 'NONE',  ( 26.91963614581376874, 6.107751173605064920, -232.2246916053503298 ) ) ;
#13873=CARTESIAN_POINT ( 'NONE',  ( -9.523248388595575875, 12.31121908620753125, -221.6288572946744182 ) ) ;
#13874=CARTESIAN_POINT ( 'NONE',  ( 5.264801124131998300, 10.54092478143144795, -226.4890466082630098 ) ) ;
#13876=CARTESIAN_POINT ( 'NONE',  ( -13.92046207272054303, -0.1600067567908077248, -224.5811699126800818 ) ) ;
#13877=CARTESIAN_POINT ( 'NONE',  ( -30.16874246778906254, -1.865472247480548962, -231.1182156560653880 ) ) ;
#13878=CARTESIAN_POINT ( 'NONE',  ( -14.84457943406284208, -4.054717634150219574, -219.4128920803699430 ) ) ;
#13879=CARTESIAN_POINT ( 'NONE',  ( -16.38161496430853248, 17.22219235543852989, -215.3343469598664797 ) ) ;
#13880=CARTESIAN_POINT ( 'NONE',  ( -5.804961988600464196, -12.67915086496026511, -228.7923277404792088 ) ) ;
#13881=CARTESIAN_POINT ( 'NONE',  ( -11.26857159993117996, 28.96895336474501192, -225.6039696848669678 ) ) ;
#13882=CARTESIAN_POINT ( 'NONE',  ( 17.88855223994683286, -5.550763357372503037, -216.0002797835408614 ) ) ;
#13886=CARTESIAN_POINT ( 'NONE',  ( 24.52160379727246209, 5.049198597839295033, -215.7868787176665535 ) ) ;
#13888=CARTESIAN_POINT ( 'NONE',  ( -3.071946796551161984, 23.17078151772539485, -231.0066194318698933 ) ) ;
#13889=CARTESIAN_POINT ( 'NONE',  ( -18.14952719657095415, 1.368063294522122275, -218.0005379682515922 ) ) ;
#13890=CARTESIAN_POINT ( 'NONE',  ( 13.69275646168278371, 8.674223198772375909, -220.8699857572541987 ) ) ;
#13891=CARTESIAN_POINT ( 'NONE',  ( 12.43753614017300713, 2.441361880258234862, -222.2750447601761721 ) ) ;
#13892=CARTESIAN_POINT ( 'NONE',  ( -0.6614632862528592172, -26.57152937425246719, -233.3304277112415548 ) ) ;
#13893=CARTESIAN_POINT ( 'NONE',  ( 1.773237071419721422, 13.09828209437875302, -220.6531024550077404 ) ) ;
#13895=CARTESIAN_POINT ( 'NONE',  ( 0.09627406729119250550, -13.23594471221713142, -227.7621942207877339 ) ) ;
#13896=CARTESIAN_POINT ( 'NONE',  ( -6.720912670637915198, 19.69156892798266512, -217.8848069150180891 ) ) ;
#13898=CARTESIAN_POINT ( 'NONE',  ( 13.82984244654956107, 22.51831320572884820, -232.1830460045772213 ) ) ;
#13900=CARTESIAN_POINT ( 'NONE',  ( -15.89118508636071958, -1.798691612803976492, -229.3605869667087234 ) ) ;
#13901=CARTESIAN_POINT ( 'NONE',  ( -23.67953786836281083, 9.946055673977088674, -229.5560005648173671 ) ) ;
#13902=CARTESIAN_POINT ( 'NONE',  ( -19.92987771446595957, 11.92619342620000999, -232.5382020162021206 ) ) ;
#13903=CARTESIAN_POINT ( 'NONE',  ( 12.91815243135930480, 5.607966342865584153, -224.2227256053222959 ) ) ;
#13905=CARTESIAN_POINT ( 'NONE',  ( 4.354034006296288339, 14.09944204372416188, -221.2519525881239417 ) ) ;
#13906=CARTESIAN_POINT ( 'NONE',  ( 17.04113992636424513, -19.77713422747145700, -220.8032168804961373 ) ) ;
#13907=CARTESIAN_POINT ( 'NONE',  ( 12.12535264607833341, -6.902938132833007501, -227.3565233277489597 ) ) ;
#13908=CARTESIAN_POINT ( 'NONE',  ( 0.04449911090679885967, 16.51968908208873899, -222.9067194156212111 ) ) ;
#13911=CARTESIAN_POINT ( 'NONE',  ( 12.23063869552301242, 12.84118223717021934, -218.8273164334868284 ) ) ;
#13912=CARTESIAN_POINT ( 'NONE',  ( -23.43110653090080930, -15.10372739875494297, -233.3642232949313211 ) ) ;
#13913=CARTESIAN_POINT ( 'NONE',  ( -5.240862053303020573, -11.96147391800445270, -224.1453450823045443 ) ) ;
#13914=CARTESIAN_POINT ( 'NONE',  ( 1.836136847161299990, -12.84546502099244591, -226.1727064218434293 ) ) ;
#13915=CARTESIAN_POINT ( 'NONE',  ( -2.532949683519015949, 17.18298404079579100, -229.0924323441805086 ) ) ;
#13917=CARTESIAN_POINT ( 'NONE',  ( 28.46362550855882745, 7.392895870364313282, -223.4682258299149566 ) ) ;
#13918=CARTESIAN_POINT ( 'NONE',  ( -11.79584727357715934, 6.509288465425584036, -222.6080315736180921 ) ) ;
#13919=CARTESIAN_POINT ( 'NONE',  ( -8.467651734177735534, 23.23776955534497546, -231.2693664226804913 ) ) ;
#13920=CARTESIAN_POINT ( 'NONE',  ( -0.9249541874382023465, 14.55235618511626328, -223.7321818898853962 ) ) ;
#13921=CARTESIAN_POINT ( 'NONE',  ( 14.46993441875745390, 0.2699826811589002284, -230.0986938382904157 ) ) ;
#13922=CARTESIAN_POINT ( 'NONE',  ( 15.89102655998366664, 24.10108298038447572, -232.7733025413564008 ) ) ;
#13923=CARTESIAN_POINT ( 'NONE',  ( 7.680972971696337304, -18.49313070787806623, -217.8811398819712508 ) ) ;
#13924=CARTESIAN_POINT ( 'NONE',  ( 13.72333679673841900, 0.3386527829963648095, -228.4185608440243413 ) ) ;
#13926=CARTESIAN_POINT ( 'NONE',  ( -11.42613629117093765, 28.09170287990588832, -228.7150250545069241 ) ) ;
#13927=CARTESIAN_POINT ( 'NONE',  ( -30.16874246778906254, -1.865472247480548962, -231.1182156560653880 ) ) ;
#13928=CARTESIAN_POINT ( 'NONE',  ( 27.96460686140487084, -1.872811165202790340, -220.9791906660856000 ) ) ;
#13929=CARTESIAN_POINT ( 'NONE',  ( 17.99029889091409018, 9.613712288440757092, -232.0298403238024036 ) ) ;
#13930=CARTESIAN_POINT ( 'NONE',  ( -27.29953305526601426, 11.21644211419729054, -229.3676346105362995 ) ) ;
#13931=CARTESIAN_POINT ( 'NONE',  ( 15.34510829589250491, -24.56813251781886009, -230.1307231235174982 ) ) ;
#13933=CARTESIAN_POINT ( 'NONE',  ( -6.571166997218196748, 12.74865329367398736, -229.9840124400968762 ) ) ;
#13934=CARTESIAN_POINT ( 'NONE',  ( -26.74045434827795020, 12.41518252455047744, -220.4617428697642652 ) ) ;
#13935=CARTESIAN_POINT ( 'NONE',  ( -1.198425787605166715, -24.00698511249634137, -218.1862405767648170 ) ) ;
#13937=CARTESIAN_POINT ( 'NONE',  ( 18.54610009393809023, 0.6523581019769808531, -231.1787333216317677 ) ) ;
#13938=CARTESIAN_POINT ( 'NONE',  ( -21.93900267957129557, 7.862893636934532360, -233.4951761057262161 ) ) ;
#13939=CARTESIAN_POINT ( 'NONE',  ( 12.89329787743523070, -9.350464391519500040, -225.0861735818250224 ) ) ;
#13940=CARTESIAN_POINT ( 'NONE',  ( -29.22168435891936156, -1.352755938724206519, -225.9547066689444250 ) ) ;
#13943=CARTESIAN_POINT ( 'NONE',  ( 21.15841376125116824, 4.865517895153391947, -217.1795922978051578 ) ) ;
#13944=CARTESIAN_POINT ( 'NONE',  ( -15.42311360645077301, 11.97619046995196079, -234.9244673706848801 ) ) ;
#13945=CARTESIAN_POINT ( 'NONE',  ( 24.14003655968566520, 13.76285650325712773, -228.1266575292093819 ) ) ;
#13946=CARTESIAN_POINT ( 'NONE',  ( 4.375292991814291987, -28.67199747747994465, -220.8092881619367631 ) ) ;
#13947=CARTESIAN_POINT ( 'NONE',  ( 29.08354724566992644, -8.084875104304042992, -220.4391609833976133 ) ) ;
#13949=CARTESIAN_POINT ( 'NONE',  ( 2.508382434586714282, 15.09451298870656011, -220.9010239894319625 ) ) ;
#13950=CARTESIAN_POINT ( 'NONE',  ( -21.67128887413246119, 15.53484693247673043, -229.0088198863946900 ) ) ;
#13951=CARTESIAN_POINT ( 'NONE',  ( -11.30246491834384770, 5.534029070539333794, -225.8243940897388597 ) ) ;
#13952=CARTESIAN_POINT ( 'NONE',  ( -16.95213199947759009, -16.93177456301608785, -219.4409135693619817 ) ) ;
#13955=CARTESIAN_POINT ( 'NONE',  ( 28.09488075336259527, 3.911739131332936381, -227.7543364642411632 ) ) ;
#13956=CARTESIAN_POINT ( 'NONE',  ( 12.70100985296128115, -15.77027744429350165, -219.4156470604730202 ) ) ;
#13957=CARTESIAN_POINT ( 'NONE',  ( 14.31308345469695453, 12.76656023072872159, -231.9445021321040770 ) ) ;
#13958=CARTESIAN_POINT ( 'NONE',  ( -11.49049084071896409, 11.06834963248926940, -218.3354249205727058 ) ) ;
#13959=CARTESIAN_POINT ( 'NONE',  ( 26.56239871811266440, 9.439457669498057868, -217.7226690415261885 ) ) ;
#13960=CARTESIAN_POINT ( 'NONE',  ( 15.91295838535984331, 21.88410254487826379, -230.9583961155862823 ) ) ;
#13962=CARTESIAN_POINT ( 'NONE',  ( 1.904360901363437275, -12.77109371939166138, -224.5066922355585177 ) ) ;
#13963=CARTESIAN_POINT ( 'NONE',  ( 9.918856707546316542, -11.48950767347732871, -219.9734948840342668 ) ) ;
#13966=CARTESIAN_POINT ( 'NONE',  ( -13.00859847561873117, 4.399982435993697649, -231.0885370824921097 ) ) ;
#13967=CARTESIAN_POINT ( 'NONE',  ( -16.80743794350546594, -8.145538706591455735, -220.2004866397506078 ) ) ;
#13968=CARTESIAN_POINT ( 'NONE',  ( -17.43458823433387650, 2.804998135793385750, -231.8077100320880959 ) ) ;
#13969=CARTESIAN_POINT ( 'NONE',  ( 3.160467108836292116, 14.95099014189016629, -228.9242958482614370 ) ) ;
#13970=CARTESIAN_POINT ( 'NONE',  ( 5.711092584709906106, 26.13380667269736790, -220.5232813324456629 ) ) ;
#13972=CARTESIAN_POINT ( 'NONE',  ( 16.03771109128167538, -13.01076189404929195, -214.9179096003404084 ) ) ;
#13973=CARTESIAN_POINT ( 'NONE',  ( 26.29894631880581812, 12.29609390142961090, -226.3100047295820332 ) ) ;
#13974=CARTESIAN_POINT ( 'NONE',  ( -13.25293905438448405, 17.39325876214774524, -215.6628841494472510 ) ) ;
#13975=CARTESIAN_POINT ( 'NONE',  ( -23.89856910807799295, 17.42297078648622843, -222.0178620725767757 ) ) ;
#13976=CARTESIAN_POINT ( 'NONE',  ( -13.66944713747931139, -25.56883467164384527, -222.3908458502962731 ) ) ;
#13983=CARTESIAN_POINT ( 'NONE',  ( -15.15469129103955304, 15.56563882170958024, -231.6314069158229643 ) ) ;
#13984=CARTESIAN_POINT ( 'NONE',  ( 20.82555317450757215, 14.06078233701296476, -215.4201375757437802 ) ) ;
#13985=CARTESIAN_POINT ( 'NONE',  ( -26.02440924314744919, 2.824604386891162111, -232.0644005296583430 ) ) ;
#13986=CARTESIAN_POINT ( 'NONE',  ( -25.88730550323791491, -2.172607277783750845, -234.4881349215252726 ) ) ;
#13988=CARTESIAN_POINT ( 'NONE',  ( -15.34124043857492303, -4.213426711746545372, -218.8308339851419078 ) ) ;
#13990=CARTESIAN_POINT ( 'NONE',  ( -7.399925907206128528, 10.29859031525428037, -227.1614041762800298 ) ) ;
#13991=CARTESIAN_POINT ( 'NONE',  ( -7.531388159411753769, -21.98719092781708540, -216.0713624712111312 ) ) ;
#13992=CARTESIAN_POINT ( 'NONE',  ( 5.069241901512100412, 14.34986542013820632, -229.6420000777802954 ) ) ;
#13993=CARTESIAN_POINT ( 'NONE',  ( 9.163585743560105357, -20.90777124155954425, -214.7369711139705259 ) ) ;
#13994=CARTESIAN_POINT ( 'NONE',  ( -28.42127686227592420, -0.6461176296494712812, -221.6028628238154567 ) ) ;
#13995=CARTESIAN_POINT ( 'NONE',  ( -16.27882490622757672, 1.520697279646460398, -219.2607721384596289 ) ) ;
#13997=CARTESIAN_POINT ( 'NONE',  ( -2.532949683519015949, 17.18298404079579100, -229.0924323441805086 ) ) ;
#13998=CARTESIAN_POINT ( 'NONE',  ( 13.98152565379061052, 2.156981915107639036, -230.5667344709999611 ) ) ;
#13999=CARTESIAN_POINT ( 'NONE',  ( -12.13692969104051400, -0.3108940857385004697, -222.6170402347994184 ) ) ;
#14000=CARTESIAN_POINT ( 'NONE',  ( 11.83256327006771969, 5.988634687709346593, -225.8999299265561831 ) ) ;
#14001=CARTESIAN_POINT ( 'NONE',  ( -3.624336683137088677, -15.65024371637965039, -218.6393395577867977 ) ) ;
#14002=CARTESIAN_POINT ( 'NONE',  ( 9.168912942254459963, 16.03578711007639157, -234.6923200900793347 ) ) ;
#14003=CARTESIAN_POINT ( 'NONE',  ( 16.07305932912010960, 0.9253679043337685872, -229.0409936706996064 ) ) ;
#14004=CARTESIAN_POINT ( 'NONE',  ( -14.99584720478923572, -27.01727836854440312, -219.7524089968786996 ) ) ;
#14005=CARTESIAN_POINT ( 'NONE',  ( -4.490213599459100813, 14.55066867058898694, -222.6488251579668827 ) ) ;
#14006=CARTESIAN_POINT ( 'NONE',  ( 10.70175380652492336, 7.370128018021000038, -224.3479584370086286 ) ) ;
#14007=CARTESIAN_POINT ( 'NONE',  ( -14.73155177304599306, -1.817590056890399763, -226.9769936995019748 ) ) ;
#14008=CARTESIAN_POINT ( 'NONE',  ( -15.37153448429513602, 5.014568651886798456, -224.5085656291724945 ) ) ;
#14009=CARTESIAN_POINT ( 'NONE',  ( -4.531689447889125866, 14.11317536318881416, -231.6806015375303502 ) ) ;
#14010=CARTESIAN_POINT ( 'NONE',  ( 16.10828274231666768, 3.530956590605524692, -220.6574330336208050 ) ) ;
#14012=CARTESIAN_POINT ( 'NONE',  ( 7.764422566766373990, -15.81008911711046672, -220.9836405809557220 ) ) ;
#14014=CARTESIAN_POINT ( 'NONE',  ( 5.133806223762193532, -16.42362916962670383, -230.4968203642818310 ) ) ;
#14015=CARTESIAN_POINT ( 'NONE',  ( -2.906906946766868227, 27.66682465340607422, -226.6559963821499082 ) ) ;
#14018=CARTESIAN_POINT ( 'NONE',  ( 13.69275646168278371, 8.674223198772375909, -220.8699857572541987 ) ) ;
#14019=CARTESIAN_POINT ( 'NONE',  ( 28.22932473237819551, -8.039268142081398949, -226.6539694142420558 ) ) ;
#14020=CARTESIAN_POINT ( 'NONE',  ( -16.39524763169126942, -10.97410814576847926, -232.9630882351523837 ) ) ;
#14021=CARTESIAN_POINT ( 'NONE',  ( 1.127544764349826867, -27.89617517048659323, -231.9509945439240823 ) ) ;
#14022=CARTESIAN_POINT ( 'NONE',  ( -5.764806379010653181, 14.19340719117484007, -223.8851086052821415 ) ) ;
#14024=CARTESIAN_POINT ( 'NONE',  ( 19.67070349224072956, 16.44307963282299312, -220.0378483479504439 ) ) ;
#14025=CARTESIAN_POINT ( 'NONE',  ( -15.66530208164916260, 23.23467148471576849, -218.1250122661128046 ) ) ;
#14026=CARTESIAN_POINT ( 'NONE',  ( -10.94147694953847250, 13.90730769817462864, -218.7797619932150042 ) ) ;
#14028=CARTESIAN_POINT ( 'NONE',  ( 7.772443558932104146, 25.24620711463332157, -231.7813173736589931 ) ) ;
#14029=CARTESIAN_POINT ( 'NONE',  ( -27.28038240442402440, 5.683827137705129040, -226.0726697751923382 ) ) ;
#14030=CARTESIAN_POINT ( 'NONE',  ( 13.49694890958685711, 2.186465430673721677, -228.8273158381700512 ) ) ;
#14031=CARTESIAN_POINT ( 'NONE',  ( 19.66153801111809685, -22.47763448259700780, -224.4992982350615023 ) ) ;
#14034=CARTESIAN_POINT ( 'NONE',  ( -6.201839134465864767, 11.37481922992157379, -223.7040893475979146 ) ) ;
#14035=CARTESIAN_POINT ( 'NONE',  ( 27.35305420947085153, -2.513179086165481912, -228.1718430395816881 ) ) ;
#14037=CARTESIAN_POINT ( 'NONE',  ( 22.18132842682159733, 5.591149267797686839, -232.0584733989884114 ) ) ;
#14038=CARTESIAN_POINT ( 'NONE',  ( -13.92046207272054303, -0.1600067567908077248, -224.5811699126800818 ) ) ;
#14039=CARTESIAN_POINT ( 'NONE',  ( 7.080148886126969465, -28.65852557119563926, -219.9679292432588227 ) ) ;
#14041=CARTESIAN_POINT ( 'NONE',  ( -8.501641725227710111, 25.47064987787527102, -217.3358698761548737 ) ) ;
#14042=CARTESIAN_POINT ( 'NONE',  ( -12.26337789213896201, 9.274758280606999250, -219.9806108963443876 ) ) ;
#14044=CARTESIAN_POINT ( 'NONE',  ( -16.63766460830045091, 5.158675778507696208, -232.1659425527909093 ) ) ;
#14045=CARTESIAN_POINT ( 'NONE',  ( -10.30161254035895091, -9.966167094494833734, -223.3409979381218875 ) ) ;
#14048=CARTESIAN_POINT ( 'NONE',  ( -27.82842955277035202, 11.70195273568964112, -227.9294339757464911 ) ) ;
#14049=CARTESIAN_POINT ( 'NONE',  ( 3.737366178615106893, -15.16223317163647621, -230.3303395318446292 ) ) ;
#14052=CARTESIAN_POINT ( 'NONE',  ( 20.90058474538433231, 18.60939544422136294, -225.8027644507526475 ) ) ;
#14053=CARTESIAN_POINT ( 'NONE',  ( -16.96626096607909417, 26.06638125783293347, -227.3272535207661349 ) ) ;
#14055=CARTESIAN_POINT ( 'NONE',  ( 15.54095364727189299, 10.52000078266145700, -230.2714373371992735 ) ) ;
#14056=CARTESIAN_POINT ( 'NONE',  ( -2.278185930139247084, -29.13041568434719863, -223.8160414879089046 ) ) ;
#14057=CARTESIAN_POINT ( 'NONE',  ( 13.45252989138277400, -0.3779036657139918098, -224.7462000225944792 ) ) ;
#14060=CARTESIAN_POINT ( 'NONE',  ( 1.656472371294090085, 27.29382523973669095, -230.4991099578876117 ) ) ;
#14061=CARTESIAN_POINT ( 'NONE',  ( -16.88145396433676027, 5.002512658926777434, -221.2364783498041731 ) ) ;
#14062=CARTESIAN_POINT ( 'NONE',  ( -23.49520248890869212, 11.82830312093803649, -233.3871405502527807 ) ) ;
#14063=CARTESIAN_POINT ( 'NONE',  ( -14.19990609618026056, -7.901335420714983293, -227.4892254059333823 ) ) ;
#14066=CARTESIAN_POINT ( 'NONE',  ( 27.16757474806794903, 2.676291341565463888, -220.8863403533574115 ) ) ;
#14067=CARTESIAN_POINT ( 'NONE',  ( -2.821634405314548566, -24.60373223977012458, -232.0829149086248435 ) ) ;
#14068=CARTESIAN_POINT ( 'NONE',  ( 13.43730899468209294, 8.427513769504761498, -221.4030804848920297 ) ) ;
#14069=CARTESIAN_POINT ( 'NONE',  ( -9.740348021262962064, 16.12529029871877384, -216.4361617420699702 ) ) ;
#14071=CARTESIAN_POINT ( 'NONE',  ( 27.08260752785270853, 4.114838227474355570, -232.2882281786467331 ) ) ;
#14072=CARTESIAN_POINT ( 'NONE',  ( 5.623554730548537606, 15.65270319720736225, -231.3185741195121068 ) ) ;
#14074=CARTESIAN_POINT ( 'NONE',  ( -8.257247207528708444, -26.39349301559143512, -217.9383130379005138 ) ) ;
#14075=CARTESIAN_POINT ( 'NONE',  ( 20.98776729843937972, -13.55153944770713359, -217.5092423276211946 ) ) ;
#14078=CARTESIAN_POINT ( 'NONE',  ( -13.91932826323387395, 8.983986115891950064, -216.4624824187541776 ) ) ;
#14079=CARTESIAN_POINT ( 'NONE',  ( 23.66932040738428356, 1.377632087272899541, -234.6098499860491415 ) ) ;
#14080=CARTESIAN_POINT ( 'NONE',  ( 21.17011458613547248, 1.652544727609948527, -234.6098499860487152 ) ) ;
#14081=CARTESIAN_POINT ( 'NONE',  ( 1.939863782649466017, 28.20584428268631783, -229.4487744520996273 ) ) ;
#14082=CARTESIAN_POINT ( 'NONE',  ( 5.248013545904832711, 18.51731616863089158, -219.3673127389703552 ) ) ;
#14084=CARTESIAN_POINT ( 'NONE',  ( 13.86864723624500328, -7.301706307425273046, -233.2436966314882909 ) ) ;
#14086=CARTESIAN_POINT ( 'NONE',  ( 24.03642272140365677, 3.646960756862087205, -218.2320643939070806 ) ) ;
#14087=CARTESIAN_POINT ( 'NONE',  ( -17.20794623181132721, 21.97849129791581291, -217.9187454682870850 ) ) ;
#14088=CARTESIAN_POINT ( 'NONE',  ( -16.88427011841620029, 9.219900108593305887, -231.9155403335099948 ) ) ;
#14089=CARTESIAN_POINT ( 'NONE',  ( -15.33992272861872763, -7.600289318192222865, -231.6130094852651951 ) ) ;
#14090=CARTESIAN_POINT ( 'NONE',  ( -11.46843428684449151, 6.508406145394057596, -225.7212143570321814 ) ) ;
#14094=CARTESIAN_POINT ( 'NONE',  ( 12.88374853655145458, 4.106359831454843068, -228.1016120772327440 ) ) ;
#14096=CARTESIAN_POINT ( 'NONE',  ( -13.41250421226414069, 17.27419134292087577, -217.6844171132545966 ) ) ;
#14097=CARTESIAN_POINT ( 'NONE',  ( 15.79748369401691122, 19.19631269170049137, -215.0096632418193963 ) ) ;
#14098=CARTESIAN_POINT ( 'NONE',  ( -13.10651848559790444, 3.262242204071156948, -224.3513854875720597 ) ) ;
#14099=CARTESIAN_POINT ( 'NONE',  ( -22.78031074599627814, -9.151179398885634697, -235.0532497368941733 ) ) ;
#14101=CARTESIAN_POINT ( 'NONE',  ( -19.18273340400098448, -14.85130345181434741, -232.7114379411565039 ) ) ;
#14103=CARTESIAN_POINT ( 'NONE',  ( -12.38801939673351704, 9.361418580567464787, -232.8075769614211765 ) ) ;
#14104=CARTESIAN_POINT ( 'NONE',  ( -8.258403559667634397, -29.80786866836635696, -223.3983869762195127 ) ) ;
#14105=CARTESIAN_POINT ( 'NONE',  ( 4.354034006296288339, 14.09944204372416188, -221.2519525881239417 ) ) ;
#14106=CARTESIAN_POINT ( 'NONE',  ( 11.14866046433140490, -17.10865642060806024, -235.2771047445726822 ) ) ;
#14107=CARTESIAN_POINT ( 'NONE',  ( -27.09167109716269550, -0.2825935922571593539, -219.8389404328913486 ) ) ;
#14108=CARTESIAN_POINT ( 'NONE',  ( -18.04772061096520375, 5.916925414182395038, -217.8829197293425750 ) ) ;
#14110=CARTESIAN_POINT ( 'NONE',  ( -9.106229537879125147, 25.89784491087598184, -228.9807674929363372 ) ) ;
#14111=CARTESIAN_POINT ( 'NONE',  ( -28.31595744342370580, 5.786754998807587924, -229.0820962600229223 ) ) ;
#14113=CARTESIAN_POINT ( 'NONE',  ( 26.29894631880581812, 12.29609390142961090, -226.3100047295820332 ) ) ;
#14114=CARTESIAN_POINT ( 'NONE',  ( 14.55590852435181226, 2.816890518231522034, -218.5131513550309990 ) ) ;
#14115=CARTESIAN_POINT ( 'NONE',  ( -15.44264673875841432, -21.96030778071044054, -219.6531968376115174 ) ) ;
#14117=CARTESIAN_POINT ( 'NONE',  ( 6.550054208186137039, 12.38618022562281595, -231.5087189857719068 ) ) ;
#14119=CARTESIAN_POINT ( 'NONE',  ( -13.66010072360327676, -23.28416639572314750, -215.9262288161416166 ) ) ;
#14120=CARTESIAN_POINT ( 'NONE',  ( -4.080659539198054020, 15.43130099126780408, -228.8058965243247656 ) ) ;
#14121=CARTESIAN_POINT ( 'NONE',  ( 8.554868430186942874, 10.42313681336814568, -223.0114508542762621 ) ) ;
#14123=CARTESIAN_POINT ( 'NONE',  ( -15.82068653568960137, 8.372322471091806051, -220.7139663195713979 ) ) ;
#14124=CARTESIAN_POINT ( 'NONE',  ( -0.04850409037381671340, 14.20520396026658716, -231.8092226852533031 ) ) ;
#14125=CARTESIAN_POINT ( 'NONE',  ( 24.78377098693636427, 3.871650763546384155, -231.3521132786341923 ) ) ;
#14127=CARTESIAN_POINT ( 'NONE',  ( 13.12950778469841318, -23.99547238938880511, -222.5250877844293029 ) ) ;
#14129=CARTESIAN_POINT ( 'NONE',  ( 19.57710422433000019, -21.48596639614413562, -228.6055549924913635 ) ) ;
#14130=CARTESIAN_POINT ( 'NONE',  ( -2.554014161526931392, 17.56271496069470572, -229.4905841158208659 ) ) ;
#14132=CARTESIAN_POINT ( 'NONE',  ( 22.02796522526679723, 16.41909032291435366, -220.1590600991317217 ) ) ;
#14133=CARTESIAN_POINT ( 'NONE',  ( -30.56371166594826150, 0.09613004385584933420, -226.3268674980304525 ) ) ;
#14134=CARTESIAN_POINT ( 'NONE',  ( -21.52428768452188734, -21.65989873160339840, -225.4304055049964006 ) ) ;
#14135=CARTESIAN_POINT ( 'NONE',  ( 6.589392574981438599, -17.08498810221841069, -232.9613445306918322 ) ) ;
#14136=CARTESIAN_POINT ( 'NONE',  ( -8.881241380679488984, 27.18697625135247975, -224.4474391433207927 ) ) ;
#14138=CARTESIAN_POINT ( 'NONE',  ( 20.59763700141659015, 7.383112456150029423, -232.0722244125682039 ) ) ;
#14139=CARTESIAN_POINT ( 'NONE',  ( -9.540790481621398200, 9.981116473660406996, -228.6478862620407995 ) ) ;
#14140=CARTESIAN_POINT ( 'NONE',  ( -3.926352947695993745, 17.69140300707508473, -220.1607884481205986 ) ) ;
#14144=CARTESIAN_POINT ( 'NONE',  ( 7.450672702945051462, 17.42371045663376705, -217.2894981592719432 ) ) ;
#14145=CARTESIAN_POINT ( 'NONE',  ( -18.94009481283715957, 3.115208415279245191, -230.3622730452590588 ) ) ;
#14146=CARTESIAN_POINT ( 'NONE',  ( 13.70863938672594529, 6.616599615120571265, -232.1343637516268643 ) ) ;
#14147=CARTESIAN_POINT ( 'NONE',  ( 12.20621255000322947, -21.57429421806300240, -232.1397031738524674 ) ) ;
#14148=CARTESIAN_POINT ( 'NONE',  ( 18.40125535140034430, 0.01434342441762339639, -233.2485400239426099 ) ) ;
#14150=CARTESIAN_POINT ( 'NONE',  ( 7.769483725421269860, 20.68783433326350263, -233.2348178266662728 ) ) ;
#14151=CARTESIAN_POINT ( 'NONE',  ( 22.49864633775863609, -6.670857247392108391, -230.7634588385486438 ) ) ;
#14153=CARTESIAN_POINT ( 'NONE',  ( 14.80394259695730064, 1.224172658189580432, -225.4564070658925061 ) ) ;
#14154=CARTESIAN_POINT ( 'NONE',  ( 1.799766247726228174, -14.75051420185460849, -230.6199496058247291 ) ) ;
#14156=CARTESIAN_POINT ( 'NONE',  ( -18.39892766464214446, 25.11039525536027739, -225.3444503920457294 ) ) ;
#14158=CARTESIAN_POINT ( 'NONE',  ( -9.251743101293765648, 14.06372330290396278, -232.4239003576353468 ) ) ;
#14160=CARTESIAN_POINT ( 'NONE',  ( -15.82069055112642353, 8.315535108674763976, -217.2800172218543935 ) ) ;
#14161=CARTESIAN_POINT ( 'NONE',  ( -14.31049420963804586, -8.435107166214018903, -218.7432863707801403 ) ) ;
#14165=CARTESIAN_POINT ( 'NONE',  ( -14.68037037322036475, 3.441677802729143920, -220.1396515630443389 ) ) ;
#14166=CARTESIAN_POINT ( 'NONE',  ( 6.028509222145709501, -20.27756025184508815, -216.6192952284833950 ) ) ;
#14168=CARTESIAN_POINT ( 'NONE',  ( 25.53003411612920459, 7.940385729200389875, -230.5495695598654322 ) ) ;
#14169=CARTESIAN_POINT ( 'NONE',  ( -15.64710113362562183, 25.90300453978063189, -220.8637308366217269 ) ) ;
#14171=CARTESIAN_POINT ( 'NONE',  ( 10.73846460100926592, 12.62787417135106161, -222.6344468496098159 ) ) ;
#14172=CARTESIAN_POINT ( 'NONE',  ( -0.6326494355537284342, -15.87741594504987219, -229.6822519216137266 ) ) ;
#14174=CARTESIAN_POINT ( 'NONE',  ( -0.7041916573665241152, 14.60214745152014437, -226.3818583194645555 ) ) ;
#14175=CARTESIAN_POINT ( 'NONE',  ( -18.09605518090995702, 22.22778748761825085, -222.5443354630425290 ) ) ;
#14176=CARTESIAN_POINT ( 'NONE',  ( -22.57344584932824105, 14.14390280519600473, -217.2212543695777924 ) ) ;
#14177=CARTESIAN_POINT ( 'NONE',  ( -13.89163392164661204, -16.46234366268243221, -230.8566716434345949 ) ) ;
#14181=CARTESIAN_POINT ( 'NONE',  ( 21.92281339924938877, 16.67475415235398017, -231.9828670874568957 ) ) ;
#14182=CARTESIAN_POINT ( 'NONE',  ( 7.033108278341462238, -17.71891568601925826, -230.1509483552532060 ) ) ;
#14183=CARTESIAN_POINT ( 'NONE',  ( 21.39553407250273054, 8.453402029343234148, -217.9531594780983141 ) ) ;
#14184=CARTESIAN_POINT ( 'NONE',  ( -10.65455960636934662, 10.37188583052882862, -219.5197110153079620 ) ) ;
#14185=CARTESIAN_POINT ( 'NONE',  ( 29.08100487150598212, 12.14819438347179670, -226.9621620069135020 ) ) ;
#14187=CARTESIAN_POINT ( 'NONE',  ( 11.82943521288609823, 27.58963564415041247, -226.1180395413371400 ) ) ;
#14189=CARTESIAN_POINT ( 'NONE',  ( -14.84823930505322132, -23.35465403802561823, -218.3226235040776260 ) ) ;
#14190=CARTESIAN_POINT ( 'NONE',  ( 17.02763684969102798, -14.67205317233652195, -233.2001291093645818 ) ) ;
#14194=CARTESIAN_POINT ( 'NONE',  ( -13.58389614404818069, 15.11490620317918676, -215.3922994348461941 ) ) ;
#14195=CARTESIAN_POINT ( 'NONE',  ( -21.01940116658287749, -3.333607517048045032, -230.8803659671980597 ) ) ;
#14196=CARTESIAN_POINT ( 'NONE',  ( -20.97727766418175932, 9.381545086430262970, -232.5968905491617420 ) ) ;
#14197=CARTESIAN_POINT ( 'NONE',  ( 8.903385417657583289, 10.41040586594612272, -227.6527940987422198 ) ) ;
#14198=CARTESIAN_POINT ( 'NONE',  ( 5.195682580001069084, 14.86321519495278665, -224.7851167466743334 ) ) ;
#14200=CARTESIAN_POINT ( 'NONE',  ( 20.62543286083822380, -24.26207512693059343, -224.4080524747341201 ) ) ;
#14202=CARTESIAN_POINT ( 'NONE',  ( 14.95414693437772868, 8.262206471704862665, -230.1862972580043163 ) ) ;
#14203=CARTESIAN_POINT ( 'NONE',  ( -23.89856910807799295, 17.42297078648622843, -222.0178620725767757 ) ) ;
#14204=CARTESIAN_POINT ( 'NONE',  ( -9.251743101293765648, 14.06372330290396278, -232.4239003576353468 ) ) ;
#14205=CARTESIAN_POINT ( 'NONE',  ( -23.85568197540453994, -15.41036827548725618, -219.8503866864575969 ) ) ;
#14206=CARTESIAN_POINT ( 'NONE',  ( -22.17339560624464312, 16.26550580028390769, -232.0582861498566274 ) ) ;
#14208=CARTESIAN_POINT ( 'NONE',  ( 17.22423229049764970, 1.395540479540137380, -217.3898520248025363 ) ) ;
#14210=CARTESIAN_POINT ( 'NONE',  ( -10.24168223636446662, 16.14271751156598356, -231.4847994864913971 ) ) ;
#14211=CARTESIAN_POINT ( 'NONE',  ( 9.168912942254459963, 16.03578711007639157, -234.6923200900793347 ) ) ;
#14212=CARTESIAN_POINT ( 'NONE',  ( -15.23434562258889891, -0.4010941804143903222, -220.4743703065900036 ) ) ;
#14213=CARTESIAN_POINT ( 'NONE',  ( -12.22852564478610482, -7.025360622849957437, -222.3415469712626589 ) ) ;
#14214=CARTESIAN_POINT ( 'NONE',  ( 2.601379523478754674, 17.36677895276155681, -230.4357129074444117 ) ) ;
#14215=CARTESIAN_POINT ( 'NONE',  ( -1.890995374385051608, -13.09686096954197509, -227.5694739903412085 ) ) ;
#14216=CARTESIAN_POINT ( 'NONE',  ( 7.762960416026701616, 12.60702317161859121, -221.9096828323375235 ) ) ;
#14217=CARTESIAN_POINT ( 'NONE',  ( 22.52555938611480002, -22.70209057424856525, -227.7033606670069332 ) ) ;
#14220=CARTESIAN_POINT ( 'NONE',  ( 17.41909632439413969, 2.006477695503792624, -233.4081875040758121 ) ) ;
#14221=FILL_AREA_STYLE_COLOUR ( '', #7057 ) ;
#14222=CARTESIAN_POINT ( 'NONE',  ( 26.86480837698434243, -8.606671353193281249, -231.2046318962545683 ) ) ;
#14223=CARTESIAN_POINT ( 'NONE',  ( 7.017641603801325623, 14.96204511409594673, -228.1064041248110073 ) ) ;
#14224=CARTESIAN_POINT ( 'NONE',  ( 21.27683256847563698, 4.223177115764435108, -215.2584548172064842 ) ) ;
#14225=CARTESIAN_POINT ( 'NONE',  ( 19.20300624114736721, 0.6066039755357417462, -231.5046416827383950 ) ) ;
#14226=CARTESIAN_POINT ( 'NONE',  ( -14.02540557227298024, -18.71004003062420651, -218.0769645724313932 ) ) ;
#14229=CARTESIAN_POINT ( 'NONE',  ( 2.892356176081334773, 24.03953794589038395, -215.3901262983647200 ) ) ;
#14231=CARTESIAN_POINT ( 'NONE',  ( -6.183400735100206269, -24.17720054222102277, -215.4627583112813625 ) ) ;
#14232=CARTESIAN_POINT ( 'NONE',  ( -10.91003322996498071, 12.84665145358222382, -229.9786893781767958 ) ) ;
#14234=CARTESIAN_POINT ( 'NONE',  ( 5.803912621764987456, 13.01725692290267844, -221.8367675400179166 ) ) ;
#14235=CARTESIAN_POINT ( 'NONE',  ( -20.92673740658815973, 5.672885432599523270, -219.1433548642331459 ) ) ;
#14236=CARTESIAN_POINT ( 'NONE',  ( 0.9169988354999972779, 20.59043933275470550, -235.2854195559275752 ) ) ;
#14237=CARTESIAN_POINT ( 'NONE',  ( 19.29259174080182504, 0.5828707127177102931, -219.2781652733668807 ) ) ;
#14238=CARTESIAN_POINT ( 'NONE',  ( 9.638496285600583136, -13.08983061985817464, -223.8709389748426588 ) ) ;
#14241=CARTESIAN_POINT ( 'NONE',  ( 10.05661706967825353, -14.25456047934742365, -218.9909083857680230 ) ) ;
#14242=CARTESIAN_POINT ( 'NONE',  ( -1.364406401035816785, 24.33111505239456918, -219.5658712396381418 ) ) ;
#14245=CARTESIAN_POINT ( 'NONE',  ( 25.80927844399814930, 11.21489550116160316, -221.3538377621514996 ) ) ;
#14246=CARTESIAN_POINT ( 'NONE',  ( -26.73251495235368225, -0.6309583860051256599, -232.5016102969711085 ) ) ;
#14247=CARTESIAN_POINT ( 'NONE',  ( -18.89430729770302975, -12.42271633246521212, -233.2230176520695295 ) ) ;
#14248=CARTESIAN_POINT ( 'NONE',  ( -8.379125946468517938, -29.31735857037017468, -221.8060643354269814 ) ) ;
#14249=CARTESIAN_POINT ( 'NONE',  ( -9.106229537879125147, 25.89784491087598184, -228.9807674929363372 ) ) ;
#14251=CARTESIAN_POINT ( 'NONE',  ( 15.54095364727189299, 10.52000078266145700, -230.2714373371992735 ) ) ;
#14252=CARTESIAN_POINT ( 'NONE',  ( -8.172572110426221670, 16.86653848210977813, -233.4220330256369493 ) ) ;
#14253=CARTESIAN_POINT ( 'NONE',  ( -13.40354389326479456, 23.35336998323175450, -219.8517474526506987 ) ) ;
#14256=CARTESIAN_POINT ( 'NONE',  ( 1.104227501629593045, 25.05528885094460989, -231.9808705443460326 ) ) ;
#14257=CARTESIAN_POINT ( 'NONE',  ( -25.17056316833229701, 11.10725809642625705, -227.0225660235207386 ) ) ;
#14258=CARTESIAN_POINT ( 'NONE',  ( 12.71499452845021416, 2.172589307656224378, -223.9381607050773084 ) ) ;
#14259=CARTESIAN_POINT ( 'NONE',  ( 6.755953262402430326, -28.44658494672641424, -224.7309905328439754 ) ) ;
#14261=CARTESIAN_POINT ( 'NONE',  ( 21.04928763009552384, -0.2309942901367783852, -233.9427286327411366 ) ) ;
#14263=CARTESIAN_POINT ( 'NONE',  ( 10.85888002857596923, 15.81835858589122878, -232.3913150909872627 ) ) ;
#14264=CARTESIAN_POINT ( 'NONE',  ( 27.03411061974195562, -3.460823241630351710, -221.7771387205989413 ) ) ;
#14265=CARTESIAN_POINT ( 'NONE',  ( 15.09054553479285588, -1.912330756057289527, -222.3157747520536702 ) ) ;
#14267=CARTESIAN_POINT ( 'NONE',  ( 10.30328786010431052, -20.08430705480546408, -216.1847100135515802 ) ) ;
#14268=CARTESIAN_POINT ( 'NONE',  ( -19.00318367631585659, 13.14621133775862916, -233.8403879275295765 ) ) ;
#14270=CARTESIAN_POINT ( 'NONE',  ( -9.578110717394128670, 23.64032677849093034, -215.7669555765890550 ) ) ;
#14272=CARTESIAN_POINT ( 'NONE',  ( -11.69688825528096388, 18.63404371591177622, -215.8612738028812714 ) ) ;
#14273=CARTESIAN_POINT ( 'NONE',  ( -11.96453848309674228, -6.796862595549911568, -223.8262896469332759 ) ) ;
#14276=CARTESIAN_POINT ( 'NONE',  ( -16.74550766701807447, 3.787526820511904813, -217.9802846976114381 ) ) ;
#14277=CARTESIAN_POINT ( 'NONE',  ( 0.5037192024386412115, -21.28831724695581684, -215.7417742237681466 ) ) ;
#14278=CARTESIAN_POINT ( 'NONE',  ( 23.74723497152361062, 5.524508269105988134, -217.6012181427065002 ) ) ;
#14279=CARTESIAN_POINT ( 'NONE',  ( -23.70973587455150522, 20.45398817402440983, -228.9005348699235469 ) ) ;
#14281=CARTESIAN_POINT ( 'NONE',  ( 12.51085646230496273, 9.582567546749562126, -224.6200301875240939 ) ) ;
#14282=CARTESIAN_POINT ( 'NONE',  ( 5.681636183907174065, -27.87860296351749767, -230.4665658140699804 ) ) ;
#14284=CARTESIAN_POINT ( 'NONE',  ( 3.219568897812384645, 28.82511222849302257, -221.5626884747494216 ) ) ;
#14285=CARTESIAN_POINT ( 'NONE',  ( -11.69222874857179484, 25.57550432052970280, -219.9467848335519591 ) ) ;
#14286=CARTESIAN_POINT ( 'NONE',  ( -15.00242079508237936, 7.335218745534954898, -232.9526071471669013 ) ) ;
#14288=CARTESIAN_POINT ( 'NONE',  ( -12.03049011398204726, -11.12540611457240480, -223.2385418847515268 ) ) ;
#14291=CARTESIAN_POINT ( 'NONE',  ( -17.84981083811007707, 0.8485253248287054628, -231.8041300026935119 ) ) ;
#14292=CARTESIAN_POINT ( 'NONE',  ( 0.5598654370342924791, -17.79304497667748564, -219.0037976856824571 ) ) ;
#14293=CARTESIAN_POINT ( 'NONE',  ( 17.60676319847677007, 21.31475060840986302, -219.8266339603936785 ) ) ;
#14294=CARTESIAN_POINT ( 'NONE',  ( 4.389496648589924277, 14.47660514356954131, -220.6151178996808540 ) ) ;
#14296=CARTESIAN_POINT ( 'NONE',  ( 15.87399429023076003, -1.683916961781461552, -230.8621029165058758 ) ) ;
#14297=CARTESIAN_POINT ( 'NONE',  ( 4.343013938751969505, 13.02036404005131587, -224.7825435359082178 ) ) ;
#14299=CARTESIAN_POINT ( 'NONE',  ( -10.42804209284631156, -14.08702332024887305, -217.7386024361820489 ) ) ;
#14300=CARTESIAN_POINT ( 'NONE',  ( 14.18709644517307922, -11.45356969546147496, -232.2178450427173004 ) ) ;
#14303=CARTESIAN_POINT ( 'NONE',  ( -16.38161496430853248, 17.22219235543852989, -215.3343469598664797 ) ) ;
#14304=CARTESIAN_POINT ( 'NONE',  ( -21.95460872137175201, -8.074699112730320039, -230.7190249947325071 ) ) ;
#14305=CARTESIAN_POINT ( 'NONE',  ( -13.37045227479810094, 5.250293981428504786, -224.2914120185227205 ) ) ;
#14306=CARTESIAN_POINT ( 'NONE',  ( 15.88043104796248528, 11.88135572392608807, -216.2525917828042168 ) ) ;
#14307=CARTESIAN_POINT ( 'NONE',  ( -2.117958212721558375, 27.20243410318316535, -230.7086725634165418 ) ) ;
#14309=CARTESIAN_POINT ( 'NONE',  ( 10.59985392024617745, -10.68425835910226418, -232.2123170752960277 ) ) ;
#14310=CARTESIAN_POINT ( 'NONE',  ( 26.48990917286906921, 12.16675355942207659, -225.0153622588060216 ) ) ;
#14311=CARTESIAN_POINT ( 'NONE',  ( -2.577721557973523314, 25.83760098923793791, -215.4660676095525389 ) ) ;
#14313=CARTESIAN_POINT ( 'NONE',  ( -13.25293905438448405, 17.39325876214774524, -215.6628841494472510 ) ) ;
#14314=CARTESIAN_POINT ( 'NONE',  ( -13.36955836198420577, -3.222265253903016990, -227.4060678739157026 ) ) ;
#14315=CARTESIAN_POINT ( 'NONE',  ( -9.250876228778270871, 9.538614635316015722, -227.1332118982684563 ) ) ;
#14317=CARTESIAN_POINT ( 'NONE',  ( 17.95694455891925756, -3.510678534943489026, -231.2643001502910067 ) ) ;
#14318=CARTESIAN_POINT ( 'NONE',  ( -12.70465517376339193, 12.03139199664008530, -229.6235454691090752 ) ) ;
#14319=CARTESIAN_POINT ( 'NONE',  ( -18.93763370444446181, -0.7340653299870684156, -219.7345063954518594 ) ) ;
#14320=CARTESIAN_POINT ( 'NONE',  ( 28.62253243811995418, 3.652502539191337494, -225.4068779441649326 ) ) ;
#14321=CARTESIAN_POINT ( 'NONE',  ( 15.91295838535984331, 21.88410254487826379, -230.9583961155862823 ) ) ;
#14322=CARTESIAN_POINT ( 'NONE',  ( -12.65123680455331190, -6.798726433138870817, -228.2089845657881710 ) ) ;
#14324=CARTESIAN_POINT ( 'NONE',  ( 0.7903203334012884884, 21.30772501796948859, -217.9064416298261619 ) ) ;
#14325=CARTESIAN_POINT ( 'NONE',  ( -3.300598509645395584, -18.18730530649546395, -233.4303386612170925 ) ) ;
#14326=CARTESIAN_POINT ( 'NONE',  ( 18.23324537670537993, 23.47692953258263771, -224.8333321331434433 ) ) ;
#14327=CARTESIAN_POINT ( 'NONE',  ( 5.002389762228888870, -13.81148461055073362, -218.0662212534467983 ) ) ;
#14328=DIRECTION ( 'NONE',  ( 0.03647168421188083653, 0.3315607655626302552, 0.9427286327412950362 ) ) ;
#14329=CARTESIAN_POINT ( 'NONE',  ( -10.16319438574952372, 11.71174522937666040, -227.8434026503654479 ) ) ;
#14330=CARTESIAN_POINT ( 'NONE',  ( 24.64273247744971229, -10.07127014888436278, -217.7281412196979602 ) ) ;
#14331=CARTESIAN_POINT ( 'NONE',  ( 3.060417506408009469, 27.46204888741655026, -226.6022202862033623 ) ) ;
#14332=CARTESIAN_POINT ( 'NONE',  ( -18.94992041651601156, 14.87246523864368974, -232.0280096192260828 ) ) ;
#14333=CARTESIAN_POINT ( 'NONE',  ( -20.87212828950092813, -0.8819659211619411687, -215.0000000018925448 ) ) ;
#14335=CARTESIAN_POINT ( 'NONE',  ( -13.33153391309230074, -13.53657406488594184, -231.3594229707590557 ) ) ;
#14336=CARTESIAN_POINT ( 'NONE',  ( 15.65443801613259467, 7.488839228060037989, -233.6469817377710569 ) ) ;
#14338=CARTESIAN_POINT ( 'NONE',  ( 0.3570725323625942860, -15.31465789365257102, -218.3993834748477525 ) ) ;
#14339=CARTESIAN_POINT ( 'NONE',  ( 10.25948093768852054, 28.38842464930171872, -224.3436940787075855 ) ) ;
#14340=CARTESIAN_POINT ( 'NONE',  ( 10.95881707662767290, 12.06788758096456782, -231.4359029166177208 ) ) ;
#14342=CARTESIAN_POINT ( 'NONE',  ( -13.14888680331901583, 26.03314517226533908, -227.7900104434697539 ) ) ;
#14344=CARTESIAN_POINT ( 'NONE',  ( -5.467362224022371819, 23.92882567691090046, -234.7811165710531611 ) ) ;
#14345=CARTESIAN_POINT ( 'NONE',  ( 27.50364976068844669, 3.973406265104437729, -228.8805639113908228 ) ) ;
#14347=CARTESIAN_POINT ( 'NONE',  ( 11.43327405580198608, -14.46863304034511799, -220.4355838810013495 ) ) ;
#14349=CARTESIAN_POINT ( 'NONE',  ( 9.037704487505543227, -20.74919929927824214, -217.6023494967207625 ) ) ;
#14350=CARTESIAN_POINT ( 'NONE',  ( -3.926352947695993745, 17.69140300707508473, -220.1607884481205986 ) ) ;
#14352=CARTESIAN_POINT ( 'NONE',  ( 15.52719855059926424, 1.633696074270991172, -221.7349885876216433 ) ) ;
#14353=CARTESIAN_POINT ( 'NONE',  ( 23.48720700658024896, -2.145453947144424500, -217.8824464111000054 ) ) ;
#14354=CARTESIAN_POINT ( 'NONE',  ( -11.36971918743327237, -8.287084598727400220, -223.1364763414170227 ) ) ;
#14355=CARTESIAN_POINT ( 'NONE',  ( 8.115778909262310492, -29.92983049028717346, -224.5060555478150377 ) ) ;
#14356=CARTESIAN_POINT ( 'NONE',  ( 3.614175329767659761, 21.98488100320606264, -219.0898850257099753 ) ) ;
#14358=CARTESIAN_POINT ( 'NONE',  ( -15.64716994811699813, 6.210654946517923491, -217.0002936794128345 ) ) ;
#14359=CARTESIAN_POINT ( 'NONE',  ( -12.90983082593748676, 14.84936372681532823, -233.8009687022269532 ) ) ;
#14360=CARTESIAN_POINT ( 'NONE',  ( -2.554014161526931392, 17.56271496069470572, -229.4905841158208659 ) ) ;
#14362=CARTESIAN_POINT ( 'NONE',  ( 23.44028133050380802, 19.87677100428751231, -223.1503774981096342 ) ) ;
#14363=CARTESIAN_POINT ( 'NONE',  ( -15.15469129103955304, 15.56563882170958024, -231.6314069158229643 ) ) ;
#14364=CARTESIAN_POINT ( 'NONE',  ( 30.65249971456167799, 3.724008896938769464, -225.4815109119605552 ) ) ;
#14365=CARTESIAN_POINT ( 'NONE',  ( -1.097449620509919788, -25.21235133823365260, -218.6697740411501059 ) ) ;
#14368=CARTESIAN_POINT ( 'NONE',  ( 4.340445191644851874, 29.86837761166362881, -227.4879512554873315 ) ) ;
#14369=CARTESIAN_POINT ( 'NONE',  ( -31.58308234758948174, -0.5371106682196264970, -221.7519263543700845 ) ) ;
#14371=CARTESIAN_POINT ( 'NONE',  ( -0.1947256686167265494, -30.94043057420685727, -223.1178397439027492 ) ) ;
#14372=PRODUCT_CONTEXT ( 'NONE', #6851, 'mechanical' ) ;
#14373=CARTESIAN_POINT ( 'NONE',  ( -10.51143808951550085, 11.41308718311005066, -231.3573069600382439 ) ) ;
#14374=CARTESIAN_POINT ( 'NONE',  ( -7.403072389817287657, 18.92851032520892929, -215.2068968469505137 ) ) ;
#14376=CARTESIAN_POINT ( 'NONE',  ( -9.151299407007059017, 9.196974979111923076, -223.9483834032048719 ) ) ;
#14377=CARTESIAN_POINT ( 'NONE',  ( -24.78729321827560739, -16.46449136890227294, -222.3867555963062443 ) ) ;
#14380=CARTESIAN_POINT ( 'NONE',  ( -18.47334320050258327, 24.79293862780133040, -226.9986786077537317 ) ) ;
#14381=CARTESIAN_POINT ( 'NONE',  ( 3.568716337251232051, -21.91366830329386772, -233.6537821856145172 ) ) ;
#14383=CARTESIAN_POINT ( 'NONE',  ( -22.99617382825321599, 17.18101613848176967, -230.9512687019100099 ) ) ;
#14384=CARTESIAN_POINT ( 'NONE',  ( 20.22510869507564024, 17.05975164568011238, -220.7829296213589316 ) ) ;
#14386=CARTESIAN_POINT ( 'NONE',  ( 5.365126951644291431, 19.60085171667039816, -218.9155869426879519 ) ) ;
#14388=CARTESIAN_POINT ( 'NONE',  ( 14.40184562439531213, 6.414772937171507650, -227.4651811604036595 ) ) ;
#14389=CARTESIAN_POINT ( 'NONE',  ( -14.65844530258765310, -17.20867344037294444, -230.8340913472024170 ) ) ;
#14392=CARTESIAN_POINT ( 'NONE',  ( -0.5888410438786807477, 14.99789765555501475, -227.7044550383138244 ) ) ;
#14393=CARTESIAN_POINT ( 'NONE',  ( -11.55316006017064012, 19.79513644261079719, -232.3088878043970453 ) ) ;
#14394=CARTESIAN_POINT ( 'NONE',  ( -8.112279890008961658, 11.99566605360304727, -225.9834628568286519 ) ) ;
#14395=CARTESIAN_POINT ( 'NONE',  ( -20.35224420216377439, -13.00389602580315085, -219.1266045330881980 ) ) ;
#14398=CARTESIAN_POINT ( 'NONE',  ( -15.23434562258889891, -0.4010941804143903222, -220.4743703065900036 ) ) ;
#14399=CARTESIAN_POINT ( 'NONE',  ( -0.6467335922136470128, -17.26771294536504442, -230.4732896975262122 ) ) ;
#14400=CARTESIAN_POINT ( 'NONE',  ( 12.85408565574548412, 7.821283853063205171, -223.1248833997948111 ) ) ;
#14401=CARTESIAN_POINT ( 'NONE',  ( 0.7245137624042983227, 13.44764381486384330, -223.4043886706536455 ) ) ;
#14403=CARTESIAN_POINT ( 'NONE',  ( -15.12838653695630420, 3.161599240781852949, -225.7834014684609656 ) ) ;
#14404=CARTESIAN_POINT ( 'NONE',  ( 12.56362091610784049, 9.747446748398973071, -231.6428467497164547 ) ) ;
#14405=CARTESIAN_POINT ( 'NONE',  ( 13.43730899468209294, 8.427513769504761498, -221.4030804848920297 ) ) ;
#14407=CARTESIAN_POINT ( 'NONE',  ( -15.74157322273402748, -13.22745315869835636, -216.7831660370879661 ) ) ;
#14408=CARTESIAN_POINT ( 'NONE',  ( 2.178520447619924472, -13.56847537563065487, -221.4085897031499428 ) ) ;
#14411=CARTESIAN_POINT ( 'NONE',  ( -11.10543627608095285, 3.497967533612860613, -224.1342318769322617 ) ) ;
#14412=CARTESIAN_POINT ( 'NONE',  ( 18.88835481822873774, -3.841660717124094848, -234.8883833189080974 ) ) ;
#14413=CARTESIAN_POINT ( 'NONE',  ( 14.69853173970351179, 23.44775873627089524, -231.2711109634281001 ) ) ;
#14414=CARTESIAN_POINT ( 'NONE',  ( 8.162622027327667951, 13.88735946031204094, -224.7165241036068153 ) ) ;
#14416=CARTESIAN_POINT ( 'NONE',  ( 11.82206472115893447, -5.594380913675770728, -219.9420363600394239 ) ) ;
#14417=CARTESIAN_POINT ( 'NONE',  ( 17.99029889091409018, 9.613712288440757092, -232.0298403238024036 ) ) ;
#14418=CARTESIAN_POINT ( 'NONE',  ( -0.4465333940385243228, 12.27026616490476485, -221.3722328744566425 ) ) ;
#14419=CARTESIAN_POINT ( 'NONE',  ( -18.70090456008720992, 23.36146401084868884, -220.3989740370807056 ) ) ;
#14420=CARTESIAN_POINT ( 'NONE',  ( -17.04082806826102470, -4.797954729550726327, -217.3726213297937306 ) ) ;
#14421=CARTESIAN_POINT ( 'NONE',  ( -11.98736441306973077, 11.45674391201457176, -217.8252237716743025 ) ) ;
#14423=CARTESIAN_POINT ( 'NONE',  ( 26.48152825632016061, -2.044474411990439666, -219.3412966555575565 ) ) ;
#14425=CARTESIAN_POINT ( 'NONE',  ( 1.898427734299754421, 12.47096978853034521, -227.5043976727869506 ) ) ;
#14426=CARTESIAN_POINT ( 'NONE',  ( 20.96405783751201213, 6.249056650590980588, -215.6254004080763309 ) ) ;
#14427=CARTESIAN_POINT ( 'NONE',  ( -23.52999999174766543, 19.39566142560855866, -221.9446938626390704 ) ) ;
#14428=CARTESIAN_POINT ( 'NONE',  ( 4.301648988406530094, 13.23079486486395240, -223.2766268961034655 ) ) ;
#14430=CARTESIAN_POINT ( 'NONE',  ( 5.466128392039544259, 27.94759090250835243, -223.5617905851570981 ) ) ;
#14431=CARTESIAN_POINT ( 'NONE',  ( -9.606889355748592152, -11.26588727105406385, -229.9123324032181586 ) ) ;
#14432=CARTESIAN_POINT ( 'NONE',  ( 11.13678936984666912, 26.95732789089726111, -228.8350761760834757 ) ) ;
#14433=CARTESIAN_POINT ( 'NONE',  ( 22.36312131198404174, -23.32398317548372546, -224.0789201928890861 ) ) ;
#14435=CARTESIAN_POINT ( 'NONE',  ( -24.39036648059286350, 13.21953970265592027, -220.1632778389106591 ) ) ;
#14436=CARTESIAN_POINT ( 'NONE',  ( 16.80562970167152415, -4.609754314392994878, -232.4812892975905356 ) ) ;
#14437=CARTESIAN_POINT ( 'NONE',  ( 9.425340689562565544, 25.38932416188112384, -221.3391712389563963 ) ) ;
#14438=CARTESIAN_POINT ( 'NONE',  ( -17.99720854823001659, 13.97888873227035056, -232.2992184661552244 ) ) ;
#14439=CARTESIAN_POINT ( 'NONE',  ( 19.19288224840068935, 10.13059690604263174, -232.1906135022504998 ) ) ;
#14440=CARTESIAN_POINT ( 'NONE',  ( -11.58793217866213787, -13.88438693436061477, -219.4860661588769801 ) ) ;
#14441=CARTESIAN_POINT ( 'NONE',  ( 24.61409543538958289, 19.88121288930873476, -228.5015986536257344 ) ) ;
#14443=CARTESIAN_POINT ( 'NONE',  ( -23.03165807712271373, -11.67016847039487892, -215.7330867557714384 ) ) ;
#14444=CARTESIAN_POINT ( 'NONE',  ( 2.535512286608554433, 13.86868953312499109, -224.9313928733152181 ) ) ;
#14445=CARTESIAN_POINT ( 'NONE',  ( 20.10109416526603709, 2.018147939476731434, -216.1034161917718848 ) ) ;
#14447=CARTESIAN_POINT ( 'NONE',  ( -12.80756961294691010, 26.82110654133967387, -223.7464923486294026 ) ) ;
#14448=CARTESIAN_POINT ( 'NONE',  ( -12.80532875684362715, 24.61139456694233374, -232.5885756414849084 ) ) ;
#14449=CARTESIAN_POINT ( 'NONE',  ( 20.54442553493903389, -1.409480604460696007, -231.2888200459364327 ) ) ;
#14450=CARTESIAN_POINT ( 'NONE',  ( 0.4541713596374759021, -15.35025901140449989, -222.0332685144132370 ) ) ;
#14452=CARTESIAN_POINT ( 'NONE',  ( 5.380811198380419214, -14.52623441703906160, -221.9013399998540024 ) ) ;
#14455=CARTESIAN_POINT ( 'NONE',  ( 26.24002132888527328, 11.62331517472360964, -222.5300873157218859 ) ) ;
#14456=CARTESIAN_POINT ( 'NONE',  ( 28.78651053433536333, -0.9604905981993369091, -227.3547688931310233 ) ) ;
#14457=CARTESIAN_POINT ( 'NONE',  ( -15.74157322273402748, -13.22745315869835636, -216.7831660370879661 ) ) ;
#14458=CARTESIAN_POINT ( 'NONE',  ( -6.722478243781921492, -14.20656108661463612, -231.4169491518476889 ) ) ;
#14459=CARTESIAN_POINT ( 'NONE',  ( 3.786538429322381383, 16.06208591393598084, -226.9891439814428793 ) ) ;
#14461=CARTESIAN_POINT ( 'NONE',  ( -13.33011381921379090, 5.829915729572584304, -219.4453182727427816 ) ) ;
#14462=CARTESIAN_POINT ( 'NONE',  ( -6.571166997218196748, 12.74865329367398736, -229.9840124400968762 ) ) ;
#14463=CARTESIAN_POINT ( 'NONE',  ( 3.786538429322381383, 16.06208591393598084, -226.9891439814428793 ) ) ;
#14464=CARTESIAN_POINT ( 'NONE',  ( 13.62633932172415641, -0.5436634383532278347, -227.0682007726617542 ) ) ;
#14466=CARTESIAN_POINT ( 'NONE',  ( 16.55626903245587656, 22.80423546114836952, -218.9884947126587633 ) ) ;
#14467=CARTESIAN_POINT ( 'NONE',  ( -18.36252859017411510, 21.06344830687906367, -228.5073589488702623 ) ) ;
#14468=CARTESIAN_POINT ( 'NONE',  ( 14.54999166170408209, 3.068772298969228096, -219.4784171371563275 ) ) ;
#14469=CARTESIAN_POINT ( 'NONE',  ( 2.936803900436826709, -18.74190719154852758, -218.5197582523356061 ) ) ;
#14473=CARTESIAN_POINT ( 'NONE',  ( 6.093530912645064745, 16.79941505724243811, -232.1766444656230419 ) ) ;
#14474=CARTESIAN_POINT ( 'NONE',  ( 15.57890332219703389, -7.739300371747003027, -228.5080386124398899 ) ) ;
#14476=CARTESIAN_POINT ( 'NONE',  ( -15.17658589853145479, -26.64966442869902252, -226.8090782225333442 ) ) ;
#14478=CARTESIAN_POINT ( 'NONE',  ( -3.205260335674071648, 17.52234722004434531, -232.9754319808710363 ) ) ;
#14479=CARTESIAN_POINT ( 'NONE',  ( 4.401501667365108617, 18.53594119471695123, -215.1186850315663150 ) ) ;
#14481=CARTESIAN_POINT ( 'NONE',  ( -22.04257564474043818, 18.72061943465525857, -219.1781831295219263 ) ) ;
#14482=CARTESIAN_POINT ( 'NONE',  ( -10.35216574861945560, -14.43870810227675605, -231.1876371800402126 ) ) ;
#14485=CARTESIAN_POINT ( 'NONE',  ( -2.735889804569492600, 12.71735652435744512, -225.1194195722198117 ) ) ;
#14486=CARTESIAN_POINT ( 'NONE',  ( 2.478093603766003294, -30.50979708220057063, -227.6059245187310012 ) ) ;
#14489=CARTESIAN_POINT ( 'NONE',  ( -13.55591840520136770, 8.363404288414606924, -231.2690188357804857 ) ) ;
#14491=CARTESIAN_POINT ( 'NONE',  ( -16.40095417437164471, 2.582410108382750646, -233.5151473761628154 ) ) ;
#14492=CARTESIAN_POINT ( 'NONE',  ( -1.243734262319729389, 14.23902626181890518, -226.4313640849764795 ) ) ;
#14494=CARTESIAN_POINT ( 'NONE',  ( 17.02590609996173754, 6.796709046606974169, -230.8496778635019098 ) ) ;
#14495=CARTESIAN_POINT ( 'NONE',  ( -8.081326109241135924, -15.70152450856234871, -229.3783721713404304 ) ) ;
#14497=ORIENTED_EDGE ( 'NONE', *, *, #10591, .T. ) ;
#14498=CARTESIAN_POINT ( 'NONE',  ( 14.69853173970351179, 23.44775873627089524, -231.2711109634281001 ) ) ;
#14499=CARTESIAN_POINT ( 'NONE',  ( -6.804439720554941395, 15.25609613835249156, -218.7834354895107651 ) ) ;
#14500=CARTESIAN_POINT ( 'NONE',  ( -11.88513743913613752, 17.65694776598872195, -232.6054623148957035 ) ) ;
#14501=CARTESIAN_POINT ( 'NONE',  ( -24.12156516248416693, -2.505154625461648799, -217.3585533157102248 ) ) ;
#14504=CARTESIAN_POINT ( 'NONE',  ( -20.26851768784797869, -0.8260594303982465858, -217.1279713726092098 ) ) ;
#14505=CARTESIAN_POINT ( 'NONE',  ( 6.592356972974974916, -14.93599889844929862, -226.9608163220883625 ) ) ;
#14507=CARTESIAN_POINT ( 'NONE',  ( -2.808235066048971440, 30.42019778760651150, -222.6481917607299295 ) ) ;
#14508=CARTESIAN_POINT ( 'NONE',  ( 14.71815190947063812, -2.961536556857895075, -225.5177375088865404 ) ) ;
#14510=( BOUNDED_SURFACE ( )  B_SPLINE_SURFACE ( 3, 3, ( 
 ( #20095, #7667, #681, #19574, #2254, #2881, #17684, #14953, #4270, #15060, #4163, #14423, #9877, #8193, #16742, #16108, #1321, #19684, #9354, #15997, #21900, #19359, #17799, #3940, #7555, #10816, #10926, #7449, #14317, #21150, #16214, #5737, #12617, #19461, #2366, #9248, #12841, #21256, #5848, #12729, #11042, #17908, #11149, #2473, #21372, #5965, #9762, #6378, #16627, #8086, #6608, #8532, #6947, #4911, #3555, #10324, #15288, #18976, #193, #16964, #18869, #8419, #22136, #17187, #18656, #3444, #9992, #18543, #13477, #12121, #5240, #3217, #17293, #16853, #6835, #4798, #1764, #8750, #6725, #1541, #10100, #20539, #5021, #13594, #8638, #20316, #10433, #20432, #11896, #20657, #18759, #11790, #3328, #8303, #3110, #15498, #1429, #15169, #22012, #10212, #17079, #1658, #15396, #76, #13357, #1869, #20201, #13819, #22244, #13703, #15612, #5128, #12010, #11673, #19520, #7174, #13931, #5348, #9194, #12563, #19082, #19409, #2091, #10986, #14267, #19307, #2418, #4106, #9302, #3992, #16162, #12460, #8863, #410, #12230, #304, #10541, #5461, #7063, #17855, #21100, #5685, #7398, #628, #8969, #3658, #20766, #10658, #15944, #10869, #14039, #15834, #20875, #16057, #520, #3885, #17411, #1983, #15727, #3776, #7285, #12343, #19196, #17524, #14154, #10765, #7504, #20991, #5581, #17630, #2197, #9078, #17743, #2308, #14371, #21205, #5792, #12672, #8053, #16378, #9848, #957, #14919, #2850, #732, #9517, #9732, #21309, #21760, #841, #11421, #4654, #16267, #18181, #16595, #14592, #13221, #19958, #2637, #6349, #7608, #4318, #6237, #18066, #7831, #14697, #20067, #4429, #11527, #2745, #21531, #2526, #19842, #6122, #7938, #4215, #19737, #4545, #2962, #6015, #7720, #12888, #18397, #14476, #5906, #14801, #12784, #19631, #12994, #21426, #21644, #11311, #9626, #11095, #1177, #16488, #17962, #13111, #11200, #1064, #18291, #9404, #16822, #10181, #20400, #5097, #21980, #16710, #12091, #17049, #15139, #1290, #11866, #3295, #18730, #15367, #15470, #20624, #18946, #6459, #8609, #20285, #21870, #13565, #22213, #1735, #18625, #8504, #6574, #3521, #17159, #4990, #4881, #16934, #13328, #6804, #15030, #11978, #1625, #8164, #1510, #11760, #43, #5208, #13785, #13445, #6915, #13671, #6693, #20170, #4764, #11641, #3187, #18512, #10070, #3077, #1399, #9962, #8272, #8389, #20507, #15257, #22104, #18840, #3413, #10294, #271, #157, #19053, #5315, #10401, #17261, #20843, #1834, #10509, #15694, #7141, #17493, #15579, #14007, #7026, #8712, #13900, #1950, #20735, #5426, #12197, #12309, #17374, #8828, #3628, #19164, #2060, #3739, #10624, #8938, #15805, #12660, #3675, #19726 ),
 ( #11188, #209, #2407, #829, #20782, #4306, #4204, #8880, #12876, #16367, #10559, #12771, #1999, #15744, #323, #18054, #10972, #2623, #9288, #7191, #8767, #4096, #14057, #14464, #10448, #17429, #11083, #9506, #12247, #7078, #19098, #6965, #13836, #21414, #21297, #20673, #12136, #5779, #13947, #5894, #20893, #17842, #5256, #7709, #19506, #18992, #19619, #5363, #16149, #721, #3571, #7595, #17950, #2514, #9392, #16254, #17308, #1884, #14578, #6004, #15628, #18387, #9837, #2950, #21859, #21970, #4872, #18617, #12983, #15131, #4535, #6112, #20057, #6448, #8264, #2841, #15019, #13100, #10062, #1389, #11517, #11411, #1166, #19830, #13318, #21520, #18504, #8154, #3178, #8041, #18280, #6563, #11751, #20277, #19946, #13435, #1280, #944, #7821, #9723, #20159, #16585, #14909, #21749, #14686, #4644, #4416, #16699, #6339, #2735, #4752, #13212, #11631, #11300, #3066, #9954, #18171, #6224, #1054, #16813, #9615, #16477, #7927, #14790, #21632, #22094, #15464, #10173, #1827, #8603, #5201, #5419, #17366, #11970, #6684, #150, #15360, #17042, #6796, #19155, #1618, #10395, #20615, #5309, #22207, #16926, #12302, #17255, #13664, #1500, #12084, #3515, #18940, #15570, #15687, #20837, #3733, #13556, #8822, #20500, #20391, #13776, #7018, #1942, #18832, #8704, #5090, #8379, #265, #13892, #3406, #17152, #4984, #20729, #15248, #12191, #19046, #11859, #1729, #10287, #7135, #18724, #14001, #37, #3289, #3622, #6907, #8496, #10501, #12858, #9041, #9371, #21062, #16231, #17594, #2054, #7245, #11059, #593, #20951, #8932, #19701, #807, #21391, #12635, #5539, #19376, #698, #17486, #10615, #2383, #5983, #5650, #16016, #7466, #12747, #15799, #14555, #3849, #5755, #4183, #2161, #7686, #7574, #12528, #377, #16125, #14115, #3957, #14226, #484, #17818, #2271, #10832, #14440, #10729, #12417, #17704, #7359, #17928, #9154, #15907, #14335, #19269, #21168, #21275, #19482, #4070, #10946, #9267, #5866, #19594, #2491, #21836, #13408, #16791, #11166, #4727, #11390, #18258, #18478, #16561, #14882, #3041, #1366, #4392, #18033, #2602, #6426, #9812, #16343, #16675, #21609, #8241, #11496, #1140, #21946, #15109, #6537, #1255, #4287, #9701, #6088, #19922, #9483, #19808, #7800, #2712, #919, #14665, #18364, #2925, #4622, #20137, #6201, #21499, #12964, #7907, #13190, #8130, #11277, #13078, #18146, #13296, #20034, #8018, #9595, #16458, #1032, #14768, #4509, #2822, #21723, #6316, #14997, #11607, #9927, #8468, #22067, #3154, #7108, #13639, #8575, #4956, #11942, #17229, #15440, #3596, #5282, #20474, #20251, #5066, #12163, #124, #4846, #6770, #6992, #18592, #19019, #20365 ),
 ( #3377, #10258, #13864, #10039, #17016, #10473, #11834, #16899, #18700, #17336, #1915, #3263, #8797, #1475, #13750, #11722, #3490, #15658, #18807, #1592, #10147, #5174, #17125, #1702, #10366, #13524, #238, #15335, #22181, #8351, #10, #6879, #20588, #15222, #6656, #1802, #12056, #18913, #8678, #15542, #20704, #10807, #455, #9241, #778, #4154, #20812, #14416, #21037, #5625, #5840, #3932, #2244, #12720, #11034, #14084, #5388, #12272, #16101, #19453, #3705, #4040, #9013, #17901, #21142, #17673, #9347, #2464, #16207, #10919, #13972, #19350, #15772, #7332, #19125, #7219, #17457, #12390, #10587, #2026, #5729, #12609, #14309, #7548, #15878, #8906, #350, #17567, #565, #17791, #20922, #14200, #5511, #672, #7441, #9126, #19240, #3820, #10703, #2136, #12503, #15988, #2356, #21248, #19567, #11363, #8103, #18120, #9457, #12833, #16762, #1006, #18232, #14640, #21583, #4593, #2792, #13269, #14969, #7881, #7658, #14743, #21810, #9781, #14530, #16431, #16646, #5956, #6398, #7770, #18337, #13048, #6171, #2687, #20112, #18449, #4700, #4365, #11576, #7988, #19896, #19676, #3014, #9898, #6064, #21364, #9569, #4263, #21472, #11141, #18009, #2574, #4484, #16318, #894, #12938, #19784, #11249, #9675, #16534, #1113, #20007, #14852, #21697, #6288, #13162, #11469, #2898, #1229, #3466, #21920, #5261, #16874, #18783, #17207, #15193, #13842, #20563, #3237, #6970, #10453, #4933, #6855, #18676, #10121, #16986, #20679, #5040, #12141, #3349, #1565, #3130, #20451, #8440, #8553, #4819, #20337, #5149, #3576, #6629, #1450, #13499, #18997, #1340, #15517, #15417, #8212, #6510, #22157, #8323, #22260, #15309, #11917, #15084, #1781, #6746, #13380, #13723, #22037, #11809, #13614, #20222, #10232, #17100, #1679, #12031, #18891, #11696, #18565, #10344, #8656, #10010, #100, #3910, #12483, #15967, #16080, #21227, #12696, #7085, #9217, #20900, #216, #14177, #541, #2332, #19218, #9101, #7197, #4130, #17767, #5602, #5485, #17547, #13952, #7419, #15636, #12586, #2220, #19542, #19431, #14288, #20788, #21121, #12368, #5817, #5709, #7307, #17314, #7527, #1890, #4016, #8773, #433, #19103, #10683, #5368, #10564, #12252, #15750, #3680, #14395, #10892, #649, #17653, #17435, #3799, #2004, #8886, #2114, #10786, #329, #14063, #8993, #15856, #21014, #19330, #7854, #7632, #9324, #1200, #7743, #11224, #21335, #21783, #16291, #13243, #14720, #11444, #21449, #12808, #16184, #20087, #4339, #21556, #17985, #2659, #7960, #6146, #16619, #18312, #18091, #11011, #9541, #2872, #13135, #17879, #19759, #19981, #755, #9754, #11117, #21670, #16403, #14615, #8077, #2547, #14501, #9430, #14943 ),
 ( #866, #6370, #14826, #12913, #2441, #5929, #6038, #16509, #979, #13021, #19868, #19652, #4453, #4237, #11335, #18206, #2767, #9648, #1086, #6261, #4568, #1420, #1649, #6939, #9984, #4788, #16845, #1756, #10316, #18860, #18750, #13809, #9868, #3209, #20193, #11888, #18648, #15279, #66, #17179, #4674, #8524, #11549, #10091, #6481, #20306, #16733, #11663, #8185, #3101, #18421, #8630, #3320, #10203, #5012, #20530, #22004, #1312, #2985, #8294, #13586, #17070, #18533, #6599, #15161, #13693, #20423, #1533, #15052, #21892, #15490, #13467, #4903, #13350, #11782, #16956, #8411, #22128, #5119, #6716, #15388, #22236, #6826, #12001, #3435, #5340, #12335, #17623, #15826, #3986, #5678, #14031, #7497, #20867, #12556, #514, #20649, #7165, #7390, #18969, #19403, #20758, #9070, #3765, #17401, #10861, #12222, #3547, #19074, #17737, #2302, #3649, #9186, #17285, #14147, #12113, #3877, #16049, #5452, #1974, #10533, #5572, #19188, #10649, #10758, #13923, #620, #8852, #15719, #5232, #17516, #296, #2084, #15605, #10424, #2189, #1860, #8740, #183, #7053, #8962, #403, #7277, #15939, #20984, #12450, #19300, #21093, #14259, #21419, #6231, #4311, #2630, #13104, #4539, #14469, #21198, #12665, #16481, #19835, #4100, #4422, #9397, #18283, #21524, #11194, #19513, #11304, #12776, #21303, #4209, #16588, #5900, #7825, #18059, #2739, #19624, #14365, #9726, #14690, #11088, #5786, #9511, #949, #16372, #12987, #19950, #2844, #1169, #10978, #11414, #17955, #17848, #6116, #18175, #21636, #16259, #9619, #2520, #2412, #14794, #1058, #835, #14584, #9294, #7931, #16156, #726, #7601, #7714, #6009, #12881, #19731, #19130, #5393, #4755, #15662, #8683, #20593, #13215, #12278, #10593, #6451, #7112, #18811, #13976, #15022, #21752, #4647, #8801, #5179, #18390, #6342, #17462, #20816, #3710, #10371, #2954, #17131, #20709, #14913, #8046, #128, #20060, #3382, #13754, #12061, #10477, #11521, #9842, #1283, #3495, #1920, #21862, #16703, #5287, #10263, #8157, #13321, #11947, #13868, #1707, #8581, #15445, #20162, #18919, #15, #17235, #6885, #1806, #15549, #6996, #12167, #19023, #3601, #17342, #243, #7338, #2141, #14205, #21368, #7664, #16211, #16105, #4267, #7224, #570, #17572, #9245, #15994, #12613, #12837, #2469, #19355, #15883, #14089, #9018, #783, #14534, #21041, #5960, #20929, #17795, #15777, #7552, #19681, #17679, #5631, #12508, #677, #7446, #2251, #14420, #461, #11145, #3937, #10812, #9351, #9131, #14314, #21146, #19246, #5516, #5845, #12395, #3826, #10708, #5734, #19458, #4046, #10923, #19571, #2032, #8911, #356, #2361, #21253, #12724, #4158, #11039 ),
 ( #17905, #21925, #2903, #7994, #13384, #8217, #20228, #14974, #4823, #1118, #19787, #11368, #898, #11254, #21476, #16435, #18013, #15089, #9788, #16653, #18342, #11582, #13056, #7775, #2579, #21588, #4598, #1234, #18124, #19901, #2691, #4705, #11474, #14859, #14645, #16322, #6514, #14747, #18237, #6070, #9462, #1010, #12942, #21702, #18456, #6177, #4370, #9573, #7885, #2797, #6293, #4489, #9680, #21815, #13167, #1346, #3019, #16539, #20012, #8108, #9904, #20116, #6404, #13274, #16767, #10015, #3580, #11813, #104, #17104, #8445, #1894, #19001, #13618, #3470, #1572, #20792, #12145, #22264, #15314, #11921, #16879, #10348, #1454, #6975, #18895, #7089, #18787, #6750, #17318, #220, #8779, #22161, #10457, #12035, #1683, #8327, #15640, #13956, #10126, #11700, #20456, #18570, #18680, #3134, #15197, #22044, #8557, #6633, #13504, #20341, #4937, #3242, #13727, #16991, #5044, #1785, #3355, #10237, #17211, #15421, #6859, #20567, #5155, #13846, #8660, #15521, #20683, #5265, #21231, #19223, #17883, #2337, #7311, #11015, #14505, #8997, #10896, #437, #14182, #21019, #2445, #9105, #9328, #546, #5606, #7201, #2224, #12487, #12590, #8890, #2118, #9221, #7636, #10687, #5489, #17551, #16188, #760, #19546, #19435, #5372, #10569, #3914, #20903, #4020, #19334, #15972, #12256, #5821, #10790, #17439, #17771, #3803, #12373, #15860, #19107, #17657, #21125, #7423, #16084, #14292, #3684, #2008, #5713, #653, #15754, #7531, #14399, #12700, #4136, #333, #14067, #16738, #11121, #13246, #2663, #4241, #18210, #19985, #9547, #17989, #2771, #4572, #6374, #984, #13141, #11227, #8189, #21787, #9652, #16408, #21560, #2551, #11448, #19656, #16623, #6265, #1316, #6150, #7858, #4678, #9872, #18425, #18096, #20091, #21674, #11340, #9435, #2989, #21339, #19763, #11553, #14724, #5934, #6042, #12812, #16295, #870, #16513, #7749, #14619, #21453, #12917, #4343, #1090, #13025, #19872, #18316, #4458, #7964, #2876, #14830, #9758, #1204, #8081, #14949, #13354, #18972, #8299, #10207, #8634, #6603, #5236, #12005, #16960, #20653, #1864, #18652, #20534, #10096, #1537, #8415, #12117, #18755, #3551, #17074, #15283, #16849, #11892, #22132, #22240, #18539, #11786, #18864, #17289, #20311, #15165, #4907, #10428, #15056, #6943, #6831, #21896, #20197, #13590, #22007, #13699, #6720, #3324, #6484, #15494, #20428, #4792, #5124, #13471, #3213, #5017, #11667, #1654, #8528, #15392, #3440, #10320, #3105, #9988, #17183, #1760, #1425, #71, #13814, #3882, #7394, #7501, #12670, #4104, #20762, #625, #20988, #13927, #19518, #10982, #7170, #14369, #19192, #21203, #15723, #188, #5344, #9190 ),
 ( #300, #12226, #8859, #5790, #17853, #14035, #8745, #19078, #2194, #7059, #14264, #15609, #2088, #12339, #20871, #15942, #407, #8966, #21097, #1978, #3653, #3769, #5456, #16054, #15831, #10655, #7281, #10537, #17406, #12561, #17521, #14151, #5576, #12456, #19304, #10762, #17627, #3990, #9074, #518, #5682, #19407, #10866, #17741, #2306, #14694, #12991, #16593, #14917, #2524, #9298, #730, #4543, #7935, #14474, #14799, #19735, #6347, #9623, #21529, #20064, #21756, #4651, #21641, #11525, #7829, #4213, #18063, #7606, #17959, #5904, #839, #2416, #13219, #16485, #1062, #2743, #18287, #4315, #21307, #16160, #6013, #11309, #6235, #9401, #11198, #16265, #11419, #18179, #6119, #12780, #19629, #11092, #21424, #2635, #7718, #14588, #12885, #9515, #19840, #2848, #16375, #954, #4426, #13108, #19955, #9730, #1175, #8050, #9959, #16931, #13325, #8161, #22210, #21866, #1287, #6456, #20167, #15136, #15254, #4877, #13668, #5204, #8606, #2960, #18836, #3183, #10067, #10290, #8386, #6688, #17156, #15466, #18509, #9846, #16707, #20503, #1622, #15027, #8499, #13442, #40, #3292, #22100, #13782, #6911, #20621, #15364, #18395, #1506, #4761, #11756, #11638, #3071, #16818, #1395, #8269, #21977, #10177, #17046, #18727, #11975, #20282, #6571, #18622, #13562, #4987, #6800, #20396, #11862, #5094, #3410, #1732, #8935, #8708, #10398, #2276, #8825, #12305, #154, #596, #17371, #14338, #15802, #12531, #268, #13895, #17258, #21171, #5423, #380, #19050, #3736, #9044, #7248, #17708, #19379, #19160, #12087, #10620, #3960, #14231, #18943, #20840, #21066, #1830, #10835, #12194, #490, #17489, #15690, #9159, #3625, #15575, #10504, #16021, #7469, #1946, #3518, #7023, #5543, #20732, #17597, #5312, #2057, #7138, #14004, #19273, #14119, #20955, #2164, #12422, #3852, #10732, #15910, #7363, #5654, #4075, #7910, #11281, #17823, #18151, #810, #9705, #12967, #18037, #1145, #18261, #8021, #2716, #14887, #11169, #7577, #21395, #10950, #21278, #9270, #4186, #5758, #2825, #19812, #4396, #6092, #21613, #7691, #2385, #12638, #9374, #14668, #9598, #5871, #14559, #12751, #14773, #21502, #2605, #16128, #701, #16565, #2494, #5987, #14443, #19485, #11062, #19599, #9487, #6204, #16234, #17932, #12861, #19705, #4290, #16349, #923, #7803, #16461, #1036, #11393, #13082, #19927, #4513, #4733, #15228, #10044, #21728, #11610, #1481, #20038, #22073, #1259, #16905, #16794, #6430, #13533, #8134, #4625, #15000, #6663, #20371, #21838, #4963, #11499, #6543, #13193, #11729, #11840, #18482, #13299, #20140, #20255, #9932, #3045, #18597, #16679, #6319, #1369, #8245, #18368, #21950, #15113 ),
 ( #2929, #9816, #13414, #4852, #3160, #8358, #2894, #11464, #11358, #21805, #2460, #18115, #12828, #20003, #7876, #888, #19779, #9343, #18227, #17897, #14848, #4478, #14965, #4360, #14635, #9777, #8098, #16642, #16313, #4588, #19890, #9564, #16202, #1224, #6393, #18004, #18333, #7765, #19563, #4258, #11030, #773, #4150, #16426, #7653, #14524, #21359, #5951, #19671, #21578, #11136, #6059, #9670, #2568, #9452, #2787, #21467, #12933, #2682, #1001, #21692, #11243, #14738, #6166, #13043, #13157, #16529, #1108, #7983, #6283, #18885, #94, #16869, #18777, #8317, #15187, #22031, #3459, #16980, #10338, #8434, #6622, #15079, #10115, #13492, #20445, #16757, #10006, #10226, #15512, #18560, #13375, #3126, #17202, #1777, #5144, #5034, #13264, #18445, #11803, #6504, #11911, #4927, #1559, #8651, #13718, #20331, #3008, #3343, #11689, #20217, #1446, #20108, #4812, #6740, #15301, #1672, #18670, #4696, #11571, #13608, #3231, #9892, #22151, #17095, #8547, #15411, #12025, #1335, #8207, #21915, #22256, #6849, #20557, #15323, #8786, #1580, #8564, #13627, #228, #113, #17113, #3365, #20801, #20574, #5053, #12044, #8454, #3249, #17326, #17001, #18687, #22169, #6757, #10246, #10355, #2730, #15647, #340, #3692, #20350, #13962, #5162, #18902, #5379, #3477, #1791, #12262, #10576, #20463, #4945, #11821, #7098, #19009, #10134, #3586, #15428, #17447, #20694, #17218, #8896, #2016, #15762, #10463, #13512, #8667, #11929, #6866, #18796, #1691, #13736, #15530, #6981, #13853, #5271, #12152, #1903, #19115, #2234, #19230, #14074, #20912, #9003, #2454, #17557, #9114, #7319, #16196, #16091, #4030, #3810, #5499, #19665, #3921, #7431, #2126, #17998, #12493, #9446, #10906, #7647, #17663, #15867, #12379, #16307, #554, #17780, #14189, #21132, #4144, #2345, #12822, #14518, #14299, #7208, #5719, #21350, #9336, #10693, #15978, #768, #445, #5945, #21026, #17891, #12598, #10798, #4252, #5615, #19340, #19443, #11130, #2561, #9231, #662, #7538, #14407, #21239, #12709, #5831, #19556, #11023, #13037, #8093, #14843, #1103, #6386, #16420, #20212, #4807, #6498, #15072, #14960, #3121, #6054, #21686, #996, #21800, #6277, #11459, #11683, #1330, #18222, #12928, #13259, #21573, #7871, #19884, #10001, #14734, #16637, #4583, #11565, #6160, #882, #18555, #1218, #4472, #7758, #18328, #9771, #2889, #20102, #21910, #14630, #21462, #19774, #13369, #11352, #13151, #19997, #4353, #11238, #2781, #4691, #9665, #18108, #8202, #18440, #16524, #7977, #2676, #3003, #9558, #9886, #16751, #12240, #17089, #11905, #202, #5357, #13940, #13603, #1877, #17195, #6844, #22026, #20775, #19091, #15296 ) ),
 .UNSPECIFIED., .T., .F., .F. ) 
 B_SPLINE_SURFACE_WITH_KNOTS ( ( 4, 3, 4 ),
 ( 4, 2, 2, 2, 2, 2, 2, 2, 2, 2, 2, 2, 2, 2, 2, 2, 2, 2, 2, 2, 2, 2, 2, 2, 2, 2, 2, 2, 2, 2, 2, 2, 2, 2, 2, 2, 2, 2, 2, 2, 2, 2, 2, 2, 2, 2, 2, 2, 2, 2, 2, 2, 2, 2, 2, 2, 2, 2, 2, 2, 2, 2, 2, 2, 2, 2, 2, 2, 2, 2, 2, 2, 2, 2, 2, 2, 2, 2, 2, 2, 2, 2, 2, 2, 2, 2, 2, 2, 2, 2, 2, 2, 2, 2, 2, 2, 2, 2, 2, 2, 2, 2, 2, 2, 2, 2, 2, 2, 2, 2, 2, 2, 2, 2, 2, 2, 2, 2, 2, 2, 2, 2, 2, 2, 2, 2, 2, 2, 2, 2, 2, 2, 2, 2, 2, 2, 2, 2, 2, 2, 2, 2, 2, 2, 2, 2, 2, 2, 2, 2, 2, 2, 2, 2, 2, 2, 2, 2, 2, 2, 2, 2, 2, 2, 2, 2, 2, 2, 2, 4 ),
 ( 0.000000000000000000, 0.5000000000000000000, 1.000000000000000000 ),
 ( 0.4999446919652688059, 0.5028747035357847839, 0.5058047151063008728, 0.5087347266768169618, 0.5116647382473329397, 0.5145947498178489177, 0.5175247613883648956, 0.5204547729588808735, 0.5233847845293969625, 0.5268031313616656774, 0.5285123047777999794, 0.5302214781939342814, 0.5336398250262029963, 0.5353489984423374093, 0.5370581718584717112, 0.5404765186907403152, 0.5438948655230090301, 0.5473132123552777450, 0.5507315591875463490, 0.5541499060198149529, 0.5575682528520836678, 0.5609865996843523828, 0.5644049465166209867, 0.5661141199327552886, 0.5678232933488895906, 0.5712416401811581945, 0.5729508135972924965, 0.5746599870134267984, 0.5780783338456955134, 0.5814966806779642283, 0.5849150275102328322, 0.5883333743425015472, 0.5917517211747702621, 0.5951700680070388660, 0.5985884148393075810, 0.6020067616715762959, 0.6037159350877105979, 0.6054251085038448998, 0.6088434553361135038, 0.6122618021683822187, 0.6139709755845166317, 0.6156801490006509336, 0.6190984958329195376, 0.6225168426651882525, 0.6259351894974569674, 0.6293535363297255714, 0.6327718831619942863, 0.6361902299942630012, 0.6396085768265316052, 0.6430269236588003201, 0.6447360970749347331, 0.6464452704910690350, 0.6498636173233376390, 0.6532819641556063539, 0.6549911375717407669, 0.6567003109878750688, 0.6601186578201436728, 0.6635370046524122767, 0.6669553514846809916, 0.6703736983169497066, 0.6737920451492183105, 0.6772103919814870254, 0.6806287388137557404, 0.6840470856460243443, 0.6857562590621586462, 0.6866108457702257972, 0.6874654324782930592, 0.6908837793105617742, 0.6943021261428303781, 0.6960112995589646800, 0.6977204729750989820, 0.7011388198073676969, 0.7045571666396364119, 0.7079755134719050158, 0.7113938603041736197, 0.7148122071364423347, 0.7182305539687110496, 0.7216489008009796535, 0.7250672476332483685, 0.7267764210493827814, 0.7284855944655170834, 0.7319039412977856873, 0.7353222881300544023, 0.7387406349623231172, 0.7421589817945917211, 0.7455773286268603250, 0.7489956754591290400, 0.7524140222913977549, 0.7558323691236663588, 0.7592507159559350738, 0.7626690627882037887, 0.7660874096204723926, 0.7695057564527411076, 0.7729241032850098225, 0.7763424501172784264, 0.7797607969495471414, 0.7831791437818158563, 0.7865974906140844602, 0.7900158374463531752, 0.7934341842786218901, 0.7968525311108904940, 0.8002708779431590980, 0.8036892247754278129, 0.8053983981915622259, 0.8071075716076965278, 0.8105259184399651318, 0.8122350918560994337, 0.8139442652722337357, 0.8173626121045024506, 0.8207809589367711656, 0.8241993057690397695, 0.8276176526013083734, 0.8310359994335770883, 0.8344543462658458033, 0.8378726930981144072, 0.8412910399303831221, 0.8430002133465175351, 0.8447093867626518371, 0.8481277335949204410, 0.8515460804271891559, 0.8549644272594578709, 0.8583827740917264748, 0.8618011209239951897, 0.8652194677562639047, 0.8686378145885325086, 0.8720561614208012235, 0.8754745082530699385, 0.8788928550853385424, 0.8823112019176071463, 0.8857295487498758613, 0.8874387221660102743, 0.8891478955821445762, 0.8925662424144131801, 0.8942754158305474821, 0.8959845892466818951, 0.8994029360789506100, 0.9028212829112192139, 0.9062396297434879289, 0.9096579765757566438, 0.9130763234080252477, 0.9164946702402939627, 0.9199130170725626776, 0.9233313639048312815, 0.9250405373209655835, 0.9267497107370999965, 0.9301680575693687114, 0.9335864044016373153, 0.9352955778177716173, 0.9370047512339059192, 0.9404230980661746342, 0.9438414448984433491, 0.9472597917307119531, 0.9506781385629806680, 0.9540964853952493829, 0.9575148322275179869, 0.9609331790597867018, 0.9643515258920554167, 0.9660606993081897187, 0.9677698727243240207, 0.9711882195565927356, 0.9728973929727271486, 0.9746065663888614505, 0.9780249132211300545, 0.9814432600533987694, 0.9848616068856674843, 0.9882799537179360883, 0.9912099652884520662, 0.9941399768589680441, 0.9970699884294840221, 1.000000000000000000 ),
 .UNSPECIFIED. ) 
 GEOMETRIC_REPRESENTATION_ITEM ( )  RATIONAL_B_SPLINE_SURFACE ( (
 ( 1.000000000000000000, 1.000000000000000000, 1.000000000000000000, 1.000000000000000000, 1.000000000000000000, 1.000000000000000000, 1.000000000000000000, 1.000000000000000000, 1.000000000000000000, 1.000000000000000000, 1.000000000000000000, 1.000000000000000000, 1.000000000000000000, 1.000000000000000000, 1.000000000000000000, 1.000000000000000000, 1.000000000000000000, 1.000000000000000000, 1.000000000000000000, 1.000000000000000000, 1.000000000000000000, 1.000000000000000000, 1.000000000000000000, 1.000000000000000000, 1.000000000000000000, 1.000000000000000000, 1.000000000000000000, 1.000000000000000000, 1.000000000000000000, 1.000000000000000000, 1.000000000000000000, 1.000000000000000000, 1.000000000000000000, 1.000000000000000000, 1.000000000000000000, 1.000000000000000000, 1.000000000000000000, 1.000000000000000000, 1.000000000000000000, 1.000000000000000000, 1.000000000000000000, 1.000000000000000000, 1.000000000000000000, 1.000000000000000000, 1.000000000000000000, 1.000000000000000000, 1.000000000000000000, 1.000000000000000000, 1.000000000000000000, 1.000000000000000000, 1.000000000000000000, 1.000000000000000000, 1.000000000000000000, 1.000000000000000000, 1.000000000000000000, 1.000000000000000000, 1.000000000000000000, 1.000000000000000000, 1.000000000000000000, 1.000000000000000000, 1.000000000000000000, 1.000000000000000000, 1.000000000000000000, 1.000000000000000000, 1.000000000000000000, 1.000000000000000000, 1.000000000000000000, 1.000000000000000000, 1.000000000000000000, 1.000000000000000000, 1.000000000000000000, 1.000000000000000000, 1.000000000000000000, 1.000000000000000000, 1.000000000000000000, 1.000000000000000000, 1.000000000000000000, 1.000000000000000000, 1.000000000000000000, 1.000000000000000000, 1.000000000000000000, 1.000000000000000000, 1.000000000000000000, 1.000000000000000000, 1.000000000000000000, 1.000000000000000000, 1.000000000000000000, 1.000000000000000000, 1.000000000000000000, 1.000000000000000000, 1.000000000000000000, 1.000000000000000000, 1.000000000000000000, 1.000000000000000000, 1.000000000000000000, 1.000000000000000000, 1.000000000000000000, 1.000000000000000000, 1.000000000000000000, 1.000000000000000000, 1.000000000000000000, 1.000000000000000000, 1.000000000000000000, 1.000000000000000000, 1.000000000000000000, 1.000000000000000000, 1.000000000000000000, 1.000000000000000000, 1.000000000000000000, 1.000000000000000000, 1.000000000000000000, 1.000000000000000000, 1.000000000000000000, 1.000000000000000000, 1.000000000000000000, 1.000000000000000000, 1.000000000000000000, 1.000000000000000000, 1.000000000000000000, 1.000000000000000000, 1.000000000000000000, 1.000000000000000000, 1.000000000000000000, 1.000000000000000000, 1.000000000000000000, 1.000000000000000000, 1.000000000000000000, 1.000000000000000000, 1.000000000000000000, 1.000000000000000000, 1.000000000000000000, 1.000000000000000000, 1.000000000000000000, 1.000000000000000000, 1.000000000000000000, 1.000000000000000000, 1.000000000000000000, 1.000000000000000000, 1.000000000000000000, 1.000000000000000000, 1.000000000000000000, 1.000000000000000000, 1.000000000000000000, 1.000000000000000000, 1.000000000000000000, 1.000000000000000000, 1.000000000000000000, 1.000000000000000000, 1.000000000000000000, 1.000000000000000000, 1.000000000000000000, 1.000000000000000000, 1.000000000000000000, 1.000000000000000000, 1.000000000000000000, 1.000000000000000000, 1.000000000000000000, 1.000000000000000000, 1.000000000000000000, 1.000000000000000000, 1.000000000000000000, 1.000000000000000000, 1.000000000000000000, 1.000000000000000000, 1.000000000000000000, 1.000000000000000000, 1.000000000000000000, 1.000000000000000000, 1.000000000000000000, 1.000000000000000000, 1.000000000000000000, 1.000000000000000000, 1.000000000000000000, 1.000000000000000000, 1.000000000000000000, 1.000000000000000000, 1.000000000000000000, 1.000000000000000000, 1.000000000000000000, 1.000000000000000000, 1.000000000000000000, 1.000000000000000000, 1.000000000000000000, 1.000000000000000000, 1.000000000000000000, 1.000000000000000000, 1.000000000000000000, 1.000000000000000000, 1.000000000000000000, 1.000000000000000000, 1.000000000000000000, 1.000000000000000000, 1.000000000000000000, 1.000000000000000000, 1.000000000000000000, 1.000000000000000000, 1.000000000000000000, 1.000000000000000000, 1.000000000000000000, 1.000000000000000000, 1.000000000000000000, 1.000000000000000000, 1.000000000000000000, 1.000000000000000000, 1.000000000000000000, 1.000000000000000000, 1.000000000000000000, 1.000000000000000000, 1.000000000000000000, 1.000000000000000000, 1.000000000000000000, 1.000000000000000000, 1.000000000000000000, 1.000000000000000000, 1.000000000000000000, 1.000000000000000000, 1.000000000000000000, 1.000000000000000000, 1.000000000000000000, 1.000000000000000000, 1.000000000000000000, 1.000000000000000000, 1.000000000000000000, 1.000000000000000000, 1.000000000000000000, 1.000000000000000000, 1.000000000000000000, 1.000000000000000000, 1.000000000000000000, 1.000000000000000000, 1.000000000000000000, 1.000000000000000000, 1.000000000000000000, 1.000000000000000000, 1.000000000000000000, 1.000000000000000000, 1.000000000000000000, 1.000000000000000000, 1.000000000000000000, 1.000000000000000000, 1.000000000000000000, 1.000000000000000000, 1.000000000000000000, 1.000000000000000000, 1.000000000000000000, 1.000000000000000000, 1.000000000000000000, 1.000000000000000000, 1.000000000000000000, 1.000000000000000000, 1.000000000000000000, 1.000000000000000000, 1.000000000000000000, 1.000000000000000000, 1.000000000000000000, 1.000000000000000000, 1.000000000000000000, 1.000000000000000000, 1.000000000000000000, 1.000000000000000000, 1.000000000000000000, 1.000000000000000000, 1.000000000000000000, 1.000000000000000000, 1.000000000000000000, 1.000000000000000000, 1.000000000000000000, 1.000000000000000000, 1.000000000000000000, 1.000000000000000000, 1.000000000000000000, 1.000000000000000000, 1.000000000000000000, 1.000000000000000000, 1.000000000000000000, 1.000000000000000000, 1.000000000000000000, 1.000000000000000000, 1.000000000000000000, 1.000000000000000000, 1.000000000000000000, 1.000000000000000000, 1.000000000000000000, 1.000000000000000000, 1.000000000000000000, 1.000000000000000000, 1.000000000000000000, 1.000000000000000000, 1.000000000000000000, 1.000000000000000000, 1.000000000000000000, 1.000000000000000000, 1.000000000000000000, 1.000000000000000000, 1.000000000000000000, 1.000000000000000000, 1.000000000000000000, 1.000000000000000000, 1.000000000000000000, 1.000000000000000000, 1.000000000000000000, 1.000000000000000000, 1.000000000000000000, 1.000000000000000000, 1.000000000000000000, 1.000000000000000000, 1.000000000000000000, 1.000000000000000000, 1.000000000000000000, 1.000000000000000000, 1.000000000000000000, 1.000000000000000000, 1.000000000000000000, 1.000000000000000000, 1.000000000000000000, 1.000000000000000000, 1.000000000000000000, 1.000000000000000000, 1.000000000000000000, 1.000000000000000000, 1.000000000000000000, 1.000000000000000000, 1.000000000000000000, 1.000000000000000000, 1.000000000000000000, 1.000000000000000000, 1.000000000000000000, 1.000000000000000000, 1.000000000000000000, 1.000000000000000000, 1.000000000000000000, 1.000000000000000000, 1.000000000000000000, 1.000000000000000000, 1.000000000000000000, 1.000000000000000000, 1.000000000000000000, 1.000000000000000000, 1.000000000000000000, 1.000000000000000000),
 ( 0.3333333333333333703, 0.3333333333333333703, 0.3333333333333333703, 0.3333333333333333703, 0.3333333333333333703, 0.3333333333333333703, 0.3333333333333333703, 0.3333333333333333703, 0.3333333333333333703, 0.3333333333333333703, 0.3333333333333333703, 0.3333333333333333703, 0.3333333333333333703, 0.3333333333333333703, 0.3333333333333333703, 0.3333333333333333703, 0.3333333333333333703, 0.3333333333333333703, 0.3333333333333333703, 0.3333333333333333703, 0.3333333333333333703, 0.3333333333333333703, 0.3333333333333333703, 0.3333333333333333703, 0.3333333333333333703, 0.3333333333333333703, 0.3333333333333333703, 0.3333333333333333703, 0.3333333333333333703, 0.3333333333333333703, 0.3333333333333333703, 0.3333333333333333703, 0.3333333333333333703, 0.3333333333333333703, 0.3333333333333333703, 0.3333333333333333703, 0.3333333333333333703, 0.3333333333333333703, 0.3333333333333333703, 0.3333333333333333703, 0.3333333333333333703, 0.3333333333333333703, 0.3333333333333333703, 0.3333333333333333703, 0.3333333333333333703, 0.3333333333333333703, 0.3333333333333333703, 0.3333333333333333703, 0.3333333333333333703, 0.3333333333333333703, 0.3333333333333333703, 0.3333333333333333703, 0.3333333333333333703, 0.3333333333333333703, 0.3333333333333333703, 0.3333333333333333703, 0.3333333333333333703, 0.3333333333333333703, 0.3333333333333333703, 0.3333333333333333703, 0.3333333333333333703, 0.3333333333333333703, 0.3333333333333333703, 0.3333333333333333703, 0.3333333333333333703, 0.3333333333333333703, 0.3333333333333333703, 0.3333333333333333703, 0.3333333333333333703, 0.3333333333333333703, 0.3333333333333333703, 0.3333333333333333703, 0.3333333333333333703, 0.3333333333333333703, 0.3333333333333333703, 0.3333333333333333703, 0.3333333333333333703, 0.3333333333333333703, 0.3333333333333333703, 0.3333333333333333703, 0.3333333333333333703, 0.3333333333333333703, 0.3333333333333333703, 0.3333333333333333703, 0.3333333333333333703, 0.3333333333333333703, 0.3333333333333333703, 0.3333333333333333703, 0.3333333333333333703, 0.3333333333333333703, 0.3333333333333333703, 0.3333333333333333703, 0.3333333333333333703, 0.3333333333333333703, 0.3333333333333333703, 0.3333333333333333703, 0.3333333333333333703, 0.3333333333333333703, 0.3333333333333333703, 0.3333333333333333703, 0.3333333333333333703, 0.3333333333333333703, 0.3333333333333333703, 0.3333333333333333703, 0.3333333333333333703, 0.3333333333333333703, 0.3333333333333333703, 0.3333333333333333703, 0.3333333333333333703, 0.3333333333333333703, 0.3333333333333333703, 0.3333333333333333703, 0.3333333333333333703, 0.3333333333333333703, 0.3333333333333333703, 0.3333333333333333703, 0.3333333333333333703, 0.3333333333333333703, 0.3333333333333333703, 0.3333333333333333703, 0.3333333333333333703, 0.3333333333333333703, 0.3333333333333333703, 0.3333333333333333703, 0.3333333333333333703, 0.3333333333333333703, 0.3333333333333333703, 0.3333333333333333703, 0.3333333333333333703, 0.3333333333333333703, 0.3333333333333333703, 0.3333333333333333703, 0.3333333333333333703, 0.3333333333333333703, 0.3333333333333333703, 0.3333333333333333703, 0.3333333333333333703, 0.3333333333333333703, 0.3333333333333333703, 0.3333333333333333703, 0.3333333333333333703, 0.3333333333333333703, 0.3333333333333333703, 0.3333333333333333703, 0.3333333333333333703, 0.3333333333333333703, 0.3333333333333333703, 0.3333333333333333703, 0.3333333333333333703, 0.3333333333333333703, 0.3333333333333333703, 0.3333333333333333703, 0.3333333333333333703, 0.3333333333333333703, 0.3333333333333333703, 0.3333333333333333703, 0.3333333333333333703, 0.3333333333333333703, 0.3333333333333333703, 0.3333333333333333703, 0.3333333333333333703, 0.3333333333333333703, 0.3333333333333333703, 0.3333333333333333703, 0.3333333333333333703, 0.3333333333333333703, 0.3333333333333333703, 0.3333333333333333703, 0.3333333333333333703, 0.3333333333333333703, 0.3333333333333333703, 0.3333333333333333703, 0.3333333333333333703, 0.3333333333333333703, 0.3333333333333333703, 0.3333333333333333703, 0.3333333333333333703, 0.3333333333333333703, 0.3333333333333333703, 0.3333333333333333703, 0.3333333333333333703, 0.3333333333333333703, 0.3333333333333333703, 0.3333333333333333703, 0.3333333333333333703, 0.3333333333333333703, 0.3333333333333333703, 0.3333333333333333703, 0.3333333333333333703, 0.3333333333333333703, 0.3333333333333333703, 0.3333333333333333703, 0.3333333333333333703, 0.3333333333333333703, 0.3333333333333333703, 0.3333333333333333703, 0.3333333333333333703, 0.3333333333333333703, 0.3333333333333333703, 0.3333333333333333703, 0.3333333333333333703, 0.3333333333333333703, 0.3333333333333333703, 0.3333333333333333703, 0.3333333333333333703, 0.3333333333333333703, 0.3333333333333333703, 0.3333333333333333703, 0.3333333333333333703, 0.3333333333333333703, 0.3333333333333333703, 0.3333333333333333703, 0.3333333333333333703, 0.3333333333333333703, 0.3333333333333333703, 0.3333333333333333703, 0.3333333333333333703, 0.3333333333333333703, 0.3333333333333333703, 0.3333333333333333703, 0.3333333333333333703, 0.3333333333333333703, 0.3333333333333333703, 0.3333333333333333703, 0.3333333333333333703, 0.3333333333333333703, 0.3333333333333333703, 0.3333333333333333703, 0.3333333333333333703, 0.3333333333333333703, 0.3333333333333333703, 0.3333333333333333703, 0.3333333333333333703, 0.3333333333333333703, 0.3333333333333333703, 0.3333333333333333703, 0.3333333333333333703, 0.3333333333333333703, 0.3333333333333333703, 0.3333333333333333703, 0.3333333333333333703, 0.3333333333333333703, 0.3333333333333333703, 0.3333333333333333703, 0.3333333333333333703, 0.3333333333333333703, 0.3333333333333333703, 0.3333333333333333703, 0.3333333333333333703, 0.3333333333333333703, 0.3333333333333333703, 0.3333333333333333703, 0.3333333333333333703, 0.3333333333333333703, 0.3333333333333333703, 0.3333333333333333703, 0.3333333333333333703, 0.3333333333333333703, 0.3333333333333333703, 0.3333333333333333703, 0.3333333333333333703, 0.3333333333333333703, 0.3333333333333333703, 0.3333333333333333703, 0.3333333333333333703, 0.3333333333333333703, 0.3333333333333333703, 0.3333333333333333703, 0.3333333333333333703, 0.3333333333333333703, 0.3333333333333333703, 0.3333333333333333703, 0.3333333333333333703, 0.3333333333333333703, 0.3333333333333333703, 0.3333333333333333703, 0.3333333333333333703, 0.3333333333333333703, 0.3333333333333333703, 0.3333333333333333703, 0.3333333333333333703, 0.3333333333333333703, 0.3333333333333333703, 0.3333333333333333703, 0.3333333333333333703, 0.3333333333333333703, 0.3333333333333333703, 0.3333333333333333703, 0.3333333333333333703, 0.3333333333333333703, 0.3333333333333333703, 0.3333333333333333703, 0.3333333333333333703, 0.3333333333333333703, 0.3333333333333333703, 0.3333333333333333703, 0.3333333333333333703, 0.3333333333333333703, 0.3333333333333333703, 0.3333333333333333703, 0.3333333333333333703, 0.3333333333333333703, 0.3333333333333333703, 0.3333333333333333703, 0.3333333333333333703, 0.3333333333333333703, 0.3333333333333333703, 0.3333333333333333703, 0.3333333333333333703, 0.3333333333333333703, 0.3333333333333333703, 0.3333333333333333703, 0.3333333333333333703, 0.3333333333333333703, 0.3333333333333333703, 0.3333333333333333703, 0.3333333333333333703, 0.3333333333333333703, 0.3333333333333333703, 0.3333333333333333703, 0.3333333333333333703, 0.3333333333333333703, 0.3333333333333333703, 0.3333333333333333703, 0.3333333333333333703, 0.3333333333333333703, 0.3333333333333333703, 0.3333333333333333703, 0.3333333333333333703, 0.3333333333333333703, 0.3333333333333333703, 0.3333333333333333703, 0.3333333333333333703, 0.3333333333333333703, 0.3333333333333333703, 0.3333333333333333703, 0.3333333333333333703, 0.3333333333333333703, 0.3333333333333333703, 0.3333333333333333703),
 ( 0.3333333333333333703, 0.3333333333333333703, 0.3333333333333333703, 0.3333333333333333703, 0.3333333333333333703, 0.3333333333333333703, 0.3333333333333333703, 0.3333333333333333703, 0.3333333333333333703, 0.3333333333333333703, 0.3333333333333333703, 0.3333333333333333703, 0.3333333333333333703, 0.3333333333333333703, 0.3333333333333333703, 0.3333333333333333703, 0.3333333333333333703, 0.3333333333333333703, 0.3333333333333333703, 0.3333333333333333703, 0.3333333333333333703, 0.3333333333333333703, 0.3333333333333333703, 0.3333333333333333703, 0.3333333333333333703, 0.3333333333333333703, 0.3333333333333333703, 0.3333333333333333703, 0.3333333333333333703, 0.3333333333333333703, 0.3333333333333333703, 0.3333333333333333703, 0.3333333333333333703, 0.3333333333333333703, 0.3333333333333333703, 0.3333333333333333703, 0.3333333333333333703, 0.3333333333333333703, 0.3333333333333333703, 0.3333333333333333703, 0.3333333333333333703, 0.3333333333333333703, 0.3333333333333333703, 0.3333333333333333703, 0.3333333333333333703, 0.3333333333333333703, 0.3333333333333333703, 0.3333333333333333703, 0.3333333333333333703, 0.3333333333333333703, 0.3333333333333333703, 0.3333333333333333703, 0.3333333333333333703, 0.3333333333333333703, 0.3333333333333333703, 0.3333333333333333703, 0.3333333333333333703, 0.3333333333333333703, 0.3333333333333333703, 0.3333333333333333703, 0.3333333333333333703, 0.3333333333333333703, 0.3333333333333333703, 0.3333333333333333703, 0.3333333333333333703, 0.3333333333333333703, 0.3333333333333333703, 0.3333333333333333703, 0.3333333333333333703, 0.3333333333333333703, 0.3333333333333333703, 0.3333333333333333703, 0.3333333333333333703, 0.3333333333333333703, 0.3333333333333333703, 0.3333333333333333703, 0.3333333333333333703, 0.3333333333333333703, 0.3333333333333333703, 0.3333333333333333703, 0.3333333333333333703, 0.3333333333333333703, 0.3333333333333333703, 0.3333333333333333703, 0.3333333333333333703, 0.3333333333333333703, 0.3333333333333333703, 0.3333333333333333703, 0.3333333333333333703, 0.3333333333333333703, 0.3333333333333333703, 0.3333333333333333703, 0.3333333333333333703, 0.3333333333333333703, 0.3333333333333333703, 0.3333333333333333703, 0.3333333333333333703, 0.3333333333333333703, 0.3333333333333333703, 0.3333333333333333703, 0.3333333333333333703, 0.3333333333333333703, 0.3333333333333333703, 0.3333333333333333703, 0.3333333333333333703, 0.3333333333333333703, 0.3333333333333333703, 0.3333333333333333703, 0.3333333333333333703, 0.3333333333333333703, 0.3333333333333333703, 0.3333333333333333703, 0.3333333333333333703, 0.3333333333333333703, 0.3333333333333333703, 0.3333333333333333703, 0.3333333333333333703, 0.3333333333333333703, 0.3333333333333333703, 0.3333333333333333703, 0.3333333333333333703, 0.3333333333333333703, 0.3333333333333333703, 0.3333333333333333703, 0.3333333333333333703, 0.3333333333333333703, 0.3333333333333333703, 0.3333333333333333703, 0.3333333333333333703, 0.3333333333333333703, 0.3333333333333333703, 0.3333333333333333703, 0.3333333333333333703, 0.3333333333333333703, 0.3333333333333333703, 0.3333333333333333703, 0.3333333333333333703, 0.3333333333333333703, 0.3333333333333333703, 0.3333333333333333703, 0.3333333333333333703, 0.3333333333333333703, 0.3333333333333333703, 0.3333333333333333703, 0.3333333333333333703, 0.3333333333333333703, 0.3333333333333333703, 0.3333333333333333703, 0.3333333333333333703, 0.3333333333333333703, 0.3333333333333333703, 0.3333333333333333703, 0.3333333333333333703, 0.3333333333333333703, 0.3333333333333333703, 0.3333333333333333703, 0.3333333333333333703, 0.3333333333333333703, 0.3333333333333333703, 0.3333333333333333703, 0.3333333333333333703, 0.3333333333333333703, 0.3333333333333333703, 0.3333333333333333703, 0.3333333333333333703, 0.3333333333333333703, 0.3333333333333333703, 0.3333333333333333703, 0.3333333333333333703, 0.3333333333333333703, 0.3333333333333333703, 0.3333333333333333703, 0.3333333333333333703, 0.3333333333333333703, 0.3333333333333333703, 0.3333333333333333703, 0.3333333333333333703, 0.3333333333333333703, 0.3333333333333333703, 0.3333333333333333703, 0.3333333333333333703, 0.3333333333333333703, 0.3333333333333333703, 0.3333333333333333703, 0.3333333333333333703, 0.3333333333333333703, 0.3333333333333333703, 0.3333333333333333703, 0.3333333333333333703, 0.3333333333333333703, 0.3333333333333333703, 0.3333333333333333703, 0.3333333333333333703, 0.3333333333333333703, 0.3333333333333333703, 0.3333333333333333703, 0.3333333333333333703, 0.3333333333333333703, 0.3333333333333333703, 0.3333333333333333703, 0.3333333333333333703, 0.3333333333333333703, 0.3333333333333333703, 0.3333333333333333703, 0.3333333333333333703, 0.3333333333333333703, 0.3333333333333333703, 0.3333333333333333703, 0.3333333333333333703, 0.3333333333333333703, 0.3333333333333333703, 0.3333333333333333703, 0.3333333333333333703, 0.3333333333333333703, 0.3333333333333333703, 0.3333333333333333703, 0.3333333333333333703, 0.3333333333333333703, 0.3333333333333333703, 0.3333333333333333703, 0.3333333333333333703, 0.3333333333333333703, 0.3333333333333333703, 0.3333333333333333703, 0.3333333333333333703, 0.3333333333333333703, 0.3333333333333333703, 0.3333333333333333703, 0.3333333333333333703, 0.3333333333333333703, 0.3333333333333333703, 0.3333333333333333703, 0.3333333333333333703, 0.3333333333333333703, 0.3333333333333333703, 0.3333333333333333703, 0.3333333333333333703, 0.3333333333333333703, 0.3333333333333333703, 0.3333333333333333703, 0.3333333333333333703, 0.3333333333333333703, 0.3333333333333333703, 0.3333333333333333703, 0.3333333333333333703, 0.3333333333333333703, 0.3333333333333333703, 0.3333333333333333703, 0.3333333333333333703, 0.3333333333333333703, 0.3333333333333333703, 0.3333333333333333703, 0.3333333333333333703, 0.3333333333333333703, 0.3333333333333333703, 0.3333333333333333703, 0.3333333333333333703, 0.3333333333333333703, 0.3333333333333333703, 0.3333333333333333703, 0.3333333333333333703, 0.3333333333333333703, 0.3333333333333333703, 0.3333333333333333703, 0.3333333333333333703, 0.3333333333333333703, 0.3333333333333333703, 0.3333333333333333703, 0.3333333333333333703, 0.3333333333333333703, 0.3333333333333333703, 0.3333333333333333703, 0.3333333333333333703, 0.3333333333333333703, 0.3333333333333333703, 0.3333333333333333703, 0.3333333333333333703, 0.3333333333333333703, 0.3333333333333333703, 0.3333333333333333703, 0.3333333333333333703, 0.3333333333333333703, 0.3333333333333333703, 0.3333333333333333703, 0.3333333333333333703, 0.3333333333333333703, 0.3333333333333333703, 0.3333333333333333703, 0.3333333333333333703, 0.3333333333333333703, 0.3333333333333333703, 0.3333333333333333703, 0.3333333333333333703, 0.3333333333333333703, 0.3333333333333333703, 0.3333333333333333703, 0.3333333333333333703, 0.3333333333333333703, 0.3333333333333333703, 0.3333333333333333703, 0.3333333333333333703, 0.3333333333333333703, 0.3333333333333333703, 0.3333333333333333703, 0.3333333333333333703, 0.3333333333333333703, 0.3333333333333333703, 0.3333333333333333703, 0.3333333333333333703, 0.3333333333333333703, 0.3333333333333333703, 0.3333333333333333703, 0.3333333333333333703, 0.3333333333333333703, 0.3333333333333333703, 0.3333333333333333703, 0.3333333333333333703, 0.3333333333333333703, 0.3333333333333333703, 0.3333333333333333703, 0.3333333333333333703, 0.3333333333333333703, 0.3333333333333333703, 0.3333333333333333703, 0.3333333333333333703, 0.3333333333333333703, 0.3333333333333333703, 0.3333333333333333703, 0.3333333333333333703, 0.3333333333333333703, 0.3333333333333333703, 0.3333333333333333703, 0.3333333333333333703, 0.3333333333333333703, 0.3333333333333333703, 0.3333333333333333703, 0.3333333333333333703, 0.3333333333333333703, 0.3333333333333333703, 0.3333333333333333703),
 ( 1.000000000000000000, 1.000000000000000000, 1.000000000000000000, 1.000000000000000000, 1.000000000000000000, 1.000000000000000000, 1.000000000000000000, 1.000000000000000000, 1.000000000000000000, 1.000000000000000000, 1.000000000000000000, 1.000000000000000000, 1.000000000000000000, 1.000000000000000000, 1.000000000000000000, 1.000000000000000000, 1.000000000000000000, 1.000000000000000000, 1.000000000000000000, 1.000000000000000000, 1.000000000000000000, 1.000000000000000000, 1.000000000000000000, 1.000000000000000000, 1.000000000000000000, 1.000000000000000000, 1.000000000000000000, 1.000000000000000000, 1.000000000000000000, 1.000000000000000000, 1.000000000000000000, 1.000000000000000000, 1.000000000000000000, 1.000000000000000000, 1.000000000000000000, 1.000000000000000000, 1.000000000000000000, 1.000000000000000000, 1.000000000000000000, 1.000000000000000000, 1.000000000000000000, 1.000000000000000000, 1.000000000000000000, 1.000000000000000000, 1.000000000000000000, 1.000000000000000000, 1.000000000000000000, 1.000000000000000000, 1.000000000000000000, 1.000000000000000000, 1.000000000000000000, 1.000000000000000000, 1.000000000000000000, 1.000000000000000000, 1.000000000000000000, 1.000000000000000000, 1.000000000000000000, 1.000000000000000000, 1.000000000000000000, 1.000000000000000000, 1.000000000000000000, 1.000000000000000000, 1.000000000000000000, 1.000000000000000000, 1.000000000000000000, 1.000000000000000000, 1.000000000000000000, 1.000000000000000000, 1.000000000000000000, 1.000000000000000000, 1.000000000000000000, 1.000000000000000000, 1.000000000000000000, 1.000000000000000000, 1.000000000000000000, 1.000000000000000000, 1.000000000000000000, 1.000000000000000000, 1.000000000000000000, 1.000000000000000000, 1.000000000000000000, 1.000000000000000000, 1.000000000000000000, 1.000000000000000000, 1.000000000000000000, 1.000000000000000000, 1.000000000000000000, 1.000000000000000000, 1.000000000000000000, 1.000000000000000000, 1.000000000000000000, 1.000000000000000000, 1.000000000000000000, 1.000000000000000000, 1.000000000000000000, 1.000000000000000000, 1.000000000000000000, 1.000000000000000000, 1.000000000000000000, 1.000000000000000000, 1.000000000000000000, 1.000000000000000000, 1.000000000000000000, 1.000000000000000000, 1.000000000000000000, 1.000000000000000000, 1.000000000000000000, 1.000000000000000000, 1.000000000000000000, 1.000000000000000000, 1.000000000000000000, 1.000000000000000000, 1.000000000000000000, 1.000000000000000000, 1.000000000000000000, 1.000000000000000000, 1.000000000000000000, 1.000000000000000000, 1.000000000000000000, 1.000000000000000000, 1.000000000000000000, 1.000000000000000000, 1.000000000000000000, 1.000000000000000000, 1.000000000000000000, 1.000000000000000000, 1.000000000000000000, 1.000000000000000000, 1.000000000000000000, 1.000000000000000000, 1.000000000000000000, 1.000000000000000000, 1.000000000000000000, 1.000000000000000000, 1.000000000000000000, 1.000000000000000000, 1.000000000000000000, 1.000000000000000000, 1.000000000000000000, 1.000000000000000000, 1.000000000000000000, 1.000000000000000000, 1.000000000000000000, 1.000000000000000000, 1.000000000000000000, 1.000000000000000000, 1.000000000000000000, 1.000000000000000000, 1.000000000000000000, 1.000000000000000000, 1.000000000000000000, 1.000000000000000000, 1.000000000000000000, 1.000000000000000000, 1.000000000000000000, 1.000000000000000000, 1.000000000000000000, 1.000000000000000000, 1.000000000000000000, 1.000000000000000000, 1.000000000000000000, 1.000000000000000000, 1.000000000000000000, 1.000000000000000000, 1.000000000000000000, 1.000000000000000000, 1.000000000000000000, 1.000000000000000000, 1.000000000000000000, 1.000000000000000000, 1.000000000000000000, 1.000000000000000000, 1.000000000000000000, 1.000000000000000000, 1.000000000000000000, 1.000000000000000000, 1.000000000000000000, 1.000000000000000000, 1.000000000000000000, 1.000000000000000000, 1.000000000000000000, 1.000000000000000000, 1.000000000000000000, 1.000000000000000000, 1.000000000000000000, 1.000000000000000000, 1.000000000000000000, 1.000000000000000000, 1.000000000000000000, 1.000000000000000000, 1.000000000000000000, 1.000000000000000000, 1.000000000000000000, 1.000000000000000000, 1.000000000000000000, 1.000000000000000000, 1.000000000000000000, 1.000000000000000000, 1.000000000000000000, 1.000000000000000000, 1.000000000000000000, 1.000000000000000000, 1.000000000000000000, 1.000000000000000000, 1.000000000000000000, 1.000000000000000000, 1.000000000000000000, 1.000000000000000000, 1.000000000000000000, 1.000000000000000000, 1.000000000000000000, 1.000000000000000000, 1.000000000000000000, 1.000000000000000000, 1.000000000000000000, 1.000000000000000000, 1.000000000000000000, 1.000000000000000000, 1.000000000000000000, 1.000000000000000000, 1.000000000000000000, 1.000000000000000000, 1.000000000000000000, 1.000000000000000000, 1.000000000000000000, 1.000000000000000000, 1.000000000000000000, 1.000000000000000000, 1.000000000000000000, 1.000000000000000000, 1.000000000000000000, 1.000000000000000000, 1.000000000000000000, 1.000000000000000000, 1.000000000000000000, 1.000000000000000000, 1.000000000000000000, 1.000000000000000000, 1.000000000000000000, 1.000000000000000000, 1.000000000000000000, 1.000000000000000000, 1.000000000000000000, 1.000000000000000000, 1.000000000000000000, 1.000000000000000000, 1.000000000000000000, 1.000000000000000000, 1.000000000000000000, 1.000000000000000000, 1.000000000000000000, 1.000000000000000000, 1.000000000000000000, 1.000000000000000000, 1.000000000000000000, 1.000000000000000000, 1.000000000000000000, 1.000000000000000000, 1.000000000000000000, 1.000000000000000000, 1.000000000000000000, 1.000000000000000000, 1.000000000000000000, 1.000000000000000000, 1.000000000000000000, 1.000000000000000000, 1.000000000000000000, 1.000000000000000000, 1.000000000000000000, 1.000000000000000000, 1.000000000000000000, 1.000000000000000000, 1.000000000000000000, 1.000000000000000000, 1.000000000000000000, 1.000000000000000000, 1.000000000000000000, 1.000000000000000000, 1.000000000000000000, 1.000000000000000000, 1.000000000000000000, 1.000000000000000000, 1.000000000000000000, 1.000000000000000000, 1.000000000000000000, 1.000000000000000000, 1.000000000000000000, 1.000000000000000000, 1.000000000000000000, 1.000000000000000000, 1.000000000000000000, 1.000000000000000000, 1.000000000000000000, 1.000000000000000000, 1.000000000000000000, 1.000000000000000000, 1.000000000000000000, 1.000000000000000000, 1.000000000000000000, 1.000000000000000000, 1.000000000000000000, 1.000000000000000000, 1.000000000000000000, 1.000000000000000000, 1.000000000000000000, 1.000000000000000000, 1.000000000000000000, 1.000000000000000000, 1.000000000000000000, 1.000000000000000000, 1.000000000000000000, 1.000000000000000000, 1.000000000000000000, 1.000000000000000000, 1.000000000000000000, 1.000000000000000000, 1.000000000000000000, 1.000000000000000000, 1.000000000000000000, 1.000000000000000000, 1.000000000000000000, 1.000000000000000000, 1.000000000000000000, 1.000000000000000000, 1.000000000000000000, 1.000000000000000000, 1.000000000000000000, 1.000000000000000000, 1.000000000000000000, 1.000000000000000000, 1.000000000000000000, 1.000000000000000000, 1.000000000000000000, 1.000000000000000000, 1.000000000000000000, 1.000000000000000000, 1.000000000000000000, 1.000000000000000000, 1.000000000000000000, 1.000000000000000000),
 ( 0.3333333333333333703, 0.3333333333333333703, 0.3333333333333333703, 0.3333333333333333703, 0.3333333333333333703, 0.3333333333333333703, 0.3333333333333333703, 0.3333333333333333703, 0.3333333333333333703, 0.3333333333333333703, 0.3333333333333333703, 0.3333333333333333703, 0.3333333333333333703, 0.3333333333333333703, 0.3333333333333333703, 0.3333333333333333703, 0.3333333333333333703, 0.3333333333333333703, 0.3333333333333333703, 0.3333333333333333703, 0.3333333333333333703, 0.3333333333333333703, 0.3333333333333333703, 0.3333333333333333703, 0.3333333333333333703, 0.3333333333333333703, 0.3333333333333333703, 0.3333333333333333703, 0.3333333333333333703, 0.3333333333333333703, 0.3333333333333333703, 0.3333333333333333703, 0.3333333333333333703, 0.3333333333333333703, 0.3333333333333333703, 0.3333333333333333703, 0.3333333333333333703, 0.3333333333333333703, 0.3333333333333333703, 0.3333333333333333703, 0.3333333333333333703, 0.3333333333333333703, 0.3333333333333333703, 0.3333333333333333703, 0.3333333333333333703, 0.3333333333333333703, 0.3333333333333333703, 0.3333333333333333703, 0.3333333333333333703, 0.3333333333333333703, 0.3333333333333333703, 0.3333333333333333703, 0.3333333333333333703, 0.3333333333333333703, 0.3333333333333333703, 0.3333333333333333703, 0.3333333333333333703, 0.3333333333333333703, 0.3333333333333333703, 0.3333333333333333703, 0.3333333333333333703, 0.3333333333333333703, 0.3333333333333333703, 0.3333333333333333703, 0.3333333333333333703, 0.3333333333333333703, 0.3333333333333333703, 0.3333333333333333703, 0.3333333333333333703, 0.3333333333333333703, 0.3333333333333333703, 0.3333333333333333703, 0.3333333333333333703, 0.3333333333333333703, 0.3333333333333333703, 0.3333333333333333703, 0.3333333333333333703, 0.3333333333333333703, 0.3333333333333333703, 0.3333333333333333703, 0.3333333333333333703, 0.3333333333333333703, 0.3333333333333333703, 0.3333333333333333703, 0.3333333333333333703, 0.3333333333333333703, 0.3333333333333333703, 0.3333333333333333703, 0.3333333333333333703, 0.3333333333333333703, 0.3333333333333333703, 0.3333333333333333703, 0.3333333333333333703, 0.3333333333333333703, 0.3333333333333333703, 0.3333333333333333703, 0.3333333333333333703, 0.3333333333333333703, 0.3333333333333333703, 0.3333333333333333703, 0.3333333333333333703, 0.3333333333333333703, 0.3333333333333333703, 0.3333333333333333703, 0.3333333333333333703, 0.3333333333333333703, 0.3333333333333333703, 0.3333333333333333703, 0.3333333333333333703, 0.3333333333333333703, 0.3333333333333333703, 0.3333333333333333703, 0.3333333333333333703, 0.3333333333333333703, 0.3333333333333333703, 0.3333333333333333703, 0.3333333333333333703, 0.3333333333333333703, 0.3333333333333333703, 0.3333333333333333703, 0.3333333333333333703, 0.3333333333333333703, 0.3333333333333333703, 0.3333333333333333703, 0.3333333333333333703, 0.3333333333333333703, 0.3333333333333333703, 0.3333333333333333703, 0.3333333333333333703, 0.3333333333333333703, 0.3333333333333333703, 0.3333333333333333703, 0.3333333333333333703, 0.3333333333333333703, 0.3333333333333333703, 0.3333333333333333703, 0.3333333333333333703, 0.3333333333333333703, 0.3333333333333333703, 0.3333333333333333703, 0.3333333333333333703, 0.3333333333333333703, 0.3333333333333333703, 0.3333333333333333703, 0.3333333333333333703, 0.3333333333333333703, 0.3333333333333333703, 0.3333333333333333703, 0.3333333333333333703, 0.3333333333333333703, 0.3333333333333333703, 0.3333333333333333703, 0.3333333333333333703, 0.3333333333333333703, 0.3333333333333333703, 0.3333333333333333703, 0.3333333333333333703, 0.3333333333333333703, 0.3333333333333333703, 0.3333333333333333703, 0.3333333333333333703, 0.3333333333333333703, 0.3333333333333333703, 0.3333333333333333703, 0.3333333333333333703, 0.3333333333333333703, 0.3333333333333333703, 0.3333333333333333703, 0.3333333333333333703, 0.3333333333333333703, 0.3333333333333333703, 0.3333333333333333703, 0.3333333333333333703, 0.3333333333333333703, 0.3333333333333333703, 0.3333333333333333703, 0.3333333333333333703, 0.3333333333333333703, 0.3333333333333333703, 0.3333333333333333703, 0.3333333333333333703, 0.3333333333333333703, 0.3333333333333333703, 0.3333333333333333703, 0.3333333333333333703, 0.3333333333333333703, 0.3333333333333333703, 0.3333333333333333703, 0.3333333333333333703, 0.3333333333333333703, 0.3333333333333333703, 0.3333333333333333703, 0.3333333333333333703, 0.3333333333333333703, 0.3333333333333333703, 0.3333333333333333703, 0.3333333333333333703, 0.3333333333333333703, 0.3333333333333333703, 0.3333333333333333703, 0.3333333333333333703, 0.3333333333333333703, 0.3333333333333333703, 0.3333333333333333703, 0.3333333333333333703, 0.3333333333333333703, 0.3333333333333333703, 0.3333333333333333703, 0.3333333333333333703, 0.3333333333333333703, 0.3333333333333333703, 0.3333333333333333703, 0.3333333333333333703, 0.3333333333333333703, 0.3333333333333333703, 0.3333333333333333703, 0.3333333333333333703, 0.3333333333333333703, 0.3333333333333333703, 0.3333333333333333703, 0.3333333333333333703, 0.3333333333333333703, 0.3333333333333333703, 0.3333333333333333703, 0.3333333333333333703, 0.3333333333333333703, 0.3333333333333333703, 0.3333333333333333703, 0.3333333333333333703, 0.3333333333333333703, 0.3333333333333333703, 0.3333333333333333703, 0.3333333333333333703, 0.3333333333333333703, 0.3333333333333333703, 0.3333333333333333703, 0.3333333333333333703, 0.3333333333333333703, 0.3333333333333333703, 0.3333333333333333703, 0.3333333333333333703, 0.3333333333333333703, 0.3333333333333333703, 0.3333333333333333703, 0.3333333333333333703, 0.3333333333333333703, 0.3333333333333333703, 0.3333333333333333703, 0.3333333333333333703, 0.3333333333333333703, 0.3333333333333333703, 0.3333333333333333703, 0.3333333333333333703, 0.3333333333333333703, 0.3333333333333333703, 0.3333333333333333703, 0.3333333333333333703, 0.3333333333333333703, 0.3333333333333333703, 0.3333333333333333703, 0.3333333333333333703, 0.3333333333333333703, 0.3333333333333333703, 0.3333333333333333703, 0.3333333333333333703, 0.3333333333333333703, 0.3333333333333333703, 0.3333333333333333703, 0.3333333333333333703, 0.3333333333333333703, 0.3333333333333333703, 0.3333333333333333703, 0.3333333333333333703, 0.3333333333333333703, 0.3333333333333333703, 0.3333333333333333703, 0.3333333333333333703, 0.3333333333333333703, 0.3333333333333333703, 0.3333333333333333703, 0.3333333333333333703, 0.3333333333333333703, 0.3333333333333333703, 0.3333333333333333703, 0.3333333333333333703, 0.3333333333333333703, 0.3333333333333333703, 0.3333333333333333703, 0.3333333333333333703, 0.3333333333333333703, 0.3333333333333333703, 0.3333333333333333703, 0.3333333333333333703, 0.3333333333333333703, 0.3333333333333333703, 0.3333333333333333703, 0.3333333333333333703, 0.3333333333333333703, 0.3333333333333333703, 0.3333333333333333703, 0.3333333333333333703, 0.3333333333333333703, 0.3333333333333333703, 0.3333333333333333703, 0.3333333333333333703, 0.3333333333333333703, 0.3333333333333333703, 0.3333333333333333703, 0.3333333333333333703, 0.3333333333333333703, 0.3333333333333333703, 0.3333333333333333703, 0.3333333333333333703, 0.3333333333333333703, 0.3333333333333333703, 0.3333333333333333703, 0.3333333333333333703, 0.3333333333333333703, 0.3333333333333333703, 0.3333333333333333703, 0.3333333333333333703, 0.3333333333333333703, 0.3333333333333333703, 0.3333333333333333703, 0.3333333333333333703, 0.3333333333333333703, 0.3333333333333333703, 0.3333333333333333703, 0.3333333333333333703, 0.3333333333333333703, 0.3333333333333333703, 0.3333333333333333703, 0.3333333333333333703, 0.3333333333333333703, 0.3333333333333333703, 0.3333333333333333703, 0.3333333333333333703, 0.3333333333333333703, 0.3333333333333333703, 0.3333333333333333703),
 ( 0.3333333333333333703, 0.3333333333333333703, 0.3333333333333333703, 0.3333333333333333703, 0.3333333333333333703, 0.3333333333333333703, 0.3333333333333333703, 0.3333333333333333703, 0.3333333333333333703, 0.3333333333333333703, 0.3333333333333333703, 0.3333333333333333703, 0.3333333333333333703, 0.3333333333333333703, 0.3333333333333333703, 0.3333333333333333703, 0.3333333333333333703, 0.3333333333333333703, 0.3333333333333333703, 0.3333333333333333703, 0.3333333333333333703, 0.3333333333333333703, 0.3333333333333333703, 0.3333333333333333703, 0.3333333333333333703, 0.3333333333333333703, 0.3333333333333333703, 0.3333333333333333703, 0.3333333333333333703, 0.3333333333333333703, 0.3333333333333333703, 0.3333333333333333703, 0.3333333333333333703, 0.3333333333333333703, 0.3333333333333333703, 0.3333333333333333703, 0.3333333333333333703, 0.3333333333333333703, 0.3333333333333333703, 0.3333333333333333703, 0.3333333333333333703, 0.3333333333333333703, 0.3333333333333333703, 0.3333333333333333703, 0.3333333333333333703, 0.3333333333333333703, 0.3333333333333333703, 0.3333333333333333703, 0.3333333333333333703, 0.3333333333333333703, 0.3333333333333333703, 0.3333333333333333703, 0.3333333333333333703, 0.3333333333333333703, 0.3333333333333333703, 0.3333333333333333703, 0.3333333333333333703, 0.3333333333333333703, 0.3333333333333333703, 0.3333333333333333703, 0.3333333333333333703, 0.3333333333333333703, 0.3333333333333333703, 0.3333333333333333703, 0.3333333333333333703, 0.3333333333333333703, 0.3333333333333333703, 0.3333333333333333703, 0.3333333333333333703, 0.3333333333333333703, 0.3333333333333333703, 0.3333333333333333703, 0.3333333333333333703, 0.3333333333333333703, 0.3333333333333333703, 0.3333333333333333703, 0.3333333333333333703, 0.3333333333333333703, 0.3333333333333333703, 0.3333333333333333703, 0.3333333333333333703, 0.3333333333333333703, 0.3333333333333333703, 0.3333333333333333703, 0.3333333333333333703, 0.3333333333333333703, 0.3333333333333333703, 0.3333333333333333703, 0.3333333333333333703, 0.3333333333333333703, 0.3333333333333333703, 0.3333333333333333703, 0.3333333333333333703, 0.3333333333333333703, 0.3333333333333333703, 0.3333333333333333703, 0.3333333333333333703, 0.3333333333333333703, 0.3333333333333333703, 0.3333333333333333703, 0.3333333333333333703, 0.3333333333333333703, 0.3333333333333333703, 0.3333333333333333703, 0.3333333333333333703, 0.3333333333333333703, 0.3333333333333333703, 0.3333333333333333703, 0.3333333333333333703, 0.3333333333333333703, 0.3333333333333333703, 0.3333333333333333703, 0.3333333333333333703, 0.3333333333333333703, 0.3333333333333333703, 0.3333333333333333703, 0.3333333333333333703, 0.3333333333333333703, 0.3333333333333333703, 0.3333333333333333703, 0.3333333333333333703, 0.3333333333333333703, 0.3333333333333333703, 0.3333333333333333703, 0.3333333333333333703, 0.3333333333333333703, 0.3333333333333333703, 0.3333333333333333703, 0.3333333333333333703, 0.3333333333333333703, 0.3333333333333333703, 0.3333333333333333703, 0.3333333333333333703, 0.3333333333333333703, 0.3333333333333333703, 0.3333333333333333703, 0.3333333333333333703, 0.3333333333333333703, 0.3333333333333333703, 0.3333333333333333703, 0.3333333333333333703, 0.3333333333333333703, 0.3333333333333333703, 0.3333333333333333703, 0.3333333333333333703, 0.3333333333333333703, 0.3333333333333333703, 0.3333333333333333703, 0.3333333333333333703, 0.3333333333333333703, 0.3333333333333333703, 0.3333333333333333703, 0.3333333333333333703, 0.3333333333333333703, 0.3333333333333333703, 0.3333333333333333703, 0.3333333333333333703, 0.3333333333333333703, 0.3333333333333333703, 0.3333333333333333703, 0.3333333333333333703, 0.3333333333333333703, 0.3333333333333333703, 0.3333333333333333703, 0.3333333333333333703, 0.3333333333333333703, 0.3333333333333333703, 0.3333333333333333703, 0.3333333333333333703, 0.3333333333333333703, 0.3333333333333333703, 0.3333333333333333703, 0.3333333333333333703, 0.3333333333333333703, 0.3333333333333333703, 0.3333333333333333703, 0.3333333333333333703, 0.3333333333333333703, 0.3333333333333333703, 0.3333333333333333703, 0.3333333333333333703, 0.3333333333333333703, 0.3333333333333333703, 0.3333333333333333703, 0.3333333333333333703, 0.3333333333333333703, 0.3333333333333333703, 0.3333333333333333703, 0.3333333333333333703, 0.3333333333333333703, 0.3333333333333333703, 0.3333333333333333703, 0.3333333333333333703, 0.3333333333333333703, 0.3333333333333333703, 0.3333333333333333703, 0.3333333333333333703, 0.3333333333333333703, 0.3333333333333333703, 0.3333333333333333703, 0.3333333333333333703, 0.3333333333333333703, 0.3333333333333333703, 0.3333333333333333703, 0.3333333333333333703, 0.3333333333333333703, 0.3333333333333333703, 0.3333333333333333703, 0.3333333333333333703, 0.3333333333333333703, 0.3333333333333333703, 0.3333333333333333703, 0.3333333333333333703, 0.3333333333333333703, 0.3333333333333333703, 0.3333333333333333703, 0.3333333333333333703, 0.3333333333333333703, 0.3333333333333333703, 0.3333333333333333703, 0.3333333333333333703, 0.3333333333333333703, 0.3333333333333333703, 0.3333333333333333703, 0.3333333333333333703, 0.3333333333333333703, 0.3333333333333333703, 0.3333333333333333703, 0.3333333333333333703, 0.3333333333333333703, 0.3333333333333333703, 0.3333333333333333703, 0.3333333333333333703, 0.3333333333333333703, 0.3333333333333333703, 0.3333333333333333703, 0.3333333333333333703, 0.3333333333333333703, 0.3333333333333333703, 0.3333333333333333703, 0.3333333333333333703, 0.3333333333333333703, 0.3333333333333333703, 0.3333333333333333703, 0.3333333333333333703, 0.3333333333333333703, 0.3333333333333333703, 0.3333333333333333703, 0.3333333333333333703, 0.3333333333333333703, 0.3333333333333333703, 0.3333333333333333703, 0.3333333333333333703, 0.3333333333333333703, 0.3333333333333333703, 0.3333333333333333703, 0.3333333333333333703, 0.3333333333333333703, 0.3333333333333333703, 0.3333333333333333703, 0.3333333333333333703, 0.3333333333333333703, 0.3333333333333333703, 0.3333333333333333703, 0.3333333333333333703, 0.3333333333333333703, 0.3333333333333333703, 0.3333333333333333703, 0.3333333333333333703, 0.3333333333333333703, 0.3333333333333333703, 0.3333333333333333703, 0.3333333333333333703, 0.3333333333333333703, 0.3333333333333333703, 0.3333333333333333703, 0.3333333333333333703, 0.3333333333333333703, 0.3333333333333333703, 0.3333333333333333703, 0.3333333333333333703, 0.3333333333333333703, 0.3333333333333333703, 0.3333333333333333703, 0.3333333333333333703, 0.3333333333333333703, 0.3333333333333333703, 0.3333333333333333703, 0.3333333333333333703, 0.3333333333333333703, 0.3333333333333333703, 0.3333333333333333703, 0.3333333333333333703, 0.3333333333333333703, 0.3333333333333333703, 0.3333333333333333703, 0.3333333333333333703, 0.3333333333333333703, 0.3333333333333333703, 0.3333333333333333703, 0.3333333333333333703, 0.3333333333333333703, 0.3333333333333333703, 0.3333333333333333703, 0.3333333333333333703, 0.3333333333333333703, 0.3333333333333333703, 0.3333333333333333703, 0.3333333333333333703, 0.3333333333333333703, 0.3333333333333333703, 0.3333333333333333703, 0.3333333333333333703, 0.3333333333333333703, 0.3333333333333333703, 0.3333333333333333703, 0.3333333333333333703, 0.3333333333333333703, 0.3333333333333333703, 0.3333333333333333703, 0.3333333333333333703, 0.3333333333333333703, 0.3333333333333333703, 0.3333333333333333703, 0.3333333333333333703, 0.3333333333333333703, 0.3333333333333333703, 0.3333333333333333703, 0.3333333333333333703, 0.3333333333333333703, 0.3333333333333333703, 0.3333333333333333703, 0.3333333333333333703, 0.3333333333333333703, 0.3333333333333333703, 0.3333333333333333703, 0.3333333333333333703, 0.3333333333333333703, 0.3333333333333333703, 0.3333333333333333703),
 ( 1.000000000000000000, 1.000000000000000000, 1.000000000000000000, 1.000000000000000000, 1.000000000000000000, 1.000000000000000000, 1.000000000000000000, 1.000000000000000000, 1.000000000000000000, 1.000000000000000000, 1.000000000000000000, 1.000000000000000000, 1.000000000000000000, 1.000000000000000000, 1.000000000000000000, 1.000000000000000000, 1.000000000000000000, 1.000000000000000000, 1.000000000000000000, 1.000000000000000000, 1.000000000000000000, 1.000000000000000000, 1.000000000000000000, 1.000000000000000000, 1.000000000000000000, 1.000000000000000000, 1.000000000000000000, 1.000000000000000000, 1.000000000000000000, 1.000000000000000000, 1.000000000000000000, 1.000000000000000000, 1.000000000000000000, 1.000000000000000000, 1.000000000000000000, 1.000000000000000000, 1.000000000000000000, 1.000000000000000000, 1.000000000000000000, 1.000000000000000000, 1.000000000000000000, 1.000000000000000000, 1.000000000000000000, 1.000000000000000000, 1.000000000000000000, 1.000000000000000000, 1.000000000000000000, 1.000000000000000000, 1.000000000000000000, 1.000000000000000000, 1.000000000000000000, 1.000000000000000000, 1.000000000000000000, 1.000000000000000000, 1.000000000000000000, 1.000000000000000000, 1.000000000000000000, 1.000000000000000000, 1.000000000000000000, 1.000000000000000000, 1.000000000000000000, 1.000000000000000000, 1.000000000000000000, 1.000000000000000000, 1.000000000000000000, 1.000000000000000000, 1.000000000000000000, 1.000000000000000000, 1.000000000000000000, 1.000000000000000000, 1.000000000000000000, 1.000000000000000000, 1.000000000000000000, 1.000000000000000000, 1.000000000000000000, 1.000000000000000000, 1.000000000000000000, 1.000000000000000000, 1.000000000000000000, 1.000000000000000000, 1.000000000000000000, 1.000000000000000000, 1.000000000000000000, 1.000000000000000000, 1.000000000000000000, 1.000000000000000000, 1.000000000000000000, 1.000000000000000000, 1.000000000000000000, 1.000000000000000000, 1.000000000000000000, 1.000000000000000000, 1.000000000000000000, 1.000000000000000000, 1.000000000000000000, 1.000000000000000000, 1.000000000000000000, 1.000000000000000000, 1.000000000000000000, 1.000000000000000000, 1.000000000000000000, 1.000000000000000000, 1.000000000000000000, 1.000000000000000000, 1.000000000000000000, 1.000000000000000000, 1.000000000000000000, 1.000000000000000000, 1.000000000000000000, 1.000000000000000000, 1.000000000000000000, 1.000000000000000000, 1.000000000000000000, 1.000000000000000000, 1.000000000000000000, 1.000000000000000000, 1.000000000000000000, 1.000000000000000000, 1.000000000000000000, 1.000000000000000000, 1.000000000000000000, 1.000000000000000000, 1.000000000000000000, 1.000000000000000000, 1.000000000000000000, 1.000000000000000000, 1.000000000000000000, 1.000000000000000000, 1.000000000000000000, 1.000000000000000000, 1.000000000000000000, 1.000000000000000000, 1.000000000000000000, 1.000000000000000000, 1.000000000000000000, 1.000000000000000000, 1.000000000000000000, 1.000000000000000000, 1.000000000000000000, 1.000000000000000000, 1.000000000000000000, 1.000000000000000000, 1.000000000000000000, 1.000000000000000000, 1.000000000000000000, 1.000000000000000000, 1.000000000000000000, 1.000000000000000000, 1.000000000000000000, 1.000000000000000000, 1.000000000000000000, 1.000000000000000000, 1.000000000000000000, 1.000000000000000000, 1.000000000000000000, 1.000000000000000000, 1.000000000000000000, 1.000000000000000000, 1.000000000000000000, 1.000000000000000000, 1.000000000000000000, 1.000000000000000000, 1.000000000000000000, 1.000000000000000000, 1.000000000000000000, 1.000000000000000000, 1.000000000000000000, 1.000000000000000000, 1.000000000000000000, 1.000000000000000000, 1.000000000000000000, 1.000000000000000000, 1.000000000000000000, 1.000000000000000000, 1.000000000000000000, 1.000000000000000000, 1.000000000000000000, 1.000000000000000000, 1.000000000000000000, 1.000000000000000000, 1.000000000000000000, 1.000000000000000000, 1.000000000000000000, 1.000000000000000000, 1.000000000000000000, 1.000000000000000000, 1.000000000000000000, 1.000000000000000000, 1.000000000000000000, 1.000000000000000000, 1.000000000000000000, 1.000000000000000000, 1.000000000000000000, 1.000000000000000000, 1.000000000000000000, 1.000000000000000000, 1.000000000000000000, 1.000000000000000000, 1.000000000000000000, 1.000000000000000000, 1.000000000000000000, 1.000000000000000000, 1.000000000000000000, 1.000000000000000000, 1.000000000000000000, 1.000000000000000000, 1.000000000000000000, 1.000000000000000000, 1.000000000000000000, 1.000000000000000000, 1.000000000000000000, 1.000000000000000000, 1.000000000000000000, 1.000000000000000000, 1.000000000000000000, 1.000000000000000000, 1.000000000000000000, 1.000000000000000000, 1.000000000000000000, 1.000000000000000000, 1.000000000000000000, 1.000000000000000000, 1.000000000000000000, 1.000000000000000000, 1.000000000000000000, 1.000000000000000000, 1.000000000000000000, 1.000000000000000000, 1.000000000000000000, 1.000000000000000000, 1.000000000000000000, 1.000000000000000000, 1.000000000000000000, 1.000000000000000000, 1.000000000000000000, 1.000000000000000000, 1.000000000000000000, 1.000000000000000000, 1.000000000000000000, 1.000000000000000000, 1.000000000000000000, 1.000000000000000000, 1.000000000000000000, 1.000000000000000000, 1.000000000000000000, 1.000000000000000000, 1.000000000000000000, 1.000000000000000000, 1.000000000000000000, 1.000000000000000000, 1.000000000000000000, 1.000000000000000000, 1.000000000000000000, 1.000000000000000000, 1.000000000000000000, 1.000000000000000000, 1.000000000000000000, 1.000000000000000000, 1.000000000000000000, 1.000000000000000000, 1.000000000000000000, 1.000000000000000000, 1.000000000000000000, 1.000000000000000000, 1.000000000000000000, 1.000000000000000000, 1.000000000000000000, 1.000000000000000000, 1.000000000000000000, 1.000000000000000000, 1.000000000000000000, 1.000000000000000000, 1.000000000000000000, 1.000000000000000000, 1.000000000000000000, 1.000000000000000000, 1.000000000000000000, 1.000000000000000000, 1.000000000000000000, 1.000000000000000000, 1.000000000000000000, 1.000000000000000000, 1.000000000000000000, 1.000000000000000000, 1.000000000000000000, 1.000000000000000000, 1.000000000000000000, 1.000000000000000000, 1.000000000000000000, 1.000000000000000000, 1.000000000000000000, 1.000000000000000000, 1.000000000000000000, 1.000000000000000000, 1.000000000000000000, 1.000000000000000000, 1.000000000000000000, 1.000000000000000000, 1.000000000000000000, 1.000000000000000000, 1.000000000000000000, 1.000000000000000000, 1.000000000000000000, 1.000000000000000000, 1.000000000000000000, 1.000000000000000000, 1.000000000000000000, 1.000000000000000000, 1.000000000000000000, 1.000000000000000000, 1.000000000000000000, 1.000000000000000000, 1.000000000000000000, 1.000000000000000000, 1.000000000000000000, 1.000000000000000000, 1.000000000000000000, 1.000000000000000000, 1.000000000000000000, 1.000000000000000000, 1.000000000000000000, 1.000000000000000000, 1.000000000000000000, 1.000000000000000000, 1.000000000000000000, 1.000000000000000000, 1.000000000000000000, 1.000000000000000000, 1.000000000000000000, 1.000000000000000000, 1.000000000000000000, 1.000000000000000000, 1.000000000000000000, 1.000000000000000000, 1.000000000000000000, 1.000000000000000000, 1.000000000000000000, 1.000000000000000000, 1.000000000000000000, 1.000000000000000000) ) ) 
 REPRESENTATION_ITEM ( '' )  SURFACE ( )  );
#14513=CARTESIAN_POINT ( 'NONE',  ( -18.93763370444446181, -0.7340653299870684156, -219.7345063954518594 ) ) ;
#14514=CARTESIAN_POINT ( 'NONE',  ( 12.46318849118074112, 25.01309605388695445, -216.9820503660967859 ) ) ;
#14515=CARTESIAN_POINT ( 'NONE',  ( 24.57222455393806015, 12.08236629421828212, -229.7319216558644541 ) ) ;
#14517=CARTESIAN_POINT ( 'NONE',  ( -11.51027863121307782, -1.790843358437596677, -225.0773512427349203 ) ) ;
#14518=CARTESIAN_POINT ( 'NONE',  ( -11.06377138986482933, -15.30386857868810857, -217.0411070525910873 ) ) ;
#14519=CARTESIAN_POINT ( 'NONE',  ( 9.358654279681809740, -11.94480763145079472, -229.8864256833185777 ) ) ;
#14522=CARTESIAN_POINT ( 'NONE',  ( -1.696080206444520844, 14.74162257415073540, -222.2455536759108838 ) ) ;
#14523=CARTESIAN_POINT ( 'NONE',  ( 13.42370487565828796, -6.089723759188163221, -217.7532606872487406 ) ) ;
#14524=CARTESIAN_POINT ( 'NONE',  ( 15.50779141722566656, -5.694711448414747856, -219.6385356284298211 ) ) ;
#14526=CARTESIAN_POINT ( 'NONE',  ( -16.28025842329327944, 6.985656672962045732, -231.4191468057695715 ) ) ;
#14527=CARTESIAN_POINT ( 'NONE',  ( 22.20554449732931346, 18.01468431515759860, -218.9348803756412849 ) ) ;
#14528=CARTESIAN_POINT ( 'NONE',  ( 11.00580183749007190, 25.74996642444834904, -225.8602305833924788 ) ) ;
#14530=CARTESIAN_POINT ( 'NONE',  ( 7.898002370961310525, -21.57266348603731387, -216.1546105971396798 ) ) ;
#14532=CARTESIAN_POINT ( 'NONE',  ( 4.966801760238292118, 27.41406605988239420, -216.4490579899774900 ) ) ;
#14533=CARTESIAN_POINT ( 'NONE',  ( -8.929606928624414408, 11.65278034267609186, -219.1999234847403386 ) ) ;
#14534=CARTESIAN_POINT ( 'NONE',  ( -19.29805292978571885, -8.785194383212417080, -233.3520286081516133 ) ) ;
#14535=CARTESIAN_POINT ( 'NONE',  ( -16.65698539163286540, 11.03290537638306112, -233.6474915129378758 ) ) ;
#14536=FACE_OUTER_BOUND ( 'NONE', #4522, .T. ) ;
#14538=CARTESIAN_POINT ( 'NONE',  ( -7.266348978356541366, 16.38312187400933340, -217.9429203627011873 ) ) ;
#14539=CARTESIAN_POINT ( 'NONE',  ( -21.28804099221702018, -0.9277163183344186992, -219.0000000002572733 ) ) ;
#14540=CARTESIAN_POINT ( 'NONE',  ( -14.00380962569832199, 8.747390586476997854, -231.7950903513155936 ) ) ;
#14542=CARTESIAN_POINT ( 'NONE',  ( 21.39553407250273054, 8.453402029343234148, -217.9531594780983141 ) ) ;
#14545=CARTESIAN_POINT ( 'NONE',  ( -1.268862717067444024, 15.25222216985846480, -229.0661283592426116 ) ) ;
#14546=CARTESIAN_POINT ( 'NONE',  ( -20.76924187596804217, -21.50248317380421170, -228.3679492147379335 ) ) ;
#14547=CARTESIAN_POINT ( 'NONE',  ( 18.50911814746675788, 15.92944434255054453, -232.0449215596906072 ) ) ;
#14548=CARTESIAN_POINT ( 'NONE',  ( -9.869267615102224056, -25.54258770546914903, -218.7733540664615930 ) ) ;
#14550=CARTESIAN_POINT ( 'NONE',  ( -25.64868633208605786, 12.30364128039660798, -229.0020209687957049 ) ) ;
#14551=CARTESIAN_POINT ( 'NONE',  ( 18.24334571313621467, -21.83696521683136282, -220.5798317591433886 ) ) ;
#14552=CARTESIAN_POINT ( 'NONE',  ( 8.179023008129211902, 20.84698146175953681, -218.6376653143925921 ) ) ;
#14553=CARTESIAN_POINT ( 'NONE',  ( -13.37045227479810094, 5.250293981428504786, -224.2914120185227205 ) ) ;
#14554=CARTESIAN_POINT ( 'NONE',  ( -9.503027668167838726, 6.959046566381404730, -225.7241663910276941 ) ) ;
#14555=CARTESIAN_POINT ( 'NONE',  ( -10.33268794075157082, -17.24452578398873115, -232.5240627438851959 ) ) ;
#14556=CARTESIAN_POINT ( 'NONE',  ( 15.06072304412464291, 3.291435955319735651, -218.8606307204261725 ) ) ;
#14559=CARTESIAN_POINT ( 'NONE',  ( -18.91688971021567767, -12.73417920357403688, -235.2301191595167040 ) ) ;
#14560=CARTESIAN_POINT ( 'NONE',  ( 1.656472371294090085, 27.29382523973669095, -230.4991099578876117 ) ) ;
#14562=CARTESIAN_POINT ( 'NONE',  ( 15.39025625686376841, 1.044190007782545226, -218.9203249718910911 ) ) ;
#14563=CARTESIAN_POINT ( 'NONE',  ( -11.55316006017064012, 19.79513644261079719, -232.3088878043970453 ) ) ;
#14564=CARTESIAN_POINT ( 'NONE',  ( 17.04685026979186446, 18.05617612716381970, -216.0910122987878310 ) ) ;
#14566=CARTESIAN_POINT ( 'NONE',  ( 5.446054363465077763, -20.62119468428589997, -218.5301445808800622 ) ) ;
#14567=CARTESIAN_POINT ( 'NONE',  ( -5.805911442544755552, -26.83424102279996504, -229.6222293353685302 ) ) ;
#14568=CARTESIAN_POINT ( 'NONE',  ( 27.75679124201660741, 4.911524026080384075, -221.4430403652340829 ) ) ;
#14569=CARTESIAN_POINT ( 'NONE',  ( 19.06435866915521515, -20.24829071055443563, -218.8318535520223804 ) ) ;
#14570=CARTESIAN_POINT ( 'NONE',  ( -15.46216926290318305, -2.495270579625169738, -221.2150947962298631 ) ) ;
#14572=CARTESIAN_POINT ( 'NONE',  ( -9.294226473174397540, -12.00440878504259601, -219.6990993854437875 ) ) ;
#14573=CARTESIAN_POINT ( 'NONE',  ( 7.067550969709256670, 17.75197616922148569, -219.3387126207321955 ) ) ;
#14575=CARTESIAN_POINT ( 'NONE',  ( 14.18323607655884722, 3.286047475533308226, -222.8710065128477140 ) ) ;
#14576=CARTESIAN_POINT ( 'NONE',  ( 5.017623471397871349, 29.83561274492976878, -222.9769172135417250 ) ) ;
#14577=CARTESIAN_POINT ( 'NONE',  ( -0.7879796667336372851, 21.22375955577181372, -219.1554080315090118 ) ) ;
#14578=CARTESIAN_POINT ( 'NONE',  ( 20.72180063689699026, -9.651256082433341987, -234.7026181832539180 ) ) ;
#14580=CARTESIAN_POINT ( 'NONE',  ( 15.88043104796248528, 11.88135572392608807, -216.2525917828042168 ) ) ;
#14582=CARTESIAN_POINT ( 'NONE',  ( -22.38528940623734798, 16.50235888036280230, -227.1443357386333162 ) ) ;
#14583=CARTESIAN_POINT ( 'NONE',  ( -17.91769793922991028, 3.277678596821882007, -219.5526088240203819 ) ) ;
#14584=CARTESIAN_POINT ( 'NONE',  ( -5.980659577089002532, -19.45286470896024156, -217.9322865582606710 ) ) ;
#14587=CARTESIAN_POINT ( 'NONE',  ( 4.559463107227270662, 13.27337529356814017, -226.9596205199204633 ) ) ;
#14588=CARTESIAN_POINT ( 'NONE',  ( 16.32467020957917114, -16.75837631771952019, -218.4891864258081853 ) ) ;
#14590=CARTESIAN_POINT ( 'NONE',  ( -20.00523085820573499, 3.356386534894876927, -232.9491364426554298 ) ) ;
#14592=CARTESIAN_POINT ( 'NONE',  ( -7.460068573003235670, -29.58770008691625364, -228.1902472473001637 ) ) ;
#14593=CARTESIAN_POINT ( 'NONE',  ( -3.855805549595750392, 26.68244055262801950, -232.4569730455296508 ) ) ;
#14594=CARTESIAN_POINT ( 'NONE',  ( -4.695076324262313250, 31.85502299853856201, -223.8918597786031341 ) ) ;
#14596=CARTESIAN_POINT ( 'NONE',  ( -22.17339560624464312, 16.26550580028390769, -232.0582861498566274 ) ) ;
#14597=CARTESIAN_POINT ( 'NONE',  ( 18.84909589690502685, -4.856542942594316514, -217.9726137486037771 ) ) ;
#14600=CARTESIAN_POINT ( 'NONE',  ( -16.39453490553961856, 20.24836633112041184, -233.1722131570092245 ) ) ;
#14601=CARTESIAN_POINT ( 'NONE',  ( -4.226568860449858356, -15.17239585821433678, -217.2407179915541349 ) ) ;
#14602=CARTESIAN_POINT ( 'NONE',  ( 27.36047156164216787, -8.591464759722228450, -221.3690063136810977 ) ) ;
#14603=CARTESIAN_POINT ( 'NONE',  ( -11.46843428684449151, 6.508406145394057596, -225.7212143570321814 ) ) ;
#14604=CARTESIAN_POINT ( 'NONE',  ( -29.50764134580612463, 7.783340782857166573, -219.9768238800827191 ) ) ;
#14605=CARTESIAN_POINT ( 'NONE',  ( -4.824452364631481416, 22.01523768541901305, -216.8350837474290245 ) ) ;
#14606=CARTESIAN_POINT ( 'NONE',  ( -29.30406754532526037, 5.063969254119831120, -221.8212091093853076 ) ) ;
#14607=CARTESIAN_POINT ( 'NONE',  ( 14.23294950300690331, 6.961167337017927892, -222.0879133937260974 ) ) ;
#14608=CARTESIAN_POINT ( 'NONE',  ( -14.04270955969662360, -23.25437626513260980, -222.0989702864435174 ) ) ;
#14609=CIRCLE ( 'NONE', #4879, 1.000000000000013323 ) ;
#14612=CARTESIAN_POINT ( 'NONE',  ( 6.566035546683759883, 15.06745272174450712, -218.8330720708048034 ) ) ;
#14613=CARTESIAN_POINT ( 'NONE',  ( -11.83954511762131112, 10.58068896997146346, -226.6171226499791089 ) ) ;
#14614=CARTESIAN_POINT ( 'NONE',  ( -14.64425879132321384, 10.88727730234500868, -217.2315376225554644 ) ) ;
#14615=CARTESIAN_POINT ( 'NONE',  ( -28.53682043726378836, -3.412203979905605866, -221.0207037827091767 ) ) ;
#14618=CARTESIAN_POINT ( 'NONE',  ( -15.15110768032078070, 3.517015312212880218, -219.5479300368539270 ) ) ;
#14619=CARTESIAN_POINT ( 'NONE',  ( -8.876630286717240637, -14.53920553942005256, -232.5681369007955368 ) ) ;
#14620=CARTESIAN_POINT ( 'NONE',  ( 13.50203797739595402, 0.4864885784468633290, -227.9631964266715443 ) ) ;
#14621=CARTESIAN_POINT ( 'NONE',  ( 0.4042326456706432647, 15.50845657815858303, -219.2680337625893401 ) ) ;
#14624=CARTESIAN_POINT ( 'NONE',  ( -19.35155980425159683, 1.157993580480985552, -230.3698774940947942 ) ) ;
#14626=CARTESIAN_POINT ( 'NONE',  ( 19.29971334243027314, 24.42889259816135095, -228.2141526116784291 ) ) ;
#14627=CARTESIAN_POINT ( 'NONE',  ( 18.29617186523616468, 23.20920553663278341, -223.4372550713720216 ) ) ;
#14629=CARTESIAN_POINT ( 'NONE',  ( -13.08850661186922260, -6.354795836388488439, -231.9371199848366984 ) ) ;
#14630=CARTESIAN_POINT ( 'NONE',  ( -28.46519324992292965, -8.397260794665152517, -225.6705986409035347 ) ) ;
#14632=CARTESIAN_POINT ( 'NONE',  ( -11.24282496690421596, 12.44430180464951086, -232.4405891940542404 ) ) ;
#14633=CARTESIAN_POINT ( 'NONE',  ( -6.079211283031130897, 16.94466709905296753, -232.9163774423793711 ) ) ;
#14634=CARTESIAN_POINT ( 'NONE',  ( 19.51310828881794990, -1.786742129898636344, -215.1201286626718741 ) ) ;
#14635=CARTESIAN_POINT ( 'NONE',  ( 15.05575868828727515, -2.428864548505686560, -227.9368649688638584 ) ) ;
#14636=CARTESIAN_POINT ( 'NONE',  ( -13.81390866287826746, 1.832988708064121175, -224.4361041349432639 ) ) ;
#14637=CARTESIAN_POINT ( 'NONE',  ( 13.82984244654956107, 22.51831320572884820, -232.1830460045772213 ) ) ;
#14638=CARTESIAN_POINT ( 'NONE',  ( 16.01130065545721592, 20.79417322911648114, -220.9619135886794652 ) ) ;
#14640=CARTESIAN_POINT ( 'NONE',  ( 11.05135090310477786, -21.04892152267781569, -234.3520113253972568 ) ) ;
#14641=CARTESIAN_POINT ( 'NONE',  ( 16.91879448796214191, 0.8271603773820436212, -230.0510230802265710 ) ) ;
#14643=CARTESIAN_POINT ( 'NONE',  ( 4.754245974719506940, 31.05377813473586102, -220.6166503949300193 ) ) ;
#14644=CARTESIAN_POINT ( 'NONE',  ( -17.15943377049709184, 17.77880916606822836, -233.2929083076029144 ) ) ;
#14645=CARTESIAN_POINT ( 'NONE',  ( 26.05530571436537457, -9.878918321867194763, -229.2327836737675284 ) ) ;
#14646=CARTESIAN_POINT ( 'NONE',  ( -3.082945806077231676, 30.69897765966285874, -224.2387254578930822 ) ) ;
#14648=CARTESIAN_POINT ( 'NONE',  ( 2.000982021813747291, 12.72833461843010205, -228.3416607300594308 ) ) ;
#14649=CARTESIAN_POINT ( 'NONE',  ( 16.53896178738450828, 2.691624496798088462, -232.5974196329879078 ) ) ;
#14650=CARTESIAN_POINT ( 'NONE',  ( -22.99617382825321599, 17.18101613848176967, -230.9512687019100099 ) ) ;
#14651=CARTESIAN_POINT ( 'NONE',  ( 24.57222455393806015, 12.08236629421828212, -229.7319216558644541 ) ) ;
#14653=ORIENTED_EDGE ( 'NONE', *, *, #18200, .F. ) ;
#14654=CARTESIAN_POINT ( 'NONE',  ( 0.9879969248128627202, 20.02408072508558945, -218.2055348255049410 ) ) ;
#14655=CARTESIAN_POINT ( 'NONE',  ( -18.44715843167851688, -19.86029123650958184, -231.9563062773970046 ) ) ;
#14656=CARTESIAN_POINT ( 'NONE',  ( 10.57926812561479757, 10.00910231482511215, -225.8341706491384286 ) ) ;
#14657=CARTESIAN_POINT ( 'NONE',  ( -4.239735564391798661, -14.20018808486349116, -230.2489621771221380 ) ) ;
#14659=CARTESIAN_POINT ( 'NONE',  ( -24.18895665211001500, 11.26087434487096139, -231.0040666710689550 ) ) ;
#14660=CARTESIAN_POINT ( 'NONE',  ( 8.158223302632384488, -13.44420475212243993, -229.3230086144918403 ) ) ;
#14662=CARTESIAN_POINT ( 'NONE',  ( 6.136979247480394584, 21.37054498543370684, -230.9985475420231467 ) ) ;
#14663=CARTESIAN_POINT ( 'NONE',  ( -26.11114532382342901, 12.73400870066318902, -227.7653936945517046 ) ) ;
#14664=CARTESIAN_POINT ( 'NONE',  ( -31.76239872120898511, 5.177298019713663990, -226.5714959923072342 ) ) ;
#14665=CARTESIAN_POINT ( 'NONE',  ( -14.98971194994906853, -6.742389346827670771, -223.0360336987919823 ) ) ;
#14666=CARTESIAN_POINT ( 'NONE',  ( 12.71499452845021416, 2.172589307656224378, -223.9381607050773084 ) ) ;
#14668=CARTESIAN_POINT ( 'NONE',  ( -12.42228566111607968, -8.873047627549107474, -232.6540845750675999 ) ) ;
#14669=CARTESIAN_POINT ( 'NONE',  ( 3.291078285693179950, 23.55624334554876498, -217.3208248278388623 ) ) ;
#14670=CARTESIAN_POINT ( 'NONE',  ( 17.57135037026572277, 0.09191994211922807634, -232.8447871904542410 ) ) ;
#14671=CARTESIAN_POINT ( 'NONE',  ( -9.222253059793434460, 13.27185325399938165, -229.0864811363590547 ) ) ;
#14672=CARTESIAN_POINT ( 'NONE',  ( 10.61539692146153691, 8.157890242340682718, -227.5705019877536301 ) ) ;
#14674=CARTESIAN_POINT ( 'NONE',  ( 3.849154133940814848, -15.34907234289524958, -223.0340372416051196 ) ) ;
#14676=CARTESIAN_POINT ( 'NONE',  ( -1.432270239486107766, -17.91381153981195951, -219.1344183636291802 ) ) ;
#14677=CARTESIAN_POINT ( 'NONE',  ( 13.49011766416699842, 7.659170998773840111, -228.1905628957712793 ) ) ;
#14678=CARTESIAN_POINT ( 'NONE',  ( 10.24538335401965661, -11.82980241027587276, -219.3753974371782363 ) ) ;
#14679=CARTESIAN_POINT ( 'NONE',  ( -22.05223281125446633, 0.4748437386657422543, -217.8785187290425256 ) ) ;
#14680=CARTESIAN_POINT ( 'NONE',  ( -8.803769170443210612, -17.82266517633203406, -233.6972128408098683 ) ) ;
#14681=CARTESIAN_POINT ( 'NONE',  ( 4.894897393135387631, 18.48819632322109996, -230.2131424875790628 ) ) ;
#14683=CARTESIAN_POINT ( 'NONE',  ( 15.58465056415575312, 2.812367138262562349, -229.5090343034091234 ) ) ;
#14684=CARTESIAN_POINT ( 'NONE',  ( 7.168644370073567806, 19.32044210858112265, -233.1278450877711634 ) ) ;
#14685=CARTESIAN_POINT ( 'NONE',  ( 8.686008240521225332, 26.11221116136006515, -227.6539570933143466 ) ) ;
#14686=CARTESIAN_POINT ( 'NONE',  ( 7.023652882903417272, -9.473209335044964874, -223.0206350579724983 ) ) ;
#14687=CARTESIAN_POINT ( 'NONE',  ( 19.40629804599390340, 15.10110417999774057, -216.3942729496570223 ) ) ;
#14688=CARTESIAN_POINT ( 'NONE',  ( -24.40185606299549192, 11.66496215664722236, -221.9473669705449765 ) ) ;
#14689=CARTESIAN_POINT ( 'NONE',  ( -18.63458318964815774, 8.046101765467303935, -217.8151248213926863 ) ) ;
#14690=CARTESIAN_POINT ( 'NONE',  ( -1.339836966046043631, -21.49735173129188581, -217.9043760890963313 ) ) ;
#14693=CARTESIAN_POINT ( 'NONE',  ( 13.49011766416699842, 7.659170998773840111, -228.1905628957712793 ) ) ;
#14694=CARTESIAN_POINT ( 'NONE',  ( 16.49868092868510061, -6.867418253114158766, -220.9302697977882133 ) ) ;
#14695=CARTESIAN_POINT ( 'NONE',  ( -16.27882490622757672, 1.520697279646460398, -219.2607721384596289 ) ) ;
#14697=CARTESIAN_POINT ( 'NONE',  ( -6.052919920376759855, -15.38051382379660836, -218.0337201863237624 ) ) ;
#14699=CARTESIAN_POINT ( 'NONE',  ( 4.301648988406530094, 13.23079486486395240, -223.2766268961034655 ) ) ;
#14700=CARTESIAN_POINT ( 'NONE',  ( -2.577721557973523314, 25.83760098923793791, -215.4660676095525389 ) ) ;
#14702=CARTESIAN_POINT ( 'NONE',  ( -20.18153419852512442, 14.25141268122526483, -233.5059133483111964 ) ) ;
#14703=CARTESIAN_POINT ( 'NONE',  ( -22.19673167533144564, -9.562764463827019057, -233.1557790568585062 ) ) ;
#14706=CARTESIAN_POINT ( 'NONE',  ( -9.749377714296398878, 10.28442384816749922, -229.3722863967025205 ) ) ;
#14707=CARTESIAN_POINT ( 'NONE',  ( -14.64285150619984677, -17.93374633926643824, -235.3168067477300838 ) ) ;
#14708=CARTESIAN_POINT ( 'NONE',  ( 23.36729170583618398, -5.500043712341283531, -232.1593072787115375 ) ) ;
#14709=CARTESIAN_POINT ( 'NONE',  ( -8.823862513872974489, 14.92351368520778898, -217.1499513473673346 ) ) ;
#14710=CARTESIAN_POINT ( 'NONE',  ( 17.92683513449900445, 4.153309877386362814, -218.0960491240478234 ) ) ;
#14712=CARTESIAN_POINT ( 'NONE',  ( -6.072587425033909803, 24.65158735603439055, -217.4249768037189767 ) ) ;
#14714=CARTESIAN_POINT ( 'NONE',  ( 25.53003411612920459, 7.940385729200389875, -230.5495695598654322 ) ) ;
#14715=CARTESIAN_POINT ( 'NONE',  ( -11.97657177269377371, -18.30092786828533846, -219.1278344157730942 ) ) ;
#14717=CARTESIAN_POINT ( 'NONE',  ( -12.43544732248594720, 12.69828336922617318, -219.3367909706387877 ) ) ;
#14718=CARTESIAN_POINT ( 'NONE',  ( 9.774133712851615030, 11.09751083462123766, -229.6876724410067823 ) ) ;
#14719=CARTESIAN_POINT ( 'NONE',  ( 2.892356176081334773, 24.03953794589038395, -215.3901262983647200 ) ) ;
#14720=CARTESIAN_POINT ( 'NONE',  ( -24.95561420934758701, -9.148537957313763513, -219.7769960911953149 ) ) ;
#14723=CARTESIAN_POINT ( 'NONE',  ( -12.78558550453068854, 7.693178343823584342, -230.0800953344970878 ) ) ;
#14724=CARTESIAN_POINT ( 'NONE',  ( -7.835169104947472540, -15.11139199849201908, -217.2594261031170220 ) ) ;
#14726=CARTESIAN_POINT ( 'NONE',  ( -3.368164009525018265, 19.03203264544105622, -233.5986411977714567 ) ) ;
#14728=CARTESIAN_POINT ( 'NONE',  ( -26.88784739727922357, 10.07520213145270915, -227.1866063047054922 ) ) ;
#14729=CARTESIAN_POINT ( 'NONE',  ( 8.454338299486085617, 13.28844197278511530, -217.6979371188311632 ) ) ;
#14731=CARTESIAN_POINT ( 'NONE',  ( 12.71450444683213021, 7.595266944807587350, -224.4213778964231665 ) ) ;
#14733=CARTESIAN_POINT ( 'NONE',  ( 14.87638776485545122, -7.040696290218329878, -226.6726542491997805 ) ) ;
#14734=CARTESIAN_POINT ( 'NONE',  ( -13.52935284690462758, -5.503084506376929141, -222.3607690796775671 ) ) ;
#14736=CARTESIAN_POINT ( 'NONE',  ( -2.129100187576105530, 26.11057959790866789, -231.5939360033278547 ) ) ;
#14737=CARTESIAN_POINT ( 'NONE',  ( 31.43562455973156844, -0.2326399569828876968, -228.1442589022926484 ) ) ;
#14738=CARTESIAN_POINT ( 'NONE',  ( 25.46470895113276711, -14.41152162994631070, -228.1811935238409035 ) ) ;
#14739=CARTESIAN_POINT ( 'NONE',  ( -14.57944476639264764, 6.129437248167259433, -229.4766146696829310 ) ) ;
#14740=CARTESIAN_POINT ( 'NONE',  ( 13.86383614057800884, 4.939477956453596441, -219.6543243356308324 ) ) ;
#14741=CARTESIAN_POINT ( 'NONE',  ( 10.89019654021101857, 23.08162452736882031, -220.1893104909416934 ) ) ;
#14743=CARTESIAN_POINT ( 'NONE',  ( 11.19883971596842720, -26.43874323075700161, -218.8478122585937626 ) ) ;
#14745=CARTESIAN_POINT ( 'NONE',  ( -0.6224962293416278492, 14.12372964796689701, -218.2103911528446645 ) ) ;
#14746=CARTESIAN_POINT ( 'NONE',  ( 0.1645309800062008665, 15.56029994314186382, -233.1129172884685943 ) ) ;
#14747=CARTESIAN_POINT ( 'NONE',  ( 26.62161015268053177, -11.01850213254573951, -223.2145259598937344 ) ) ;
#14748=CARTESIAN_POINT ( 'NONE',  ( -0.1571923090946999446, 19.34188126963334398, -216.6893131123363787 ) ) ;
#14750=CARTESIAN_POINT ( 'NONE',  ( 1.682843645364419993, 12.02583837823347679, -224.9288196625490457 ) ) ;
#14751=CARTESIAN_POINT ( 'NONE',  ( 26.75877786246624623, 11.80320999550499117, -231.5572967531201414 ) ) ;
#14752=CARTESIAN_POINT ( 'NONE',  ( -27.82842955277035202, 11.70195273568964112, -227.9294339757464911 ) ) ;
#14753=CARTESIAN_POINT ( 'NONE',  ( 17.34727976380017722, 4.822939981779328811, -230.8836217450937909 ) ) ;
#14754=CARTESIAN_POINT ( 'NONE',  ( 8.179023008129211902, 20.84698146175953681, -218.6376653143925921 ) ) ;
#14757=CARTESIAN_POINT ( 'NONE',  ( 5.446894657575932719, 15.00061806465251557, -226.4498309983864317 ) ) ;
#14758=CARTESIAN_POINT ( 'NONE',  ( -11.49803752765619258, -8.459563989871591971, -222.4296168992866853 ) ) ;
#14759=CARTESIAN_POINT ( 'NONE',  ( 14.32085100525799248, 9.220655089380342062, -219.9006227404039464 ) ) ;
#14760=CARTESIAN_POINT ( 'NONE',  ( -7.534279315020126155, -14.09704863723370494, -220.2840498463326355 ) ) ;
#14762=CARTESIAN_POINT ( 'NONE',  ( -11.94782396647286049, 8.456988817430419303, -225.5094493096559063 ) ) ;
#14764=CARTESIAN_POINT ( 'NONE',  ( 10.08089751255479527, -9.763210684072014089, -226.4220581413412390 ) ) ;
#14765=CARTESIAN_POINT ( 'NONE',  ( 12.11771628698343051, 17.56545729485151952, -218.0322663566023493 ) ) ;
#14766=CARTESIAN_POINT ( 'NONE',  ( -13.31590776630363315, 5.340120742929252096, -225.6956515496373186 ) ) ;
#14767=CARTESIAN_POINT ( 'NONE',  ( -10.59650102373989533, 7.849913810122476576, -230.0486530042683171 ) ) ;
#14768=CARTESIAN_POINT ( 'NONE',  ( -22.35893676869521229, -6.243268429983856116, -219.2540196962538062 ) ) ;
#14771=CARTESIAN_POINT ( 'NONE',  ( 11.50837930502119733, 10.86662242793286381, -233.1728506169798436 ) ) ;
#14773=CARTESIAN_POINT ( 'NONE',  ( -23.43110653090080930, -15.10372739875494297, -233.3642232949313211 ) ) ;
#14774=CARTESIAN_POINT ( 'NONE',  ( 7.450672702945051462, 17.42371045663376705, -217.2894981592719432 ) ) ;
#14775=CARTESIAN_POINT ( 'NONE',  ( 23.21336156720804667, 12.57464006230432574, -232.9346648124233070 ) ) ;
#14776=CARTESIAN_POINT ( 'NONE',  ( -11.79656379827575918, 10.43402410864828589, -226.0519616335988076 ) ) ;
#14778=CARTESIAN_POINT ( 'NONE',  ( 17.88619020626327938, 19.43517936004721847, -216.7078103882350604 ) ) ;
#14779=CARTESIAN_POINT ( 'NONE',  ( -1.602612909676673469, -20.69807258397210248, -232.3153362903766492 ) ) ;
#14780=CARTESIAN_POINT ( 'NONE',  ( -6.749503758482277682, -23.22604375411988187, -218.1095993038993299 ) ) ;
#14781=CARTESIAN_POINT ( 'NONE',  ( -11.10543627608095285, 3.497967533612860613, -224.1342318769322617 ) ) ;
#14782=CARTESIAN_POINT ( 'NONE',  ( 22.14341918773124362, -7.622004812940091689, -217.4502831791021720 ) ) ;
#14784=CARTESIAN_POINT ( 'NONE',  ( -23.14980455159086503, 0.3541108476526578785, -217.8785187302087536 ) ) ;
#14785=CARTESIAN_POINT ( 'NONE',  ( -15.17658589853145479, -26.64966442869902252, -226.8090782225333442 ) ) ;
#14786=CARTESIAN_POINT ( 'NONE',  ( 8.321021197036545303, 25.59447019508656140, -228.6184429848799482 ) ) ;
#14787=CARTESIAN_POINT ( 'NONE',  ( 16.26115440404298340, 3.800605480264513059, -219.2833057824682612 ) ) ;
#14788=CARTESIAN_POINT ( 'NONE',  ( 5.141746912158045468, 22.01688500372448232, -216.6678693612369386 ) ) ;
#14789=CARTESIAN_POINT ( 'NONE',  ( 3.241594727517011609, 27.64703009302456138, -225.5540025036233374 ) ) ;
#14790=CARTESIAN_POINT ( 'NONE',  ( 10.16297913136807907, -22.49776018550796408, -215.0507767410722977 ) ) ;
#14791=CARTESIAN_POINT ( 'NONE',  ( 11.98894270675143225, 20.38243841428667835, -233.2283128908360084 ) ) ;
#14792=CARTESIAN_POINT ( 'NONE',  ( -15.47996233766743934, 8.203483081506188768, -221.0931279926996353 ) ) ;
#14793=CARTESIAN_POINT ( 'NONE',  ( -19.35155980425159683, 1.157993580480985552, -230.3698774940947942 ) ) ;
#14794=CARTESIAN_POINT ( 'NONE',  ( -7.084830653876206696, -25.45310193036084456, -219.3007580301989492 ) ) ;
#14798=CARTESIAN_POINT ( 'NONE',  ( 14.31308345469695453, 12.76656023072872159, -231.9445021321040770 ) ) ;
#14799=CARTESIAN_POINT ( 'NONE',  ( 16.44812011099018889, -8.334251478664654655, -229.6488175962812761 ) ) ;
#14800=CARTESIAN_POINT ( 'NONE',  ( -29.16153046926437753, 6.356672163541281506, -226.4393515956758165 ) ) ;
#14801=CARTESIAN_POINT ( 'NONE',  ( -15.62091161899253855, -26.00636881980398840, -222.1463585103649905 ) ) ;
#14803=CARTESIAN_POINT ( 'NONE',  ( 4.656903975822286768, 13.45000048768594780, -227.6722060245555497 ) ) ;
#14805=CARTESIAN_POINT ( 'NONE',  ( -4.296082356836364191, 12.57880442405704002, -229.5247240216588125 ) ) ;
#14807=CARTESIAN_POINT ( 'NONE',  ( -3.368164009525018265, 19.03203264544105622, -233.5986411977714567 ) ) ;
#14808=CARTESIAN_POINT ( 'NONE',  ( -15.92941692657317354, -7.780888323563449838, -232.0381278758927976 ) ) ;
#14811=CARTESIAN_POINT ( 'NONE',  ( -17.75316132689678383, 25.03468689048078843, -222.1645193425721061 ) ) ;
#14812=CARTESIAN_POINT ( 'NONE',  ( -7.274850400134849515, -18.40080456867533698, -234.8703629377345692 ) ) ;
#14813=CARTESIAN_POINT ( 'NONE',  ( 23.44296991241933981, -12.51566675729016964, -231.4065378011870564 ) ) ;
#14814=CARTESIAN_POINT ( 'NONE',  ( -10.24288955603410933, 28.30762631303078791, -220.8855665231519083 ) ) ;
#14816=CARTESIAN_POINT ( 'NONE',  ( -19.59898341672158040, 3.279988180491820504, -234.9371679595475086 ) ) ;
#14817=CARTESIAN_POINT ( 'NONE',  ( -1.582540545905128049, 14.52388882916313584, -222.9138157219475147 ) ) ;
#14818=CARTESIAN_POINT ( 'NONE',  ( -18.71530386740073126, -0.6857509888707814527, -217.6195632122020527 ) ) ;
#14819=CARTESIAN_POINT ( 'NONE',  ( 15.33128967029630729, 6.504525012335983902, -229.0514072561169883 ) ) ;
#14820=CARTESIAN_POINT ( 'NONE',  ( -13.27091111731893847, -21.09541201825366841, -219.8810390191036106 ) ) ;
#14822=CARTESIAN_POINT ( 'NONE',  ( -19.74163224554151697, 8.726897413558679872, -232.6665747339030190 ) ) ;
#14823=CARTESIAN_POINT ( 'NONE',  ( 14.20064147608437821, 14.63411858269657806, -233.6150408276221242 ) ) ;
#14824=CARTESIAN_POINT ( 'NONE',  ( -0.7286890422672397394, 21.00519367000705273, -234.2149015821977969 ) ) ;
#14826=CARTESIAN_POINT ( 'NONE',  ( 24.68983475587330645, -0.6584631617853404784, -233.6195837498767958 ) ) ;
#14829=CARTESIAN_POINT ( 'NONE',  ( -21.02719846458807851, 18.12262440796364871, -218.0220709499931502 ) ) ;
#14830=CARTESIAN_POINT ( 'NONE',  ( -19.56933409648781108, -21.97186532644649759, -218.6835957583845982 ) ) ;
#14831=CARTESIAN_POINT ( 'NONE',  ( 20.89184612657454920, 5.404957034965973683, -232.0952743654565609 ) ) ;
#14832=CARTESIAN_POINT ( 'NONE',  ( 8.812073984913094904, 13.12649198322903210, -229.9172071780580495 ) ) ;
#14835=CARTESIAN_POINT ( 'NONE',  ( -11.59479561055411345, 9.544396733298208702, -229.1494558965577255 ) ) ;
#14837=CARTESIAN_POINT ( 'NONE',  ( 9.533850545951205291, 16.09136358716069637, -215.9093469876620475 ) ) ;
#14839=CARTESIAN_POINT ( 'NONE',  ( 14.31543143644129579, 0.1402917260236258845, -222.0030278161239039 ) ) ;
#14840=CARTESIAN_POINT ( 'NONE',  ( 14.31308345469695453, 12.76656023072872159, -231.9445021321040770 ) ) ;
#14842=CARTESIAN_POINT ( 'NONE',  ( 23.43833711860394686, -7.060024820847174531, -230.3984000052215606 ) ) ;
#14843=CARTESIAN_POINT ( 'NONE',  ( -11.39823187951283501, -7.998194509987097689, -226.8062974464413912 ) ) ;
#14846=CARTESIAN_POINT ( 'NONE',  ( -0.7292515499105728383, 28.18841485102515776, -220.8637599502617093 ) ) ;
#14847=CARTESIAN_POINT ( 'NONE',  ( 22.56961104628404868, -1.854966590244772950, -214.8717168148014025 ) ) ;
#14848=CARTESIAN_POINT ( 'NONE',  ( 14.90979066288448429, -1.927202206923867234, -222.7790985701595616 ) ) ;
#14849=CARTESIAN_POINT ( 'NONE',  ( -26.02492405343843984, 6.940268742526972900, -218.8798307745116460 ) ) ;
#14850=CARTESIAN_POINT ( 'NONE',  ( 18.40125535140034430, 0.01434342441762339639, -233.2485400239426099 ) ) ;
#14851=CARTESIAN_POINT ( 'NONE',  ( 16.07044873961816123, 22.39643131523411412, -226.8512752114033901 ) ) ;
#14852=CARTESIAN_POINT ( 'NONE',  ( -0.4481215836501183380, -14.49514564254841353, -225.8120917640279970 ) ) ;
#14855=CARTESIAN_POINT ( 'NONE',  ( -14.74212732455322161, 0.2624230007780231633, -231.8143822214177874 ) ) ;
#14857=CARTESIAN_POINT ( 'NONE',  ( 12.46318849118074112, 25.01309605388695445, -216.9820503660967859 ) ) ;
#14858=CARTESIAN_POINT ( 'NONE',  ( 4.966801760238292118, 27.41406605988239420, -216.4490579899774900 ) ) ;
#14859=CARTESIAN_POINT ( 'NONE',  ( 25.31834813234691595, -9.473547856983202564, -230.2364162768838298 ) ) ;
#14860=CARTESIAN_POINT ( 'NONE',  ( 0.6364901924797052857, 13.89978473517355617, -221.8840706290426397 ) ) ;
#14861=CARTESIAN_POINT ( 'NONE',  ( -20.43618815875133521, 1.403378831510147196, -232.9646741665398224 ) ) ;
#14863=CARTESIAN_POINT ( 'NONE',  ( -5.566280468132954518, 29.91920859341914962, -222.2705790733167817 ) ) ;
#14864=CARTESIAN_POINT ( 'NONE',  ( -15.51814470728089645, 2.949994979016113739, -222.8331727603033130 ) ) ;
#14865=CARTESIAN_POINT ( 'NONE',  ( -15.48255455842386219, 10.01793346089237069, -233.1197357361336913 ) ) ;
#14866=CARTESIAN_POINT ( 'NONE',  ( 14.63113973005795643, 4.926264598692385199, -222.4866305912601945 ) ) ;
#14868=CARTESIAN_POINT ( 'NONE',  ( 4.044213993247089967, 16.45246633354041421, -227.9255899743332918 ) ) ;
#14872=CARTESIAN_POINT ( 'NONE',  ( 8.132753622789847370, 14.44084924206385701, -222.7013822740049704 ) ) ;
#14873=CARTESIAN_POINT ( 'NONE',  ( -8.491902988188710921, -10.37035003683405066, -223.9502466269643435 ) ) ;
#14874=CARTESIAN_POINT ( 'NONE',  ( 14.95414693437772868, 8.262206471704862665, -230.1862972580043163 ) ) ;
#14875=CARTESIAN_POINT ( 'NONE',  ( -0.1378023845299804762, -12.51091464425689104, -226.1051157421467508 ) ) ;
#14877=CARTESIAN_POINT ( 'NONE',  ( -5.365396334125453137, 16.47374957271378904, -219.4721119688156534 ) ) ;
#14878=CARTESIAN_POINT ( 'NONE',  ( 21.50885124049339936, -13.38680967545814404, -232.7305552638522954 ) ) ;
#14879=CARTESIAN_POINT ( 'NONE',  ( 21.27834046766391651, 19.84195992785746654, -221.8454931627593965 ) ) ;
#14880=CARTESIAN_POINT ( 'NONE',  ( -9.810154340578240095, 25.84808829058669488, -220.5759521898573610 ) ) ;
#14881=CARTESIAN_POINT ( 'NONE',  ( -10.54177647804913320, 7.401649028325941515, -220.3980514230326264 ) ) ;
#14882=CARTESIAN_POINT ( 'NONE',  ( -13.04844958635619001, -9.307545681632840129, -223.5508123433884009 ) ) ;
#14883=CARTESIAN_POINT ( 'NONE',  ( 18.59615491886314231, -0.2392802120807639710, -217.5848846836084078 ) ) ;
#14887=CARTESIAN_POINT ( 'NONE',  ( -22.35094797335686678, -23.29487558099128108, -223.4832390375085538 ) ) ;
#14888=CARTESIAN_POINT ( 'NONE',  ( 11.98894270675143225, 20.38243841428667835, -233.2283128908360084 ) ) ;
#14890=CARTESIAN_POINT ( 'NONE',  ( 30.60340911705754863, 5.703403611927857497, -225.1938343315648297 ) ) ;
#14891=CARTESIAN_POINT ( 'NONE',  ( -1.406618399933933006, 16.47239985789244443, -232.2564017133012726 ) ) ;
#14892=CARTESIAN_POINT ( 'NONE',  ( 16.11883106748507188, 21.48229216499086291, -233.4985352728212433 ) ) ;
#14895=CARTESIAN_POINT ( 'NONE',  ( -5.577337716965932835, -27.36628652700976971, -219.4670492756933413 ) ) ;
#14897=CARTESIAN_POINT ( 'NONE',  ( -5.693514143275418604, -18.22526881224050754, -218.3451910747569968 ) ) ;
#14898=CARTESIAN_POINT ( 'NONE',  ( -28.76901170826145560, 13.32870333992657663, -228.6722616467874616 ) ) ;
#14899=CARTESIAN_POINT ( 'NONE',  ( 10.99893791904045415, -12.61823049403341201, -218.3266956685045841 ) ) ;
#14900=CARTESIAN_POINT ( 'NONE',  ( -28.55814054826834791, -1.660722980825670048, -228.2640858091212408 ) ) ;
#14901=CARTESIAN_POINT ( 'NONE',  ( -14.84823930505322132, -23.35465403802561823, -218.3226235040776260 ) ) ;
#14902=CARTESIAN_POINT ( 'NONE',  ( 11.75069299018312208, 6.043853022588032253, -224.2604610870103841 ) ) ;
#14904=CARTESIAN_POINT ( 'NONE',  ( -12.39654240422350462, 9.886262337642440556, -219.1620329226848014 ) ) ;
#14905=CARTESIAN_POINT ( 'NONE',  ( 26.39436175479395885, 14.32821500273865034, -221.6819523832376149 ) ) ;
#14907=CARTESIAN_POINT ( 'NONE',  ( -1.881996891245037995, 28.05344686410985489, -218.6379207300106202 ) ) ;
#14908=CARTESIAN_POINT ( 'NONE',  ( 19.70286159681817750, 17.87637900817293612, -218.6154571368943493 ) ) ;
#14909=CARTESIAN_POINT ( 'NONE',  ( 8.343550503364536297, -10.95302570107183726, -218.8523668966870446 ) ) ;
#14910=CARTESIAN_POINT ( 'NONE',  ( 21.52074627118099315, 8.791036694007010155, -215.9547738671300294 ) ) ;
#14911=CARTESIAN_POINT ( 'NONE',  ( -6.415689407129693045, 29.32186846096819011, -228.3852515614991887 ) ) ;
#14913=CARTESIAN_POINT ( 'NONE',  ( -8.983992482398329926, -13.08794618741998761, -229.3325301586503713 ) ) ;
#14914=CARTESIAN_POINT ( 'NONE',  ( -22.47200958260654957, 4.697452857301940732, -216.5879371680706242 ) ) ;
#14916=CARTESIAN_POINT ( 'NONE',  ( 23.49048926389013658, 9.645778135078892035, -218.7307869890797463 ) ) ;
#14917=CARTESIAN_POINT ( 'NONE',  ( 15.34439776706934921, -6.609831973102724412, -222.6284221295667862 ) ) ;
#14919=CARTESIAN_POINT ( 'NONE',  ( -1.633632075387274840, -15.48245080501611071, -218.5193615163172751 ) ) ;
#14920=CARTESIAN_POINT ( 'NONE',  ( -3.643097910890548796, 22.16888955197135047, -233.9701981029593298 ) ) ;
#14922=CARTESIAN_POINT ( 'NONE',  ( -3.309130212696198559, 28.80211350556483296, -217.4284252357080334 ) ) ;
#14923=ORIENTED_EDGE ( 'NONE', *, *, #315, .T. ) ;
#14924=CARTESIAN_POINT ( 'NONE',  ( -3.326157069579807946, 13.92020081821418565, -220.5733722327383930 ) ) ;
#14925=CARTESIAN_POINT ( 'NONE',  ( -27.06419889410506485, -1.187659473326917237, -217.6367138431444630 ) ) ;
#14926=MECHANICAL_DESIGN_GEOMETRIC_PRESENTATION_REPRESENTATION('',(#21375),#21726);
#14929=CARTESIAN_POINT ( 'NONE',  ( 5.331555957413248059, 27.50712867803999728, -219.0801070358024276 ) ) ;
#14930=CARTESIAN_POINT ( 'NONE',  ( -14.63769981573866552, -28.59145599960802642, -226.8825043222271631 ) ) ;
#14931=CARTESIAN_POINT ( 'NONE',  ( 5.953549895739506326, -12.70069413479034104, -221.3143591192976203 ) ) ;
#14932=CARTESIAN_POINT ( 'NONE',  ( 17.28140336138120858, -11.48510652344925020, -216.9852223368602893 ) ) ;
#14933=CARTESIAN_POINT ( 'NONE',  ( -12.27164519775873686, 10.97713184439464840, -231.6269036897678291 ) ) ;
#14934=CARTESIAN_POINT ( 'NONE',  ( 11.21155440434494643, 24.57152134148167733, -221.7155903571010356 ) ) ;
#14935=CARTESIAN_POINT ( 'NONE',  ( -24.68906941503829700, 2.445024713909649705, -232.6803430500543755 ) ) ;
#14936=CARTESIAN_POINT ( 'NONE',  ( -17.18633058961025029, 6.481319267413964802, -216.1357216783315494 ) ) ;
#14937=CARTESIAN_POINT ( 'NONE',  ( -24.66391263913385856, -10.62169550967977472, -229.5175364317193498 ) ) ;
#14938=ORIENTED_EDGE ( 'NONE', *, *, #10238, .F. ) ;
#14939=CARTESIAN_POINT ( 'NONE',  ( -15.36327147092456791, 5.453733681707060299, -220.0043800961136355 ) ) ;
#14940=CARTESIAN_POINT ( 'NONE',  ( 2.785859284650920031, 14.19821255961969619, -226.9946081512528906 ) ) ;
#14941=CARTESIAN_POINT ( 'NONE',  ( 2.068961274655788607, 15.13167107497539376, -217.8084559455312501 ) ) ;
#14943=CARTESIAN_POINT ( 'NONE',  ( -21.75565187119130428, -2.221346625543990427, -217.0768970814220609 ) ) ;
#14948=CARTESIAN_POINT ( 'NONE',  ( -10.65455960636934662, 10.37188583052882862, -219.5197110153079620 ) ) ;
#14949=CARTESIAN_POINT ( 'NONE',  ( -13.74974073587016576, -14.61773948691506142, -215.3128624239759290 ) ) ;
#14950=CARTESIAN_POINT ( 'NONE',  ( 16.00819137755116373, 4.595691552992191120, -229.5669508871464757 ) ) ;
#14951=CARTESIAN_POINT ( 'NONE',  ( 10.57926812561479757, 10.00910231482511215, -225.8341706491384286 ) ) ;
#14953=CARTESIAN_POINT ( 'NONE',  ( 29.17814965709308694, -1.309718763918959139, -225.2029557489520926 ) ) ;
#14954=CARTESIAN_POINT ( 'NONE',  ( -19.58639255110637478, 14.91076398872931819, -217.1105532241463720 ) ) ;
#14955=CARTESIAN_POINT ( 'NONE',  ( 13.89183999136464820, 6.553741795688899252, -220.8646181278399752 ) ) ;
#14957=CARTESIAN_POINT ( 'NONE',  ( 14.73698509926073186, 4.443590625350892331, -227.4062002049096236 ) ) ;
#14958=CARTESIAN_POINT ( 'NONE',  ( 16.49868092868510061, -6.867418253114158766, -220.9302697977882133 ) ) ;
#14960=CARTESIAN_POINT ( 'NONE',  ( -20.18470553695442860, -13.13924840112635195, -232.9662461559857718 ) ) ;
#14963=CARTESIAN_POINT ( 'NONE',  ( -5.298027976154672025, 13.43376398981453157, -220.6333279128949982 ) ) ;
#14964=CARTESIAN_POINT ( 'NONE',  ( 13.17262855481386374, -26.22572064374609013, -230.8671443076513583 ) ) ;
#14965=CARTESIAN_POINT ( 'NONE',  ( 14.56914850832129815, -2.041740472307377985, -224.7121590863160350 ) ) ;
#14966=CARTESIAN_POINT ( 'NONE',  ( -24.79507334250576278, 6.844873424762779379, -218.1074956078844878 ) ) ;
#14967=CARTESIAN_POINT ( 'NONE',  ( 25.38325563848796662, 11.05100313887457553, -217.8685524735130628 ) ) ;
#14968=CARTESIAN_POINT ( 'NONE',  ( 15.54095364727189299, 10.52000078266145700, -230.2714373371992735 ) ) ;
#14969=CARTESIAN_POINT ( 'NONE',  ( 13.44856294975069488, -28.16358066815265460, -226.3235907536142406 ) ) ;
#14971=CARTESIAN_POINT ( 'NONE',  ( -25.32262741784088078, 2.623212696197013472, -234.6011982779809841 ) ) ;
#14972=CARTESIAN_POINT ( 'NONE',  ( 10.46530733675539793, 8.351728317179080818, -222.7431177495969621 ) ) ;
#14973=CARTESIAN_POINT ( 'NONE',  ( 4.213939275857851108, 16.79797086795582928, -215.8378124706958943 ) ) ;
#14974=CARTESIAN_POINT ( 'NONE',  ( 29.78177645116457128, -4.041743286679309044, -225.6339783681140432 ) ) ;
#14975=CARTESIAN_POINT ( 'NONE',  ( -3.673551555920188783, 29.81207051619892923, -228.8770490300152005 ) ) ;
#14976=CARTESIAN_POINT ( 'NONE',  ( -26.58771759052039485, 5.114955214121561511, -218.2823714869195442 ) ) ;
#14978=CARTESIAN_POINT ( 'NONE',  ( 8.681721411120292942, 8.442847255497570202, -228.0516816418615065 ) ) ;
#14979=CARTESIAN_POINT ( 'NONE',  ( -27.32994399549947673, 3.379920396491164603, -227.9326384921875217 ) ) ;
#14980=CARTESIAN_POINT ( 'NONE',  ( -10.24288955603410933, 28.30762631303078791, -220.8855665231519083 ) ) ;
#14981=CARTESIAN_POINT ( 'NONE',  ( 14.95414693437772868, 8.262206471704862665, -230.1862972580043163 ) ) ;
#14982=CARTESIAN_POINT ( 'NONE',  ( 11.39755372583812587, 20.40856199875060639, -231.2895618162029621 ) ) ;
#14983=CARTESIAN_POINT ( 'NONE',  ( 17.95694455891925756, -3.510678534943489026, -231.2643001502910067 ) ) ;
#14985=CARTESIAN_POINT ( 'NONE',  ( -22.53818779203657741, -7.663114047788936567, -232.6164956747681458 ) ) ;
#14986=CARTESIAN_POINT ( 'NONE',  ( 21.35706335192880445, 15.67286272432725092, -219.2578158352350783 ) ) ;
#14987=CARTESIAN_POINT ( 'NONE',  ( -7.442430984977708164, -13.68264719635657301, -220.8544524341123747 ) ) ;
#14989=CARTESIAN_POINT ( 'NONE',  ( -8.407534899841293097, 16.91942258446019665, -231.3029992963236339 ) ) ;
#14992=CARTESIAN_POINT ( 'NONE',  ( 22.55746627616819566, -14.21542447219996852, -231.9819121152456205 ) ) ;
#14993=CARTESIAN_POINT ( 'NONE',  ( 24.49559427486850893, 14.86117239466233642, -230.3058416388274736 ) ) ;
#14994=CARTESIAN_POINT ( 'NONE',  ( -7.284474494690100776, 13.60812129561547046, -227.7414351104868331 ) ) ;
#14995=CARTESIAN_POINT ( 'NONE',  ( -12.19796877179171446, 17.24929682309303658, -234.5722138766719809 ) ) ;
#14997=CARTESIAN_POINT ( 'NONE',  ( -17.01759357405825668, -4.262369086395770168, -221.2289172648622184 ) ) ;
#14998=CARTESIAN_POINT ( 'NONE',  ( 25.09997929702755926, 1.294103573351435221, -217.0485712200477906 ) ) ;
#15000=CARTESIAN_POINT ( 'NONE',  ( -14.05955845762884238, -0.8719634938775207011, -221.0475910153949428 ) ) ;
#15001=CARTESIAN_POINT ( 'NONE',  ( 15.26539804565921621, 9.309431686815628382, -232.9129599938668207 ) ) ;
#15002=CARTESIAN_POINT ( 'NONE',  ( -25.20870746202117729, 11.68425842440532136, -223.9066764530103342 ) ) ;
#15003=CARTESIAN_POINT ( 'NONE',  ( 11.31331191788792623, 29.23420701778062281, -220.7538464529627333 ) ) ;
#15004=CARTESIAN_POINT ( 'NONE',  ( 11.00045714400293306, 20.20239058357963913, -215.1666500215986275 ) ) ;
#15006=CARTESIAN_POINT ( 'NONE',  ( -6.241914139598351952, -12.26321662989467320, -220.9276712261616353 ) ) ;
#15008=CARTESIAN_POINT ( 'NONE',  ( 6.679827377097204533, -23.59744646493245668, -231.8618301756397670 ) ) ;
#15009=CARTESIAN_POINT ( 'NONE',  ( -26.12939716039095117, 11.33146045174629357, -233.1192402782019997 ) ) ;
#15010=CARTESIAN_POINT ( 'NONE',  ( 17.01060404384151781, -6.151862203644831162, -218.3248062500343849 ) ) ;
#15011=CARTESIAN_POINT ( 'NONE',  ( 27.20328812258980378, -0.4806365347271125965, -218.3128023695579998 ) ) ;
#15012=CARTESIAN_POINT ( 'NONE',  ( -28.46519324992292965, -8.397260794665152517, -225.6705986409035347 ) ) ;
#15013=CARTESIAN_POINT ( 'NONE',  ( 20.54489901492447501, 10.52141067440427591, -216.2005526543161693 ) ) ;
#15015=CARTESIAN_POINT ( 'NONE',  ( -20.04070223234628756, 18.12164545743767263, -231.9292141396248610 ) ) ;
#15016=CARTESIAN_POINT ( 'NONE',  ( 12.55473222622303986, 11.30320364856893001, -218.8964119182764989 ) ) ;
#15017=CARTESIAN_POINT ( 'NONE',  ( 0.9908753270255351575, 13.79205759140780430, -228.0165926715089881 ) ) ;
#15018=CARTESIAN_POINT ( 'NONE',  ( 9.425340689562565544, 25.38932416188112384, -221.3391712389563963 ) ) ;
#15019=CARTESIAN_POINT ( 'NONE',  ( 10.25809576580632232, -7.052396458808492419, -221.5466685117269208 ) ) ;
#15020=CARTESIAN_POINT ( 'NONE',  ( -21.75607741976026333, 20.26169853110213381, -228.4128163609909450 ) ) ;
#15021=CARTESIAN_POINT ( 'NONE',  ( -0.9851030586975465519, 19.34066537597387381, -233.8273485600932418 ) ) ;
#15022=CARTESIAN_POINT ( 'NONE',  ( -13.55429797312971374, -24.97278848321653300, -221.1627755146857908 ) ) ;
#15023=CARTESIAN_POINT ( 'NONE',  ( -21.89065952084848021, -0.9940043559354364566, -216.9999999999999716 ) ) ;
#15026=CARTESIAN_POINT ( 'NONE',  ( 15.76910524310159900, 5.601482066865847820, -220.3440822020379528 ) ) ;
#15027=CARTESIAN_POINT ( 'NONE',  ( 7.829076659910394476, -15.59360078984655651, -230.7142312655459762 ) ) ;
#15028=CARTESIAN_POINT ( 'NONE',  ( -20.47640197314466093, 18.50423766437512541, -220.4440130802851456 ) ) ;
#15029=CARTESIAN_POINT ( 'NONE',  ( -0.9249541874382023465, 14.55235618511626328, -223.7321818898853962 ) ) ;
#15030=CARTESIAN_POINT ( 'NONE',  ( -25.61235545225478560, -15.41032726095661509, -226.9890212492312855 ) ) ;
#15031=CARTESIAN_POINT ( 'NONE',  ( 29.89309326230132058, 6.052383583152112223, -228.3539431708548477 ) ) ;
#15032=CARTESIAN_POINT ( 'NONE',  ( 14.65697969206133067, 11.40587726087447606, -233.3943609825344652 ) ) ;
#15034=CARTESIAN_POINT ( 'NONE',  ( -2.817219543927646175, 14.13981714106644993, -229.6779615865167443 ) ) ;
#15035=CARTESIAN_POINT ( 'NONE',  ( 15.06969459085678942, -9.685035337269850331, -230.1890524597188801 ) ) ;
#15038=CARTESIAN_POINT ( 'NONE',  ( 2.837900457371055563, 25.11342719071438978, -232.9871906064174709 ) ) ;
#15039=CARTESIAN_POINT ( 'NONE',  ( -3.456580335739853016, -11.82839499582713749, -226.8096787805597501 ) ) ;
#15040=CARTESIAN_POINT ( 'NONE',  ( 13.99926435381047618, -21.11851526759364006, -232.9234173943665951 ) ) ;
#15041=CARTESIAN_POINT ( 'NONE',  ( 20.80196158924851701, -7.261721507697286526, -217.3074963141844194 ) ) ;
#15042=CARTESIAN_POINT ( 'NONE',  ( -12.39654240422350462, 9.886262337642440556, -219.1620329226848014 ) ) ;
#15043=CARTESIAN_POINT ( 'NONE',  ( 11.73428189025226942, 12.46434742632455084, -228.1539301014595083 ) ) ;
#15044=CARTESIAN_POINT ( 'NONE',  ( -13.92046207272054303, -0.1600067567908077248, -224.5811699126800818 ) ) ;
#15045=CARTESIAN_POINT ( 'NONE',  ( -21.72273972318264867, 21.08396222359856864, -224.0477214759881690 ) ) ;
#15046=CARTESIAN_POINT ( 'NONE',  ( -14.19990609618026056, -7.901335420714983293, -227.4892254059333823 ) ) ;
#15047=ORIENTED_EDGE ( 'NONE', *, *, #11743, .F. ) ;
#15048=CARTESIAN_POINT ( 'NONE',  ( -11.03778527004271659, 26.96286968643956428, -225.4057095641571209 ) ) ;
#15049=CARTESIAN_POINT ( 'NONE',  ( 13.48097272627202159, 8.509510470709432894, -231.5257201610278059 ) ) ;
#15050=CARTESIAN_POINT ( 'NONE',  ( -4.974038791218384326, 28.61915055369004079, -219.5057940952933961 ) ) ;
#15052=CARTESIAN_POINT ( 'NONE',  ( 20.07985072697885442, -15.33367264652052953, -217.4666949641080294 ) ) ;
#15055=CARTESIAN_POINT ( 'NONE',  ( -16.65698539163286540, 11.03290537638306112, -233.6474915129378758 ) ) ;
#15056=CARTESIAN_POINT ( 'NONE',  ( -10.39490437715664228, -5.549361993742060406, -223.4983083630424403 ) ) ;
#15058=CARTESIAN_POINT ( 'NONE',  ( 7.995304978256253747, 13.28024228361502779, -220.6535174700288451 ) ) ;
#15060=CARTESIAN_POINT ( 'NONE',  ( 28.52058947142581502, -1.755848367977142610, -221.9695116608532715 ) ) ;
#15062=CARTESIAN_POINT ( 'NONE',  ( -16.20072894238734307, 0.5024448614660336210, -230.4554067149722130 ) ) ;
#15063=CARTESIAN_POINT ( 'NONE',  ( -19.61183938075907918, 22.25855138946451106, -229.5731876748794207 ) ) ;
#15064=CARTESIAN_POINT ( 'NONE',  ( 24.32561047128371001, 1.769413244618101011, -218.8629106451077462 ) ) ;
#15065=FILL_AREA_STYLE ('',( #4466 ) ) ;
#15070=CARTESIAN_POINT ( 'NONE',  ( -20.43618815875133521, 1.403378831510147196, -232.9646741665398224 ) ) ;
#15071=CARTESIAN_POINT ( 'NONE',  ( 16.16137015560671131, -6.751010448487875237, -221.3181884246570519 ) ) ;
#15072=CARTESIAN_POINT ( 'NONE',  ( -18.89430729770302975, -12.42271633246521212, -233.2230176520695295 ) ) ;
#15076=CARTESIAN_POINT ( 'NONE',  ( 2.208705534715813101, 15.26926593729510984, -227.3643075380122980 ) ) ;
#15078=CARTESIAN_POINT ( 'NONE',  ( 11.27265965248755819, -10.15440342946296148, -217.7707216267749573 ) ) ;
#15079=CARTESIAN_POINT ( 'NONE',  ( 13.04434844185555420, -10.19049307777131297, -230.8679447648462713 ) ) ;
#15080=CARTESIAN_POINT ( 'NONE',  ( -20.57288920227272655, 16.51351902378409520, -230.8484733908063333 ) ) ;
#15081=CARTESIAN_POINT ( 'NONE',  ( 20.10109416526603709, 2.018147939476731434, -216.1034161917718848 ) ) ;
#15082=CARTESIAN_POINT ( 'NONE',  ( 17.32394486779715592, 4.028159306070694612, -218.4253989884176690 ) ) ;
#15084=CARTESIAN_POINT ( 'NONE',  ( -7.461655027780660809, -14.63259296063595727, -227.5661480528262075 ) ) ;
#15086=CARTESIAN_POINT ( 'NONE',  ( -27.68973657932738064, 5.930811633061950694, -216.7842770206311513 ) ) ;
#15087=CARTESIAN_POINT ( 'NONE',  ( 17.10545320562996352, 22.53742678899184781, -232.4605876935045785 ) ) ;
#15088=CARTESIAN_POINT ( 'NONE',  ( -1.584125552723561592, 20.48724127025963782, -214.7515060525244621 ) ) ;
#15089=CARTESIAN_POINT ( 'NONE',  ( 16.69326964758149856, -4.763004462669847783, -219.2590076381798951 ) ) ;
#15090=CARTESIAN_POINT ( 'NONE',  ( -10.84997096467605182, 25.01800101807719301, -232.4518260228253155 ) ) ;
#15091=CARTESIAN_POINT ( 'NONE',  ( -16.63766460830045091, 5.158675778507696208, -232.1659425527909093 ) ) ;
#15092=CARTESIAN_POINT ( 'NONE',  ( 10.85325209735074559, 11.82487774067193342, -216.5214842375702062 ) ) ;
#15093=CARTESIAN_POINT ( 'NONE',  ( -16.40443871513620522, 4.023423476741658789, -228.9829044427089002 ) ) ;
#15094=CARTESIAN_POINT ( 'NONE',  ( -8.966714183099560032, 19.05224306381768073, -234.0879867025980445 ) ) ;
#15095=CARTESIAN_POINT ( 'NONE',  ( 17.07668571305246985, 2.037405138410691485, -219.7626854147787867 ) ) ;
#15096=CARTESIAN_POINT ( 'NONE',  ( 15.56183105618911355, 23.93598532278018354, -223.2746693648072664 ) ) ;
#15100=CARTESIAN_POINT ( 'NONE',  ( -16.99821283087967672, -0.5135051709387361552, -216.2173766440975555 ) ) ;
#15101=CARTESIAN_POINT ( 'NONE',  ( -14.93311267495276518, -24.05029333330348251, -229.1587772033057888 ) ) ;
#15103=CARTESIAN_POINT ( 'NONE',  ( -7.240690404266621805, 13.01623002570985044, -225.3000933658701967 ) ) ;
#15104=CARTESIAN_POINT ( 'NONE',  ( 7.045253012492558753, -17.38872841331140862, -218.3726031779064556 ) ) ;
#15105=CARTESIAN_POINT ( 'NONE',  ( 10.98110116949302828, 13.70618071521442971, -230.2797640191687378 ) ) ;
#15106=CARTESIAN_POINT ( 'NONE',  ( -9.661739055621840322, 20.41227307912577871, -232.0920144483423257 ) ) ;
#15107=CARTESIAN_POINT ( 'NONE',  ( -7.399925907206128528, 10.29859031525428037, -227.1614041762800298 ) ) ;
#15109=CARTESIAN_POINT ( 'NONE',  ( -24.24026017931571175, -14.11860166261188354, -224.3835235244768569 ) ) ;
#15110=CARTESIAN_POINT ( 'NONE',  ( 7.639528166734322667, 11.92751229241157596, -224.6077814063189635 ) ) ;
#15111=CARTESIAN_POINT ( 'NONE',  ( 22.69522586737246783, 3.669837464059151344, -234.0947686933411944 ) ) ;
#15113=CARTESIAN_POINT ( 'NONE',  ( -22.24434812881145618, 2.221346625544017961, -216.9231029185778254 ) ) ;
#15114=CARTESIAN_POINT ( 'NONE',  ( 11.43247012502872728, 12.44034019618676190, -231.9336559008378629 ) ) ;
#15115=CARTESIAN_POINT ( 'NONE',  ( -16.56270003954679382, 4.935922114544952777, -221.6503923146493378 ) ) ;
#15116=CARTESIAN_POINT ( 'NONE',  ( 3.711349367426693746, 16.84755988915346236, -233.7359972593521888 ) ) ;
#15117=CARTESIAN_POINT ( 'NONE',  ( 15.46952826979347151, 3.173892190046953665, -221.7237849701489552 ) ) ;
#15118=CARTESIAN_POINT ( 'NONE',  ( -17.92393051735373888, -14.45097846726422830, -234.9711082062119374 ) ) ;
#15120=CARTESIAN_POINT ( 'NONE',  ( -15.28220591200235390, -15.65475725988279443, -217.1155325995422913 ) ) ;
#15121=CARTESIAN_POINT ( 'NONE',  ( -13.63292518690856170, 3.968236334994402981, -218.3158317831635316 ) ) ;
#15122=CARTESIAN_POINT ( 'NONE',  ( 7.486336813247038258, -29.35413437595724773, -221.4114973598149447 ) ) ;
#15123=CARTESIAN_POINT ( 'NONE',  ( 17.05764047735875266, -11.29112887239367424, -214.9748062598841898 ) ) ;
#15124=CARTESIAN_POINT ( 'NONE',  ( -26.07210576407111446, -8.413030596423759278, -230.6002792590230115 ) ) ;
#15125=CARTESIAN_POINT ( 'NONE',  ( 16.97369223523349646, 15.19068754808448851, -217.0779026324121332 ) ) ;
#15127=CARTESIAN_POINT ( 'NONE',  ( -13.30451247859013897, 19.85560227862636040, -232.3493821534129609 ) ) ;
#15128=CARTESIAN_POINT ( 'NONE',  ( 20.85755584069816493, 20.53615333921957742, -227.2010381488614996 ) ) ;
#15129=CARTESIAN_POINT ( 'NONE',  ( 20.41153371889344825, 17.18812948447019551, -230.7531656956970778 ) ) ;
#15130=CARTESIAN_POINT ( 'NONE',  ( 10.59524789654300925, 9.532374763983630928, -223.0758647391057821 ) ) ;
#15131=CARTESIAN_POINT ( 'NONE',  ( 18.64433268355766415, -12.21264687082605782, -214.8850304513305502 ) ) ;
#15132=CARTESIAN_POINT ( 'NONE',  ( -4.974038791218384326, 28.61915055369004079, -219.5057940952933961 ) ) ;
#15135=CARTESIAN_POINT ( 'NONE',  ( 12.23063869552301242, 12.84118223717021934, -218.8273164334868284 ) ) ;
#15136=CARTESIAN_POINT ( 'NONE',  ( 15.76600796393256410, -24.40864267010898558, -225.5036181134576907 ) ) ;
#15137=CARTESIAN_POINT ( 'NONE',  ( -22.24722865165759345, 18.77558306771206986, -226.5077042908023941 ) ) ;
#15138=CARTESIAN_POINT ( 'NONE',  ( -3.223980134944351317, 26.83284996841001302, -219.5167893230652965 ) ) ;
#15139=CARTESIAN_POINT ( 'NONE',  ( -21.63546480557098306, -21.44004028177477750, -223.8762611443524122 ) ) ;
#15141=CARTESIAN_POINT ( 'NONE',  ( 30.60340911705754863, 5.703403611927857497, -225.1938343315648297 ) ) ;
#15142=CARTESIAN_POINT ( 'NONE',  ( 21.92281339924938877, 16.67475415235398017, -231.9828670874568957 ) ) ;
#15144=CARTESIAN_POINT ( 'NONE',  ( 5.343558017910363667, 26.29639771561252459, -218.1010331760174665 ) ) ;
#15145=CARTESIAN_POINT ( 'NONE',  ( 16.71284463105542883, -8.832875790685479345, -219.1937169315102949 ) ) ;
#15146=CARTESIAN_POINT ( 'NONE',  ( 12.99512476935412231, -3.120572961704727977, -223.7636045402963987 ) ) ;
#15148=CARTESIAN_POINT ( 'NONE',  ( 5.069241901512100412, 14.34986542013820632, -229.6420000777802954 ) ) ;
#15149=CARTESIAN_POINT ( 'NONE',  ( -27.52442056016948868, -15.72718643249855397, -222.0944556419597689 ) ) ;
#15150=CARTESIAN_POINT ( 'NONE',  ( 11.32394539683753720, -15.63383003174572572, -233.0723040138117881 ) ) ;
#15151=CARTESIAN_POINT ( 'NONE',  ( 15.10937218716165020, -26.44221868192832758, -222.7999243300199907 ) ) ;
#15152=CARTESIAN_POINT ( 'NONE',  ( -9.734169867326336600, 14.53420431798807755, -231.2442251076483046 ) ) ;
#15153=CARTESIAN_POINT ( 'NONE',  ( 13.96918721733258195, 14.12724320058294403, -230.4946432816737172 ) ) ;
#15154=CARTESIAN_POINT ( 'NONE',  ( -15.15110768032078070, 3.517015312212880218, -219.5479300368539270 ) ) ;
#15155=CARTESIAN_POINT ( 'NONE',  ( -29.98527381603928887, 6.316825171121390525, -230.1108345570740994 ) ) ;
#15156=CARTESIAN_POINT ( 'NONE',  ( -16.02921639098982709, -5.689335215210093999, -220.0011032104688979 ) ) ;
#15158=CARTESIAN_POINT ( 'NONE',  ( -8.030397104878142400, 15.90963402996711373, -230.6518438502475590 ) ) ;
#15159=CARTESIAN_POINT ( 'NONE',  ( 19.40629804599390340, 15.10110417999774057, -216.3942729496570223 ) ) ;
#15160=CARTESIAN_POINT ( 'NONE',  ( -0.9851030586975465519, 19.34066537597387381, -233.8273485600932418 ) ) ;
#15161=CARTESIAN_POINT ( 'NONE',  ( 24.96165930385824794, -17.14663603160204275, -224.2745859498249672 ) ) ;
#15164=CARTESIAN_POINT ( 'NONE',  ( -9.749377714296398878, 10.28442384816749922, -229.3722863967025205 ) ) ;
#15165=CARTESIAN_POINT ( 'NONE',  ( -12.37311134093142506, -6.729359123088276995, -218.5215259163429380 ) ) ;
#15167=CARTESIAN_POINT ( 'NONE',  ( 11.87982377808925527, 10.85265283465803421, -229.5027252913499183 ) ) ;
#15169=CARTESIAN_POINT ( 'NONE',  ( 13.91151814069282722, -15.58123622716646572, -216.5183035683795367 ) ) ;
#15170=CARTESIAN_POINT ( 'NONE',  ( -13.92046207272054303, -0.1600067567908077248, -224.5811699126800818 ) ) ;
#15172=CARTESIAN_POINT ( 'NONE',  ( -13.48133478602219171, 10.24771958306113362, -218.3822527490931691 ) ) ;
#15173=CARTESIAN_POINT ( 'NONE',  ( 27.58248235015124550, 10.80791576765187934, -226.6933256641281389 ) ) ;
#15174=CARTESIAN_POINT ( 'NONE',  ( -5.688232406366994454, -14.80527619068227629, -228.6723097085491645 ) ) ;
#15176=CARTESIAN_POINT ( 'NONE',  ( 13.54927135793711557, 0.6749664302445949060, -222.0769159577524192 ) ) ;
#15179=CARTESIAN_POINT ( 'NONE',  ( 15.67226265972355392, -3.922905252720024105, -226.2579514984929858 ) ) ;
#15180=CARTESIAN_POINT ( 'NONE',  ( 14.44181943480797159, -1.924641616899158914, -227.3019274429727830 ) ) ;
#15185=CARTESIAN_POINT ( 'NONE',  ( 5.064106757301036765, 16.06517852189101703, -221.6413221086847329 ) ) ;
#15186=CARTESIAN_POINT ( 'NONE',  ( 17.65733440236621732, -13.95165017647719452, -214.8231966952668301 ) ) ;
#15187=CARTESIAN_POINT ( 'NONE',  ( 12.31511859722645852, -8.491226738247512174, -220.9006323875693738 ) ) ;
#15189=CARTESIAN_POINT ( 'NONE',  ( -9.627017372966443887, 15.60690227900018279, -218.8878023709062859 ) ) ;
#15190=CARTESIAN_POINT ( 'NONE',  ( 24.19635128940818447, 10.31396593861802380, -216.9479509989864425 ) ) ;
#15191=CARTESIAN_POINT ( 'NONE',  ( 21.68053922431529301, 13.05890675940072931, -230.5667798303363440 ) ) ;
#15193=CARTESIAN_POINT ( 'NONE',  ( -2.652888268066178945, -28.18865072326549637, -221.4226523288203623 ) ) ;
#15195=CARTESIAN_POINT ( 'NONE',  ( -9.924247690135956645, 7.079756654796299564, -222.1205998075789694 ) ) ;
#15196=CARTESIAN_POINT ( 'NONE',  ( 12.56362091610784049, 9.747446748398973071, -231.6428467497164547 ) ) ;
#15197=CARTESIAN_POINT ( 'NONE',  ( 9.379155480182538085, -13.23755613463586300, -225.9392943819708250 ) ) ;
#15199=CARTESIAN_POINT ( 'NONE',  ( 5.141746912158045468, 22.01688500372448232, -216.6678693612369386 ) ) ;
#15200=CARTESIAN_POINT ( 'NONE',  ( -22.47200958260654957, 4.697452857301940732, -216.5879371680706242 ) ) ;
#15201=AXIS2_PLACEMENT_3D ( 'NONE', #17221, #15765, #9006 ) ;
#15202=CARTESIAN_POINT ( 'NONE',  ( 24.61409543538958289, 19.88121288930873476, -228.5015986536257344 ) ) ;
#15203=CARTESIAN_POINT ( 'NONE',  ( -14.08236938285573636, 6.062428076406559008, -221.7923619418395447 ) ) ;
#15205=CARTESIAN_POINT ( 'NONE',  ( -7.395406416482832590, 12.93623984139929739, -219.2606224730616873 ) ) ;
#15206=CARTESIAN_POINT ( 'NONE',  ( 20.34032485158648029, 2.741617426884598530, -217.9827731991294968 ) ) ;
#15207=CARTESIAN_POINT ( 'NONE',  ( 1.455106383990497187, 21.12056149333958999, -230.8076663600630241 ) ) ;
#15210=CARTESIAN_POINT ( 'NONE',  ( -20.85586116824185510, -1.996934699305910499, -232.3804859832740135 ) ) ;
#15211=CARTESIAN_POINT ( 'NONE',  ( -12.13692969104051400, -0.3108940857385004697, -222.6170402347994184 ) ) ;
#15212=CARTESIAN_POINT ( 'NONE',  ( -11.03528491614390994, -18.43141318057359612, -232.7233776306152038 ) ) ;
#15216=CARTESIAN_POINT ( 'NONE',  ( -13.51991436508781597, 16.61129329384914755, -232.1184346153593197 ) ) ;
#15217=CARTESIAN_POINT ( 'NONE',  ( 4.788325992165110456, -24.70830725884669121, -218.5516572218182603 ) ) ;
#15218=CARTESIAN_POINT ( 'NONE',  ( 24.20411255886326529, 12.66254860825103634, -218.0144359054998802 ) ) ;
#15219=CARTESIAN_POINT ( 'NONE',  ( -4.866400999161825780, 25.69921167300892861, -231.0100031340613782 ) ) ;
#15220=CARTESIAN_POINT ( 'NONE',  ( -10.49339404011726984, 12.66576824096800991, -217.2681947942554643 ) ) ;
#15222=CARTESIAN_POINT ( 'NONE',  ( 28.41126862162173694, -7.739794849403359933, -232.1728475156252500 ) ) ;
#15224=CARTESIAN_POINT ( 'NONE',  ( 12.10245006109274080, 26.02147364279441888, -220.6079829738538649 ) ) ;
#15225=CARTESIAN_POINT ( 'NONE',  ( -17.59913672443795463, -0.5356773789333074687, -220.7342471185320960 ) ) ;
#15226=CARTESIAN_POINT ( 'NONE',  ( -16.66929017373293931, 3.065794289431343689, -220.7800282905443794 ) ) ;
#15228=CARTESIAN_POINT ( 'NONE',  ( -28.63642022368215478, -8.327690832987633129, -230.6787490302224057 ) ) ;
#15229=CARTESIAN_POINT ( 'NONE',  ( 15.88043104796248528, 11.88135572392608807, -216.2525917828042168 ) ) ;
#15230=CARTESIAN_POINT ( 'NONE',  ( -16.51501534778698854, 10.61825396983174485, -230.5082364903317966 ) ) ;
#15232=CARTESIAN_POINT ( 'NONE',  ( -6.260151855817680300, 29.88549235135308635, -226.8929519981915064 ) ) ;
#15233=CARTESIAN_POINT ( 'NONE',  ( 15.07212457412616224, 2.472408313530222390, -227.3472192494155024 ) ) ;
#15234=CARTESIAN_POINT ( 'NONE',  ( -8.876630286717240637, -14.53920553942005256, -232.5681369007955368 ) ) ;
#15236=CARTESIAN_POINT ( 'NONE',  ( -10.46545893407769157, -9.768586176915025732, -226.8636372813723199 ) ) ;
#15237=CARTESIAN_POINT ( 'NONE',  ( -23.68377094563794572, 13.02263794644603578, -215.9752901280847652 ) ) ;
#15238=CARTESIAN_POINT ( 'NONE',  ( 2.378655016347637652, -14.31292064579845302, -219.9942319014987220 ) ) ;
#15239=CARTESIAN_POINT ( 'NONE',  ( -0.3969026096611234511, 20.89748314411456676, -216.3289738411752978 ) ) ;
#15240=CARTESIAN_POINT ( 'NONE',  ( 12.92161125358352791, -8.797851723037126703, -217.2061419145261425 ) ) ;
#15241=CARTESIAN_POINT ( 'NONE',  ( -14.93108815068229589, -1.792787290847115633, -227.6165763581034582 ) ) ;
#15242=CARTESIAN_POINT ( 'NONE',  ( 10.98110116949302828, 13.70618071521442971, -230.2797640191687378 ) ) ;
#15244=CARTESIAN_POINT ( 'NONE',  ( -13.40354389326479456, 23.35336998323175450, -219.8517474526506987 ) ) ;
#15245=CARTESIAN_POINT ( 'NONE',  ( 21.46274988498219471, 20.25395488059580984, -223.1777011585387243 ) ) ;
#15246=CARTESIAN_POINT ( 'NONE',  ( 15.85665641241444668, 18.24713744004561988, -217.7195292979064902 ) ) ;
#15247=CARTESIAN_POINT ( 'NONE',  ( 18.75523091462765990, 19.46592657336209697, -230.4909883316157391 ) ) ;
#15248=CARTESIAN_POINT ( 'NONE',  ( -2.170317331930874172, -31.11073952835316803, -223.3804330553629995 ) ) ;
#15249=CARTESIAN_POINT ( 'NONE',  ( -10.45265333418718612, 16.71118685480038479, -231.7490466715443631 ) ) ;
#15251=CARTESIAN_POINT ( 'NONE',  ( -21.89482327431018760, 1.733733432562314158, -233.1353281693111796 ) ) ;
#15253=CARTESIAN_POINT ( 'NONE',  ( 15.05360126642391450, 1.481754003466396963, -222.9454997252120734 ) ) ;
#15254=CARTESIAN_POINT ( 'NONE',  ( 15.36293661829273027, -24.44941682316833464, -223.0188286856611626 ) ) ;
#15255=CARTESIAN_POINT ( 'NONE',  ( -13.31590776630363315, 5.340120742929252096, -225.6956515496373186 ) ) ;
#15256=CARTESIAN_POINT ( 'NONE',  ( 2.951582164238582440, 19.39026647431845873, -217.4356918981242472 ) ) ;
#15257=CARTESIAN_POINT ( 'NONE',  ( -26.07210576407111446, -8.413030596423759278, -230.6002792590230115 ) ) ;
#15259=CARTESIAN_POINT ( 'NONE',  ( 14.00715608756928532, 4.299235856235253728, -230.2440235370780215 ) ) ;
#15260=CARTESIAN_POINT ( 'NONE',  ( 10.35958063030883025, 8.003303894222913328, -225.9303204057916048 ) ) ;
#15261=CARTESIAN_POINT ( 'NONE',  ( -3.060450601941519189, 13.29454208326677289, -222.0135664617158682 ) ) ;
#15262=CARTESIAN_POINT ( 'NONE',  ( 26.05530571436537457, -9.878918321867194763, -229.2327836737675284 ) ) ;
#15263=CARTESIAN_POINT ( 'NONE',  ( 16.07480884343054939, -7.767425703123992164, -217.5935768756353923 ) ) ;
#15265=CARTESIAN_POINT ( 'NONE',  ( -2.817219543927646175, 14.13981714106644993, -229.6779615865167443 ) ) ;
#15266=CARTESIAN_POINT ( 'NONE',  ( -22.27532461284199528, -3.712691205162892416, -215.8122794664481603 ) ) ;
#15267=CARTESIAN_POINT ( 'NONE',  ( -2.270280637033633475, -14.48864307936496765, -230.4581659391201072 ) ) ;
#15268=CARTESIAN_POINT ( 'NONE',  ( 8.649266908999912573, -10.50942778440553482, -226.4415026780416440 ) ) ;
#15269=CARTESIAN_POINT ( 'NONE',  ( -14.83806045519817829, 13.18806197935771074, -233.4179411789645542 ) ) ;
#15270=CARTESIAN_POINT ( 'NONE',  ( 5.195682580001069084, 14.86321519495278665, -224.7851167466743334 ) ) ;
#15271=CARTESIAN_POINT ( 'NONE',  ( -15.20262116893801974, 8.038155052917188570, -217.6767387945475036 ) ) ;
#15272=CARTESIAN_POINT ( 'NONE',  ( -15.64716994811699813, 6.210654946517923491, -217.0002936794128345 ) ) ;
#15273=CARTESIAN_POINT ( 'NONE',  ( -13.72210242120180901, -11.34614737046836908, -229.0742334187831659 ) ) ;
#15275=CARTESIAN_POINT ( 'NONE',  ( -4.067324790461362305, 15.10342260507846746, -228.2464404076259257 ) ) ;
#15277=CARTESIAN_POINT ( 'NONE',  ( 20.76808360334631232, 5.412616674732960931, -234.1222385626545304 ) ) ;
#15278=CARTESIAN_POINT ( 'NONE',  ( 16.71363093372661979, 20.70203100498337179, -215.6856694095356488 ) ) ;
#15279=CARTESIAN_POINT ( 'NONE',  ( 28.46281617689634302, -10.50803404096709137, -222.5507679334694728 ) ) ;
#15282=CARTESIAN_POINT ( 'NONE',  ( -2.958555384449997661, 13.07587799061801093, -222.7767538261418565 ) ) ;
#15283=CARTESIAN_POINT ( 'NONE',  ( -26.69331514234889013, -17.84497232456928373, -223.5918739730229845 ) ) ;
#15286=CARTESIAN_POINT ( 'NONE',  ( 21.25094435758043332, 17.68230636442804027, -229.7964888993842010 ) ) ;
#15288=CARTESIAN_POINT ( 'NONE',  ( 16.85953475301105442, -7.801609028127129086, -231.9437213283852941 ) ) ;
#15289=CARTESIAN_POINT ( 'NONE',  ( -25.80904414196669450, 12.19501778665756220, -219.1732313092283846 ) ) ;
#15290=CARTESIAN_POINT ( 'NONE',  ( 16.56146809408446430, -0.9616313295950813522, -228.5729530379900609 ) ) ;
#15291=CARTESIAN_POINT ( 'NONE',  ( -11.96638064467250473, -24.81952708901905069, -229.8544473269683692 ) ) ;
#15295=CARTESIAN_POINT ( 'NONE',  ( 12.89891433044458502, -16.86700836158627936, -231.6320225002741040 ) ) ;
#15296=CARTESIAN_POINT ( 'NONE',  ( -22.05223281125446633, 0.4748437386657422543, -217.8785187290425256 ) ) ;
#15298=CARTESIAN_POINT ( 'NONE',  ( 11.05872493453861161, 12.09300746323778775, -226.7727269015348952 ) ) ;
#15299=CARTESIAN_POINT ( 'NONE',  ( 5.720314275582434327, 25.17872937134267630, -219.7530083620574430 ) ) ;
#15300=CARTESIAN_POINT ( 'NONE',  ( 18.85502272441424765, -23.46047257272994102, -219.5236553823413317 ) ) ;
#15301=CARTESIAN_POINT ( 'NONE',  ( 14.99336262864975211, -23.54026314425397004, -231.3018640253376361 ) ) ;
#15305=CARTESIAN_POINT ( 'NONE',  ( -7.375127652145912371, 13.01042140126078195, -223.9959097520547004 ) ) ;
#15306=CARTESIAN_POINT ( 'NONE',  ( -27.28038240442402440, 5.683827137705129040, -226.0726697751923382 ) ) ;
#15307=CARTESIAN_POINT ( 'NONE',  ( 14.68130101653174613, 6.427210486143660084, -228.0153742661088074 ) ) ;
#15309=CARTESIAN_POINT ( 'NONE',  ( -7.103355004864593703, -14.30675315766165312, -225.9889059232917532 ) ) ;
#15313=CARTESIAN_POINT ( 'NONE',  ( 6.839751633953758514, 19.11639828585652623, -235.1218211620789873 ) ) ;
#15314=CARTESIAN_POINT ( 'NONE',  ( 11.86025528723659050, -11.55469215893994850, -227.5711990284272872 ) ) ;
#15315=CARTESIAN_POINT ( 'NONE',  ( 10.66614775643814994, 26.29080367171353672, -230.0818785118670178 ) ) ;
#15316=CARTESIAN_POINT ( 'NONE',  ( -13.92046207272054303, -0.1600067567908077248, -224.5811699126800818 ) ) ;
#15318=CARTESIAN_POINT ( 'NONE',  ( 21.77779027533950540, 18.43917590911969029, -232.9503911151153659 ) ) ;
#15320=CARTESIAN_POINT ( 'NONE',  ( -19.35155980425159683, 1.157993580480985552, -230.3698774940947942 ) ) ;
#15321=CARTESIAN_POINT ( 'NONE',  ( -17.17400284685640344, 24.63223427531467280, -220.6313524368512162 ) ) ;
#15322=CYLINDRICAL_SURFACE ( 'NONE', #1925, 3.000000000000002665 ) ;
#15323=CARTESIAN_POINT ( 'NONE',  ( 5.434900225474387447, -11.93567727083262042, -224.7511004068755369 ) ) ;
#15324=CARTESIAN_POINT ( 'NONE',  ( 19.63495056682994289, -4.096126682090319271, -232.1271738766904207 ) ) ;
#15326=CARTESIAN_POINT ( 'NONE',  ( -23.10791503177032880, -5.282985115830100220, -217.6364121950018671 ) ) ;
#15327=CARTESIAN_POINT ( 'NONE',  ( -11.89542918462869103, -0.2773029175206048191, -224.4556830488584467 ) ) ;
#15328=CARTESIAN_POINT ( 'NONE',  ( -23.54933555373352050, -14.29320362656835997, -227.5895276738501423 ) ) ;
#15330=CARTESIAN_POINT ( 'NONE',  ( 4.725966861008204845, -14.24791254766627624, -227.2781441550517343 ) ) ;
#15331=CARTESIAN_POINT ( 'NONE',  ( -14.07336028695978314, 1.752429266630609828, -222.9750305084206161 ) ) ;
#15332=CARTESIAN_POINT ( 'NONE',  ( -7.240690404266621805, 13.01623002570985044, -225.3000933658701967 ) ) ;
#15333=CARTESIAN_POINT ( 'NONE',  ( -6.079211283031130897, 16.94466709905296753, -232.9163774423793711 ) ) ;
#15335=CARTESIAN_POINT ( 'NONE',  ( 15.86371404000427887, -2.776058937659206638, -233.1947532464443213 ) ) ;
#15336=CARTESIAN_POINT ( 'NONE',  ( 8.496844655769807630, 14.66037471857024599, -219.1631158796573118 ) ) ;
#15338=CARTESIAN_POINT ( 'NONE',  ( -18.88344489807484905, 1.071113352238720617, -230.0966926586188208 ) ) ;
#15339=CARTESIAN_POINT ( 'NONE',  ( -18.04102731735134313, 0.8647102676311391178, -229.4625228093430849 ) ) ;
#15340=CARTESIAN_POINT ( 'NONE',  ( 16.55626903245587656, 22.80423546114836952, -218.9884947126587633 ) ) ;
#15341=CARTESIAN_POINT ( 'NONE',  ( -15.83894155097017631, 1.950284868793920712, -224.5615909987450038 ) ) ;
#15342=CARTESIAN_POINT ( 'NONE',  ( 1.660345614755502686, 12.19060476922103931, -223.1112690039082906 ) ) ;
#15343=CARTESIAN_POINT ( 'NONE',  ( 16.31458447723494132, 2.619382102851042671, -229.5862799001085364 ) ) ;
#15344=CARTESIAN_POINT ( 'NONE',  ( -20.46754208161335598, -23.96478097336112256, -223.3311283152840758 ) ) ;
#15346=CARTESIAN_POINT ( 'NONE',  ( -12.79488508867961549, -11.10380203712096581, -230.9440799972209106 ) ) ;
#15347=ADVANCED_FACE ( 'NONE', ( #13738 ), #22055, .F. ) ;
#15348=CARTESIAN_POINT ( 'NONE',  ( -9.045741320599788082, 11.46901338045063312, -219.0588111342715365 ) ) ;
#15349=CARTESIAN_POINT ( 'NONE',  ( 1.836136847161299990, -12.84546502099244591, -226.1727064218434293 ) ) ;
#15350=CARTESIAN_POINT ( 'NONE',  ( -3.855805549595750392, 26.68244055262801950, -232.4569730455296508 ) ) ;
#15351=CARTESIAN_POINT ( 'NONE',  ( 27.04962740251871978, -7.854494666110665158, -217.8595067830158882 ) ) ;
#15352=CARTESIAN_POINT ( 'NONE',  ( -28.18501077041064562, -8.523171531337160545, -227.0531053546762337 ) ) ;
#15354=CARTESIAN_POINT ( 'NONE',  ( 11.54460987479198053, 9.649171130674412566, -228.7280371210653698 ) ) ;
#15356=CARTESIAN_POINT ( 'NONE',  ( -8.463283775975803280, 12.69606588598396613, -228.6351674091961286 ) ) ;
#15357=CARTESIAN_POINT ( 'NONE',  ( 26.51393280883522863, 15.12455065102723495, -226.1955201378414415 ) ) ;
#15358=CARTESIAN_POINT ( 'NONE',  ( 14.68783945462866924, 9.535285537539673228, -219.4694094309942045 ) ) ;
#15359=CARTESIAN_POINT ( 'NONE',  ( 8.829458998963966465, 22.90677303676718779, -219.2026791561175685 ) ) ;
#15360=CARTESIAN_POINT ( 'NONE',  ( 3.784839621866231241, -12.46827349529254469, -229.8854786719440426 ) ) ;
#15361=CARTESIAN_POINT ( 'NONE',  ( -2.121548062149551495, 13.26065194155116345, -221.8830439064491884 ) ) ;
#15363=CARTESIAN_POINT ( 'NONE',  ( 28.02123297569005089, 5.903198806000402143, -227.5759114383273811 ) ) ;
#15364=CARTESIAN_POINT ( 'NONE',  ( 9.745394341301471641, -28.41975495766811832, -225.7559345954832963 ) ) ;
#15365=CARTESIAN_POINT ( 'NONE',  ( -15.11329978779464689, 11.41628732213579411, -231.7124318929555500 ) ) ;
#15366=CARTESIAN_POINT ( 'NONE',  ( 2.508382434586714282, 15.09451298870656011, -220.9010239894319625 ) ) ;
#15367=CARTESIAN_POINT ( 'NONE',  ( -16.75313578746775889, -14.38352658620038937, -216.6304878158699978 ) ) ;
#15368=CARTESIAN_POINT ( 'NONE',  ( 17.22423229049764970, 1.395540479540137380, -217.3898520248025363 ) ) ;
#15369=CARTESIAN_POINT ( 'NONE',  ( 12.46318849118074112, 25.01309605388695445, -216.9820503660967859 ) ) ;
#15371=CARTESIAN_POINT ( 'NONE',  ( 7.769483725421269860, 20.68783433326350263, -233.2348178266662728 ) ) ;
#15372=CARTESIAN_POINT ( 'NONE',  ( 15.03150297321239925, -8.313127316319620874, -220.7815108570360394 ) ) ;
#15373=CARTESIAN_POINT ( 'NONE',  ( 23.17317677245511831, -6.950782331930943414, -233.5406539459643227 ) ) ;
#15375=CARTESIAN_POINT ( 'NONE',  ( 0.4042326456706432647, 15.50845657815858303, -219.2680337625893401 ) ) ;
#15376=CARTESIAN_POINT ( 'NONE',  ( -15.15102066082706678, -13.26725641419114510, -214.8414790003043322 ) ) ;
#15377=CARTESIAN_POINT ( 'NONE',  ( -6.512931564893298386, -17.32529878264574563, -216.7284160531958719 ) ) ;
#15378=CARTESIAN_POINT ( 'NONE',  ( 6.374306683232226156, -13.38367253400339330, -219.9651431149896723 ) ) ;
#15379=CARTESIAN_POINT ( 'NONE',  ( -18.16160515720599022, 12.42447964075808997, -216.1086293678848449 ) ) ;
#15380=CARTESIAN_POINT ( 'NONE',  ( 15.70200226922815290, 22.14006925444000018, -227.8255507828836244 ) ) ;
#15381=CARTESIAN_POINT ( 'NONE',  ( -12.78558550453068854, 7.693178343823584342, -230.0800953344970878 ) ) ;
#15382=CARTESIAN_POINT ( 'NONE',  ( -30.35034897870229287, 7.696526532841741819, -221.5749790623549416 ) ) ;
#15383=CARTESIAN_POINT ( 'NONE',  ( -22.54540532658949914, -16.00113133426942724, -227.3151344909721843 ) ) ;
#15385=CARTESIAN_POINT ( 'NONE',  ( -10.91003322996498071, 12.84665145358222382, -229.9786893781767958 ) ) ;
#15386=CARTESIAN_POINT ( 'NONE',  ( 24.81079154715000357, 3.171651085595392772, -216.4177249688571578 ) ) ;
#15387=CARTESIAN_POINT ( 'NONE',  ( 11.31331191788792623, 29.23420701778062281, -220.7538464529627333 ) ) ;
#15388=CARTESIAN_POINT ( 'NONE',  ( 10.73531068932428667, -10.59494929936097307, -229.0901643129046192 ) ) ;
#15391=CARTESIAN_POINT ( 'NONE',  ( -8.501641725227710111, 25.47064987787527102, -217.3358698761548737 ) ) ;
#15392=CARTESIAN_POINT ( 'NONE',  ( -18.30187879049682209, -3.992092017665997972, -215.1717549395094693 ) ) ;
#15394=CARTESIAN_POINT ( 'NONE',  ( 28.57344184061583192, 5.631897254180425527, -225.1192013637692355 ) ) ;
#15395=CARTESIAN_POINT ( 'NONE',  ( -26.02440924314744919, 2.824604386891162111, -232.0644005296583430 ) ) ;
#15396=CARTESIAN_POINT ( 'NONE',  ( 9.918856707546316542, -11.48950767347732871, -219.9734948840342668 ) ) ;
#15398=CARTESIAN_POINT ( 'NONE',  ( -14.29986196492902550, 0.06805469746732484282, -227.4167624117703213 ) ) ;
#15399=CARTESIAN_POINT ( 'NONE',  ( 15.28706223449149348, 2.473424253736659306, -227.9634568993954531 ) ) ;
#15400=CARTESIAN_POINT ( 'NONE',  ( -1.339836966046043631, -21.49735173129188581, -217.9043760890963313 ) ) ;
#15402=CARTESIAN_POINT ( 'NONE',  ( 14.85123888640019452, 5.067529763532427012, -221.9058491819374979 ) ) ;
#15403=CARTESIAN_POINT ( 'NONE',  ( -17.84981083811007707, 0.8485253248287054628, -231.8041300026935119 ) ) ;
#15404=CARTESIAN_POINT ( 'NONE',  ( 22.59847068942421444, -14.29990159211854106, -221.3422834976353499 ) ) ;
#15405=CARTESIAN_POINT ( 'NONE',  ( 12.79806454121929349, -2.903405038957567186, -225.7792874317651410 ) ) ;
#15407=CARTESIAN_POINT ( 'NONE',  ( 5.195682580001069084, 14.86321519495278665, -224.7851167466743334 ) ) ;
#15409=CARTESIAN_POINT ( 'NONE',  ( 9.280831573919673616, 14.67893982993557422, -228.6940810986570796 ) ) ;
#15410=CARTESIAN_POINT ( 'NONE',  ( 15.43596206743521826, -16.12492210025319750, -235.0559386399467314 ) ) ;
#15411=CARTESIAN_POINT ( 'NONE',  ( 7.958080982411646076, -16.12895853103474408, -217.0903302464454612 ) ) ;
#15413=CARTESIAN_POINT ( 'NONE',  ( -16.74094048923576494, 16.03040267675914521, -217.9177456399057178 ) ) ;
#15414=CARTESIAN_POINT ( 'NONE',  ( -14.67397018911906770, 9.031553917454052893, -228.4349422195089119 ) ) ;
#15415=CARTESIAN_POINT ( 'NONE',  ( 15.08139719848974103, 12.15862464477973504, -219.3112749338812080 ) ) ;
#15417=CARTESIAN_POINT ( 'NONE',  ( -7.149118023545313783, -16.86598457999096823, -220.1902049135764514 ) ) ;
#15420=CARTESIAN_POINT ( 'NONE',  ( 15.07212457412616224, 2.472408313530222390, -227.3472192494155024 ) ) ;
#15421=CARTESIAN_POINT ( 'NONE',  ( 13.12950778469841318, -23.99547238938880511, -222.5250877844293029 ) ) ;
#15422=CARTESIAN_POINT ( 'NONE',  ( 6.093530912645064745, 16.79941505724243811, -232.1766444656230419 ) ) ;
#15423=CARTESIAN_POINT ( 'NONE',  ( -9.151299407007059017, 9.196974979111923076, -223.9483834032048719 ) ) ;
#15425=CARTESIAN_POINT ( 'NONE',  ( 13.49694890958685711, 2.186465430673721677, -228.8273158381700512 ) ) ;
#15426=CARTESIAN_POINT ( 'NONE',  ( -18.47334320050258327, 24.79293862780133040, -226.9986786077537317 ) ) ;
#15428=CARTESIAN_POINT ( 'NONE',  ( -0.8413160509385254615, -28.71376977722865931, -218.8117683208458288 ) ) ;
#15429=CARTESIAN_POINT ( 'NONE',  ( 23.48720700658024896, -2.145453947144424500, -217.8824464111000054 ) ) ;
#15431=CARTESIAN_POINT ( 'NONE',  ( -28.30937415889876618, -7.921132361018833556, -222.9755670691803857 ) ) ;
#15432=CARTESIAN_POINT ( 'NONE',  ( 21.31262902390056624, 0.4111834581965390645, -232.0572713672585792 ) ) ;
#15433=CARTESIAN_POINT ( 'NONE',  ( -24.13163560393529394, -13.84165259829251227, -223.2936513752361805 ) ) ;
#15435=CARTESIAN_POINT ( 'NONE',  ( 6.203932113039332563, -21.09630782756332223, -232.3325312104709894 ) ) ;
#15436=CARTESIAN_POINT ( 'NONE',  ( -29.16153046926437753, 6.356672163541281506, -226.4393515956758165 ) ) ;
#15437=CARTESIAN_POINT ( 'NONE',  ( 2.703362520412529779, 29.60004130108520215, -225.6165589735000481 ) ) ;
#15438=CARTESIAN_POINT ( 'NONE',  ( -15.64710113362562183, 25.90300453978063189, -220.8637308366217269 ) ) ;
#15439=EDGE_LOOP ( 'NONE', ( #20850, #8322, #3660, #3211, #15047 ) ) ;
#15440=CARTESIAN_POINT ( 'NONE',  ( -22.11234321210701737, -3.359691084028018526, -230.9311713419302521 ) ) ;
#15442=CARTESIAN_POINT ( 'NONE',  ( 10.83706092800007781, 10.12544885278926543, -227.1716144446442343 ) ) ;
#15443=CARTESIAN_POINT ( 'NONE',  ( -16.28135616697389310, 20.98764039357472200, -216.9434553755565958 ) ) ;
#15444=CARTESIAN_POINT ( 'NONE',  ( -25.11055959288653128, 8.701823109978603199, -230.2231080656787583 ) ) ;
#15445=CARTESIAN_POINT ( 'NONE',  ( -10.22552941266963877, -9.699191453761107695, -225.4315674810442545 ) ) ;
#15447=CARTESIAN_POINT ( 'NONE',  ( 24.19635128940818447, 10.31396593861802380, -216.9479509989864425 ) ) ;
#15448=CARTESIAN_POINT ( 'NONE',  ( -18.94009481283715957, 3.115208415279245191, -230.3622730452590588 ) ) ;
#15449=CARTESIAN_POINT ( 'NONE',  ( 12.75306435971521068, 14.56583715532477186, -214.9711136650476533 ) ) ;
#15450=CARTESIAN_POINT ( 'NONE',  ( 24.78377098693636427, 3.871650763546384155, -231.3521132786341923 ) ) ;
#15451=CARTESIAN_POINT ( 'NONE',  ( -18.76818401764774080, -23.60322278862490109, -229.9112526505913365 ) ) ;
#15452=CARTESIAN_POINT ( 'NONE',  ( -10.71823000853037655, -10.52987076429259794, -221.3501620068516331 ) ) ;
#15453=CARTESIAN_POINT ( 'NONE',  ( -14.08083899843152231, 10.81596681319144970, -234.3239311387574446 ) ) ;
#15454=CARTESIAN_POINT ( 'NONE',  ( 1.623338700557370951, -21.82196275546919040, -234.1129525514646730 ) ) ;
#15455=CARTESIAN_POINT ( 'NONE',  ( -1.881996891245037995, 28.05344686410985489, -218.6379207300106202 ) ) ;
#15456=CARTESIAN_POINT ( 'NONE',  ( 14.59690920037431638, -12.12875852167710988, -234.7370354398910877 ) ) ;
#15457=CARTESIAN_POINT ( 'NONE',  ( -16.05483997570105714, -7.226811045751038165, -218.5819178105544438 ) ) ;
#15459=CARTESIAN_POINT ( 'NONE',  ( -14.06164063153489252, 2.050767714179807744, -227.2881998904968270 ) ) ;
#15460=CARTESIAN_POINT ( 'NONE',  ( -5.600903697806950632, 21.62055466701630735, -218.6671277943675307 ) ) ;
#15461=CARTESIAN_POINT ( 'NONE',  ( 24.52160379727246209, 5.049198597839295033, -215.7868787176665535 ) ) ;
#15462=CARTESIAN_POINT ( 'NONE',  ( 18.50911814746675788, 15.92944434255054453, -232.0449215596906072 ) ) ;
#15463=CARTESIAN_POINT ( 'NONE',  ( 22.16327814861754675, 7.634676377199016706, -234.0520676664821735 ) ) ;
#15464=CARTESIAN_POINT ( 'NONE',  ( 6.415926650623908323, -16.27382107952271895, -215.7995092914603674 ) ) ;
#15465=CARTESIAN_POINT ( 'NONE',  ( 2.165130313308041288, 31.55305250914585002, -225.6791154433767304 ) ) ;
#15466=CARTESIAN_POINT ( 'NONE',  ( 7.813662449283098610, -13.08401493520405445, -221.9442578939891177 ) ) ;
#15467=CARTESIAN_POINT ( 'NONE',  ( -12.06153928353927540, 8.661506524875534296, -226.8425068572842349 ) ) ;
#15469=CARTESIAN_POINT ( 'NONE',  ( 0.3632086708616291126, 21.06287758167331958, -232.5112839711303820 ) ) ;
#15470=CARTESIAN_POINT ( 'NONE',  ( -15.74157322273402748, -13.22745315869835636, -216.7831660370879661 ) ) ;
#15471=CARTESIAN_POINT ( 'NONE',  ( 22.42925200799500729, 5.652256920629083581, -234.0734181799116698 ) ) ;
#15472=CARTESIAN_POINT ( 'NONE',  ( 17.10545320562996352, 22.53742678899184781, -232.4605876935045785 ) ) ;
#15474=CARTESIAN_POINT ( 'NONE',  ( 11.13678936984666912, 26.95732789089726111, -228.8350761760834757 ) ) ;
#15475=CARTESIAN_POINT ( 'NONE',  ( 14.12786214016513675, -4.771276416369937046, -223.8547069812204029 ) ) ;
#15476=CARTESIAN_POINT ( 'NONE',  ( 21.85730963248023428, -9.423385237436111339, -216.6089804361807580 ) ) ;
#15477=CARTESIAN_POINT ( 'NONE',  ( 20.41153371889344825, 17.18812948447019551, -230.7531656956970778 ) ) ;
#15478=CARTESIAN_POINT ( 'NONE',  ( -19.82723516873631908, -6.367811336401608457, -234.7370909334860869 ) ) ;
#15479=CARTESIAN_POINT ( 'NONE',  ( -6.012234575298915473, -13.00555924700598709, -229.4955436083688483 ) ) ;
#15481=CARTESIAN_POINT ( 'NONE',  ( 5.451525948382545117, -12.45300865616632713, -227.8545162512558306 ) ) ;
#15482=CARTESIAN_POINT ( 'NONE',  ( -3.130917144532865848, 26.01013079854885390, -229.4331404728494874 ) ) ;
#15483=CARTESIAN_POINT ( 'NONE',  ( 21.68053922431529301, 13.05890675940072931, -230.5667798303363440 ) ) ;
#15484=CARTESIAN_POINT ( 'NONE',  ( -13.58874046263339608, 12.73011668665171392, -216.5659449791897941 ) ) ;
#15485=CARTESIAN_POINT ( 'NONE',  ( -10.30040261405712698, 19.75576125044891285, -218.0811964201226658 ) ) ;
#15486=CARTESIAN_POINT ( 'NONE',  ( 16.07480884343054939, -7.767425703123992164, -217.5935768756353923 ) ) ;
#15487=CARTESIAN_POINT ( 'NONE',  ( -7.240690404266621805, 13.01623002570985044, -225.3000933658701967 ) ) ;
#15488=CARTESIAN_POINT ( 'NONE',  ( 25.62718606866737403, 13.33219119508369310, -230.9315691959737933 ) ) ;
#15489=CARTESIAN_POINT ( 'NONE',  ( 25.41781277602550304, 19.49958712797920057, -223.1230538376805441 ) ) ;
#15490=CARTESIAN_POINT ( 'NONE',  ( 16.26147397530412420, -13.20473954510486081, -216.9283256773164794 ) ) ;
#15491=CARTESIAN_POINT ( 'NONE',  ( 14.46993441875745390, 0.2699826811589002284, -230.0986938382904157 ) ) ;
#15493=CARTESIAN_POINT ( 'NONE',  ( 0.7245137624042983227, 13.44764381486384330, -223.4043886706536455 ) ) ;
#15494=CARTESIAN_POINT ( 'NONE',  ( -27.51824122704870135, -10.15715933399136617, -232.3556155038515669 ) ) ;
#15496=CARTESIAN_POINT ( 'NONE',  ( 17.00168025137501004, 6.212099629982537508, -219.0548246536471595 ) ) ;
#15498=CARTESIAN_POINT ( 'NONE',  ( 17.15627899979664051, -18.64955541608202694, -217.1729447097152388 ) ) ;
#15500=CARTESIAN_POINT ( 'NONE',  ( -13.93333636822611155, 3.327141996558931947, -221.4468162587888287 ) ) ;
#15501=CARTESIAN_POINT ( 'NONE',  ( -14.07917727715460821, 7.534853284453274291, -218.6337090155677458 ) ) ;
#15502=CARTESIAN_POINT ( 'NONE',  ( -4.994543945659216000, -15.01629888130124435, -221.3392717856295633 ) ) ;
#15505=CARTESIAN_POINT ( 'NONE',  ( -28.99926036811508467, 3.909990568804979194, -228.9613767892386988 ) ) ;
#15506=CARTESIAN_POINT ( 'NONE',  ( 23.95414175253014477, -14.38191447464009087, -225.3623377062671125 ) ) ;
#15507=CARTESIAN_POINT ( 'NONE',  ( 13.43601330613756595, -1.788726811927666915, -222.5908311466273517 ) ) ;
#15509=CARTESIAN_POINT ( 'NONE',  ( 11.00580183749007190, 25.74996642444834904, -225.8602305833924788 ) ) ;
#15510=CARTESIAN_POINT ( 'NONE',  ( 20.22510869507564024, 17.05975164568011238, -220.7829296213589316 ) ) ;
#15511=CARTESIAN_POINT ( 'NONE',  ( 2.920206608988989760, -13.21961856575012639, -224.5557534934820865 ) ) ;
#15512=CARTESIAN_POINT ( 'NONE',  ( 21.30961698559626427, -20.48616475849644303, -228.5322376518520002 ) ) ;
#15514=CARTESIAN_POINT ( 'NONE',  ( -10.02095171162140019, 11.02119725306997111, -224.1251327387667516 ) ) ;
#15515=CARTESIAN_POINT ( 'NONE',  ( -15.82068653568960137, 8.372322471091806051, -220.7139663195713979 ) ) ;
#15516=CARTESIAN_POINT ( 'NONE',  ( -13.33011381921379090, 5.829915729572584304, -219.4453182727427816 ) ) ;
#15517=CARTESIAN_POINT ( 'NONE',  ( -7.469054245001129466, -18.21857363335801594, -219.2823717272210047 ) ) ;
#15520=CARTESIAN_POINT ( 'NONE',  ( 24.60354977307301283, 7.993510024274534942, -218.5358880819990759 ) ) ;
#15521=CARTESIAN_POINT ( 'NONE',  ( 8.587407344280324040, -17.24386586482343375, -219.6634241328915209 ) ) ;
#15522=CARTESIAN_POINT ( 'NONE',  ( 9.333020543840051531, 16.91085096921651143, -217.7308990335875762 ) ) ;
#15524=CARTESIAN_POINT ( 'NONE',  ( -10.84997096467605182, 25.01800101807719301, -232.4518260228253155 ) ) ;
#15526=CARTESIAN_POINT ( 'NONE',  ( 22.66015888791822519, 10.43487984001084534, -234.3950629709119937 ) ) ;
#15528=CARTESIAN_POINT ( 'NONE',  ( 1.217121169770782663, 15.31158828575123110, -230.6845728599757308 ) ) ;
#15530=CARTESIAN_POINT ( 'NONE',  ( -4.670971249126254499, -22.80666086768999890, -234.0323572959307512 ) ) ;
#15531=CARTESIAN_POINT ( 'NONE',  ( 14.34945462593695531, -6.128426910066905542, -229.1128190117150041 ) ) ;
#15534=CARTESIAN_POINT ( 'NONE',  ( -15.39319649241581800, 0.3563955590804028795, -232.4397289486159082 ) ) ;
#15535=CARTESIAN_POINT ( 'NONE',  ( -9.080867962954789263, -15.08739678120475780, -231.4478131780767001 ) ) ;
#15537=CARTESIAN_POINT ( 'NONE',  ( 5.920190106170357680, -27.41802839654005197, -221.0732524667164114 ) ) ;
#15538=CARTESIAN_POINT ( 'NONE',  ( -16.27882490622757672, 1.520697279646460398, -219.2607721384596289 ) ) ;
#15539=CARTESIAN_POINT ( 'NONE',  ( 9.527502190795640757, 23.55559004943647139, -217.4101659741468211 ) ) ;
#15540=CARTESIAN_POINT ( 'NONE',  ( 1.719513778997906694, 15.52930330544231730, -222.3959083836286368 ) ) ;
#15542=CARTESIAN_POINT ( 'NONE',  ( 27.25858960103340323, -9.764658377823966617, -217.2703135185301448 ) ) ;
#15544=CARTESIAN_POINT ( 'NONE',  ( 9.333020543840051531, 16.91085096921651143, -217.7308990335875762 ) ) ;
#15547=CARTESIAN_POINT ( 'NONE',  ( -24.30769394037691100, 17.48612956801762053, -223.4340414801748693 ) ) ;
#15548=CARTESIAN_POINT ( 'NONE',  ( -15.72195651633673208, 2.938252489821347346, -222.2698596109374023 ) ) ;
#15549=CARTESIAN_POINT ( 'NONE',  ( -15.43902962033193837, -12.71219713885795422, -232.7078469548986845 ) ) ;
#15550=CARTESIAN_POINT ( 'NONE',  ( 14.99872922520050977, -2.000037915366065899, -222.7619559412280807 ) ) ;
#15551=CARTESIAN_POINT ( 'NONE',  ( 26.59731715018858011, 13.56210517473685329, -229.5787264587298466 ) ) ;
#15552=CARTESIAN_POINT ( 'NONE',  ( -15.77374768176864173, 20.07639682234129097, -218.6858893794192795 ) ) ;
#15553=CARTESIAN_POINT ( 'NONE',  ( 14.96462366732929716, 7.179279272144128754, -233.2042342402542374 ) ) ;
#15554=CARTESIAN_POINT ( 'NONE',  ( 15.88965480228581839, 12.37830464553330678, -233.8570207506254235 ) ) ;
#15556=CARTESIAN_POINT ( 'NONE',  ( -15.42652243319914085, -1.944528292506083167, -233.0911082444762030 ) ) ;
#15558=CARTESIAN_POINT ( 'NONE',  ( -4.902442737337177725, -13.94343087703807704, -224.3742458082145959 ) ) ;
#15559=CARTESIAN_POINT ( 'NONE',  ( -20.38637754046084183, 19.95723714148678241, -217.5201383746364172 ) ) ;
#15560=CARTESIAN_POINT ( 'NONE',  ( 9.358654279681809740, -11.94480763145079472, -229.8864256833185777 ) ) ;
#15561=CARTESIAN_POINT ( 'NONE',  ( 2.837900457371055563, 25.11342719071438978, -232.9871906064174709 ) ) ;
#15562=CARTESIAN_POINT ( 'NONE',  ( 15.97952439233267263, -1.339455371059026456, -231.0376074705642395 ) ) ;
#15564=CARTESIAN_POINT ( 'NONE',  ( 16.48801037644500056, 3.165716804515234628, -216.8169430726136113 ) ) ;
#15566=CARTESIAN_POINT ( 'NONE',  ( -1.158668551263366986, 23.31492692626720853, -219.2372600964201865 ) ) ;
#15567=CARTESIAN_POINT ( 'NONE',  ( -15.83178333309709629, 2.467763724635483324, -230.4064772870105458 ) ) ;
#15568=CARTESIAN_POINT ( 'NONE',  ( 17.19674704922021391, 23.07334190050143974, -228.8256488842130238 ) ) ;
#15569=CARTESIAN_POINT ( 'NONE',  ( 21.27683256847563698, 4.223177115764435108, -215.2584548172064842 ) ) ;
#15570=CARTESIAN_POINT ( 'NONE',  ( 2.898952953659251985, -22.97888022809681274, -215.2852275949887826 ) ) ;
#15571=CARTESIAN_POINT ( 'NONE',  ( 3.001892273201697048, 27.20292285420111966, -216.7800154582108689 ) ) ;
#15574=CARTESIAN_POINT ( 'NONE',  ( 15.01439307471096463, 1.118969480519667048, -226.7488225241675366 ) ) ;
#15575=CARTESIAN_POINT ( 'NONE',  ( -3.877698871368953082, -12.59008950621349676, -229.3284496285515388 ) ) ;
#15576=CARTESIAN_POINT ( 'NONE',  ( -9.233762381136051189, 19.18161952504991419, -232.0796851897838451 ) ) ;
#15577=CARTESIAN_POINT ( 'NONE',  ( 9.798337081649805214, 12.27506320122302697, -218.9346733583377613 ) ) ;
#15579=CARTESIAN_POINT ( 'NONE',  ( -14.37894460687751597, -1.926260335694933268, -225.0161641904981593 ) ) ;
#15580=CARTESIAN_POINT ( 'NONE',  ( -21.67128887413246119, 15.53484693247673043, -229.0088198863946900 ) ) ;
#15581=CARTESIAN_POINT ( 'NONE',  ( -14.58670098223046629, 7.239570004716886942, -229.3284954533748135 ) ) ;
#15582=CARTESIAN_POINT ( 'NONE',  ( 28.56567312134318826, 3.451746495494312672, -224.1550573921799412 ) ) ;
#15584=CARTESIAN_POINT ( 'NONE',  ( 5.069241901512100412, 14.34986542013820632, -229.6420000777802954 ) ) ;
#15585=CARTESIAN_POINT ( 'NONE',  ( 12.68099841568652764, -20.61692530233158394, -230.4218470428317573 ) ) ;
#15587=CARTESIAN_POINT ( 'NONE',  ( 14.58943670538545412, -3.864781073802256550, -230.4050158740328129 ) ) ;
#15588=CARTESIAN_POINT ( 'NONE',  ( -3.071946796551161984, 23.17078151772539485, -231.0066194318698933 ) ) ;
#15589=CARTESIAN_POINT ( 'NONE',  ( 15.91295838535984331, 21.88410254487826379, -230.9583961155862823 ) ) ;
#15590=CARTESIAN_POINT ( 'NONE',  ( -20.52308621596579030, -13.62600152083235905, -234.9101091540371442 ) ) ;
#15591=CARTESIAN_POINT ( 'NONE',  ( 0.7326557587344989519, -29.96088689026728602, -229.4725774697800205 ) ) ;
#15593=CARTESIAN_POINT ( 'NONE',  ( 10.10435529162921853, -13.32996982371095918, -231.5224098423250894 ) ) ;
#15595=CARTESIAN_POINT ( 'NONE',  ( -2.612157044224189484, 27.88031182936952135, -224.5292183073761692 ) ) ;
#15597=CARTESIAN_POINT ( 'NONE',  ( 15.33128967029630729, 6.504525012335983902, -229.0514072561169883 ) ) ;
#15598=CARTESIAN_POINT ( 'NONE',  ( -11.46843428684449151, 6.508406145394057596, -225.7212143570321814 ) ) ;
#15599=CARTESIAN_POINT ( 'NONE',  ( -14.98215928292561294, 22.79623052288931362, -230.3289734367122890 ) ) ;
#15600=CARTESIAN_POINT ( 'NONE',  ( -24.76242154467160717, -4.839146110080178254, -231.6857664014047202 ) ) ;
#15602=CARTESIAN_POINT ( 'NONE',  ( 2.951582164238582440, 19.39026647431845873, -217.4356918981242472 ) ) ;
#15603=CARTESIAN_POINT ( 'NONE',  ( -24.82235633397527508, 10.76243500821901300, -227.9886044494091948 ) ) ;
#15604=CARTESIAN_POINT ( 'NONE',  ( 15.51445714770079931, 9.275596138242290678, -215.8565574371285436 ) ) ;
#15605=CARTESIAN_POINT ( 'NONE',  ( 4.999282783285113219, -13.99249059192112021, -223.3817383379047214 ) ) ;
#15607=ORIENTED_EDGE ( 'NONE', *, *, #5134, .F. ) ;
#15608=CARTESIAN_POINT ( 'NONE',  ( -7.913358619554302642, 16.16796202616373890, -233.0981776325470491 ) ) ;
#15609=CARTESIAN_POINT ( 'NONE',  ( 25.75976839005050323, -3.608312289253767347, -220.3697909415571417 ) ) ;
#15610=CARTESIAN_POINT ( 'NONE',  ( 16.38151749656409351, 8.902090001712490874, -231.2955017965201989 ) ) ;
#15611=CARTESIAN_POINT ( 'NONE',  ( -13.11494368899652052, 3.355507568391938200, -225.9121440085824304 ) ) ;
#15612=CARTESIAN_POINT ( 'NONE',  ( 10.40291689048662782, -13.87512507945592333, -231.9656913702303029 ) ) ;
#15613=CARTESIAN_POINT ( 'NONE',  ( -14.73016414256368911, 22.23431809695627237, -217.1425123644553707 ) ) ;
#15615=CARTESIAN_POINT ( 'NONE',  ( 19.30248206944178335, -1.297331563427565726, -230.8957665284791290 ) ) ;
#15616=CARTESIAN_POINT ( 'NONE',  ( -7.084830653876206696, -25.45310193036084456, -219.3007580301989492 ) ) ;
#15619=CARTESIAN_POINT ( 'NONE',  ( -19.00318367631585659, 13.14621133775862916, -233.8403879275295765 ) ) ;
#15620=CARTESIAN_POINT ( 'NONE',  ( 18.63320037895408277, -18.75851321891666146, -220.1409915463867151 ) ) ;
#15621=CARTESIAN_POINT ( 'NONE',  ( 14.11699743667134399, -1.517512230688333963, -222.4120480544196994 ) ) ;
#15623=CARTESIAN_POINT ( 'NONE',  ( 20.58393751692968721, 18.55948753678544705, -226.8933397075267635 ) ) ;
#15625=CARTESIAN_POINT ( 'NONE',  ( -5.298027976154672025, 13.43376398981453157, -220.6333279128949982 ) ) ;
#15626=CARTESIAN_POINT ( 'NONE',  ( 20.90058474538433231, 18.60939544422136294, -225.8027644507526475 ) ) ;
#15627=CARTESIAN_POINT ( 'NONE',  ( -3.190684129821126813, -24.11035010539542611, -218.3286195476113392 ) ) ;
#15628=CARTESIAN_POINT ( 'NONE',  ( 24.71064586368820315, -12.65488197590634378, -232.9862317762581654 ) ) ;
#15629=VERTEX_POINT ( 'NONE', #9233 ) ;
#15631=CARTESIAN_POINT ( 'NONE',  ( 0.1556102272723409452, 19.71550568250159685, -232.1993058477363547 ) ) ;
#15632=CARTESIAN_POINT ( 'NONE',  ( -21.10507617219916199, 14.90539259013048756, -229.7677326419877488 ) ) ;
#15633=CARTESIAN_POINT ( 'NONE',  ( -19.59898341672158040, 3.279988180491820504, -234.9371679595475086 ) ) ;
#15636=CARTESIAN_POINT ( 'NONE',  ( -14.93084585968405875, -14.53813297593447373, -219.1962364975631772 ) ) ;
#15639=CARTESIAN_POINT ( 'NONE',  ( 17.66865342763861690, 2.849170916951684784, -230.9175656266857004 ) ) ;
#15640=CARTESIAN_POINT ( 'NONE',  ( 13.43702744235484303, -16.51261215982735209, -219.1853238157515875 ) ) ;
#15641=CARTESIAN_POINT ( 'NONE',  ( 13.69275646168278371, 8.674223198772375909, -220.8699857572541987 ) ) ;
#15642=CARTESIAN_POINT ( 'NONE',  ( -9.540790481621398200, 9.981116473660406996, -228.6478862620407995 ) ) ;
#15643=CARTESIAN_POINT ( 'NONE',  ( 11.75404126451729070, 5.688294280104953415, -229.3533586468489602 ) ) ;
#15644=CARTESIAN_POINT ( 'NONE',  ( 12.53674998645855787, 17.96979015029927851, -232.8843215672231679 ) ) ;
#15647=CARTESIAN_POINT ( 'NONE',  ( 2.513843158659109456, -14.78137297724497401, -219.3443999184743518 ) ) ;
#15649=CARTESIAN_POINT ( 'NONE',  ( 17.01060404384151781, -6.151862203644831162, -218.3248062500343849 ) ) ;
#15652=CARTESIAN_POINT ( 'NONE',  ( -22.04004491965229207, 12.41871177236473578, -215.2165492276571115 ) ) ;
#15653=CARTESIAN_POINT ( 'NONE',  ( -23.72332483825893235, -1.495203899552344007, -219.0564715008207770 ) ) ;
#15654=CARTESIAN_POINT ( 'NONE',  ( 15.89621445970763070, 6.639162626453350313, -232.5295318698041456 ) ) ;
#15655=CARTESIAN_POINT ( 'NONE',  ( 2.808299412262623473, 18.06245856371233316, -217.9832661743849656 ) ) ;
#15656=CARTESIAN_POINT ( 'NONE',  ( -1.336753021691559962, 16.04398320409420720, -230.2310715620304507 ) ) ;
#15658=CARTESIAN_POINT ( 'NONE',  ( 15.13468687495441323, -1.603572186776826447, -217.3101985623318626 ) ) ;
#15659=CARTESIAN_POINT ( 'NONE',  ( 27.40550551777678123, 5.967061366481472895, -228.7463788799179554 ) ) ;
#15660=CARTESIAN_POINT ( 'NONE',  ( -11.01414002179357610, 8.614420160880040811, -226.3770540798392972 ) ) ;
#15661=CARTESIAN_POINT ( 'NONE',  ( -13.48133478602219171, 10.24771958306113362, -218.3822527490931691 ) ) ;
#15662=CARTESIAN_POINT ( 'NONE',  ( -6.776147227169700749, -16.68571135823561846, -231.0772860317820232 ) ) ;
#15663=CARTESIAN_POINT ( 'NONE',  ( -18.08305592660031991, 4.022743421239192152, -217.2335041149100050 ) ) ;
#15667=CARTESIAN_POINT ( 'NONE',  ( 14.80781494020099132, -2.823191316056344657, -223.9669636951288965 ) ) ;
#15669=CARTESIAN_POINT ( 'NONE',  ( -21.67128887413246119, 15.53484693247673043, -229.0088198863946900 ) ) ;
#15670=CARTESIAN_POINT ( 'NONE',  ( 25.12984891811676036, 19.96069634721137476, -226.7154725927711070 ) ) ;
#15671=CARTESIAN_POINT ( 'NONE',  ( -28.59157645096996347, 5.137867505054540374, -220.4667042235044505 ) ) ;
#15672=CARTESIAN_POINT ( 'NONE',  ( -31.13345889576667247, -1.683779982087686422, -229.5421043233184264 ) ) ;
#15674=CARTESIAN_POINT ( 'NONE',  ( -15.43902962033193837, -12.71219713885795422, -232.7078469548986845 ) ) ;
#15675=CARTESIAN_POINT ( 'NONE',  ( -8.201407585998298444, 17.38801480109368924, -216.6295241303755006 ) ) ;
#15676=CARTESIAN_POINT ( 'NONE',  ( -14.84823930505322132, -23.35465403802561823, -218.3226235040776260 ) ) ;
#15677=CARTESIAN_POINT ( 'NONE',  ( 12.18657022793382794, 26.76558097653315471, -221.8882195427397335 ) ) ;
#15678=CARTESIAN_POINT ( 'NONE',  ( 9.622280932921700725, -12.40415793303572300, -216.8820201732712860 ) ) ;
#15682=CARTESIAN_POINT ( 'NONE',  ( -14.07336028695978314, 1.752429266630609828, -222.9750305084206161 ) ) ;
#15683=CARTESIAN_POINT ( 'NONE',  ( -3.504118661534079582, 16.69899759879061918, -221.4378787282527128 ) ) ;
#15684=CARTESIAN_POINT ( 'NONE',  ( -16.32047052250102581, 2.570795953410685009, -230.9329235942756213 ) ) ;
#15685=CARTESIAN_POINT ( 'NONE',  ( -14.70339349403010942, -0.4153334646997780544, -217.8790668391084466 ) ) ;
#15686=CARTESIAN_POINT ( 'NONE',  ( 15.14536540539411114, 2.907144070186200580, -217.8738854795238922 ) ) ;
#15687=CARTESIAN_POINT ( 'NONE',  ( 2.374937041136545801, -21.24827930241302099, -215.2851479487023312 ) ) ;
#15688=CARTESIAN_POINT ( 'NONE',  ( 6.523529190399725231, 13.69551997595937465, -217.3678933099786832 ) ) ;
#15689=CARTESIAN_POINT ( 'NONE',  ( 14.98418162551161714, 4.450317369940187895, -227.9894155827521161 ) ) ;
#15690=CARTESIAN_POINT ( 'NONE',  ( -3.265885032814331623, -11.59335615597398217, -224.1764024733101053 ) ) ;
#15691=CARTESIAN_POINT ( 'NONE',  ( -5.365396334125453137, 16.47374957271378904, -219.4721119688156534 ) ) ;
#15693=CARTESIAN_POINT ( 'NONE',  ( 14.69879291197755222, 10.86005690695417236, -216.7815908316746913 ) ) ;
#15694=CARTESIAN_POINT ( 'NONE',  ( -15.46216926290318305, -2.495270579625169738, -221.2150947962298631 ) ) ;
#15695=CARTESIAN_POINT ( 'NONE',  ( -22.36207348798144778, 17.12313795477538036, -223.8571857210765472 ) ) ;
#15696=CARTESIAN_POINT ( 'NONE',  ( -10.01410430826631170, 16.10970239316000630, -233.6135099156378203 ) ) ;
#15697=B_SPLINE_CURVE_WITH_KNOTS ( 'NONE', 3,
 ( #8631, #8963, #13924, #15491, #404, #7278, #14148, #20985, #14261, #19404 ),
 .UNSPECIFIED., .F., .F.,
 ( 4, 2, 2, 2, 4 ),
 ( 0.4921208414669437925, 0.4926212833915588618, 0.4960388740592901469, 0.4979917830122794764, 0.4999446919652688059 ),
 .UNSPECIFIED. ) ;
#15698=CARTESIAN_POINT ( 'NONE',  ( 17.76485367938521875, 4.373152267827974171, -218.8623009891758215 ) ) ;
#15700=CARTESIAN_POINT ( 'NONE',  ( 12.41447124200992391, -12.24348532208574269, -228.9129928441363973 ) ) ;
#15702=CARTESIAN_POINT ( 'NONE',  ( 5.377793152941013233, -17.45375835550001753, -231.2474386379397231 ) ) ;
#15703=CARTESIAN_POINT ( 'NONE',  ( -4.285397168228398890, 18.56782363833054106, -219.4990091916804715 ) ) ;
#15706=CARTESIAN_POINT ( 'NONE',  ( 15.33737796850231305, 13.57479350230705428, -232.3313557812109025 ) ) ;
#15707=CARTESIAN_POINT ( 'NONE',  ( 14.64930099072384095, -2.233284345536625803, -226.6630761355773984 ) ) ;
#15708=CARTESIAN_POINT ( 'NONE',  ( -1.608171596096409806, -16.77465153034988887, -217.4618546331240054 ) ) ;
#15709=CARTESIAN_POINT ( 'NONE',  ( 7.080148886126969465, -28.65852557119563926, -219.9679292432588227 ) ) ;
#15710=CARTESIAN_POINT ( 'NONE',  ( -3.125843203957122896, 15.99774916147792680, -222.8808123721668721 ) ) ;
#15712=CARTESIAN_POINT ( 'NONE',  ( 25.18311526135610734, 13.65721788432563955, -224.7326014392022273 ) ) ;
#15713=CARTESIAN_POINT ( 'NONE',  ( -10.30050448363967419, 10.07750059423401190, -220.1837019037183723 ) ) ;
#15714=CARTESIAN_POINT ( 'NONE',  ( -3.504118661534079582, 16.69899759879061918, -221.4378787282527128 ) ) ;
#15716=CARTESIAN_POINT ( 'NONE',  ( 1.656472371294090085, 27.29382523973669095, -230.4991099578876117 ) ) ;
#15717=CARTESIAN_POINT ( 'NONE',  ( -17.72669652144150376, 1.460525322529694581, -220.6883622781615202 ) ) ;
#15718=CARTESIAN_POINT ( 'NONE',  ( 9.169328349715531346, 20.85917603618721472, -214.7000934853629133 ) ) ;
#15719=CARTESIAN_POINT ( 'NONE',  ( 6.025688374458400887, -15.61258154445926749, -220.0079782759978002 ) ) ;
#15722=CARTESIAN_POINT ( 'NONE',  ( -3.673551555920188783, 29.81207051619892923, -228.8770490300152005 ) ) ;
#15723=CARTESIAN_POINT ( 'NONE',  ( -27.90711606799872513, 0.4679914357742857023, -216.8754026763949128 ) ) ;
#15724=CARTESIAN_POINT ( 'NONE',  ( 28.33476664927451338, -0.7768526459456059907, -228.3750448408243869 ) ) ;
#15725=CARTESIAN_POINT ( 'NONE',  ( 18.60971343765040942, 2.368090295052050820, -218.6871071987073094 ) ) ;
#15726=CARTESIAN_POINT ( 'NONE',  ( -21.93900267957129557, 7.862893636934532360, -233.4951761057262161 ) ) ;
#15727=CARTESIAN_POINT ( 'NONE',  ( 2.378655016347637652, -14.31292064579845302, -219.9942319014987220 ) ) ;
#15728=CARTESIAN_POINT ( 'NONE',  ( -8.172572110426221670, 16.86653848210977813, -233.4220330256369493 ) ) ;
#15729=CARTESIAN_POINT ( 'NONE',  ( -11.59479561055411345, 9.544396733298208702, -229.1494558965577255 ) ) ;
#15731=CARTESIAN_POINT ( 'NONE',  ( -29.88125065636863198, 4.504452993877526623, -226.2048141718237275 ) ) ;
#15732=CARTESIAN_POINT ( 'NONE',  ( -8.983992482398329926, -13.08794618741998761, -229.3325301586503713 ) ) ;
#15735=CARTESIAN_POINT ( 'NONE',  ( -17.79285498209129202, 9.187865686019035749, -216.3798185811636756 ) ) ;
#15736=CARTESIAN_POINT ( 'NONE',  ( 1.345830553852720657, -29.56269728401072783, -219.9360760428637604 ) ) ;
#15739=CARTESIAN_POINT ( 'NONE',  ( 17.51175949430614409, 14.31829016556564937, -218.8195841045835550 ) ) ;
#15740=CARTESIAN_POINT ( 'NONE',  ( -4.450022810944913587, 12.45400981846350597, -225.2098051417536340 ) ) ;
#15742=CARTESIAN_POINT ( 'NONE',  ( 15.88536911906737181, 12.85343532334862893, -218.9532478288372204 ) ) ;
#15743=CARTESIAN_POINT ( 'NONE',  ( 4.746237488610151267, -29.30821474977460639, -222.1257927337785247 ) ) ;
#15744=CARTESIAN_POINT ( 'NONE',  ( 23.77009720158773831, -0.5966687509537305090, -216.6384684467892043 ) ) ;
#15747=CARTESIAN_POINT ( 'NONE',  ( -4.224287562409271501, 29.03635716824519264, -224.1823526280761882 ) ) ;
#15748=CARTESIAN_POINT ( 'NONE',  ( -24.48812334466693486, 4.469247780253509106, -230.3044243311433945 ) ) ;
#15749=CARTESIAN_POINT ( 'NONE',  ( -11.84805200323110164, 5.835720598137266180, -228.2740675967047537 ) ) ;
#15750=CARTESIAN_POINT ( 'NONE',  ( -22.39763175122653038, -14.70415172796113623, -221.0757120432126612 ) ) ;
#15753=CARTESIAN_POINT ( 'NONE',  ( 17.81160404892403193, 9.939217752910943560, -216.9646549374535311 ) ) ;
#15754=CARTESIAN_POINT ( 'NONE',  ( 0.005738405568439595983, -15.19016956849912070, -227.2100150994057230 ) ) ;
#15755=CARTESIAN_POINT ( 'NONE',  ( 10.55627441269396094, 10.31758739525044888, -223.1990319438957613 ) ) ;
#15756=CARTESIAN_POINT ( 'NONE',  ( -17.65835845419170624, 22.55329142274348442, -231.2673511165784532 ) ) ;
#15758=CARTESIAN_POINT ( 'NONE',  ( 14.81258087342262364, 2.398747990731791013, -230.9000679928271040 ) ) ;
#15759=CARTESIAN_POINT ( 'NONE',  ( 2.837900457371055563, 25.11342719071438978, -232.9871906064174709 ) ) ;
#15760=CARTESIAN_POINT ( 'NONE',  ( 15.26418234037447164, 1.657826554291933485, -222.4969140426460683 ) ) ;
#15762=CARTESIAN_POINT ( 'NONE',  ( -1.633632075387274840, -15.48245080501611071, -218.5193615163172751 ) ) ;
#15763=CARTESIAN_POINT ( 'NONE',  ( 22.14671607713456325, -14.13547298543019437, -218.1897693226341914 ) ) ;
#15765=DIRECTION ( 'NONE',  ( 1.000000000000000000, 0.000000000000000000, 0.000000000000000000 ) ) ;
#15766=CARTESIAN_POINT ( 'NONE',  ( -9.491065840222427497, 13.31995980477872266, -232.8537120564120073 ) ) ;
#15767=CARTESIAN_POINT ( 'NONE',  ( -27.87965705189043675, -2.801641921304233840, -225.5825458398584260 ) ) ;
#15768=CARTESIAN_POINT ( 'NONE',  ( 17.34461553379066601, 6.893916422670210764, -233.3442385185644525 ) ) ;
#15769=CARTESIAN_POINT ( 'NONE',  ( 5.803912621764987456, 13.01725692290267844, -221.8367675400179166 ) ) ;
#15770=CARTESIAN_POINT ( 'NONE',  ( -2.043230952238195286, 23.63069326910348877, -232.6835180461029040 ) ) ;
#15771=ORIENTED_EDGE ( 'NONE', *, *, #10238, .T. ) ;
#15772=CARTESIAN_POINT ( 'NONE',  ( 13.13237050162318553, -11.26662123460813092, -216.1773046078333209 ) ) ;
#15774=CARTESIAN_POINT ( 'NONE',  ( 27.75679124201660741, 4.911524026080384075, -221.4430403652340829 ) ) ;
#15775=CARTESIAN_POINT ( 'NONE',  ( -13.63002737749749826, 6.315035547785179837, -227.0490028799284516 ) ) ;
#15776=CARTESIAN_POINT ( 'NONE',  ( -11.94727018630768178, 9.025563988971828877, -220.6148682757971358 ) ) ;
#15777=CARTESIAN_POINT ( 'NONE',  ( -28.43596199216294806, -10.51226423640377838, -227.0041752157952430 ) ) ;
#15778=CARTESIAN_POINT ( 'NONE',  ( -13.55591840520136770, 8.363404288414606924, -231.2690188357804857 ) ) ;
#15782=CARTESIAN_POINT ( 'NONE',  ( 14.50618777373884960, 4.375057440872940795, -230.8807389798650433 ) ) ;
#15783=CARTESIAN_POINT ( 'NONE',  ( -18.59263364681495290, 22.28600439725833482, -224.9897462721271779 ) ) ;
#15784=CARTESIAN_POINT ( 'NONE',  ( 5.784594921161807513, 11.98867617302893329, -219.3746160931291058 ) ) ;
#15785=CARTESIAN_POINT ( 'NONE',  ( 20.54442553493903389, -1.409480604460696007, -231.2888200459364327 ) ) ;
#15786=CARTESIAN_POINT ( 'NONE',  ( -17.45568254742804370, -7.678338623619185732, -234.9220303918225738 ) ) ;
#15787=CARTESIAN_POINT ( 'NONE',  ( -29.05925532287432489, -3.238226816112620199, -230.1495230746535867 ) ) ;
#15788=CARTESIAN_POINT ( 'NONE',  ( -21.64120863631820413, 17.87363223393748868, -233.1390268986752119 ) ) ;
#15789=CARTESIAN_POINT ( 'NONE',  ( -15.46269062504165781, -26.67469327287815517, -225.2085449711190677 ) ) ;
#15790=CARTESIAN_POINT ( 'NONE',  ( 7.769483725421269860, 20.68783433326350263, -233.2348178266662728 ) ) ;
#15791=CARTESIAN_POINT ( 'NONE',  ( 7.023652882903417272, -9.473209335044964874, -223.0206350579724983 ) ) ;
#15793=CARTESIAN_POINT ( 'NONE',  ( -22.13857085231108712, 6.545953331035805789, -217.2801712530867633 ) ) ;
#15795=CARTESIAN_POINT ( 'NONE',  ( 1.030230143518703345, 18.27887886751213387, -229.5791973322770616 ) ) ;
#15796=CARTESIAN_POINT ( 'NONE',  ( 12.47670316482120967, 2.249148913447538423, -227.4574095259895898 ) ) ;
#15797=CARTESIAN_POINT ( 'NONE',  ( 20.34032485158648029, 2.741617426884598530, -217.9827731991294968 ) ) ;
#15798=CARTESIAN_POINT ( 'NONE',  ( 26.75666476377482539, 8.100664119735744961, -232.1611550320539834 ) ) ;
#15799=CARTESIAN_POINT ( 'NONE',  ( -9.080867962954789263, -15.08739678120475780, -231.4478131780767001 ) ) ;
#15800=CARTESIAN_POINT ( 'NONE',  ( 2.068961274655788607, 15.13167107497539376, -217.8084559455312501 ) ) ;
#15802=CARTESIAN_POINT ( 'NONE',  ( 0.3659801352207852077, -13.50984377477715093, -221.1746532791751463 ) ) ;
#15803=CARTESIAN_POINT ( 'NONE',  ( -4.742143146070755932, 15.01230778631049567, -221.4832709320255049 ) ) ;
#15804=CARTESIAN_POINT ( 'NONE',  ( 9.211411085256067111, 16.86455563410128633, -232.8411836211112700 ) ) ;
#15805=CARTESIAN_POINT ( 'NONE',  ( -26.22594988380878789, -0.1068133454905619700, -219.1167922977186322 ) ) ;
#15806=CARTESIAN_POINT ( 'NONE',  ( -15.07599795178976443, 12.40109266655585429, -218.9921934537110815 ) ) ;
#15807=CARTESIAN_POINT ( 'NONE',  ( -6.111257124579617894, 15.89946952501658295, -216.3497764690875727 ) ) ;
#15808=CARTESIAN_POINT ( 'NONE',  ( 27.58248235015124550, 10.80791576765187934, -226.6933256641281389 ) ) ;
#15810=CARTESIAN_POINT ( 'NONE',  ( 6.772180301198498675, -16.47206380092378097, -229.1778777248402719 ) ) ;
#15812=CARTESIAN_POINT ( 'NONE',  ( 13.60960062514055657, -26.18013421850907108, -225.9721930653775246 ) ) ;
#15813=CARTESIAN_POINT ( 'NONE',  ( -2.426309470044460959, 27.69042070294474556, -223.4541227565655674 ) ) ;
#15814=CARTESIAN_POINT ( 'NONE',  ( 11.67669251569587985, 24.04736029062789981, -218.5856804285192254 ) ) ;
#15815=CARTESIAN_POINT ( 'NONE',  ( 16.50235023187294203, -3.000022380394500310, -230.0447763498268614 ) ) ;
#15816=CARTESIAN_POINT ( 'NONE',  ( -24.15031621174628285, -13.05338392360020627, -219.0842748323915714 ) ) ;
#15817=CARTESIAN_POINT ( 'NONE',  ( -4.670971249126254499, -22.80666086768999890, -234.0323572959307512 ) ) ;
#15818=CARTESIAN_POINT ( 'NONE',  ( -2.426309470044460959, 27.69042070294474556, -223.4541227565655674 ) ) ;
#15820=CARTESIAN_POINT ( 'NONE',  ( 20.58393751692968721, 18.55948753678544705, -226.8933397075267635 ) ) ;
#15821=CARTESIAN_POINT ( 'NONE',  ( -18.39892766464214446, 25.11039525536027739, -225.3444503920457294 ) ) ;
#15822=CARTESIAN_POINT ( 'NONE',  ( -12.33997807949817904, 15.01940705987184188, -217.6798968600957380 ) ) ;
#15823=CARTESIAN_POINT ( 'NONE',  ( 3.312424284731937618, 15.29837714273186045, -229.5209971419123747 ) ) ;
#15824=CARTESIAN_POINT ( 'NONE',  ( -16.54465188417290022, 6.134005835925411709, -228.8256222654843270 ) ) ;
#15825=CARTESIAN_POINT ( 'NONE',  ( 28.77543668145700195, 2.466904630248945907, -219.6646827587300947 ) ) ;
#15826=CARTESIAN_POINT ( 'NONE',  ( 18.70674991763376482, -20.04093309878971496, -230.8534322170362714 ) ) ;
#15830=CARTESIAN_POINT ( 'NONE',  ( 4.730976410881341465, 17.65764351829336931, -217.6025626048331674 ) ) ;
#15831=CARTESIAN_POINT ( 'NONE',  ( 15.95205345792057550, -4.116367354408478896, -227.2937718740910498 ) ) ;
#15832=CARTESIAN_POINT ( 'NONE',  ( 16.06750045776299629, -1.909440863493336860, -220.4398626676318713 ) ) ;
#15833=CARTESIAN_POINT ( 'NONE',  ( 14.32085100525799248, 9.220655089380342062, -219.9006227404039464 ) ) ;
#15834=CARTESIAN_POINT ( 'NONE',  ( 6.166782020495575445, -26.61202787628535660, -217.6604608484729795 ) ) ;
#15836=CARTESIAN_POINT ( 'NONE',  ( -11.69688825528096388, 18.63404371591177622, -215.8612738028812714 ) ) ;
#15837=CARTESIAN_POINT ( 'NONE',  ( -12.30606003331388543, 10.59782772616791036, -231.0021630509705801 ) ) ;
#15839=CARTESIAN_POINT ( 'NONE',  ( -19.25929423112888017, 9.818144317380269825, -216.1837936240308409 ) ) ;
#15840=CARTESIAN_POINT ( 'NONE',  ( -24.09642229725868745, -17.04339013636034750, -228.1169379854252384 ) ) ;
#15843=CARTESIAN_POINT ( 'NONE',  ( -21.02719846458807851, 18.12262440796364871, -218.0220709499931502 ) ) ;
#15844=CARTESIAN_POINT ( 'NONE',  ( 7.434033643350927534, -13.76500825175950027, -228.7793665183827159 ) ) ;
#15847=CARTESIAN_POINT ( 'NONE',  ( 15.04029996350473830, 7.457450192165341107, -220.5007084872782173 ) ) ;
#15848=CARTESIAN_POINT ( 'NONE',  ( -6.079211283031130897, 16.94466709905296753, -232.9163774423793711 ) ) ;
#15850=CARTESIAN_POINT ( 'NONE',  ( 11.87550186346493497, 14.27797038184677270, -220.2068243228838185 ) ) ;
#15851=CARTESIAN_POINT ( 'NONE',  ( 3.303203443418958773, -15.45560242990989686, -230.9065799468681917 ) ) ;
#15853=CARTESIAN_POINT ( 'NONE',  ( -1.433739110790628102, 17.19322394474796667, -219.1420620387681879 ) ) ;
#15854=CARTESIAN_POINT ( 'NONE',  ( -18.64931821476190876, 22.04453097546810270, -226.2485927806324923 ) ) ;
#15855=CARTESIAN_POINT ( 'NONE',  ( -13.84508897751235246, 5.904954704487344941, -218.7722818424232401 ) ) ;
#15856=CARTESIAN_POINT ( 'NONE',  ( -15.48718561803335625, -8.207282836869444154, -229.3046138068065147 ) ) ;
#15859=CARTESIAN_POINT ( 'NONE',  ( 13.15438416660314225, 5.520603777723624539, -227.0878346348094681 ) ) ;
#15860=CARTESIAN_POINT ( 'NONE',  ( 1.312189596842585404, -27.84482500255423432, -221.0181370286903473 ) ) ;
#15861=CARTESIAN_POINT ( 'NONE',  ( 18.50911814746675788, 15.92944434255054453, -232.0449215596906072 ) ) ;
#15862=CARTESIAN_POINT ( 'NONE',  ( -23.98802705797876200, 19.46654170242919690, -223.5293093576406989 ) ) ;
#15863=CARTESIAN_POINT ( 'NONE',  ( 15.06072304412464291, 3.291435955319735651, -218.8606307204261725 ) ) ;
#15865=CARTESIAN_POINT ( 'NONE',  ( 1.382955251742491898, 16.46353944795171032, -231.7743150979565030 ) ) ;
#15867=CARTESIAN_POINT ( 'NONE',  ( -14.24095617957673632, -25.86326826095433162, -229.7068514753157160 ) ) ;
#15868=CARTESIAN_POINT ( 'NONE',  ( 11.31395536621571019, -8.070181239749643964, -225.0898076798974614 ) ) ;
#15871=CARTESIAN_POINT ( 'NONE',  ( -19.40752943788874774, 15.61499612050012864, -234.7624367253776541 ) ) ;
#15872=CARTESIAN_POINT ( 'NONE',  ( -19.42704602366333688, -5.151203963165301936, -219.4215732619585708 ) ) ;
#15874=CARTESIAN_POINT ( 'NONE',  ( -23.20103936322198024, 10.64725167743880085, -231.7714206262400864 ) ) ;
#15875=CARTESIAN_POINT ( 'NONE',  ( 1.104227501629593045, 25.05528885094460989, -231.9808705443460326 ) ) ;
#15876=CARTESIAN_POINT ( 'NONE',  ( -1.707778556226592581, 19.51307486516442680, -232.5708079709245055 ) ) ;
#15878=CARTESIAN_POINT ( 'NONE',  ( 13.14132348467506439, -13.49276336982165780, -234.5843434792288633 ) ) ;
#15880=CARTESIAN_POINT ( 'NONE',  ( 13.49011766416699842, 7.659170998773840111, -228.1905628957712793 ) ) ;
#15881=CARTESIAN_POINT ( 'NONE',  ( -18.70090456008720992, 23.36146401084868884, -220.3989740370807056 ) ) ;
#15882=CARTESIAN_POINT ( 'NONE',  ( -23.30382222616342247, 9.914163031146200566, -218.5285240371296425 ) ) ;
#15883=CARTESIAN_POINT ( 'NONE',  ( -14.28784611495131784, -7.281039336628973402, -230.6208668958216208 ) ) ;
#15884=CARTESIAN_POINT ( 'NONE',  ( -27.29953305526601426, 11.21644211419729054, -229.3676346105362995 ) ) ;
#15886=CARTESIAN_POINT ( 'NONE',  ( 22.42925200799500729, 5.652256920629083581, -234.0734181799116698 ) ) ;
#15888=CARTESIAN_POINT ( 'NONE',  ( -8.892156391762910062, 11.89593067802204551, -225.4519868197583889 ) ) ;
#15889=CARTESIAN_POINT ( 'NONE',  ( 25.17176037151762813, 18.95054595444721102, -221.3490360113488862 ) ) ;
#15890=CARTESIAN_POINT ( 'NONE',  ( -28.17543631911187063, 3.557555778861649642, -230.1980773687482156 ) ) ;
#15891=CARTESIAN_POINT ( 'NONE',  ( -14.65326448616001898, -2.737518208283025167, -217.6605647598149744 ) ) ;
#15893=CARTESIAN_POINT ( 'NONE',  ( -18.41550138691291139, -5.273244084890690075, -216.7348800533310964 ) ) ;
#15894=CARTESIAN_POINT ( 'NONE',  ( -1.238249567024760189, 29.30580384236933966, -223.2399636023643836 ) ) ;
#15895=CARTESIAN_POINT ( 'NONE',  ( -13.60146639818222702, -25.11808310587244009, -230.9974232610874196 ) ) ;
#15896=CARTESIAN_POINT ( 'NONE',  ( 12.10245006109274080, 26.02147364279441888, -220.6079829738538649 ) ) ;
#15897=CARTESIAN_POINT ( 'NONE',  ( 14.71544223636061410, -24.97731814513734605, -232.6985170686097320 ) ) ;
#15899=CARTESIAN_POINT ( 'NONE',  ( 25.30228294196351868, 7.987863777258004561, -233.0744943826964573 ) ) ;
#15902=CARTESIAN_POINT ( 'NONE',  ( -8.316066124693966444, 26.67103469786491843, -222.2304303634109885 ) ) ;
#15903=CARTESIAN_POINT ( 'NONE',  ( 29.01678366425524658, 8.126504218505314014, -229.6975090854573125 ) ) ;
#15905=CARTESIAN_POINT ( 'NONE',  ( 28.02123297569005089, 5.903198806000402143, -227.5759114383273811 ) ) ;
#15906=CARTESIAN_POINT ( 'NONE',  ( -24.15814485343234352, 4.373587128574028426, -232.6698675874553430 ) ) ;
#15907=CARTESIAN_POINT ( 'NONE',  ( -12.55242351043508542, -12.71283815946331686, -230.7436264644880737 ) ) ;
#15908=CARTESIAN_POINT ( 'NONE',  ( 11.20713200305815427, 28.28922876448651635, -219.1239564724620834 ) ) ;
#15910=CARTESIAN_POINT ( 'NONE',  ( -8.649444225544010934, -13.15555178350489918, -216.8547715670961509 ) ) ;
#15911=CARTESIAN_POINT ( 'NONE',  ( -4.784012432433236484, 23.31984772163034947, -232.0554186943449508 ) ) ;
#15913=CARTESIAN_POINT ( 'NONE',  ( 6.771176146757415637, 15.60014285904435027, -218.3493856697694753 ) ) ;
#15915=CARTESIAN_POINT ( 'NONE',  ( -12.04619960554013502, 10.22290173510000777, -223.1766370265664534 ) ) ;
#15916=CARTESIAN_POINT ( 'NONE',  ( -4.424820997438546399, 11.84746159238278373, -221.7815792475208525 ) ) ;
#15917=CARTESIAN_POINT ( 'NONE',  ( 15.07212457412616224, 2.472408313530222390, -227.3472192494155024 ) ) ;
#15918=CARTESIAN_POINT ( 'NONE',  ( 13.51502823286059929, -13.46037062290453790, -230.3041566501836144 ) ) ;
#15920=CARTESIAN_POINT ( 'NONE',  ( 11.64632602964496044, -20.35392056169815689, -232.5450580586399383 ) ) ;
#15921=CARTESIAN_POINT ( 'NONE',  ( -3.139695637132168038, 25.12735071829084177, -230.1469660918596389 ) ) ;
#15923=CARTESIAN_POINT ( 'NONE',  ( 18.29617186523616468, 23.20920553663278341, -223.4372550713720216 ) ) ;
#15924=CARTESIAN_POINT ( 'NONE',  ( 15.05575868828727515, -2.428864548505686560, -227.9368649688638584 ) ) ;
#15925=CARTESIAN_POINT ( 'NONE',  ( -13.33530847390368024, -5.065163879519744228, -226.5386329521395226 ) ) ;
#15926=CARTESIAN_POINT ( 'NONE',  ( -1.890995374385051608, -13.09686096954197509, -227.5694739903412085 ) ) ;
#15927=CARTESIAN_POINT ( 'NONE',  ( 1.296323513242173542, 20.09034598902932345, -230.5712631353794961 ) ) ;
#15929=CARTESIAN_POINT ( 'NONE',  ( 14.37653162493774239, 9.985418694807894013, -229.1686718965858063 ) ) ;
#15931=CARTESIAN_POINT ( 'NONE',  ( -10.51143808951550085, 11.41308718311005066, -231.3573069600382439 ) ) ;
#15932=CARTESIAN_POINT ( 'NONE',  ( -15.33438615632468149, 23.56248205204123991, -229.2747191038674544 ) ) ;
#15936=CARTESIAN_POINT ( 'NONE',  ( 6.566035546683759883, 15.06745272174450712, -218.8330720708048034 ) ) ;
#15937=CARTESIAN_POINT ( 'NONE',  ( -22.90687623753526125, 9.466200233939549236, -230.1557007022273638 ) ) ;
#15938=CARTESIAN_POINT ( 'NONE',  ( 25.09997929702755926, 1.294103573351435221, -217.0485712200477906 ) ) ;
#15939=CARTESIAN_POINT ( 'NONE',  ( 6.679827377097204533, -23.59744646493245668, -231.8618301756397670 ) ) ;
#15941=CARTESIAN_POINT ( 'NONE',  ( 10.02513374692848913, 18.81568788741115128, -217.1505009242214612 ) ) ;
#15942=CARTESIAN_POINT ( 'NONE',  ( 20.39962514764921409, -3.647888038500222141, -219.1338420190236036 ) ) ;
#15943=CARTESIAN_POINT ( 'NONE',  ( 23.12216041205843453, 0.2121350054995089496, -232.0572713672589202 ) ) ;
#15944=CARTESIAN_POINT ( 'NONE',  ( 8.115778909262310492, -29.92983049028717346, -224.5060555478150377 ) ) ;
#15945=CARTESIAN_POINT ( 'NONE',  ( -22.99617382825321599, 17.18101613848176967, -230.9512687019100099 ) ) ;
#15947=CARTESIAN_POINT ( 'NONE',  ( -13.48133478602219171, 10.24771958306113362, -218.3822527490931691 ) ) ;
#15949=CARTESIAN_POINT ( 'NONE',  ( 21.19180206786061405, -1.472355559550188264, -231.3901500139509722 ) ) ;
#15950=CARTESIAN_POINT ( 'NONE',  ( -24.60063047153272819, -17.11178239752603858, -226.7032704813509554 ) ) ;
#15953=CARTESIAN_POINT ( 'NONE',  ( 16.07305932912010960, 0.9253679043337685872, -229.0409936706996064 ) ) ;
#15954=CARTESIAN_POINT ( 'NONE',  ( -12.78558550453068854, 7.693178343823584342, -230.0800953344970878 ) ) ;
#15955=CARTESIAN_POINT ( 'NONE',  ( 8.168748216644726057, -13.67612414567523693, -220.8005964828080607 ) ) ;
#15958=CARTESIAN_POINT ( 'NONE',  ( 27.66944030902029539, 6.857614156517904291, -220.9860880211026313 ) ) ;
#15959=CARTESIAN_POINT ( 'NONE',  ( -8.523771322135640816, 24.09653697920728987, -233.1071395647740303 ) ) ;
#15961=CARTESIAN_POINT ( 'NONE',  ( 17.51175949430614409, 14.31829016556564937, -218.8195841045835550 ) ) ;
#15962=CARTESIAN_POINT ( 'NONE',  ( 4.683166109028750412, -21.42534054955530110, -233.6038185840237986 ) ) ;
#15964=CARTESIAN_POINT ( 'NONE',  ( 0.3632086708616291126, 21.06287758167331958, -232.5112839711303820 ) ) ;
#15965=CARTESIAN_POINT ( 'NONE',  ( -12.66290653391502907, 23.44312233264792411, -230.9359094203250606 ) ) ;
#15966=CARTESIAN_POINT ( 'NONE',  ( -11.78887577478644566, 1.715692547334320084, -224.3106172711415525 ) ) ;
#15967=CARTESIAN_POINT ( 'NONE',  ( -9.995627826723184839, -14.18420632236771439, -221.4333122433492633 ) ) ;
#15969=AXIS2_PLACEMENT_3D ( 'NONE', #20462, #18686, #1579 ) ;
#15971=CARTESIAN_POINT ( 'NONE',  ( -26.58771759052039485, 5.114955214121561511, -218.2823714869195442 ) ) ;
#15972=CARTESIAN_POINT ( 'NONE',  ( 3.112457940538468470, -21.91845672593830940, -231.6743386618371403 ) ) ;
#15973=CARTESIAN_POINT ( 'NONE',  ( 16.54345861550681107, 19.37554510112122230, -218.2240151908141002 ) ) ;
#15974=CARTESIAN_POINT ( 'NONE',  ( 4.730976410881341465, 17.65764351829336931, -217.6025626048331674 ) ) ;
#15975=CARTESIAN_POINT ( 'NONE',  ( -15.72195651633673208, 2.938252489821347346, -222.2698596109374023 ) ) ;
#15976=CARTESIAN_POINT ( 'NONE',  ( 3.763426558366607111, 28.60172112197566818, -230.1816715025297526 ) ) ;
#15978=CARTESIAN_POINT ( 'NONE',  ( -9.078153229956912540, -10.71731945587431056, -228.5228069477245469 ) ) ;
#15979=CARTESIAN_POINT ( 'NONE',  ( 24.96294718070021901, -13.86220829677249178, -229.4442241490162075 ) ) ;
#15982=CARTESIAN_POINT ( 'NONE',  ( -9.722597143579921664, 7.159547510896417499, -227.5730737101346222 ) ) ;
#15983=CARTESIAN_POINT ( 'NONE',  ( -22.11234321210701737, -3.359691084028018526, -230.9311713419302521 ) ) ;
#15984=CARTESIAN_POINT ( 'NONE',  ( -20.47640197314466093, 18.50423766437512541, -220.4440130802851456 ) ) ;
#15985=CARTESIAN_POINT ( 'NONE',  ( 15.26539804565921621, 9.309431686815628382, -232.9129599938668207 ) ) ;
#15986=CARTESIAN_POINT ( 'NONE',  ( -4.211886032913159106, 20.62037006687756602, -216.9488349035050305 ) ) ;
#15987=ORIENTED_EDGE ( 'NONE', *, *, #70, .T. ) ;
#15988=CARTESIAN_POINT ( 'NONE',  ( 7.820185266007354308, -13.10000580370673440, -218.6580452893993254 ) ) ;
#15990=CARTESIAN_POINT ( 'NONE',  ( 17.34727976380017722, 4.822939981779328811, -230.8836217450937909 ) ) ;
#15992=CARTESIAN_POINT ( 'NONE',  ( -4.378220565073127624, 31.53459173284372952, -222.0564199190954753 ) ) ;
#15993=CARTESIAN_POINT ( 'NONE',  ( -4.296082356836364191, 12.57880442405704002, -229.5247240216588125 ) ) ;
#15994=CARTESIAN_POINT ( 'NONE',  ( -12.22852564478610482, -7.025360622849957437, -222.3415469712626589 ) ) ;
#15995=CARTESIAN_POINT ( 'NONE',  ( -21.02719846458807851, 18.12262440796364871, -218.0220709499931502 ) ) ;
#15997=CARTESIAN_POINT ( 'NONE',  ( 15.13105790938820228, -1.902449014147146178, -222.1588331224812407 ) ) ;
#15999=CARTESIAN_POINT ( 'NONE',  ( -12.15411956849120756, 11.21601165624538687, -228.1895064089065670 ) ) ;
#16001=CARTESIAN_POINT ( 'NONE',  ( 20.09685469220202236, -2.033783885649083079, -233.1448060988079760 ) ) ;
#16002=CARTESIAN_POINT ( 'NONE',  ( -13.69675006931110417, 3.702342960760605539, -228.0723273272095355 ) ) ;
#16003=CARTESIAN_POINT ( 'NONE',  ( 11.67669251569587985, 24.04736029062789981, -218.5856804285192254 ) ) ;
#16004=CARTESIAN_POINT ( 'NONE',  ( -14.33274213004767716, -3.240524307521291725, -229.5155949954044559 ) ) ;
#16005=CARTESIAN_POINT ( 'NONE',  ( 1.719513778997906694, 15.52930330544231730, -222.3959083836286368 ) ) ;
#16006=CARTESIAN_POINT ( 'NONE',  ( -5.902479482706956659, -14.78727544128710214, -218.5565286504736946 ) ) ;
#16007=CARTESIAN_POINT ( 'NONE',  ( 5.248230734842167955, 23.54336384919183445, -216.8914391693808739 ) ) ;
#16008=CARTESIAN_POINT ( 'NONE',  ( 15.50373320885645079, -27.90820408561472732, -228.0623419774833280 ) ) ;
#16009=CARTESIAN_POINT ( 'NONE',  ( -24.25245498015852874, 0.2109992039763788352, -218.1398602137601301 ) ) ;
#16010=CARTESIAN_POINT ( 'NONE',  ( -11.05032764129755840, 11.65053160594169945, -221.1796278216217218 ) ) ;
#16011=( LENGTH_UNIT ( ) NAMED_UNIT ( * ) SI_UNIT ( .MILLI., .METRE. ) );
#16012=CARTESIAN_POINT ( 'NONE',  ( 20.28526114930425450, -5.837089636085359245, -233.7994602772149051 ) ) ;
#16013=CARTESIAN_POINT ( 'NONE',  ( 9.253909228257674258, 17.69332415812615977, -230.9900471521432621 ) ) ;
#16014=CARTESIAN_POINT ( 'NONE',  ( -14.57944476639264764, 6.129437248167259433, -229.4766146696829310 ) ) ;
#16015=CARTESIAN_POINT ( 'NONE',  ( 15.52719855059926424, 1.633696074270991172, -221.7349885876216433 ) ) ;
#16016=CARTESIAN_POINT ( 'NONE',  ( -7.732225105831920686, -12.76821222370703346, -228.2562058524068220 ) ) ;
#16019=CARTESIAN_POINT ( 'NONE',  ( 8.681721411120292942, 8.442847255497570202, -228.0516816418615065 ) ) ;
#16021=CARTESIAN_POINT ( 'NONE',  ( -4.907461209876205821, -14.28794023480369368, -232.2749568027591636 ) ) ;
#16022=CARTESIAN_POINT ( 'NONE',  ( 3.080453011304693511, 29.32691491905673331, -222.8956499783474499 ) ) ;
#16023=CARTESIAN_POINT ( 'NONE',  ( 8.379126514044342500, 15.76264856365358646, -232.1787896114811360 ) ) ;
#16024=CARTESIAN_POINT ( 'NONE',  ( -17.99155049254074612, 5.190958499132906745, -220.1449419322306937 ) ) ;
#16026=CARTESIAN_POINT ( 'NONE',  ( -5.340143745732740754, 22.10628181454592678, -235.0476201740528097 ) ) ;
#16027=CARTESIAN_POINT ( 'NONE',  ( 14.92135368508905202, 7.451356898669101447, -219.1823315336843621 ) ) ;
#16029=CARTESIAN_POINT ( 'NONE',  ( 18.69764316139794147, -20.69319383826335823, -224.5905439953889413 ) ) ;
#16031=CARTESIAN_POINT ( 'NONE',  ( 8.158223302632384488, -13.44420475212243993, -229.3230086144918403 ) ) ;
#16033=CARTESIAN_POINT ( 'NONE',  ( -8.115738378024497379, 16.90402287339461296, -219.0833473190803034 ) ) ;
#16036=CARTESIAN_POINT ( 'NONE',  ( 14.95414693437772868, 8.262206471704862665, -230.1862972580043163 ) ) ;
#16037=CARTESIAN_POINT ( 'NONE',  ( -20.69232116990083981, -0.6602618815637216754, -233.8806059993499957 ) ) ;
#16038=CARTESIAN_POINT ( 'NONE',  ( -13.22951852716680676, -5.246159916193459338, -223.7538483380451453 ) ) ;
#16039=CARTESIAN_POINT ( 'NONE',  ( 1.799766247726228174, -14.75051420185460849, -230.6199496058247291 ) ) ;
#16040=CARTESIAN_POINT ( 'NONE',  ( 3.241594727517011609, 27.64703009302456138, -225.5540025036233374 ) ) ;
#16042=CARTESIAN_POINT ( 'NONE',  ( -20.49711526797010208, 7.006997077916217620, -215.3369776077118445 ) ) ;
#16043=CARTESIAN_POINT ( 'NONE',  ( -4.620781219515533778, 16.99182040716223696, -217.1278208835672672 ) ) ;
#16044=CARTESIAN_POINT ( 'NONE',  ( 3.388180927852674884, 15.71154068801650538, -224.9339660840813053 ) ) ;
#16046=CARTESIAN_POINT ( 'NONE',  ( -1.975202609796049336, 20.81351768191813889, -217.5779402428482001 ) ) ;
#16047=CARTESIAN_POINT ( 'NONE',  ( -22.10934047915413814, 0.9940043559354462266, -218.9999999999999716 ) ) ;
#16048=CARTESIAN_POINT ( 'NONE',  ( 16.22460398937575121, -0.7285105026664867589, -219.3274985887512116 ) ) ;
#16049=CARTESIAN_POINT ( 'NONE',  ( 13.65368867897269389, -25.84127502057983605, -227.3223880387346867 ) ) ;
#16052=CARTESIAN_POINT ( 'NONE',  ( 21.96352831578809273, -0.3315607655629317918, -233.9427286327412503 ) ) ;
#16053=CARTESIAN_POINT ( 'NONE',  ( 12.53674998645855787, 17.96979015029927851, -232.8843215672231679 ) ) ;
#16054=CARTESIAN_POINT ( 'NONE',  ( 15.67226265972355392, -3.922905252720024105, -226.2579514984929858 ) ) ;
#16055=CARTESIAN_POINT ( 'NONE',  ( 26.16486877413895584, -0.2437668799822691745, -230.8325409000573814 ) ) ;
#16057=CARTESIAN_POINT ( 'NONE',  ( 4.682724365302521896, -22.35092628325669750, -215.9543778044225348 ) ) ;
#16060=CARTESIAN_POINT ( 'NONE',  ( -23.52999999174766543, 19.39566142560855866, -221.9446938626390704 ) ) ;
#16061=CARTESIAN_POINT ( 'NONE',  ( -19.90771709537278156, 23.83218599423810602, -225.0439263757368735 ) ) ;
#16063=CARTESIAN_POINT ( 'NONE',  ( -23.98802705797876200, 19.46654170242919690, -223.5293093576406989 ) ) ;
#16064=CARTESIAN_POINT ( 'NONE',  ( -17.90134810484358141, -14.13951559615540710, -232.9640066987647344 ) ) ;
#16066=CARTESIAN_POINT ( 'NONE',  ( -9.151299407007059017, 9.196974979111923076, -223.9483834032048719 ) ) ;
#16067=CARTESIAN_POINT ( 'NONE',  ( 3.692943796146577196, -17.43777048755501724, -232.3481250940208156 ) ) ;
#16069=CARTESIAN_POINT ( 'NONE',  ( -11.98736441306973077, 11.45674391201457176, -217.8252237716743025 ) ) ;
#16070=CARTESIAN_POINT ( 'NONE',  ( 19.31922195716811430, 9.600631919686000160, -218.1359845693048101 ) ) ;
#16071=CARTESIAN_POINT ( 'NONE',  ( -11.87391433320165746, 8.920676825367966245, -232.2044275666449096 ) ) ;
#16073=CARTESIAN_POINT ( 'NONE',  ( -16.40095417437164471, 2.582410108382750646, -233.5151473761628154 ) ) ;
#16074=CARTESIAN_POINT ( 'NONE',  ( -10.27880337231260199, -13.06498408352235430, -227.3766186522184682 ) ) ;
#16076=CARTESIAN_POINT ( 'NONE',  ( -9.810154340578240095, 25.84808829058669488, -220.5759521898573610 ) ) ;
#16078=CARTESIAN_POINT ( 'NONE',  ( -17.07311071032027172, 18.59516984069744794, -230.9440421721702137 ) ) ;
#16079=CARTESIAN_POINT ( 'NONE',  ( -12.27164519775873686, 10.97713184439464840, -231.6269036897678291 ) ) ;
#16080=CARTESIAN_POINT ( 'NONE',  ( -9.780669591740702273, -13.62818526938769104, -222.3368934028275135 ) ) ;
#16083=CARTESIAN_POINT ( 'NONE',  ( 16.40130693394614525, -0.1574073183566240264, -221.9481963320051534 ) ) ;
#16084=CARTESIAN_POINT ( 'NONE',  ( 0.6118723529980315545, -20.11903950562274446, -217.9558718073025716 ) ) ;
#16085=CARTESIAN_POINT ( 'NONE',  ( 22.86997486125673618, 17.56009411325475966, -222.3578648042903296 ) ) ;
#16086=CARTESIAN_POINT ( 'NONE',  ( 5.017623471397871349, 29.83561274492976878, -222.9769172135417250 ) ) ;
#16087=CARTESIAN_POINT ( 'NONE',  ( -25.11055959288653128, 8.701823109978603199, -230.2231080656787583 ) ) ;
#16088=CARTESIAN_POINT ( 'NONE',  ( 12.99334571784053338, 27.47142594410712846, -219.5003755906066658 ) ) ;
#16089=CARTESIAN_POINT ( 'NONE',  ( 15.33737796850231305, 13.57479350230705428, -232.3313557812109025 ) ) ;
#16090=CARTESIAN_POINT ( 'NONE',  ( 14.58114346306845377, 2.033664520579581581, -222.7937709467664149 ) ) ;
#16091=CARTESIAN_POINT ( 'NONE',  ( -5.525229149912007642, -13.32411127922494742, -220.4018445532201440 ) ) ;
#16092=CARTESIAN_POINT ( 'NONE',  ( 4.201723131641114328, -20.76291977712905279, -215.9522215885928347 ) ) ;
#16095=CARTESIAN_POINT ( 'NONE',  ( -16.95112677453439431, 10.32962960657076934, -214.9445123409346650 ) ) ;
#16096=CARTESIAN_POINT ( 'NONE',  ( -18.83136555461844708, -9.493528738360442532, -219.1308048892593945 ) ) ;
#16097=CARTESIAN_POINT ( 'NONE',  ( -15.82622499106666325, 9.895986579907866343, -218.5115209877527604 ) ) ;
#16098=CARTESIAN_POINT ( 'NONE',  ( 9.798337081649805214, 12.27506320122302697, -218.9346733583377613 ) ) ;
#16099=CARTESIAN_POINT ( 'NONE',  ( 7.951191770265756631, 20.55701948568933091, -231.2149185317973661 ) ) ;
#16101=CARTESIAN_POINT ( 'NONE',  ( 19.66172111867919270, -11.21951684559458506, -235.3531537740016972 ) ) ;
#16102=CARTESIAN_POINT ( 'NONE',  ( 14.54149994592679107, 8.070685273005897997, -229.7292930672863349 ) ) ;
#16103=CARTESIAN_POINT ( 'NONE',  ( -11.59874896804548250, 27.28969409813203484, -218.8626241359735332 ) ) ;
#16104=CARTESIAN_POINT ( 'NONE',  ( -12.39195900010699702, 23.13258866008456138, -233.4668451572263166 ) ) ;
#16105=CARTESIAN_POINT ( 'NONE',  ( -17.60306105620566441, -10.62493847279374926, -216.8163279515337649 ) ) ;
#16106=CARTESIAN_POINT ( 'NONE',  ( -11.49049084071896409, 11.06834963248926940, -218.3354249205727058 ) ) ;
#16108=CARTESIAN_POINT ( 'NONE',  ( 20.15756451863428111, -2.090604891399794774, -217.8900786001194945 ) ) ;
#16109=CARTESIAN_POINT ( 'NONE',  ( 1.773237071419721422, 13.09828209437875302, -220.6531024550077404 ) ) ;
#16110=CARTESIAN_POINT ( 'NONE',  ( -21.89065952084834166, -0.9940043559354216907, -218.9999999999999716 ) ) ;
#16111=CARTESIAN_POINT ( 'NONE',  ( -25.80904414196669450, 12.19501778665756220, -219.1732313092283846 ) ) ;
#16112=CARTESIAN_POINT ( 'NONE',  ( 4.559463107227270662, 13.27337529356814017, -226.9596205199204633 ) ) ;
#16114=CARTESIAN_POINT ( 'NONE',  ( -1.248802714212398968, 14.93471382136348602, -228.4293827518713158 ) ) ;
#16115=CARTESIAN_POINT ( 'NONE',  ( -15.19144047750087267, -10.24270553329939304, -232.4311702607364793 ) ) ;
#16116=CARTESIAN_POINT ( 'NONE',  ( 11.82943521288609823, 27.58963564415041247, -226.1180395413371400 ) ) ;
#16117=CARTESIAN_POINT ( 'NONE',  ( 20.49803729918260942, -22.47924998572259980, -218.9346008044765028 ) ) ;
#16119=CARTESIAN_POINT ( 'NONE',  ( -13.93825237094548619, 9.044872709574327985, -220.1275804576921757 ) ) ;
#16120=CARTESIAN_POINT ( 'NONE',  ( 12.94117841657163126, -3.283311917827119064, -226.8844617769393039 ) ) ;
#16121=CARTESIAN_POINT ( 'NONE',  ( 14.96080648943632241, 22.28365808184747721, -220.1237743409445216 ) ) ;
#16122=CARTESIAN_POINT ( 'NONE',  ( -19.74163224554151697, 8.726897413558679872, -232.6665747339030190 ) ) ;
#16123=CARTESIAN_POINT ( 'NONE',  ( 28.57344184061583192, 5.631897254180425527, -225.1192013637692355 ) ) ;
#16125=CARTESIAN_POINT ( 'NONE',  ( -15.97267037792306255, -23.58045393237649279, -221.6247985403941527 ) ) ;
#16126=CARTESIAN_POINT ( 'NONE',  ( 21.77779027533950540, 18.43917590911969029, -232.9503911151153659 ) ) ;
#16128=CARTESIAN_POINT ( 'NONE',  ( -27.27535713358387781, -16.47971293676793181, -227.4585470903502653 ) ) ;
#16129=CARTESIAN_POINT ( 'NONE',  ( 1.104227501629593045, 25.05528885094460989, -231.9808705443460326 ) ) ;
#16130=CARTESIAN_POINT ( 'NONE',  ( 15.96089671440110713, 1.143943728337336374, -218.3532651118343892 ) ) ;
#16131=CARTESIAN_POINT ( 'NONE',  ( -9.969679877803788060, 12.84542071557917176, -220.4758784541224657 ) ) ;
#16133=CARTESIAN_POINT ( 'NONE',  ( -8.123851230256436295, 20.56863949923577550, -215.0796075421103239 ) ) ;
#16134=CARTESIAN_POINT ( 'NONE',  ( -18.71530386740073126, -0.6857509888707814527, -217.6195632122020527 ) ) ;
#16136=CARTESIAN_POINT ( 'NONE',  ( -2.392195434554431177, -23.29395655963766387, -232.4094703796048691 ) ) ;
#16138=CARTESIAN_POINT ( 'NONE',  ( 8.339826811406878093, -13.81198187275966660, -229.8741491687588621 ) ) ;
#16140=CARTESIAN_POINT ( 'NONE',  ( 15.61962121506769385, 4.525360868525488911, -229.0684696061408090 ) ) ;
#16141=CARTESIAN_POINT ( 'NONE',  ( -13.00301829581513857, -0.4478114825397079279, -224.9470972339195214 ) ) ;
#16142=CARTESIAN_POINT ( 'NONE',  ( -18.53787071664277519, -6.556543064843903146, -232.5192140591401824 ) ) ;
#16143=CARTESIAN_POINT ( 'NONE',  ( 8.532614294830283441, -28.73326933124977955, -229.1610356131385231 ) ) ;
#16144=CARTESIAN_POINT ( 'NONE',  ( 3.433394806375676733, 19.92272173529517332, -219.3341428536850799 ) ) ;
#16146=CARTESIAN_POINT ( 'NONE',  ( -29.50764134580612463, 7.783340782857166573, -219.9768238800827191 ) ) ;
#16147=CARTESIAN_POINT ( 'NONE',  ( -8.966714183099560032, 19.05224306381768073, -234.0879867025980445 ) ) ;
#16148=CARTESIAN_POINT ( 'NONE',  ( 3.433394806375676733, 19.92272173529517332, -219.3341428536850799 ) ) ;
#16149=CARTESIAN_POINT ( 'NONE',  ( 12.70896864779121316, -3.955665148817821386, -221.1719243096075900 ) ) ;
#16152=CARTESIAN_POINT ( 'NONE',  ( 9.211411085256067111, 16.86455563410128633, -232.8411836211112700 ) ) ;
#16153=CARTESIAN_POINT ( 'NONE',  ( -18.02718827071834085, 20.33515877052379395, -229.5060669840136143 ) ) ;
#16154=CARTESIAN_POINT ( 'NONE',  ( 17.72360441613731652, -1.822637811265336749, -232.2813868768326984 ) ) ;
#16156=CARTESIAN_POINT ( 'NONE',  ( -5.218961787268129093, -16.18493974670746027, -219.8229902141834771 ) ) ;
#16159=CARTESIAN_POINT ( 'NONE',  ( 8.979547488457603421, 23.24376652602565230, -232.6628827740196357 ) ) ;
#16160=CARTESIAN_POINT ( 'NONE',  ( 13.39501375133567329, -10.34300172232987691, -228.1452887455185987 ) ) ;
#16162=CARTESIAN_POINT ( 'NONE',  ( 6.260999666360449467, -13.19315344885661645, -220.2890618333529744 ) ) ;
#16164=CARTESIAN_POINT ( 'NONE',  ( 3.449504654906655254, 27.59247159270940841, -231.3461799890608859 ) ) ;
#16165=CARTESIAN_POINT ( 'NONE',  ( -23.89856910807799295, 17.42297078648622843, -222.0178620725767757 ) ) ;
#16167=CARTESIAN_POINT ( 'NONE',  ( -13.83274569775339202, 16.20364235096346661, -234.0851861771356539 ) ) ;
#16168=CARTESIAN_POINT ( 'NONE',  ( -17.81508947870519322, -18.77243306401324219, -218.1930932538018340 ) ) ;
#16171=CARTESIAN_POINT ( 'NONE',  ( -7.189383125363055349, 14.28512618638020548, -231.7475838278701303 ) ) ;
#16172=CARTESIAN_POINT ( 'NONE',  ( 8.625046000483031605, -27.40455649025574303, -220.2318935480384710 ) ) ;
#16174=CARTESIAN_POINT ( 'NONE',  ( -23.98802705797876200, 19.46654170242919690, -223.5293093576406989 ) ) ;
#16175=CARTESIAN_POINT ( 'NONE',  ( -22.28357709049062407, 7.264818440526320309, -215.3877468064711707 ) ) ;
#16176=CARTESIAN_POINT ( 'NONE',  ( -1.238249567024760189, 29.30580384236933966, -223.2399636023643836 ) ) ;
#16178=CARTESIAN_POINT ( 'NONE',  ( 14.68130101653174613, 6.427210486143660084, -228.0153742661088074 ) ) ;
#16179=CARTESIAN_POINT ( 'NONE',  ( -10.61621529918308227, -15.65610094335291969, -220.0975530242428420 ) ) ;
#16181=CARTESIAN_POINT ( 'NONE',  ( 9.211411085256067111, 16.86455563410128633, -232.8411836211112700 ) ) ;
#16182=CARTESIAN_POINT ( 'NONE',  ( -12.69709334397052203, 10.59859500067950400, -221.6107941937004568 ) ) ;
#16183=CARTESIAN_POINT ( 'NONE',  ( -13.71158422780231056, 12.21432067443984693, -232.9166272955793033 ) ) ;
#16184=CARTESIAN_POINT ( 'NONE',  ( -18.52912398332900068, -6.554396152115366192, -218.2980051671528088 ) ) ;
#16187=CARTESIAN_POINT ( 'NONE',  ( -15.15434969228324924, 4.423874646950748613, -230.6144467931089821 ) ) ;
#16188=CARTESIAN_POINT ( 'NONE',  ( 4.239709385547987708, -16.34504625405869405, -220.9645569933060756 ) ) ;
#16189=CARTESIAN_POINT ( 'NONE',  ( 15.57223476564572984, 1.638033498045565306, -221.8258985305325268 ) ) ;
#16190=CARTESIAN_POINT ( 'NONE',  ( 3.449504654906655254, 27.59247159270940841, -231.3461799890608859 ) ) ;
#16192=CARTESIAN_POINT ( 'NONE',  ( -22.14646582578067679, 6.967411055428133437, -231.6932229095398270 ) ) ;
#16193=CARTESIAN_POINT ( 'NONE',  ( 16.71272566993619080, 8.989703107375911273, -217.4612081447889125 ) ) ;
#16194=CARTESIAN_POINT ( 'NONE',  ( 10.78187269046063435, 10.73871010366167944, -221.9206544238666368 ) ) ;
#16196=CARTESIAN_POINT ( 'NONE',  ( -5.636842872076440081, -13.76003991320737541, -219.7405193562604495 ) ) ;
#16197=CARTESIAN_POINT ( 'NONE',  ( 1.799766247726228174, -14.75051420185460849, -230.6199496058247291 ) ) ;
#16200=CARTESIAN_POINT ( 'NONE',  ( -5.607934827417612844, 15.68271927908880770, -232.1026723719274969 ) ) ;
#16201=CARTESIAN_POINT ( 'NONE',  ( 20.57969228301723419, -8.207465571703625784, -214.6085555290863454 ) ) ;
#16202=CARTESIAN_POINT ( 'NONE',  ( 24.56541673123750158, -5.996287403333383281, -231.6940117905984664 ) ) ;
#16203=CARTESIAN_POINT ( 'NONE',  ( 12.74913679152205148, 9.185760885856177893, -218.6542381594888980 ) ) ;
#16204=CARTESIAN_POINT ( 'NONE',  ( 8.539351012053531420, 16.03230746435535181, -220.6282946404833751 ) ) ;
#16207=CARTESIAN_POINT ( 'NONE',  ( 20.77649313750695370, -15.65279155457156435, -215.5859610257211898 ) ) ;
#16209=CARTESIAN_POINT ( 'NONE',  ( 4.065638640983322283, 32.08830473489500434, -226.0249194102539150 ) ) ;
#16210=CARTESIAN_POINT ( 'NONE',  ( -5.373457274256926652, 30.83572167890261184, -229.2199105909169532 ) ) ;
#16211=CARTESIAN_POINT ( 'NONE',  ( -19.98462433625633494, -12.30084073857678639, -216.8518508258974862 ) ) ;
#16212=CARTESIAN_POINT ( 'NONE',  ( -22.99617382825321599, 17.18101613848176967, -230.9512687019100099 ) ) ;
#16214=CARTESIAN_POINT ( 'NONE',  ( 20.89700225552940793, -4.547446057044195911, -232.3806459760843666 ) ) ;
#16215=CARTESIAN_POINT ( 'NONE',  ( 2.892356176081334773, 24.03953794589038395, -215.3901262983647200 ) ) ;
#16216=CARTESIAN_POINT ( 'NONE',  ( 16.67941620816951698, 4.093285459228785506, -217.1675623234529269 ) ) ;
#16217=CARTESIAN_POINT ( 'NONE',  ( -9.443239614166923701, 9.388015667058336788, -222.3195230688234290 ) ) ;
#16218=CARTESIAN_POINT ( 'NONE',  ( 20.41153371889344825, 17.18812948447019551, -230.7531656956970778 ) ) ;
#16220=CARTESIAN_POINT ( 'NONE',  ( 5.104697752190542559, 17.18208638613223016, -220.3923334988619445 ) ) ;
#16221=CARTESIAN_POINT ( 'NONE',  ( -12.04756914620937636, -13.80987496524771885, -232.8991007102355582 ) ) ;
#16222=CARTESIAN_POINT ( 'NONE',  ( 13.03557269046774714, 7.519834803053426775, -226.9490612297269081 ) ) ;
#16223=CARTESIAN_POINT ( 'NONE',  ( -2.619247311076123630, -29.90652300472198988, -220.3405913430138128 ) ) ;
#16225=CARTESIAN_POINT ( 'NONE',  ( -16.28025842329327944, 6.985656672962045732, -231.4191468057695715 ) ) ;
#16226=DIRECTION ( 'NONE',  ( 0.000000000000000000, 0.000000000000000000, 1.000000000000000000 ) ) ;
#16227=CARTESIAN_POINT ( 'NONE',  ( -29.37537067777813604, -4.151788015186005154, -225.5750753894876368 ) ) ;
#16228=CARTESIAN_POINT ( 'NONE',  ( 3.174664235197445006, 17.30896320251298448, -221.0803896709622620 ) ) ;
#16229=CARTESIAN_POINT ( 'NONE',  ( -11.05032764129755840, 11.65053160594169945, -221.1796278216217218 ) ) ;
#16230=CARTESIAN_POINT ( 'NONE',  ( -14.63872435137796302, 9.306825831109410530, -216.0000338566471214 ) ) ;
#16231=CARTESIAN_POINT ( 'NONE',  ( -7.928105003701093167, -26.09134507487772225, -231.8683635223868578 ) ) ;
#16232=CARTESIAN_POINT ( 'NONE',  ( 13.12946830070648652, 6.370976456471619365, -231.5124810213676483 ) ) ;
#16234=CARTESIAN_POINT ( 'NONE',  ( -13.68978490692228256, -5.239663260684684687, -218.7416303080107411 ) ) ;
#16235=CARTESIAN_POINT ( 'NONE',  ( -3.223980134944351317, 26.83284996841001302, -219.5167893230652965 ) ) ;
#16236=CARTESIAN_POINT ( 'NONE',  ( 21.72366288329714834, 2.385777479048636351, -215.9150265590827757 ) ) ;
#16237=CARTESIAN_POINT ( 'NONE',  ( -7.266348978356541366, 16.38312187400933340, -217.9429203627011873 ) ) ;
#16238=CARTESIAN_POINT ( 'NONE',  ( 3.764125772070460396, 11.78312483992801596, -228.3484643988637970 ) ) ;
#16240=CARTESIAN_POINT ( 'NONE',  ( 1.312189596842585404, -27.84482500255423432, -221.0181370286903473 ) ) ;
#16242=CARTESIAN_POINT ( 'NONE',  ( -1.615718423935818437, -15.01490656935555812, -223.2481059054151729 ) ) ;
#16244=AXIS2_PLACEMENT_3D ( 'NONE', #5290, #4875, #3603 ) ;
#16245=CARTESIAN_POINT ( 'NONE',  ( 14.63113973005795643, 4.926264598692385199, -222.4866305912601945 ) ) ;
#16246=CARTESIAN_POINT ( 'NONE',  ( 14.18709644517307922, -11.45356969546147496, -232.2178450427173004 ) ) ;
#16247=CARTESIAN_POINT ( 'NONE',  ( -12.14186164972853810, -9.217338937739926408, -220.4665480714278374 ) ) ;
#16248=CARTESIAN_POINT ( 'NONE',  ( -16.75313578746775889, -14.38352658620038937, -216.6304878158699978 ) ) ;
#16249=CARTESIAN_POINT ( 'NONE',  ( 4.555016420009541989, 17.65848956729471197, -229.5875910199184204 ) ) ;
#16251=CARTESIAN_POINT ( 'NONE',  ( -19.26845014167239611, 9.481468541508135672, -234.4856117705182328 ) ) ;
#16252=CARTESIAN_POINT ( 'NONE',  ( 4.730976410881341465, 17.65764351829336931, -217.6025626048331674 ) ) ;
#16253=CARTESIAN_POINT ( 'NONE',  ( -2.543684969149407227, 16.28137730373167713, -227.6987697727321915 ) ) ;
#16254=CARTESIAN_POINT ( 'NONE',  ( 15.24707275637840453, -5.950922448839978784, -232.7034617680506869 ) ) ;
#16256=CARTESIAN_POINT ( 'NONE',  ( 8.903385417657583289, 10.41040586594612272, -227.6527940987422198 ) ) ;
#16257=CARTESIAN_POINT ( 'NONE',  ( -25.20870746202117729, 11.68425842440532136, -223.9066764530103342 ) ) ;
#16258=CARTESIAN_POINT ( 'NONE',  ( 14.29548763234129538, 2.320071712424730315, -230.2610858871018422 ) ) ;
#16259=CARTESIAN_POINT ( 'NONE',  ( -6.723652888800149441, -28.28510889945508211, -226.1741921951756638 ) ) ;
#16264=CARTESIAN_POINT ( 'NONE',  ( 16.54345861550681107, 19.37554510112122230, -218.2240151908141002 ) ) ;
#16265=CARTESIAN_POINT ( 'NONE',  ( 17.83206265427627457, -15.38023228143295640, -231.0294926223175480 ) ) ;
#16267=CARTESIAN_POINT ( 'NONE',  ( -5.178973235464019886, -24.35492185057628944, -233.6431870320687381 ) ) ;
#16268=SHAPE_DEFINITION_REPRESENTATION ( #3480, #1546 ) ;
#16269=CARTESIAN_POINT ( 'NONE',  ( -3.082945806077231676, 30.69897765966285874, -224.2387254578930822 ) ) ;
#16270=CARTESIAN_POINT ( 'NONE',  ( -0.2758005215353623862, 11.79991891162212525, -226.8645588387054488 ) ) ;
#16272=CARTESIAN_POINT ( 'NONE',  ( -9.171998067665157350, 9.395241133357435714, -226.3428046914542051 ) ) ;
#16273=CARTESIAN_POINT ( 'NONE',  ( -15.33992272861872763, -7.600289318192222865, -231.6130094852651951 ) ) ;
#16276=CARTESIAN_POINT ( 'NONE',  ( -10.65455960636934662, 10.37188583052882862, -219.5197110153079620 ) ) ;
#16277=CARTESIAN_POINT ( 'NONE',  ( -18.48589171870721870, -21.38265182533571362, -233.2911668074952729 ) ) ;
#16279=CARTESIAN_POINT ( 'NONE',  ( 16.50235023187294203, -3.000022380394500310, -230.0447763498268614 ) ) ;
#16280=CARTESIAN_POINT ( 'NONE',  ( -17.65835845419170624, 22.55329142274348442, -231.2673511165784532 ) ) ;
#16282=CARTESIAN_POINT ( 'NONE',  ( -12.10179538005628963, 1.685214252672075030, -222.4835512146784424 ) ) ;
#16283=CARTESIAN_POINT ( 'NONE',  ( -1.973645837583506424, 28.78841935349527503, -228.5341874691134763 ) ) ;
#16284=CARTESIAN_POINT ( 'NONE',  ( 13.58841164691136427, 0.2900218890822029993, -227.9866932315656243 ) ) ;
#16285=CARTESIAN_POINT ( 'NONE',  ( 15.80790828609669951, 3.698719088746416972, -219.8106174092292804 ) ) ;
#16286=CARTESIAN_POINT ( 'NONE',  ( -8.398697845537501649, -22.62202615048447640, -219.0766901614751703 ) ) ;
#16288=CARTESIAN_POINT ( 'NONE',  ( 10.31623634631035991, 26.83927646318382898, -220.2315638557092541 ) ) ;
#16289=CARTESIAN_POINT ( 'NONE',  ( -5.854583994961135573, 13.10358817970001866, -222.4168379437668648 ) ) ;
#16290=CARTESIAN_POINT ( 'NONE',  ( -21.29946384424354733, 21.01772963953914442, -222.5871995662667757 ) ) ;
#16291=CARTESIAN_POINT ( 'NONE',  ( -26.61609457609114315, -10.18835510800150779, -222.8381276585760702 ) ) ;
#16294=CARTESIAN_POINT ( 'NONE',  ( -28.99926036811508467, 3.909990568804979194, -228.9613767892386988 ) ) ;
#16295=CARTESIAN_POINT ( 'NONE',  ( -5.902345112435694041, -11.50736153130091388, -224.0878888885884805 ) ) ;
#16296=CARTESIAN_POINT ( 'NONE',  ( 13.45886389386542525, 0.9032831457644521223, -227.8643385330375963 ) ) ;
#16297=CARTESIAN_POINT ( 'NONE',  ( -9.716674560061926869, 27.56227806819028103, -219.4917914922789919 ) ) ;
#16301=CARTESIAN_POINT ( 'NONE',  ( 20.09685469220202236, -2.033783885649083079, -233.1448060988079760 ) ) ;
#16302=CARTESIAN_POINT ( 'NONE',  ( 10.61539692146153691, 8.157890242340682718, -227.5705019877536301 ) ) ;
#16304=CARTESIAN_POINT ( 'NONE',  ( 16.38151749656409351, 8.902090001712490874, -231.2955017965201989 ) ) ;
#16306=CARTESIAN_POINT ( 'NONE',  ( -13.09367826499460818, -1.871088059101057244, -230.2970504731880510 ) ) ;
#16307=CARTESIAN_POINT ( 'NONE',  ( -15.46269062504165781, -26.67469327287815517, -225.2085449711190677 ) ) ;
#16310=CARTESIAN_POINT ( 'NONE',  ( -14.12265793148702464, 24.49085167151569919, -218.3312790639385241 ) ) ;
#16311=CARTESIAN_POINT ( 'NONE',  ( 22.53017539111736411, -13.33152463597901516, -234.4848520764015518 ) ) ;
#16313=CARTESIAN_POINT ( 'NONE',  ( 17.95694455891925756, -3.510678534943489026, -231.2643001502910067 ) ) ;
#16314=CARTESIAN_POINT ( 'NONE',  ( -14.06164063153489252, 2.050767714179807744, -227.2881998904968270 ) ) ;
#16315=CARTESIAN_POINT ( 'NONE',  ( 12.96449997971774870, 8.285709878278680662, -230.9518598506670628 ) ) ;
#16316=CARTESIAN_POINT ( 'NONE',  ( 11.27486163995310164, 25.12851252939060487, -222.6718455410222930 ) ) ;
#16318=CARTESIAN_POINT ( 'NONE',  ( 2.219167932009094901, -23.00164214691015729, -217.1940376169840476 ) ) ;
#16320=CARTESIAN_POINT ( 'NONE',  ( -6.111257124579617894, 15.89946952501658295, -216.3497764690875727 ) ) ;
#16321=CARTESIAN_POINT ( 'NONE',  ( -4.378220565073127624, 31.53459173284372952, -222.0564199190954753 ) ) ;
#16322=CARTESIAN_POINT ( 'NONE',  ( 26.90273745076186884, -10.52087603942467808, -226.9519702360728957 ) ) ;
#16323=CARTESIAN_POINT ( 'NONE',  ( -3.205260335674071648, 17.52234722004434531, -232.9754319808710363 ) ) ;
#16325=CARTESIAN_POINT ( 'NONE',  ( -2.917590128672695293, 18.81591489065672818, -216.3635620530855022 ) ) ;
#16326=CARTESIAN_POINT ( 'NONE',  ( 22.69522586737246783, 3.669837464059151344, -234.0947686933411944 ) ) ;
#16327=CARTESIAN_POINT ( 'NONE',  ( -17.79285498209129202, 9.187865686019035749, -216.3798185811636756 ) ) ;
#16329=CARTESIAN_POINT ( 'NONE',  ( 14.19800769603076240, 4.587407146151301518, -224.2928935459285071 ) ) ;
#16332=CARTESIAN_POINT ( 'NONE',  ( -1.973645837583506424, 28.78841935349527503, -228.5341874691134763 ) ) ;
#16333=CARTESIAN_POINT ( 'NONE',  ( -13.22951852716680676, -5.246159916193459338, -223.7538483380451453 ) ) ;
#16334=CARTESIAN_POINT ( 'NONE',  ( 21.39553407250273054, 8.453402029343234148, -217.9531594780983141 ) ) ;
#16335=CARTESIAN_POINT ( 'NONE',  ( 0.5573677079071300833, -14.80782849724859496, -218.9269569601107719 ) ) ;
#16337=CARTESIAN_POINT ( 'NONE',  ( -18.74633356284308761, 11.17209001323738704, -217.5809474206552068 ) ) ;
#16339=CARTESIAN_POINT ( 'NONE',  ( 9.020349274477036161, -13.22217574948208529, -220.4173403795374213 ) ) ;
#16340=CARTESIAN_POINT ( 'NONE',  ( 15.28499842775873319, 22.98894588155567931, -221.0942409093412095 ) ) ;
#16341=CARTESIAN_POINT ( 'NONE',  ( -21.23733589435050817, 17.25275849955597351, -229.9547908233139708 ) ) ;
#16342=CARTESIAN_POINT ( 'NONE',  ( -13.91932826323387395, 8.983986115891950064, -216.4624824187541776 ) ) ;
#16343=CARTESIAN_POINT ( 'NONE',  ( -16.98436007432217920, -11.01716238098750544, -231.0196200964405193 ) ) ;
#16345=CARTESIAN_POINT ( 'NONE',  ( 24.00840102751045890, 17.37402299239434100, -218.3110108534040137 ) ) ;
#16349=CARTESIAN_POINT ( 'NONE',  ( -12.17842630902860712, -4.030040138803427929, -228.6515579410213661 ) ) ;
#16350=CARTESIAN_POINT ( 'NONE',  ( 10.03842945413050458, 28.43460431997513638, -225.8374938385031214 ) ) ;
#16351=CARTESIAN_POINT ( 'NONE',  ( 28.03290210476798094, 13.48017620089690638, -224.9212082181537937 ) ) ;
#16352=CARTESIAN_POINT ( 'NONE',  ( -6.388048297418547961, 21.92257289597608150, -233.3290245341164848 ) ) ;
#16353=CARTESIAN_POINT ( 'NONE',  ( 10.46530733675539793, 8.351728317179080818, -222.7431177495969621 ) ) ;
#16354=CARTESIAN_POINT ( 'NONE',  ( 3.242550426224029447, -16.70085388461110654, -229.1030317736733650 ) ) ;
#16355=CARTESIAN_POINT ( 'NONE',  ( -0.3025942668150596315, -28.96010673020088788, -223.5534481764385646 ) ) ;
#16356=CARTESIAN_POINT ( 'NONE',  ( 17.00168025137501004, 6.212099629982537508, -219.0548246536471595 ) ) ;
#16357=CARTESIAN_POINT ( 'NONE',  ( 19.68037530048075112, -17.97179847169212508, -231.8517058357153076 ) ) ;
#16358=CARTESIAN_POINT ( 'NONE',  ( -15.15819830826754355, -2.370657588173597841, -221.8013720140894236 ) ) ;
#16360=CARTESIAN_POINT ( 'NONE',  ( -5.240862053303020573, -11.96147391800445270, -224.1453450823045443 ) ) ;
#16362=CARTESIAN_POINT ( 'NONE',  ( 3.673290835002071653, 15.92545533070904895, -226.4848186297188022 ) ) ;
#16364=CARTESIAN_POINT ( 'NONE',  ( -26.41026844077819291, 5.012316129610852933, -233.8406020309487872 ) ) ;
#16365=CARTESIAN_POINT ( 'NONE',  ( 0.7245137624042983227, 13.44764381486384330, -223.4043886706536455 ) ) ;
#16366=CARTESIAN_POINT ( 'NONE',  ( 7.042184411928968935, 23.28260216771182556, -230.5707103145148267 ) ) ;
#16367=CARTESIAN_POINT ( 'NONE',  ( 29.52516483900593158, -0.1522717672070824924, -221.3034020690409704 ) ) ;
#16369=CARTESIAN_POINT ( 'NONE',  ( 25.62718606866737403, 13.33219119508369310, -230.9315691959737933 ) ) ;
#16370=CARTESIAN_POINT ( 'NONE',  ( -25.36936018126600345, 11.57160208538938306, -224.9662154788713622 ) ) ;
#16371=CARTESIAN_POINT ( 'NONE',  ( -22.18165477997343871, 9.502253276305026475, -218.0070055737419636 ) ) ;
#16372=CARTESIAN_POINT ( 'NONE',  ( -1.615718423935818437, -15.01490656935555812, -223.2481059054151729 ) ) ;
#16374=CARTESIAN_POINT ( 'NONE',  ( 13.03557269046774714, 7.519834803053426775, -226.9490612297269081 ) ) ;
#16375=CARTESIAN_POINT ( 'NONE',  ( 11.76368234164141136, -12.26645877504561888, -220.6132173800162946 ) ) ;
#16378=CARTESIAN_POINT ( 'NONE',  ( -1.489322793389167288, -21.37773154815333498, -215.8826219457350817 ) ) ;
#16380=CARTESIAN_POINT ( 'NONE',  ( -6.474151797443945533, 21.29193859232740138, -215.9573456447696458 ) ) ;
#16381=CARTESIAN_POINT ( 'NONE',  ( 0.6332696906856497554, 18.74964962670039625, -234.8596399859513042 ) ) ;
#16383=CARTESIAN_POINT ( 'NONE',  ( -7.429838964355703901, 14.87322129099639234, -232.2632863647814077 ) ) ;
#16384=CARTESIAN_POINT ( 'NONE',  ( -13.83093441725390704, -7.146379636134302160, -230.0501880019394605 ) ) ;
#16387=CARTESIAN_POINT ( 'NONE',  ( -9.716674560061926869, 27.56227806819028103, -219.4917914922789919 ) ) ;
#16388=CARTESIAN_POINT ( 'NONE',  ( -3.350277215847999202, -25.10023987965119119, -233.9767109426786647 ) ) ;
#16391=CARTESIAN_POINT ( 'NONE',  ( -9.250876228778270871, 9.538614635316015722, -227.1332118982684563 ) ) ;
#16392=CARTESIAN_POINT ( 'NONE',  ( -17.17143024911216287, 2.756036084795755681, -233.9491886983466316 ) ) ;
#16393=CARTESIAN_POINT ( 'NONE',  ( 5.646952844456516019, 23.06006924884521325, -218.8221376988549878 ) ) ;
#16395=CARTESIAN_POINT ( 'NONE',  ( 27.66944030902029539, 6.857614156517904291, -220.9860880211026313 ) ) ;
#16396=CARTESIAN_POINT ( 'NONE',  ( -8.507271545618831254, -16.45592803179997787, -230.0780227380557790 ) ) ;
#16400=CARTESIAN_POINT ( 'NONE',  ( 8.554868430186942874, 10.42313681336814568, -223.0114508542762621 ) ) ;
#16401=CARTESIAN_POINT ( 'NONE',  ( 3.001892273201697048, 27.20292285420111966, -216.7800154582108689 ) ) ;
#16403=CARTESIAN_POINT ( 'NONE',  ( -29.01652113304903935, -3.607535226192160049, -222.1063433863846228 ) ) ;
#16406=CARTESIAN_POINT ( 'NONE',  ( 16.56146809408446430, -0.9616313295950813522, -228.5729530379900609 ) ) ;
#16407=CARTESIAN_POINT ( 'NONE',  ( 10.02513374692848913, 18.81568788741115128, -217.1505009242214612 ) ) ;
#16408=CARTESIAN_POINT ( 'NONE',  ( -3.174954051807135080, -13.80109495427747746, -226.5796556275459750 ) ) ;
#16409=CARTESIAN_POINT ( 'NONE',  ( 27.75679124201660741, 4.911524026080384075, -221.4430403652340829 ) ) ;
#16410=CARTESIAN_POINT ( 'NONE',  ( 1.217121169770782663, 15.31158828575123110, -230.6845728599757308 ) ) ;
#16414=CARTESIAN_POINT ( 'NONE',  ( -26.47320305716024791, 9.675235842009668019, -228.3542180911597654 ) ) ;
#16415=CARTESIAN_POINT ( 'NONE',  ( 19.66122710937851537, 22.83208755991274330, -220.0578523118790883 ) ) ;
#16416=DIRECTION ( 'NONE',  ( 0.000000000000000000, 0.000000000000000000, -1.000000000000000000 ) ) ;
#16417=CARTESIAN_POINT ( 'NONE',  ( 12.85408565574548412, 7.821283853063205171, -223.1248833997948111 ) ) ;
#16419=CARTESIAN_POINT ( 'NONE',  ( 25.63739587761438088, -9.098054415140415685, -222.2988516439644968 ) ) ;
#16420=CARTESIAN_POINT ( 'NONE',  ( -13.21314811618155716, -9.038438575223175064, -230.6430079410957603 ) ) ;
#16424=CARTESIAN_POINT ( 'NONE',  ( -1.707778556226592581, 19.51307486516442680, -232.5708079709245055 ) ) ;
#16425=CARTESIAN_POINT ( 'NONE',  ( 26.81360599170068326, -17.93330511230891844, -224.0089312182945491 ) ) ;
#16426=CARTESIAN_POINT ( 'NONE',  ( 18.22947608839760747, -6.525328669204546905, -217.7409786913911205 ) ) ;
#16427=CARTESIAN_POINT ( 'NONE',  ( -26.11114532382342901, 12.73400870066318902, -227.7653936945517046 ) ) ;
#16428=CARTESIAN_POINT ( 'NONE',  ( 8.554868430186942874, 10.42313681336814568, -223.0114508542762621 ) ) ;
#16429=CARTESIAN_POINT ( 'NONE',  ( 13.96918721733258195, 14.12724320058294403, -230.4946432816737172 ) ) ;
#16431=CARTESIAN_POINT ( 'NONE',  ( 6.264370104348762069, -18.85623240742893714, -216.4903287596617076 ) ) ;
#16433=CARTESIAN_POINT ( 'NONE',  ( -5.543543819386913540, 14.51457927969963713, -217.3847528063896846 ) ) ;
#16434=CARTESIAN_POINT ( 'NONE',  ( -19.90771709537278156, 23.83218599423810602, -225.0439263757368735 ) ) ;
#16435=CARTESIAN_POINT ( 'NONE',  ( 19.99722954683925025, -4.901308424099491745, -217.6076555004800070 ) ) ;
#16437=CARTESIAN_POINT ( 'NONE',  ( -2.698926868850080041, 12.89339462271858316, -226.7595176699009585 ) ) ;
#16440=CARTESIAN_POINT ( 'NONE',  ( 0.8673818989965740300, 28.69424263383094598, -231.7310846804014659 ) ) ;
#16441=CARTESIAN_POINT ( 'NONE',  ( 13.49694890958685711, 2.186465430673721677, -228.8273158381700512 ) ) ;
#16442=CARTESIAN_POINT ( 'NONE',  ( -11.46843428684449151, 6.508406145394057596, -225.7212143570321814 ) ) ;
#16443=CARTESIAN_POINT ( 'NONE',  ( 22.86997486125673618, 17.56009411325475966, -222.3578648042903296 ) ) ;
#16444=CARTESIAN_POINT ( 'NONE',  ( 8.321021197036545303, 25.59447019508656140, -228.6184429848799482 ) ) ;
#16445=CARTESIAN_POINT ( 'NONE',  ( 15.62880906446489959, 0.6839391200676235849, -227.9224688803754475 ) ) ;
#16447=CARTESIAN_POINT ( 'NONE',  ( 5.549682179574114471, 15.11687613544382280, -226.9959476502473308 ) ) ;
#16448=CARTESIAN_POINT ( 'NONE',  ( -19.50907964299920039, -17.77536300509877876, -217.8007844881196320 ) ) ;
#16449=CARTESIAN_POINT ( 'NONE',  ( 16.84848658399567611, 11.39632653812981644, -217.9589513831453473 ) ) ;
#16450=CARTESIAN_POINT ( 'NONE',  ( -3.624336683137088677, -15.65024371637965039, -218.6393395577867977 ) ) ;
#16452=CARTESIAN_POINT ( 'NONE',  ( -20.47640197314466093, 18.50423766437512541, -220.4440130802851456 ) ) ;
#16454=CARTESIAN_POINT ( 'NONE',  ( 24.96165930385824794, -17.14663603160204275, -224.2745859498249672 ) ) ;
#16455=CARTESIAN_POINT ( 'NONE',  ( 6.173705828530630768, 14.85108299334794957, -222.6284669816953112 ) ) ;
#16456=CARTESIAN_POINT ( 'NONE',  ( -19.65084584916038324, 18.01805631773661176, -219.5040736310571106 ) ) ;
#16457=CARTESIAN_POINT ( 'NONE',  ( -26.09112266552012471, 5.807188091516064077, -215.7774933166620883 ) ) ;
#16458=CARTESIAN_POINT ( 'NONE',  ( -24.91054099106560926, -7.366054470814448862, -220.6971974931307159 ) ) ;
#16459=CARTESIAN_POINT ( 'NONE',  ( 19.48863273024974418, 12.80680990455712909, -215.0408095016468053 ) ) ;
#16461=CARTESIAN_POINT ( 'NONE',  ( -15.25474278246548643, -4.999135024540048988, -232.7276810733381183 ) ) ;
#16462=CARTESIAN_POINT ( 'NONE',  ( 2.630208337444488453, 16.40323635460054774, -219.2570070657488088 ) ) ;
#16463=CARTESIAN_POINT ( 'NONE',  ( 21.04928763009552384, -0.2309942901367783852, -233.9427286327411366 ) ) ;
#16464=CARTESIAN_POINT ( 'NONE',  ( -5.529079411693809121, 13.00503897727793401, -226.8014833675713646 ) ) ;
#16465=CARTESIAN_POINT ( 'NONE',  ( 10.39636392256998221, 18.46527700675686035, -215.1860221565626148 ) ) ;
#16466=CARTESIAN_POINT ( 'NONE',  ( 4.144298419883110540, -16.00443160190133085, -221.4341300285535965 ) ) ;
#16467=CARTESIAN_POINT ( 'NONE',  ( 4.788325992165110456, -24.70830725884669121, -218.5516572218182603 ) ) ;
#16468=CARTESIAN_POINT ( 'NONE',  ( 17.07668571305246985, 2.037405138410691485, -219.7626854147787867 ) ) ;
#16469=CARTESIAN_POINT ( 'NONE',  ( 15.50779141722566656, -5.694711448414747856, -219.6385356284298211 ) ) ;
#16470=CARTESIAN_POINT ( 'NONE',  ( 22.24262848504226042, 2.205713500382400216, -232.7243927205662999 ) ) ;
#16471=CARTESIAN_POINT ( 'NONE',  ( -11.36971918743327237, -8.287084598727400220, -223.1364763414170227 ) ) ;
#16472=CARTESIAN_POINT ( 'NONE',  ( 7.804112641607792611, 19.76858558208418515, -218.6463059509973164 ) ) ;
#16474=CARTESIAN_POINT ( 'NONE',  ( 17.92683513449900445, 4.153309877386362814, -218.0960491240478234 ) ) ;
#16475=CARTESIAN_POINT ( 'NONE',  ( 10.66614775643814994, 26.29080367171353672, -230.0818785118670178 ) ) ;
#16476=CARTESIAN_POINT ( 'NONE',  ( -0.2748333203896175525, 17.57683079704640505, -221.1444293135629948 ) ) ;
#16477=CARTESIAN_POINT ( 'NONE',  ( 12.91141610427636621, -26.43280511468161720, -217.7946055251781274 ) ) ;
#16478=CARTESIAN_POINT ( 'NONE',  ( 12.95792863868717149, 16.83236386576623644, -216.3406066345214356 ) ) ;
#16479=CARTESIAN_POINT ( 'NONE',  ( -11.13829636790841704, 14.30978168460582189, -218.6922574227322400 ) ) ;
#16480=CARTESIAN_POINT ( 'NONE',  ( 20.92846067405557520, -2.114533307883533109, -233.2756072794335580 ) ) ;
#16481=CARTESIAN_POINT ( 'NONE',  ( 2.179383121900682951, -16.00498718933496889, -221.0566978482307832 ) ) ;
#16484=CARTESIAN_POINT ( 'NONE',  ( 14.54149994592679107, 8.070685273005897997, -229.7292930672863349 ) ) ;
#16485=CARTESIAN_POINT ( 'NONE',  ( 14.67088464789753388, -9.947482835004686663, -220.6944058341955497 ) ) ;
#16486=CARTESIAN_POINT ( 'NONE',  ( -14.58575946311604277, 2.190332613129932327, -228.6717927865686590 ) ) ;
#16488=CARTESIAN_POINT ( 'NONE',  ( -9.294226473174397540, -12.00440878504259601, -219.6990993854437875 ) ) ;
#16489=CARTESIAN_POINT ( 'NONE',  ( 5.343558017910363667, 26.29639771561252459, -218.1010331760174665 ) ) ;
#16490=CARTESIAN_POINT ( 'NONE',  ( 4.952019330116582907, 28.88045068338265509, -217.6369327391592208 ) ) ;
#16492=CARTESIAN_POINT ( 'NONE',  ( -9.517741096562200909, 20.63709896626785678, -234.1036702156204967 ) ) ;
#16493=CARTESIAN_POINT ( 'NONE',  ( -14.33274213004767716, -3.240524307521291725, -229.5155949954044559 ) ) ;
#16494=CARTESIAN_POINT ( 'NONE',  ( 30.05917755080113096, -2.930701380670650114, -221.3976229872638726 ) ) ;
#16496=CARTESIAN_POINT ( 'NONE',  ( -8.501641725227710111, 25.47064987787527102, -217.3358698761548737 ) ) ;
#16497=CARTESIAN_POINT ( 'NONE',  ( -7.264683844434491000, -10.24731347617596100, -229.2886802738593985 ) ) ;
#16498=CARTESIAN_POINT ( 'NONE',  ( 16.08921376350389920, -2.840750994787607731, -229.5571464835293796 ) ) ;
#16499=CARTESIAN_POINT ( 'NONE',  ( -12.78558550453068854, 7.693178343823584342, -230.0800953344970878 ) ) ;
#16500=CARTESIAN_POINT ( 'NONE',  ( -11.30246491834384770, 5.534029070539333794, -225.8243940897388597 ) ) ;
#16501=CARTESIAN_POINT ( 'NONE',  ( 5.079647427451626562, 16.77877517420371234, -220.7769382327915366 ) ) ;
#16502=CARTESIAN_POINT ( 'NONE',  ( 16.26115440404298340, 3.800605480264513059, -219.2833057824682612 ) ) ;
#16503=CARTESIAN_POINT ( 'NONE',  ( -7.461655027780660809, -14.63259296063595727, -227.5661480528262075 ) ) ;
#16506=CARTESIAN_POINT ( 'NONE',  ( -13.51406939156936104, 10.04301168678160749, -230.1761202643687056 ) ) ;
#16507=CARTESIAN_POINT ( 'NONE',  ( 8.903385417657583289, 10.41040586594612272, -227.6527940987422198 ) ) ;
#16508=CARTESIAN_POINT ( 'NONE',  ( -2.121548062149551495, 13.26065194155116345, -221.8830439064491884 ) ) ;
#16509=CARTESIAN_POINT ( 'NONE',  ( 30.87761267810551757, -2.376991648450896388, -225.4116222034606949 ) ) ;
#16512=CARTESIAN_POINT ( 'NONE',  ( -13.56774755469388616, 7.311522441667196226, -219.1912666243428021 ) ) ;
#16513=CARTESIAN_POINT ( 'NONE',  ( -6.651864601267788224, -12.12497212411570580, -228.9083653044881714 ) ) ;
#16514=CARTESIAN_POINT ( 'NONE',  ( 21.60524407607017849, 3.028118258437591415, -217.8361640396714449 ) ) ;
#16515=CARTESIAN_POINT ( 'NONE',  ( 11.33210854356620523, 22.81476816607802149, -217.8536224460118262 ) ) ;
#16517=CARTESIAN_POINT ( 'NONE',  ( -24.53276002501160136, 17.12571705644413811, -226.2419685911331442 ) ) ;
#16518=CARTESIAN_POINT ( 'NONE',  ( 12.58577552758108986, 11.40439409249366420, -217.4478085440898951 ) ) ;
#16519=SURFACE_STYLE_USAGE ( .BOTH. , #13363 ) ;
#16520=CYLINDRICAL_SURFACE ( 'NONE', #5506, 3.000000000000002665 ) ;
#16521=CARTESIAN_POINT ( 'NONE',  ( 11.87982377808925527, 10.85265283465803421, -229.5027252913499183 ) ) ;
#16523=CARTESIAN_POINT ( 'NONE',  ( 21.42236089941604860, -11.78161700756472641, -230.3636358161748490 ) ) ;
#16524=CARTESIAN_POINT ( 'NONE',  ( -14.73155177304599306, -1.817590056890399763, -226.9769936995019748 ) ) ;
#16527=CARTESIAN_POINT ( 'NONE',  ( -1.470815287892122125, 29.54293232078718745, -224.5855911371830302 ) ) ;
#16528=CARTESIAN_POINT ( 'NONE',  ( 12.30978816035033496, -6.276705103789536722, -231.2162571060900405 ) ) ;
#16529=CARTESIAN_POINT ( 'NONE',  ( 24.05826999138443156, -14.97270453765939102, -220.1026142722873260 ) ) ;
#16530=CARTESIAN_POINT ( 'NONE',  ( -27.52457542293397097, 5.447957517019466067, -230.2717933641555135 ) ) ;
#16531=CARTESIAN_POINT ( 'NONE',  ( 29.55842656951424985, 4.785221541509360854, -220.5134865854112718 ) ) ;
#16532=CARTESIAN_POINT ( 'NONE',  ( 15.20072702475037296, 19.31591084219522614, -219.7402199933931399 ) ) ;
#16534=CARTESIAN_POINT ( 'NONE',  ( -0.004649462380863607185, -15.32103018016390017, -221.8331694311728484 ) ) ;
#16536=CARTESIAN_POINT ( 'NONE',  ( -13.63292518690856170, 3.968236334994402981, -218.3158317831635316 ) ) ;
#16537=CARTESIAN_POINT ( 'NONE',  ( 13.09827881591457022, 28.40264942367575784, -221.1045935444571455 ) ) ;
#16538=CARTESIAN_POINT ( 'NONE',  ( -0.6224962293416278492, 14.12372964796689701, -218.2103911528446645 ) ) ;
#16539=CARTESIAN_POINT ( 'NONE',  ( 17.73959705210031146, -11.46016327460725748, -231.4839417819510459 ) ) ;
#16540=CARTESIAN_POINT ( 'NONE',  ( 0.4042326456706432647, 15.50845657815858303, -219.2680337625893401 ) ) ;
#16541=CARTESIAN_POINT ( 'NONE',  ( -15.15110768032078070, 3.517015312212880218, -219.5479300368539270 ) ) ;
#16543=CARTESIAN_POINT ( 'NONE',  ( -2.508488193221233953, 16.03207605874066033, -217.8880952293912969 ) ) ;
#16544=CARTESIAN_POINT ( 'NONE',  ( -15.72195651633673208, 2.938252489821347346, -222.2698596109374023 ) ) ;
#16545=CARTESIAN_POINT ( 'NONE',  ( -18.09776816382430908, 23.50806826204562583, -229.9568677523880638 ) ) ;
#16546=CARTESIAN_POINT ( 'NONE',  ( 21.25094435758043332, 17.68230636442804027, -229.7964888993842010 ) ) ;
#16547=CARTESIAN_POINT ( 'NONE',  ( 5.688640247940316641, 20.34961083808282822, -230.9155060479073711 ) ) ;
#16550=CARTESIAN_POINT ( 'NONE',  ( 11.40028598017942230, 13.60807601628675023, -220.9105305289655519 ) ) ;
#16551=CARTESIAN_POINT ( 'NONE',  ( -20.18470553695442860, -13.13924840112635195, -232.9662461559857718 ) ) ;
#16552=CARTESIAN_POINT ( 'NONE',  ( 14.85123888640019452, 5.067529763532427012, -221.9058491819374979 ) ) ;
#16553=CARTESIAN_POINT ( 'NONE',  ( -1.453954827973251929, -30.77017545459721859, -228.2950292831040713 ) ) ;
#16555=CARTESIAN_POINT ( 'NONE',  ( -4.879985665934096772, 15.33285679834440174, -220.9402849574511833 ) ) ;
#16557=CARTESIAN_POINT ( 'NONE',  ( 19.19076252585518105, -11.68002947460017715, -233.4322573972352188 ) ) ;
#16558=CARTESIAN_POINT ( 'NONE',  ( 20.85755584069816493, 20.53615333921957742, -227.2010381488614996 ) ) ;
#16559=CARTESIAN_POINT ( 'NONE',  ( -11.16203726658389606, 26.27101666727781648, -227.8592829514190612 ) ) ;
#16560=CARTESIAN_POINT ( 'NONE',  ( -13.55637112341987383, 4.614880311503475774, -231.8130385267184010 ) ) ;
#16561=CARTESIAN_POINT ( 'NONE',  ( -13.13160344394316503, -9.470348871083606568, -223.0142826039989075 ) ) ;
#16563=CARTESIAN_POINT ( 'NONE',  ( -25.06333669508177309, 2.553070212212491530, -230.2963116797556893 ) ) ;
#16565=CARTESIAN_POINT ( 'NONE',  ( -27.52442056016948868, -15.72718643249855397, -222.0944556419597689 ) ) ;
#16566=CARTESIAN_POINT ( 'NONE',  ( 16.69977105456987232, 16.51652889326612694, -233.6667933521891030 ) ) ;
#16567=CARTESIAN_POINT ( 'NONE',  ( 20.76808360334631232, 5.412616674732960931, -234.1222385626545304 ) ) ;
#16568=CARTESIAN_POINT ( 'NONE',  ( 1.898427734299754421, 12.47096978853034521, -227.5043976727869506 ) ) ;
#16569=CARTESIAN_POINT ( 'NONE',  ( 14.02309809840729393, 19.05079204846204277, -234.6885355850075143 ) ) ;
#16571=CARTESIAN_POINT ( 'NONE',  ( 4.239709385547987708, -16.34504625405869405, -220.9645569933060756 ) ) ;
#16573=CARTESIAN_POINT ( 'NONE',  ( -5.429593058350183910, -25.95961553913046416, -230.5291520159703111 ) ) ;
#16575=CARTESIAN_POINT ( 'NONE',  ( -20.06846544527470400, 7.877362284741439069, -235.3910773253824402 ) ) ;
#16576=CARTESIAN_POINT ( 'NONE',  ( 21.05631363308661363, -21.50266115212419393, -222.6654548186096747 ) ) ;
#16577=CARTESIAN_POINT ( 'NONE',  ( -27.88251101234890328, -7.575382714962081820, -221.6715981084135478 ) ) ;
#16578=CARTESIAN_POINT ( 'NONE',  ( -11.49803752765619258, -8.459563989871591971, -222.4296168992866853 ) ) ;
#16579=CARTESIAN_POINT ( 'NONE',  ( 9.575488824002899690, 13.89846378187365694, -220.1158735840035945 ) ) ;
#16581=CARTESIAN_POINT ( 'NONE',  ( -9.746008880186941781, 12.96562886885531896, -220.1990846131056401 ) ) ;
#16582=CARTESIAN_POINT ( 'NONE',  ( 11.17884645811568944, 10.10284797925214662, -221.0856722371208036 ) ) ;
#16583=CARTESIAN_POINT ( 'NONE',  ( 1.382955251742491898, 16.46353944795171032, -231.7743150979565030 ) ) ;
#16584=CARTESIAN_POINT ( 'NONE',  ( 16.82251835652528982, 18.18719385133374544, -231.8032941011735772 ) ) ;
#16585=CARTESIAN_POINT ( 'NONE',  ( 8.727084366397900084, -11.39314604550613375, -218.1375774943401495 ) ) ;
#16586=CARTESIAN_POINT ( 'NONE',  ( 10.95881707662767290, 12.06788758096456782, -231.4359029166177208 ) ) ;
#16587=CARTESIAN_POINT ( 'NONE',  ( -5.590964611773372894, 13.92546790642523113, -228.7941110425196882 ) ) ;
#16588=CARTESIAN_POINT ( 'NONE',  ( 0.4703770282364683197, -28.19050476347214484, -228.5103440588500519 ) ) ;
#16589=CARTESIAN_POINT ( 'NONE',  ( -29.95012366401462955, 4.746560250930182967, -224.6954343660969471 ) ) ;
#16592=CARTESIAN_POINT ( 'NONE',  ( 21.53262694368047647, 11.06794636811408594, -231.8394491640143826 ) ) ;
#16593=CARTESIAN_POINT ( 'NONE',  ( 15.58552416334512536, -6.625011841737234342, -222.1645676924547104 ) ) ;
#16595=CARTESIAN_POINT ( 'NONE',  ( -6.642805165258356404, -28.12267032419628521, -230.9452027245340560 ) ) ;
#16596=CARTESIAN_POINT ( 'NONE',  ( -3.514547081416551588, 30.38636916157537016, -227.3529586180979436 ) ) ;
#16598=CARTESIAN_POINT ( 'NONE',  ( 5.501756899793208255, 15.97909684020861043, -233.9380718515096191 ) ) ;
#16600=CARTESIAN_POINT ( 'NONE',  ( -2.208416658185406334, 29.10348627872611615, -219.8480645685746424 ) ) ;
#16601=CARTESIAN_POINT ( 'NONE',  ( -28.74911369566071784, -10.37195270599671737, -225.4617258471509729 ) ) ;
#16604=CARTESIAN_POINT ( 'NONE',  ( 2.539761864897490007, 23.64215977235053501, -233.4645566207487661 ) ) ;
#16605=CARTESIAN_POINT ( 'NONE',  ( -4.912481909026474192, -29.12074637257241250, -231.0965163926508410 ) ) ;
#16606=CARTESIAN_POINT ( 'NONE',  ( 2.098184199980985376, -13.29281380427311099, -222.1652846463370281 ) ) ;
#16607=CARTESIAN_POINT ( 'NONE',  ( 24.05826999138443156, -14.97270453765939102, -220.1026142722873260 ) ) ;
#16609=CARTESIAN_POINT ( 'NONE',  ( 14.18323607655884722, 3.286047475533308226, -222.8710065128477140 ) ) ;
#16610=CARTESIAN_POINT ( 'NONE',  ( 16.07044873961816123, 22.39643131523411412, -226.8512752114033901 ) ) ;
#16611=CARTESIAN_POINT ( 'NONE',  ( -21.89482327431018760, 1.733733432562314158, -233.1353281693111796 ) ) ;
#16612=CARTESIAN_POINT ( 'NONE',  ( -18.16160515720599022, 12.42447964075808997, -216.1086293678848449 ) ) ;
#16613=CARTESIAN_POINT ( 'NONE',  ( -19.35484598183500538, -9.368503549647014594, -231.4111816933332477 ) ) ;
#16615=CARTESIAN_POINT ( 'NONE',  ( -24.39036648059286350, 13.21953970265592027, -220.1632778389106591 ) ) ;
#16616=CARTESIAN_POINT ( 'NONE',  ( 5.702651035983461902, 12.42242820409033222, -224.7304266323218656 ) ) ;
#16617=CARTESIAN_POINT ( 'NONE',  ( 0.8673818989965740300, 28.69424263383094598, -231.7310846804014659 ) ) ;
#16619=CARTESIAN_POINT ( 'NONE',  ( -14.73475970555713310, -4.645830632990214148, -227.0446463473171832 ) ) ;
#16622=CARTESIAN_POINT ( 'NONE',  ( -20.18153419852512442, 14.25141268122526483, -233.5059133483111964 ) ) ;
#16623=CARTESIAN_POINT ( 'NONE',  ( -5.045022908720540045, -16.91549468467126616, -232.0765493255083243 ) ) ;
#16624=CARTESIAN_POINT ( 'NONE',  ( 13.57284447417419493, 1.290488679629692381, -227.7116397237339811 ) ) ;
#16625=CARTESIAN_POINT ( 'NONE',  ( 17.97843143658897347, 22.12221935793617078, -220.9346589834416079 ) ) ;
#16627=CARTESIAN_POINT ( 'NONE',  ( 14.02668320743028119, -5.282748560960272677, -221.9001732195871739 ) ) ;
#16628=CARTESIAN_POINT ( 'NONE',  ( -15.23792247720107440, 7.806131751461257373, -230.3336101049160902 ) ) ;
#16630=CARTESIAN_POINT ( 'NONE',  ( 27.16757474806794903, 2.676291341565463888, -220.8863403533574115 ) ) ;
#16634=CARTESIAN_POINT ( 'NONE',  ( 27.04607490430786854, 4.607450003618843049, -220.3758934308003461 ) ) ;
#16636=CARTESIAN_POINT ( 'NONE',  ( 20.55466028792283240, -8.067975053177056211, -219.1472888552992799 ) ) ;
#16637=CARTESIAN_POINT ( 'NONE',  ( -13.22951852716680676, -5.246159916193459338, -223.7538483380451453 ) ) ;
#16640=CARTESIAN_POINT ( 'NONE',  ( -4.813101935419741295, 13.68373293383429434, -229.7840611589179503 ) ) ;
#16641=CARTESIAN_POINT ( 'NONE',  ( 27.82583766398256486, 0.7543585032809253521, -232.9329547162639358 ) ) ;
#16642=CARTESIAN_POINT ( 'NONE',  ( 17.43540344723615476, -3.335533435063737340, -230.8961756483947738 ) ) ;
#16643=CARTESIAN_POINT ( 'NONE',  ( -18.14952719657095415, 1.368063294522122275, -218.0005379682515922 ) ) ;
#16644=CARTESIAN_POINT ( 'NONE',  ( 30.60340911705754863, 5.703403611927857497, -225.1938343315648297 ) ) ;
#16645=CARTESIAN_POINT ( 'NONE',  ( 24.14003655968566520, 13.76285650325712773, -228.1266575292093819 ) ) ;
#16646=CARTESIAN_POINT ( 'NONE',  ( 5.503098680704820111, -17.53359096179937993, -217.0817822229213618 ) ) ;
#16649=CARTESIAN_POINT ( 'NONE',  ( -21.89065952084861522, -0.9940043559354512226, -215.0000000000000000 ) ) ;
#16651=CARTESIAN_POINT ( 'NONE',  ( 17.04685026979186446, 18.05617612716381970, -216.0910122987878310 ) ) ;
#16652=CARTESIAN_POINT ( 'NONE',  ( 9.100443535964535258, 24.01370002727352215, -234.5397711707082635 ) ) ;
#16653=CARTESIAN_POINT ( 'NONE',  ( 14.78595257191855694, -4.705020206487795065, -221.9958499870062099 ) ) ;
#16654=CARTESIAN_POINT ( 'NONE',  ( -5.807479211365208727, 19.77444019604324410, -216.0778658752277863 ) ) ;
#16655=CARTESIAN_POINT ( 'NONE',  ( -25.61997837663875188, 10.01664178086244483, -231.6711741719404074 ) ) ;
#16656=CARTESIAN_POINT ( 'NONE',  ( 12.75306435971521068, 14.56583715532477186, -214.9711136650476533 ) ) ;
#16657=CARTESIAN_POINT ( 'NONE',  ( -17.89085717681497201, 10.08962028281416856, -232.3705156551908431 ) ) ;
#16658=CARTESIAN_POINT ( 'NONE',  ( -3.368164009525018265, 19.03203264544105622, -233.5986411977714567 ) ) ;
#16659=CARTESIAN_POINT ( 'NONE',  ( 21.35706335192880445, 15.67286272432725092, -219.2578158352350783 ) ) ;
#16661=CARTESIAN_POINT ( 'NONE',  ( 10.64798096806036121, 19.48085866535796740, -231.3996658690317361 ) ) ;
#16663=CARTESIAN_POINT ( 'NONE',  ( 14.56914850832129815, -2.041740472307377985, -224.7121590863160350 ) ) ;
#16665=CARTESIAN_POINT ( 'NONE',  ( -14.73155177304599306, -1.817590056890399763, -226.9769936995019748 ) ) ;
#16666=CARTESIAN_POINT ( 'NONE',  ( 14.31308345469695453, 12.76656023072872159, -231.9445021321040770 ) ) ;
#16667=CARTESIAN_POINT ( 'NONE',  ( -8.288471666609035893, -17.31860360376325403, -217.6655967056599366 ) ) ;
#16670=CARTESIAN_POINT ( 'NONE',  ( -17.08384421609436643, 23.56421365837046622, -225.2902702884460666 ) ) ;
#16671=CARTESIAN_POINT ( 'NONE',  ( 7.739744183733028748, -12.54214339878522999, -227.5419174737939159 ) ) ;
#16672=CARTESIAN_POINT ( 'NONE',  ( 11.17884645811568944, 10.10284797925214662, -221.0856722371208036 ) ) ;
#16673=CARTESIAN_POINT ( 'NONE',  ( -4.073886805163430935, 14.35067061637828623, -226.4733297826468572 ) ) ;
#16674=CARTESIAN_POINT ( 'NONE',  ( -28.88770769694534479, 14.24820799418726480, -223.2044777450442155 ) ) ;
#16675=CARTESIAN_POINT ( 'NONE',  ( -18.87172488519036762, -12.11125346135639802, -231.2159161446224402 ) ) ;
#16676=CARTESIAN_POINT ( 'NONE',  ( -17.91769793922991028, 3.277678596821882007, -219.5526088240203819 ) ) ;
#16679=CARTESIAN_POINT ( 'NONE',  ( -30.16187987321119834, 0.7031948255570967810, -222.4584828387981474 ) ) ;
#16680=CARTESIAN_POINT ( 'NONE',  ( 9.798337081649805214, 12.27506320122302697, -218.9346733583377613 ) ) ;
#16682=CARTESIAN_POINT ( 'NONE',  ( -24.40185606299549192, 11.66496215664722236, -221.9473669705449765 ) ) ;
#16683=CARTESIAN_POINT ( 'NONE',  ( -2.508488193221233953, 16.03207605874066033, -217.8880952293912969 ) ) ;
#16684=CARTESIAN_POINT ( 'NONE',  ( 4.228809304811371739, 12.93497549386982470, -230.7917784105561907 ) ) ;
#16685=CARTESIAN_POINT ( 'NONE',  ( -12.42003616114091358, -24.71691410793946986, -217.8239624370676779 ) ) ;
#16687=CARTESIAN_POINT ( 'NONE',  ( 6.203932113039332563, -21.09630782756332223, -232.3325312104709894 ) ) ;
#16688=CARTESIAN_POINT ( 'NONE',  ( -15.39319649241581800, 0.3563955590804028795, -232.4397289486159082 ) ) ;
#16689=CARTESIAN_POINT ( 'NONE',  ( 24.05826999138443156, -14.97270453765939102, -220.1026142722873260 ) ) ;
#16690=CARTESIAN_POINT ( 'NONE',  ( -21.80830016239255897, -4.781675611938959847, -217.4666014280278148 ) ) ;
#16691=CARTESIAN_POINT ( 'NONE',  ( -5.804961988600464196, -12.67915086496026511, -228.7923277404792088 ) ) ;
#16692=CARTESIAN_POINT ( 'NONE',  ( 23.08329078023534109, 11.96623404944238978, -217.1428499060670845 ) ) ;
#16694=CARTESIAN_POINT ( 'NONE',  ( -18.16160515720599022, 12.42447964075808997, -216.1086293678848449 ) ) ;
#16695=CARTESIAN_POINT ( 'NONE',  ( 10.98110116949302828, 13.70618071521442971, -230.2797640191687378 ) ) ;
#16697=CARTESIAN_POINT ( 'NONE',  ( 9.333020543840051531, 16.91085096921651143, -217.7308990335875762 ) ) ;
#16698=CARTESIAN_POINT ( 'NONE',  ( 11.17884645811568944, 10.10284797925214662, -221.0856722371208036 ) ) ;
#16699=CARTESIAN_POINT ( 'NONE',  ( 7.844578353157877437, -11.10597526584381356, -230.9016046914076128 ) ) ;
#16700=CARTESIAN_POINT ( 'NONE',  ( 14.33191776452776622, 5.147404080619256916, -219.0172570056664938 ) ) ;
#16701=CARTESIAN_POINT ( 'NONE',  ( -11.11479000491124047, 20.76372272540567110, -218.2001872134434564 ) ) ;
#16702=CARTESIAN_POINT ( 'NONE',  ( -7.266348978356541366, 16.38312187400933340, -217.9429203627011873 ) ) ;
#16703=CARTESIAN_POINT ( 'NONE',  ( -17.01799258133205228, -17.74971190556693657, -217.5843211863294755 ) ) ;
#16704=CARTESIAN_POINT ( 'NONE',  ( -28.59157645096996347, 5.137867505054540374, -220.4667042235044505 ) ) ;
#16706=CARTESIAN_POINT ( 'NONE',  ( 22.46220731426537043, 18.23201731183003460, -227.5436199598787539 ) ) ;
#16707=CARTESIAN_POINT ( 'NONE',  ( 7.317916060359300978, -13.14109500694934951, -227.5371884182924305 ) ) ;
#16708=CARTESIAN_POINT ( 'NONE',  ( -25.19248792833826300, 13.40115236862232528, -221.2817950683888455 ) ) ;
#16710=CARTESIAN_POINT ( 'NONE',  ( -20.11874861854083463, -21.11755179634840474, -229.7504124090357323 ) ) ;
#16712=CARTESIAN_POINT ( 'NONE',  ( -20.86570240061152148, 1.122719768445835875, -219.0984131021933763 ) ) ;
#16715=CARTESIAN_POINT ( 'NONE',  ( 4.228809304811371739, 12.93497549386982470, -230.7917784105561907 ) ) ;
#16717=CARTESIAN_POINT ( 'NONE',  ( -11.42613629117093765, 28.09170287990588832, -228.7150250545069241 ) ) ;
#16718=CARTESIAN_POINT ( 'NONE',  ( 29.72361553920624999, -4.223772423702004453, -224.3921473884441866 ) ) ;
#16721=CARTESIAN_POINT ( 'NONE',  ( 2.008896548638861024, 20.64812324442097591, -233.5818019448501843 ) ) ;
#16722=CARTESIAN_POINT ( 'NONE',  ( -5.856318878364832337, -22.45395696943396402, -215.0711972856051943 ) ) ;
#16723=CARTESIAN_POINT ( 'NONE',  ( 6.053458391837899910, -12.85229775019162268, -220.9645494416007523 ) ) ;
#16724=CARTESIAN_POINT ( 'NONE',  ( 24.56541673123750158, -5.996287403333383281, -231.6940117905984664 ) ) ;
#16725=CARTESIAN_POINT ( 'NONE',  ( -15.05930145804884290, 24.78193219970826533, -223.0510781988847953 ) ) ;
#16726=CARTESIAN_POINT ( 'NONE',  ( 8.858651440950676914, 22.47383302477780376, -230.7859943773311215 ) ) ;
#16728=CARTESIAN_POINT ( 'NONE',  ( -20.04070223234628756, 18.12164545743767263, -231.9292141396248610 ) ) ;
#16729=CARTESIAN_POINT ( 'NONE',  ( -15.55375487336196372, -9.676988738288478942, -219.9111427047364202 ) ) ;
#16730=CARTESIAN_POINT ( 'NONE',  ( -11.08731210905863840, 25.61052584666692766, -228.9953606804266997 ) ) ;
#16731=CARTESIAN_POINT ( 'NONE',  ( 18.81274554574540403, 10.85963742466947224, -234.0446454529665345 ) ) ;
#16732=CARTESIAN_POINT ( 'NONE',  ( 7.283976506941576723, 24.82246917020504284, -234.3244871078919402 ) ) ;
#16733=CARTESIAN_POINT ( 'NONE',  ( 13.92699808111095905, -7.117895771238833547, -219.6066573659836081 ) ) ;
#16737=CARTESIAN_POINT ( 'NONE',  ( -18.09776816382430908, 23.50806826204562583, -229.9568677523880638 ) ) ;
#16738=CARTESIAN_POINT ( 'NONE',  ( -3.664580975482237157, -26.87662451849047329, -230.7630177344243236 ) ) ;
#16740=CARTESIAN_POINT ( 'NONE',  ( 12.18657022793382794, 26.76558097653315471, -221.8882195427397335 ) ) ;
#16742=CARTESIAN_POINT ( 'NONE',  ( 22.36788034568564854, -2.140002702436959225, -217.7104380410378610 ) ) ;
#16743=CARTESIAN_POINT ( 'NONE',  ( -13.56774755469388616, 7.311522441667196226, -219.1912666243428021 ) ) ;
#16744=CARTESIAN_POINT ( 'NONE',  ( -16.09559989144903369, 12.31939076846282966, -216.7948290530243298 ) ) ;
#16745=CARTESIAN_POINT ( 'NONE',  ( 24.78377098693636427, 3.871650763546384155, -231.3521132786341923 ) ) ;
#16746=CARTESIAN_POINT ( 'NONE',  ( 13.70955873423178772, 0.4527561487833433596, -222.0331215939001197 ) ) ;
#16748=CARTESIAN_POINT ( 'NONE',  ( -14.29986196492902550, 0.06805469746732484282, -227.4167624117703213 ) ) ;
#16749=CARTESIAN_POINT ( 'NONE',  ( 24.99579664921074240, -7.791002435033769657, -229.1824765006467715 ) ) ;
#16751=CARTESIAN_POINT ( 'NONE',  ( -20.85586116824185510, -1.996934699305910499, -232.3804859832740135 ) ) ;
#16755=CARTESIAN_POINT ( 'NONE',  ( 8.961491954973460849, 17.27041174997091844, -219.7661252763212474 ) ) ;
#16756=CARTESIAN_POINT ( 'NONE',  ( 3.813635332914135923, -14.61080527247722927, -220.2619188551939828 ) ) ;
#16757=CARTESIAN_POINT ( 'NONE',  ( 18.00123703865980218, -15.82960056198189491, -233.0014896689109776 ) ) ;
#16758=CARTESIAN_POINT ( 'NONE',  ( -11.35482716595652875, 11.86850131893102223, -220.6599844941370350 ) ) ;
#16759=CARTESIAN_POINT ( 'NONE',  ( -16.37512411505367282, 2.406627362596846620, -227.7341547288202719 ) ) ;
#16760=CARTESIAN_POINT ( 'NONE',  ( 17.51175949430614409, 14.31829016556564937, -218.8195841045835550 ) ) ;
#16762=CARTESIAN_POINT ( 'NONE',  ( 7.797975340826715396, -14.61189063385648623, -232.7894517818505733 ) ) ;
#16764=CARTESIAN_POINT ( 'NONE',  ( -11.80036766549451599, 3.629178540272184783, -221.4826559383200220 ) ) ;
#16765=CARTESIAN_POINT ( 'NONE',  ( 4.024086222410633518, 12.48004227094270746, -230.0177668608922374 ) ) ;
#16766=CARTESIAN_POINT ( 'NONE',  ( 4.914880347045685660, 14.54749271951947698, -232.8668677254037789 ) ) ;
#16767=CARTESIAN_POINT ( 'NONE',  ( 23.10971261601581617, -16.35996695089516706, -224.5402406813554421 ) ) ;
#16768=CARTESIAN_POINT ( 'NONE',  ( -6.855867220396999251, 12.17758473459128332, -220.6375607554995213 ) ) ;
#16769=CARTESIAN_POINT ( 'NONE',  ( -14.07917727715460821, 7.534853284453274291, -218.6337090155677458 ) ) ;
#16771=CARTESIAN_POINT ( 'NONE',  ( 8.546572992885776543, 19.06776382077057974, -214.7173484156796519 ) ) ;
#16772=CARTESIAN_POINT ( 'NONE',  ( -22.32700334442577272, 3.978587747811427988, -218.4803616146862453 ) ) ;
#16775=CARTESIAN_POINT ( 'NONE',  ( -3.755296588130283553, 23.77975947300719284, -233.7323173085780752 ) ) ;
#16777=CARTESIAN_POINT ( 'NONE',  ( 9.253909228257674258, 17.69332415812615977, -230.9900471521432621 ) ) ;
#16778=CARTESIAN_POINT ( 'NONE',  ( 28.52058947142581502, -1.755848367977142610, -221.9695116608532715 ) ) ;
#16781=CARTESIAN_POINT ( 'NONE',  ( -27.88251101234890328, -7.575382714962081820, -221.6715981084135478 ) ) ;
#16782=CARTESIAN_POINT ( 'NONE',  ( 27.40550551777678123, 5.967061366481472895, -228.7463788799179554 ) ) ;
#16783=CARTESIAN_POINT ( 'NONE',  ( -20.23770393675990675, -19.63250941609856426, -227.7987059506201319 ) ) ;
#16785=CARTESIAN_POINT ( 'NONE',  ( -4.080659539198054020, 15.43130099126780408, -228.8058965243247656 ) ) ;
#16786=CARTESIAN_POINT ( 'NONE',  ( 19.57710422433000019, -21.48596639614413562, -228.6055549924913635 ) ) ;
#16787=CARTESIAN_POINT ( 'NONE',  ( 8.778334628954494789, 12.71782457734010841, -222.1923057070808909 ) ) ;
#16788=CARTESIAN_POINT ( 'NONE',  ( -5.775873073292457249, 17.47547275616994256, -218.7209647771908578 ) ) ;
#16789=CARTESIAN_POINT ( 'NONE',  ( -13.58389614404818069, 15.11490620317918676, -215.3922994348461941 ) ) ;
#16791=CARTESIAN_POINT ( 'NONE',  ( -17.12341639776428437, -14.09197680242149886, -218.6048700820433339 ) ) ;
#16792=CARTESIAN_POINT ( 'NONE',  ( 13.70635042947887428, -1.390919209824193592, -225.3477037409554953 ) ) ;
#16794=CARTESIAN_POINT ( 'NONE',  ( -19.19980083083115474, -2.588899828715947038, -216.2953230342753557 ) ) ;
#16795=CARTESIAN_POINT ( 'NONE',  ( 17.31940731551425827, 24.90170669671083914, -222.9868986272316533 ) ) ;
#16796=CARTESIAN_POINT ( 'NONE',  ( -17.99155049254074612, 5.190958499132906745, -220.1449419322306937 ) ) ;
#16797=CARTESIAN_POINT ( 'NONE',  ( 1.682843645364419993, 12.02583837823347679, -224.9288196625490457 ) ) ;
#16798=CARTESIAN_POINT ( 'NONE',  ( 18.84307465506600465, 4.899879697440840509, -218.2189947030338715 ) ) ;
#16800=CARTESIAN_POINT ( 'NONE',  ( -6.443428446094314310, -19.32516562084312994, -233.2789765400915201 ) ) ;
#16802=CARTESIAN_POINT ( 'NONE',  ( -19.43452863239301820, -21.19996443032342626, -221.1427059245750399 ) ) ;
#16803=CARTESIAN_POINT ( 'NONE',  ( -17.22166590524039265, 4.587137274468266135, -215.4863060638890033 ) ) ;
#16804=CARTESIAN_POINT ( 'NONE',  ( 7.958080982411646076, -16.12895853103474408, -217.0903302464454612 ) ) ;
#16805=CARTESIAN_POINT ( 'NONE',  ( 16.48937362995332734, -6.768414299447169213, -233.6525893218997680 ) ) ;
#16806=CARTESIAN_POINT ( 'NONE',  ( -19.31342342724724759, -3.870051895940637365, -217.8584481481169348 ) ) ;
#16807=CARTESIAN_POINT ( 'NONE',  ( 18.13412043358480474, 12.55378873098427128, -233.2186159706515696 ) ) ;
#16809=CARTESIAN_POINT ( 'NONE',  ( -12.27164519775873686, 10.97713184439464840, -231.6269036897678291 ) ) ;
#16810=CARTESIAN_POINT ( 'NONE',  ( 12.11771628698343051, 17.56545729485151952, -218.0322663566023493 ) ) ;
#16811=CARTESIAN_POINT ( 'NONE',  ( 10.85888002857596923, 15.81835858589122878, -232.3913150909872627 ) ) ;
#16812=CARTESIAN_POINT ( 'NONE',  ( 6.173705828530630768, 14.85108299334794957, -222.6284669816953112 ) ) ;
#16813=CARTESIAN_POINT ( 'NONE',  ( 14.85580775603058079, -28.43502054068834894, -222.5810199743787905 ) ) ;
#16814=CARTESIAN_POINT ( 'NONE',  ( -6.260151855817680300, 29.88549235135308635, -226.8929519981915064 ) ) ;
#16815=CARTESIAN_POINT ( 'NONE',  ( -20.43618815875133521, 1.403378831510147196, -232.9646741665398224 ) ) ;
#16817=CARTESIAN_POINT ( 'NONE',  ( 13.69275646168278371, 8.674223198772375909, -220.8699857572541987 ) ) ;
#16818=CARTESIAN_POINT ( 'NONE',  ( 6.028509222145709501, -20.27756025184508815, -216.6192952284833950 ) ) ;
#16819=CARTESIAN_POINT ( 'NONE',  ( -17.78731991475362406, 16.78509880370027929, -218.2387321183659310 ) ) ;
#16820=CARTESIAN_POINT ( 'NONE',  ( 1.104227501629593045, 25.05528885094460989, -231.9808705443460326 ) ) ;
#16822=CARTESIAN_POINT ( 'NONE',  ( -12.04756914620937636, -13.80987496524771885, -232.8991007102355582 ) ) ;
#16823=CARTESIAN_POINT ( 'NONE',  ( 30.52813181070726856, 5.438803974502569361, -223.5441926215666513 ) ) ;
#16824=CARTESIAN_POINT ( 'NONE',  ( 11.78717493688862206, 28.63884142527983556, -229.7724827508652652 ) ) ;
#16825=CARTESIAN_POINT ( 'NONE',  ( -6.474151797443945533, 21.29193859232740138, -215.9573456447696458 ) ) ;
#16826=CARTESIAN_POINT ( 'NONE',  ( 20.29455491689504498, -15.47394441642566143, -219.8812143983372778 ) ) ;
#16827=CARTESIAN_POINT ( 'NONE',  ( 28.96372477351199137, -10.18960100487436904, -225.5971803650229504 ) ) ;
#16829=CARTESIAN_POINT ( 'NONE',  ( 1.217121169770782663, 15.31158828575123110, -230.6845728599757308 ) ) ;
#16830=CARTESIAN_POINT ( 'NONE',  ( -10.53630953054794794, -7.637555647514923329, -229.7964863767589918 ) ) ;
#16831=CARTESIAN_POINT ( 'NONE',  ( 6.589392574981438599, -17.08498810221841069, -232.9613445306918322 ) ) ;
#16832=B_SPLINE_CURVE_WITH_KNOTS ( 'NONE', 3,
 ( #793, #2700, #1018, #18350, #906, #11154, #16445, #4168, #2808, #17913 ),
 .UNSPECIFIED., .F., .F.,
 ( 4, 2, 2, 2, 4 ),
 ( 0.005560051141765639041, 0.005841872804505881742, 0.006123694467246125310, 0.006405516129986368878, 0.006687337792726613314 ),
 .UNSPECIFIED. ) ;
#16833=CARTESIAN_POINT ( 'NONE',  ( 13.36656406724190305, -19.73987914515934960, -233.3798509643240209 ) ) ;
#16834=CARTESIAN_POINT ( 'NONE',  ( -9.746008880186941781, 12.96562886885531896, -220.1990846131056401 ) ) ;
#16836=CARTESIAN_POINT ( 'NONE',  ( 14.66646255503707152, 18.43809875292740230, -219.3480462970252063 ) ) ;
#16838=CARTESIAN_POINT ( 'NONE',  ( -26.41026844077819291, 5.012316129610852933, -233.8406020309487872 ) ) ;
#16839=CARTESIAN_POINT ( 'NONE',  ( -26.61609457609114315, -10.18835510800150779, -222.8381276585760702 ) ) ;
#16841=CARTESIAN_POINT ( 'NONE',  ( -17.08384421609436643, 23.56421365837046622, -225.2902702884460666 ) ) ;
#16842=CARTESIAN_POINT ( 'NONE',  ( 14.69879291197755222, 10.86005690695417236, -216.7815908316746913 ) ) ;
#16843=CARTESIAN_POINT ( 'NONE',  ( -5.836418080594380164, 30.19240250712089590, -223.8354869487762357 ) ) ;
#16845=CARTESIAN_POINT ( 'NONE',  ( 15.07245478799217686, -4.018468087397350175, -231.0118529037252699 ) ) ;
#16847=ORIENTED_EDGE ( 'NONE', *, *, #6721, .T. ) ;
#16848=CARTESIAN_POINT ( 'NONE',  ( -25.61997837663875188, 10.01664178086244483, -231.6711741719404074 ) ) ;
#16849=CARTESIAN_POINT ( 'NONE',  ( -26.48368569639269055, -17.40725828600530534, -221.7871577296580199 ) ) ;
#16851=CARTESIAN_POINT ( 'NONE',  ( 10.07175337281514871, 14.76776740066196325, -231.7834566702614723 ) ) ;
#16853=CARTESIAN_POINT ( 'NONE',  ( 13.96958060839473958, -9.488587112651741151, -218.7731372952745232 ) ) ;
#16855=CARTESIAN_POINT ( 'NONE',  ( -16.74550766701807447, 3.787526820511904813, -217.9802846976114381 ) ) ;
#16856=CARTESIAN_POINT ( 'NONE',  ( -10.33514150881494942, 13.62639309082336503, -216.9544063991933172 ) ) ;
#16857=CARTESIAN_POINT ( 'NONE',  ( 27.54521312182184545, 10.10774643363308023, -222.6232199463151744 ) ) ;
#16858=CARTESIAN_POINT ( 'NONE',  ( -6.749503758482277682, -23.22604375411988187, -218.1095993038993299 ) ) ;
#16860=CARTESIAN_POINT ( 'NONE',  ( 21.31262902390056624, 0.4111834581965390645, -232.0572713672585792 ) ) ;
#16863=CARTESIAN_POINT ( 'NONE',  ( 27.74277644662361197, -2.671700443591659369, -227.2909148725441355 ) ) ;
#16864=CARTESIAN_POINT ( 'NONE',  ( 14.83290459615719215, -2.296615622475745688, -226.9301701175285757 ) ) ;
#16867=CARTESIAN_POINT ( 'NONE',  ( 3.755480357635514022, 24.23367984900377436, -231.4105847235276201 ) ) ;
#16868=CARTESIAN_POINT ( 'NONE',  ( 14.43570356028121893, -19.75277720499002498, -215.7015347705405759 ) ) ;
#16869=CARTESIAN_POINT ( 'NONE',  ( 14.98777556431132219, -10.10815648641214004, -217.9795565018743844 ) ) ;
#16870=CARTESIAN_POINT ( 'NONE',  ( -14.69827142695382527, 14.49176359921644597, -217.9600391472806109 ) ) ;
#16871=CARTESIAN_POINT ( 'NONE',  ( 15.96089671440110713, 1.143943728337336374, -218.3532651118343892 ) ) ;
#16872=CARTESIAN_POINT ( 'NONE',  ( 14.40184562439531213, 6.414772937171507650, -227.4651811604036595 ) ) ;
#16874=CARTESIAN_POINT ( 'NONE',  ( -1.686103422391260764, -28.85289795882446029, -227.6662241409997876 ) ) ;
#16876=CARTESIAN_POINT ( 'NONE',  ( -16.95112677453439431, 10.32962960657076934, -214.9445123409346650 ) ) ;
#16878=CARTESIAN_POINT ( 'NONE',  ( 9.253342549662157523, 15.33540844142859605, -216.2601104504267937 ) ) ;
#16879=CARTESIAN_POINT ( 'NONE',  ( 12.41447124200992391, -12.24348532208574269, -228.9129928441363973 ) ) ;
#16880=CARTESIAN_POINT ( 'NONE',  ( 11.13678936984666912, 26.95732789089726111, -228.8350761760834757 ) ) ;
#16881=CARTESIAN_POINT ( 'NONE',  ( -14.68037037322036475, 3.441677802729143920, -220.1396515630443389 ) ) ;
#16882=CARTESIAN_POINT ( 'NONE',  ( 19.13589083395335422, 16.69125564174534659, -234.7442498487877174 ) ) ;
#16883=CARTESIAN_POINT ( 'NONE',  ( -25.94982248293519689, 10.67899231259548287, -221.1273147719203962 ) ) ;
#16884=CARTESIAN_POINT ( 'NONE',  ( -3.060450601941519189, 13.29454208326677289, -222.0135664617158682 ) ) ;
#16885=CARTESIAN_POINT ( 'NONE',  ( 20.58703255433590940, 0.4816031003617209372, -231.9427175861361263 ) ) ;
#16886=CARTESIAN_POINT ( 'NONE',  ( 4.894897393135387631, 18.48819632322109996, -230.2131424875790628 ) ) ;
#16887=CARTESIAN_POINT ( 'NONE',  ( 20.15756451863428111, -2.090604891399794774, -217.8900786001194945 ) ) ;
#16891=CARTESIAN_POINT ( 'NONE',  ( -31.84745724608465522, 5.474219582435353004, -224.7210333253351564 ) ) ;
#16892=CARTESIAN_POINT ( 'NONE',  ( -23.94935377092574669, -14.34094158514532680, -226.5194954081123342 ) ) ;
#16894=CARTESIAN_POINT ( 'NONE',  ( -10.23029362138610843, 26.44342627367518617, -221.6879936327511871 ) ) ;
#16895=CARTESIAN_POINT ( 'NONE',  ( 5.037691872308702301, -15.96383311541683270, -230.0422288358542460 ) ) ;
#16896=CARTESIAN_POINT ( 'NONE',  ( 21.46274988498219471, 20.25395488059580984, -223.1777011585387243 ) ) ;
#16897=CARTESIAN_POINT ( 'NONE',  ( -10.23029362138610843, 26.44342627367518617, -221.6879936327511871 ) ) ;
#16898=CARTESIAN_POINT ( 'NONE',  ( -23.95129667199961077, 20.99391807043993552, -227.1541646794576081 ) ) ;
#16899=CARTESIAN_POINT ( 'NONE',  ( 31.97344890504648518, -0.7122400102224841767, -225.1892660388073466 ) ) ;
#16901=CARTESIAN_POINT ( 'NONE',  ( 11.87982377808925527, 10.85265283465803421, -229.5027252913499183 ) ) ;
#16902=CARTESIAN_POINT ( 'NONE',  ( -19.84402263676350131, 8.565754689849573111, -217.6561116767911983 ) ) ;
#16903=CARTESIAN_POINT ( 'NONE',  ( 29.96674103997387206, 4.060923908484647349, -228.5323681967686298 ) ) ;
#16905=CARTESIAN_POINT ( 'NONE',  ( -22.27532461284199528, -3.712691205162892416, -215.8122794664481603 ) ) ;
#16906=CARTESIAN_POINT ( 'NONE',  ( 6.040050017043670394, 13.67534390435379699, -220.4759402345340504 ) ) ;
#16907=CARTESIAN_POINT ( 'NONE',  ( -26.64664107080812627, 5.256684826493772000, -228.0533579629717735 ) ) ;
#16908=CARTESIAN_POINT ( 'NONE',  ( -5.836418080594380164, 30.19240250712089590, -223.8354869487762357 ) ) ;
#16909=CARTESIAN_POINT ( 'NONE',  ( 27.54521312182184545, 10.10774643363308023, -222.6232199463151744 ) ) ;
#16911=CARTESIAN_POINT ( 'NONE',  ( -12.75534255189586652, -28.05386989040209400, -226.4018635127162327 ) ) ;
#16913=CARTESIAN_POINT ( 'NONE',  ( -12.58820391453271093, -22.27128923838312247, -218.3899974299303324 ) ) ;
#16914=EDGE_CURVE ( 'NONE', #8796, #9103, #3923, .T. ) ;
#16915=CARTESIAN_POINT ( 'NONE',  ( -20.73319232323294514, 5.144688277016327582, -214.6391322078443977 ) ) ;
#16916=CARTESIAN_POINT ( 'NONE',  ( 6.589392574981438599, -17.08498810221841069, -232.9613445306918322 ) ) ;
#16917=CARTESIAN_POINT ( 'NONE',  ( -7.913358619554302642, 16.16796202616373890, -233.0981776325470491 ) ) ;
#16918=CARTESIAN_POINT ( 'NONE',  ( 15.45838063607522805, -1.173615160199915630, -230.4730353221563917 ) ) ;
#16919=CARTESIAN_POINT ( 'NONE',  ( -15.58529874627549461, -6.917566422457355202, -219.0138643999995054 ) ) ;
#16920=CARTESIAN_POINT ( 'NONE',  ( 12.23475091788960434, 6.342242864926500800, -221.9572581868331156 ) ) ;
#16922=CARTESIAN_POINT ( 'NONE',  ( -9.734169867326336600, 14.53420431798807755, -231.2442251076483046 ) ) ;
#16923=CARTESIAN_POINT ( 'NONE',  ( 14.87635807518583775, 11.13002414557121789, -232.1789382499626981 ) ) ;
#16924=CARTESIAN_POINT ( 'NONE',  ( 15.91295838535984331, 21.88410254487826379, -230.9583961155862823 ) ) ;
#16925=CARTESIAN_POINT ( 'NONE',  ( 11.35656094503625901, 14.01405796444069018, -230.6944611846958537 ) ) ;
#16926=CARTESIAN_POINT ( 'NONE',  ( 7.117641012966415381, -28.94820313438933113, -231.4073019955615393 ) ) ;
#16927=CARTESIAN_POINT ( 'NONE',  ( -9.852301241816233457, 15.10013604187968461, -230.8124578431014697 ) ) ;
#16928=CARTESIAN_POINT ( 'NONE',  ( -13.11494368899652052, 3.355507568391938200, -225.9121440085824304 ) ) ;
#16930=CARTESIAN_POINT ( 'NONE',  ( 25.18785298611088308, 3.974282393449815931, -218.7636041058819956 ) ) ;
#16931=CARTESIAN_POINT ( 'NONE',  ( 11.61478720377483675, -14.40087791365289860, -230.4552745109343448 ) ) ;
#16932=CARTESIAN_POINT ( 'NONE',  ( -26.11114532382342901, 12.73400870066318902, -227.7653936945517046 ) ) ;
#16933=CARTESIAN_POINT ( 'NONE',  ( 10.03842945413050458, 28.43460431997513638, -225.8374938385031214 ) ) ;
#16934=CARTESIAN_POINT ( 'NONE',  ( -22.51170993270524789, -14.32174306031543054, -231.7292175355062795 ) ) ;
#16936=CARTESIAN_POINT ( 'NONE',  ( -17.72669652144150376, 1.460525322529694581, -220.6883622781615202 ) ) ;
#16937=CARTESIAN_POINT ( 'NONE',  ( 11.84598249547323690, 10.36127485500543699, -218.5481300776139904 ) ) ;
#16939=CARTESIAN_POINT ( 'NONE',  ( 1.773982976645536835, 19.12448993322812285, -233.2315972735944172 ) ) ;
#16940=CARTESIAN_POINT ( 'NONE',  ( 11.86025528723659050, -11.55469215893994850, -227.5711990284272872 ) ) ;
#16941=CARTESIAN_POINT ( 'NONE',  ( 13.92699808111095905, -7.117895771238833547, -219.6066573659836081 ) ) ;
#16943=CARTESIAN_POINT ( 'NONE',  ( 5.343558017910363667, 26.29639771561252459, -218.1010331760174665 ) ) ;
#16944=CARTESIAN_POINT ( 'NONE',  ( -11.72787654052445028, -3.882995534642332824, -226.9210218758430244 ) ) ;
#16945=CARTESIAN_POINT ( 'NONE',  ( -15.17658589853145479, -26.64966442869902252, -226.8090782225333442 ) ) ;
#16946=CARTESIAN_POINT ( 'NONE',  ( 12.13827923251525220, -9.172799829723585319, -229.1860353116090891 ) ) ;
#16947=CARTESIAN_POINT ( 'NONE',  ( -14.60180519431160917, 24.46340507526420893, -221.8423643191928534 ) ) ;
#16948=CARTESIAN_POINT ( 'NONE',  ( 5.446894657575932719, 15.00061806465251557, -226.4498309983864317 ) ) ;
#16949=CARTESIAN_POINT ( 'NONE',  ( -20.18153419852512442, 14.25141268122526483, -233.5059133483111964 ) ) ;
#16950=CARTESIAN_POINT ( 'NONE',  ( -27.40681729237160269, 15.04232492504307572, -225.3323746796125704 ) ) ;
#16951=CARTESIAN_POINT ( 'NONE',  ( -14.73475970555713310, -4.645830632990214148, -227.0446463473171832 ) ) ;
#16952=ADVANCED_FACE ( 'NONE', ( #9882 ), #16520, .F. ) ;
#16953=CARTESIAN_POINT ( 'NONE',  ( -4.386767007475907754, 14.39570986262862107, -223.2690175027443615 ) ) ;
#16954=CARTESIAN_POINT ( 'NONE',  ( 12.81769551943392393, 4.437328497131001193, -221.7762769673541072 ) ) ;
#16955=CARTESIAN_POINT ( 'NONE',  ( 18.26039090677515375, 26.14311541888654844, -228.1864986152887127 ) ) ;
#16956=CARTESIAN_POINT ( 'NONE',  ( 11.20610455198612598, -10.15455062626793037, -220.8168162286965526 ) ) ;
#16959=CARTESIAN_POINT ( 'NONE',  ( -17.79285498209129202, 9.187865686019035749, -216.3798185811636756 ) ) ;
#16960=CARTESIAN_POINT ( 'NONE',  ( -9.654146510541638193, -9.431978497097317060, -229.7352898675592314 ) ) ;
#16962=CARTESIAN_POINT ( 'NONE',  ( 17.43816562714825125, 15.15720016074785903, -232.3748236813696906 ) ) ;
#16964=CARTESIAN_POINT ( 'NONE',  ( 22.44368505003003378, -11.72633196808685163, -232.1179326287041533 ) ) ;
#16965=CARTESIAN_POINT ( 'NONE',  ( -13.65925618638770800, 3.289586759644148817, -222.1579143493116533 ) ) ;
#16967=CARTESIAN_POINT ( 'NONE',  ( 16.40130693394614525, -0.1574073183566240264, -221.9481963320051534 ) ) ;
#16968=CARTESIAN_POINT ( 'NONE',  ( -1.097449620509919788, -25.21235133823365260, -218.6697740411501059 ) ) ;
#16971=CARTESIAN_POINT ( 'NONE',  ( 20.89184612657454920, 5.404957034965973683, -232.0952743654565609 ) ) ;
#16972=CARTESIAN_POINT ( 'NONE',  ( -18.71530386740073126, -0.6857509888707814527, -217.6195632122020527 ) ) ;
#16973=CARTESIAN_POINT ( 'NONE',  ( 11.03497432892593721, -13.14185978141811972, -229.3300340223075011 ) ) ;
#16974=CARTESIAN_POINT ( 'NONE',  ( 12.90817018730756516, -2.541983760742972720, -223.3958483567685391 ) ) ;
#16976=CARTESIAN_POINT ( 'NONE',  ( 10.64724148863252395, 12.28344647332184181, -223.6549461381946173 ) ) ;
#16978=CARTESIAN_POINT ( 'NONE',  ( 5.446894657575932719, 15.00061806465251557, -226.4498309983864317 ) ) ;
#16979=CARTESIAN_POINT ( 'NONE',  ( 9.181101971147782592, -9.127577137574531818, -229.3209091633710273 ) ) ;
#16980=CARTESIAN_POINT ( 'NONE',  ( 11.39114332821395692, -8.257479203742953189, -226.5648397932267528 ) ) ;
#16982=CARTESIAN_POINT ( 'NONE',  ( -20.47640197314466093, 18.50423766437512541, -220.4440130802851456 ) ) ;
#16983=CARTESIAN_POINT ( 'NONE',  ( -16.27736488614644372, 5.941157768540612949, -228.4237983497913547 ) ) ;
#16984=CARTESIAN_POINT ( 'NONE',  ( 13.72034832542693827, 10.98995328009155692, -220.6189139471235592 ) ) ;
#16985=ORIENTED_EDGE ( 'NONE', *, *, #4161, .T. ) ;
#16986=CARTESIAN_POINT ( 'NONE',  ( -3.821460206879919941, -14.75247343660110921, -225.5705290259156470 ) ) ;
#16988=CARTESIAN_POINT ( 'NONE',  ( 22.03647168420945590, 0.3315607655625663064, -232.0572713672586644 ) ) ;
#16990=CARTESIAN_POINT ( 'NONE',  ( 15.88965480228581839, 12.37830464553330678, -233.8570207506254235 ) ) ;
#16991=CARTESIAN_POINT ( 'NONE',  ( 12.68099841568652764, -20.61692530233158394, -230.4218470428317573 ) ) ;
#16992=CARTESIAN_POINT ( 'NONE',  ( 4.354034006296288339, 14.09944204372416188, -221.2519525881239417 ) ) ;
#16993=CARTESIAN_POINT ( 'NONE',  ( -16.15126510923403202, -0.4755054218165427615, -219.3066569788202571 ) ) ;
#16996=CARTESIAN_POINT ( 'NONE',  ( 25.41781277602550304, 19.49958712797920057, -223.1230538376805441 ) ) ;
#16997=CARTESIAN_POINT ( 'NONE',  ( -20.84243560023798736, 1.479777185913828230, -230.9766426496277631 ) ) ;
#16999=CARTESIAN_POINT ( 'NONE',  ( -7.825349071214003693, 24.14595706726266755, -216.5959661901539732 ) ) ;
#17000=CARTESIAN_POINT ( 'NONE',  ( 16.07305932912010960, 0.9253679043337685872, -229.0409936706996064 ) ) ;
#17001=CARTESIAN_POINT ( 'NONE',  ( 7.080148886126969465, -28.65852557119563926, -219.9679292432588227 ) ) ;
#17002=CARTESIAN_POINT ( 'NONE',  ( 27.02029988085337919, -0.4174685747284823112, -230.1188858631967378 ) ) ;
#17004=CARTESIAN_POINT ( 'NONE',  ( -14.37894460687751597, -1.926260335694933268, -225.0161641904981593 ) ) ;
#17005=CARTESIAN_POINT ( 'NONE',  ( 20.89184612657454920, 5.404957034965973683, -232.0952743654565609 ) ) ;
#17006=CARTESIAN_POINT ( 'NONE',  ( -19.26019478805205054, -16.72235099301716943, -219.5158537523224993 ) ) ;
#17011=CARTESIAN_POINT ( 'NONE',  ( 4.804712767000853368, -14.77773536573586455, -228.5128529893618747 ) ) ;
#17012=CARTESIAN_POINT ( 'NONE',  ( -21.28183200535960040, 1.085030287403131233, -217.0000000015322712 ) ) ;
#17013=CARTESIAN_POINT ( 'NONE',  ( -11.08731210905863840, 25.61052584666692766, -228.9953606804266997 ) ) ;
#17014=CARTESIAN_POINT ( 'NONE',  ( -4.450022810944913587, 12.45400981846350597, -225.2098051417536340 ) ) ;
#17016=CARTESIAN_POINT ( 'NONE',  ( 29.01190720243894461, 0.5135883731763817295, -231.9442528450179566 ) ) ;
#17018=CARTESIAN_POINT ( 'NONE',  ( 17.43816562714825125, 15.15720016074785903, -232.3748236813696906 ) ) ;
#17019=CARTESIAN_POINT ( 'NONE',  ( -21.01482965301294925, 6.368220028842532798, -231.7530032521518990 ) ) ;
#17020=CARTESIAN_POINT ( 'NONE',  ( -20.67624351032310059, -0.8683020119106035217, -219.0957770725675005 ) ) ;
#17022=CARTESIAN_POINT ( 'NONE',  ( 12.08198696763335178, 15.54678077493410981, -216.6084679670902631 ) ) ;
#17024=CARTESIAN_POINT ( 'NONE',  ( -20.21481434941064848, 7.972326285609216967, -230.8475376972877484 ) ) ;
#17026=CARTESIAN_POINT ( 'NONE',  ( -0.1452471002967452851, 24.29564289358754081, -234.0861481044164805 ) ) ;
#17027=CARTESIAN_POINT ( 'NONE',  ( 14.64440749032966593, 2.523901497798496596, -225.4572725674553340 ) ) ;
#17028=CARTESIAN_POINT ( 'NONE',  ( -13.40300228573463848, -19.05792172404923690, -234.2100255530988306 ) ) ;
#17030=CARTESIAN_POINT ( 'NONE',  ( -12.35609710479046441, -10.83622032031252758, -230.4552079900997228 ) ) ;
#17031=CARTESIAN_POINT ( 'NONE',  ( -14.70339349403010942, -0.4153334646997780544, -217.8790668391084466 ) ) ;
#17032=CARTESIAN_POINT ( 'NONE',  ( 4.682724365302521896, -22.35092628325669750, -215.9543778044225348 ) ) ;
#17033=CARTESIAN_POINT ( 'NONE',  ( -3.501680520304516264, 14.31538576447642264, -219.8967178229432307 ) ) ;
#17034=CARTESIAN_POINT ( 'NONE',  ( 25.70000612522241568, -7.596455516557234944, -216.8500112287931074 ) ) ;
#17035=CARTESIAN_POINT ( 'NONE',  ( -25.95884575339096401, -1.972114683626720044, -231.2145524501483749 ) ) ;
#17036=CARTESIAN_POINT ( 'NONE',  ( 13.25330606581809789, 10.40242132629824034, -230.9170765704288044 ) ) ;
#17038=CARTESIAN_POINT ( 'NONE',  ( -16.90193019167508126, 18.45790510038867893, -217.5707532411249758 ) ) ;
#17039=CARTESIAN_POINT ( 'NONE',  ( 17.98704291748025952, 16.14142602298251461, -217.3684083235702644 ) ) ;
#17040=CARTESIAN_POINT ( 'NONE',  ( 7.743212835174657194, 11.90778931056080481, -226.0491028376908105 ) ) ;
#17041=CARTESIAN_POINT ( 'NONE',  ( 15.28499842775873319, 22.98894588155567931, -221.0942409093412095 ) ) ;
#17042=CARTESIAN_POINT ( 'NONE',  ( 4.248462565232024701, -14.07263755978623188, -232.0081791469470716 ) ) ;
#17044=CARTESIAN_POINT ( 'NONE',  ( -6.388048297418547961, 21.92257289597608150, -233.3290245341164848 ) ) ;
#17045=CARTESIAN_POINT ( 'NONE',  ( 16.91879448796214191, 0.8271603773820436212, -230.0510230802265710 ) ) ;
#17046=CARTESIAN_POINT ( 'NONE',  ( 4.150966869518468272, -13.66845483776041092, -221.7292245539943565 ) ) ;
#17047=CARTESIAN_POINT ( 'NONE',  ( -19.65084584916038324, 18.01805631773661176, -219.5040736310571106 ) ) ;
#17048=CARTESIAN_POINT ( 'NONE',  ( 2.703362520412529779, 29.60004130108520215, -225.6165589735000481 ) ) ;
#17049=CARTESIAN_POINT ( 'NONE',  ( -21.52428768452188734, -21.65989873160339840, -225.4304055049964006 ) ) ;
#17050=CARTESIAN_POINT ( 'NONE',  ( 21.04928763009552384, -0.2309942901367783852, -233.9427286327411366 ) ) ;
#17051=CARTESIAN_POINT ( 'NONE',  ( 11.41911493375616260, 8.796695304819765582, -229.7440655656592412 ) ) ;
#17053=CARTESIAN_POINT ( 'NONE',  ( 14.39473142419577023, 15.98257177912839389, -217.4557725731239373 ) ) ;
#17054=CARTESIAN_POINT ( 'NONE',  ( 26.09199240421564880, -11.03603815124446186, -222.0211821522591435 ) ) ;
#17055=CARTESIAN_POINT ( 'NONE',  ( 18.79106389458910442, -5.302521403133691358, -233.5021979784848440 ) ) ;
#17058=CARTESIAN_POINT ( 'NONE',  ( -3.205260335674071648, 17.52234722004434531, -232.9754319808710363 ) ) ;
#17059=CARTESIAN_POINT ( 'NONE',  ( -23.85689329484546661, -4.322701801676343436, -216.0188046937498996 ) ) ;
#17060=CARTESIAN_POINT ( 'NONE',  ( -10.42804209284631156, -14.08702332024887305, -217.7386024361820489 ) ) ;
#17061=CARTESIAN_POINT ( 'NONE',  ( 11.78320976064766690, -8.193118641535518165, -222.2581747538435479 ) ) ;
#17062=CARTESIAN_POINT ( 'NONE',  ( -12.67136363292824086, 22.56975222910433843, -219.0840033572168011 ) ) ;
#17063=CARTESIAN_POINT ( 'NONE',  ( 10.01015180241662605, 20.19019600914695900, -219.1042218506083543 ) ) ;
#17064=CARTESIAN_POINT ( 'NONE',  ( -21.93900267957129557, 7.862893636934532360, -233.4951761057262161 ) ) ;
#17065=CARTESIAN_POINT ( 'NONE',  ( -28.99982533490676317, 5.894721259135065949, -231.5937499788843468 ) ) ;
#17066=CARTESIAN_POINT ( 'NONE',  ( -21.38043581477633026, -15.61850963832630335, -229.1016256230698502 ) ) ;
#17067=CARTESIAN_POINT ( 'NONE',  ( -12.67219131930435694, 19.52425521811199971, -218.0046184995277372 ) ) ;
#17068=CARTESIAN_POINT ( 'NONE',  ( 23.21336156720804667, 12.57464006230432574, -232.9346648124233070 ) ) ;
#17069=CARTESIAN_POINT ( 'NONE',  ( 22.92330650806121639, 19.11387742755395180, -231.6463539987045976 ) ) ;
#17070=CARTESIAN_POINT ( 'NONE',  ( 24.14841045621385263, -15.62485098017456586, -229.9279278555176518 ) ) ;
#17073=CARTESIAN_POINT ( 'NONE',  ( -1.249406995060579062, 25.48934319316224162, -216.9406480707515072 ) ) ;
#17074=CARTESIAN_POINT ( 'NONE',  ( -26.26363215285178043, -18.18116807333735352, -227.1727963224598739 ) ) ;
#17077=CARTESIAN_POINT ( 'NONE',  ( 22.66390650824515873, 11.48342577402021725, -231.3155567808436217 ) ) ;
#17078=CARTESIAN_POINT ( 'NONE',  ( -21.89482327431018760, 1.733733432562314158, -233.1353281693111796 ) ) ;
#17079=CARTESIAN_POINT ( 'NONE',  ( 10.99893791904045415, -12.61823049403341201, -218.3266956685045841 ) ) ;
#17081=CARTESIAN_POINT ( 'NONE',  ( -26.58771759052039485, 5.114955214121561511, -218.2823714869195442 ) ) ;
#17082=CARTESIAN_POINT ( 'NONE',  ( 27.08994772491946890, 9.675875910685000747, -221.3471992134593336 ) ) ;
#17084=CARTESIAN_POINT ( 'NONE',  ( -1.544051355262263225, -15.46116467022245011, -222.0171457641791903 ) ) ;
#17086=CARTESIAN_POINT ( 'NONE',  ( 28.02123297569005089, 5.903198806000402143, -227.5759114383273811 ) ) ;
#17087=CARTESIAN_POINT ( 'NONE',  ( -18.46722752239034193, 0.9784074152395518809, -232.1633353206286188 ) ) ;
#17088=CARTESIAN_POINT ( 'NONE',  ( 15.36293661829273027, -24.44941682316833464, -223.0188286856611626 ) ) ;
#17089=CARTESIAN_POINT ( 'NONE',  ( -24.76115377241536208, -2.015397159694146456, -231.8500816169410825 ) ) ;
#17091=CARTESIAN_POINT ( 'NONE',  ( 8.312165662451315384, 13.84431584962456974, -225.8109542921768025 ) ) ;
#17092=CARTESIAN_POINT ( 'NONE',  ( 9.132190541728901323, 17.73033835127231939, -219.5524510795130766 ) ) ;
#17093=CARTESIAN_POINT ( 'NONE',  ( 11.73142668431994018, -22.53166313379442443, -233.8575593048731491 ) ) ;
#17094=AXIS2_PLACEMENT_3D ( 'NONE', #20240, #12047, #13629 ) ;
#17095=CARTESIAN_POINT ( 'NONE',  ( 10.30328786010431052, -20.08430705480546408, -216.1847100135515802 ) ) ;
#17097=CARTESIAN_POINT ( 'NONE',  ( -12.05423124486310904, 12.38527783110887803, -219.7419643105747014 ) ) ;
#17098=CARTESIAN_POINT ( 'NONE',  ( -26.87016840655871874, 6.086699737350822481, -222.9228935003981746 ) ) ;
#17099=CARTESIAN_POINT ( 'NONE',  ( 14.02802030611117878, 3.063901161068346646, -225.6350222114233475 ) ) ;
#17100=CARTESIAN_POINT ( 'NONE',  ( -13.83311471749147259, -24.17028674860418747, -226.2550113133487173 ) ) ;
#17103=CARTESIAN_POINT ( 'NONE',  ( 14.64440749032966593, 2.523901497798496596, -225.4572725674553340 ) ) ;
#17104=CARTESIAN_POINT ( 'NONE',  ( 17.47462908134004422, -13.97354901070533906, -218.8807045398700666 ) ) ;
#17105=CARTESIAN_POINT ( 'NONE',  ( 13.43170911749896490, 19.07691563292472026, -232.7497845103644636 ) ) ;
#17106=CARTESIAN_POINT ( 'NONE',  ( -6.101488798441174310, 11.33371047077072369, -225.3616985956418546 ) ) ;
#17107=CARTESIAN_POINT ( 'NONE',  ( 10.22554538262735413, 24.20440706210576209, -215.6176527921760737 ) ) ;
#17110=CARTESIAN_POINT ( 'NONE',  ( -9.747505956077446854, 15.39125695327449783, -233.2799778227147840 ) ) ;
#17111=CARTESIAN_POINT ( 'NONE',  ( -3.326157069579807946, 13.92020081821418565, -220.5733722327383930 ) ) ;
#17112=CARTESIAN_POINT ( 'NONE',  ( 21.31262902390056624, 0.4111834581965390645, -232.0572713672585792 ) ) ;
#17113=CARTESIAN_POINT ( 'NONE',  ( 7.088126259304779353, -19.25156530781288566, -233.7785425911077937 ) ) ;
#17114=CARTESIAN_POINT ( 'NONE',  ( 24.21331552874348958, 0.07051084380047288602, -231.7986140076958463 ) ) ;
#17116=CARTESIAN_POINT ( 'NONE',  ( -28.55814054826834791, -1.660722980825670048, -228.2640858091212408 ) ) ;
#17117=CARTESIAN_POINT ( 'NONE',  ( -13.06407726305387307, 3.888674610242962348, -219.0371145420960204 ) ) ;
#17118=CARTESIAN_POINT ( 'NONE',  ( -13.04844958635619001, -9.307545681632840129, -223.5508123433884009 ) ) ;
#17119=CARTESIAN_POINT ( 'NONE',  ( 1.304950495335150507, -16.28913491483048759, -229.3926418476436027 ) ) ;
#17121=CARTESIAN_POINT ( 'NONE',  ( -14.06164063153489252, 2.050767714179807744, -227.2881998904968270 ) ) ;
#17122=CARTESIAN_POINT ( 'NONE',  ( -3.494873682963683059, 27.70407912598904687, -220.5214894769905243 ) ) ;
#17123=CARTESIAN_POINT ( 'NONE',  ( -9.350291727197115321, 27.53754332352430367, -230.1504993026967441 ) ) ;
#17125=CARTESIAN_POINT ( 'NONE',  ( 11.78812147976811175, -1.482036947660514636, -224.5790252820172270 ) ) ;
#17128=CARTESIAN_POINT ( 'NONE',  ( 21.25094435758043332, 17.68230636442804027, -229.7964888993842010 ) ) ;
#17129=CARTESIAN_POINT ( 'NONE',  ( -21.16281446184100545, 3.810576631694648775, -218.4455094643457187 ) ) ;
#17130=CARTESIAN_POINT ( 'NONE',  ( -26.91858181626453472, 10.72837452931393187, -223.4556356000267670 ) ) ;
#17131=CARTESIAN_POINT ( 'NONE',  ( -7.872599071444734697, -12.17161831996831367, -225.5779045487515191 ) ) ;
#17133=LINE ( 'NONE', #20480, #119 ) ;
#17134=CARTESIAN_POINT ( 'NONE',  ( 17.23498165643884761, 6.576565757823654934, -216.5785374982484655 ) ) ;
#17135=CARTESIAN_POINT ( 'NONE',  ( -25.17056316833229701, 11.10725809642625705, -227.0225660235207386 ) ) ;
#17136=CARTESIAN_POINT ( 'NONE',  ( 11.21112214669106777, 5.418350954422431975, -227.6539796508718325 ) ) ;
#17137=CARTESIAN_POINT ( 'NONE',  ( 23.04342321161690776, 14.90264581583150694, -218.4777833225197412 ) ) ;
#17138=CARTESIAN_POINT ( 'NONE',  ( -7.243062456665192883, -20.67674855546218637, -233.5126394780404553 ) ) ;
#17140=CARTESIAN_POINT ( 'NONE',  ( -10.73077095140340376, -23.14408218571897891, -231.4559151628563995 ) ) ;
#17141=CARTESIAN_POINT ( 'NONE',  ( -4.558896566524145655, 13.01459016691503301, -228.3167740496058684 ) ) ;
#17142=CARTESIAN_POINT ( 'NONE',  ( 3.342529885312644833, -17.78621320651278737, -216.7788622297345853 ) ) ;
#17143=CARTESIAN_POINT ( 'NONE',  ( 0.9908753270255351575, 13.79205759140780430, -228.0165926715089881 ) ) ;
#17144=CARTESIAN_POINT ( 'NONE',  ( 24.23593707391374608, -4.329230177290460446, -233.5551557188744312 ) ) ;
#17145=CARTESIAN_POINT ( 'NONE',  ( -25.42089018817326007, -6.263968923056941307, -218.6542964065910439 ) ) ;
#17146=CARTESIAN_POINT ( 'NONE',  ( 26.06405806384012536, 5.488112530166501024, -216.5020692413490622 ) ) ;
#17148=CARTESIAN_POINT ( 'NONE',  ( -6.067446494494625142, 16.28408815813367028, -230.0786439517394513 ) ) ;
#17149=CARTESIAN_POINT ( 'NONE',  ( 15.14859676485869500, 2.119979922547468032, -231.9009926880791284 ) ) ;
#17150=CARTESIAN_POINT ( 'NONE',  ( 17.97843143658897347, 22.12221935793617078, -220.9346589834416079 ) ) ;
#17151=CARTESIAN_POINT ( 'NONE',  ( 29.47107563651793427, 6.731311671946880182, -220.0565342412898815 ) ) ;
#17152=CARTESIAN_POINT ( 'NONE',  ( -1.232290808404003624, -30.06229647885771428, -229.8325228448912583 ) ) ;
#17153=CARTESIAN_POINT ( 'NONE',  ( 5.434119414999338815, 11.18343085245738777, -221.0450680983404936 ) ) ;
#17156=CARTESIAN_POINT ( 'NONE',  ( 7.896007729111394369, -13.22437314876957437, -221.6501328817743683 ) ) ;
#17157=CARTESIAN_POINT ( 'NONE',  ( -15.30295614572244922, 9.661125001905515930, -218.8475896279880146 ) ) ;
#17158=CARTESIAN_POINT ( 'NONE',  ( 3.312424284731937618, 15.29837714273186045, -229.5209971419123747 ) ) ;
#17159=CARTESIAN_POINT ( 'NONE',  ( -16.39524763169126942, -10.97410814576847926, -232.9630882351523837 ) ) ;
#17160=CARTESIAN_POINT ( 'NONE',  ( 15.39025625686376841, 1.044190007782545226, -218.9203249718910911 ) ) ;
#17161=CARTESIAN_POINT ( 'NONE',  ( 10.39636392256998221, 18.46527700675686035, -215.1860221565626148 ) ) ;
#17162=CARTESIAN_POINT ( 'NONE',  ( 8.979547488457603421, 23.24376652602565230, -232.6628827740196357 ) ) ;
#17163=CARTESIAN_POINT ( 'NONE',  ( 16.48523685932656235, -13.39871719616043855, -218.9387417542926926 ) ) ;
#17164=CARTESIAN_POINT ( 'NONE',  ( 10.62272209279942992, -9.818939940036045755, -222.1403336352628344 ) ) ;
#17165=CARTESIAN_POINT ( 'NONE',  ( 13.43170911749896490, 19.07691563292472026, -232.7497845103644636 ) ) ;
#17166=CARTESIAN_POINT ( 'NONE',  ( -25.41475252190474521, -13.58614899836300260, -217.5872217295323310 ) ) ;
#17167=CARTESIAN_POINT ( 'NONE',  ( -9.625604265899946554, -19.21123364792547505, -233.9327940972253259 ) ) ;
#17168=CARTESIAN_POINT ( 'NONE',  ( 12.70477135646371281, -9.814387909761604689, -230.3443492180780652 ) ) ;
#17169=CARTESIAN_POINT ( 'NONE',  ( -10.46043650402819125, 8.998596506756641134, -222.4402691847174083 ) ) ;
#17170=CARTESIAN_POINT ( 'NONE',  ( 27.94758519801750296, 7.894658480667867018, -227.3974864124137127 ) ) ;
#17172=CARTESIAN_POINT ( 'NONE',  ( -14.70651859537745487, 4.211702956367679107, -230.0357207626005334 ) ) ;
#17173=CARTESIAN_POINT ( 'NONE',  ( -9.734169867326336600, 14.53420431798807755, -231.2442251076483046 ) ) ;
#17174=CARTESIAN_POINT ( 'NONE',  ( 21.85730963248023428, -9.423385237436111339, -216.6089804361807580 ) ) ;
#17176=CARTESIAN_POINT ( 'NONE',  ( -5.775873073292457249, 17.47547275616994256, -218.7209647771908578 ) ) ;
#17177=CARTESIAN_POINT ( 'NONE',  ( 27.13894094332088969, 12.30518789341946295, -220.2765066586875093 ) ) ;
#17178=CARTESIAN_POINT ( 'NONE',  ( 10.02118533929671074, 10.65166262057242008, -217.7534731326719566 ) ) ;
#17179=CARTESIAN_POINT ( 'NONE',  ( 25.90657540470570197, -10.31326923046670885, -218.6707845005603019 ) ) ;
#17182=CARTESIAN_POINT ( 'NONE',  ( -0.3969026096611234511, 20.89748314411456676, -216.3289738411752978 ) ) ;
#17183=CARTESIAN_POINT ( 'NONE',  ( -12.58473846644578664, -2.158129970029659006, -220.6199603830026206 ) ) ;
#17185=CARTESIAN_POINT ( 'NONE',  ( 14.85123888640019452, 5.067529763532427012, -221.9058491819374979 ) ) ;
#17186=CARTESIAN_POINT ( 'NONE',  ( -15.15110768032078070, 3.517015312212880218, -219.5479300368539270 ) ) ;
#17187=CARTESIAN_POINT ( 'NONE',  ( 25.83609367470520723, -15.13481494965009411, -225.4685613576401124 ) ) ;
#17188=CARTESIAN_POINT ( 'NONE',  ( -20.94800339253696109, 4.477632454355491731, -216.5423208360950298 ) ) ;
#17189=CARTESIAN_POINT ( 'NONE',  ( -22.47200958260654957, 4.697452857301940732, -216.5879371680706242 ) ) ;
#17190=CARTESIAN_POINT ( 'NONE',  ( -5.322766963623397629, -16.65786661440869665, -219.3972027188067671 ) ) ;
#17193=CARTESIAN_POINT ( 'NONE',  ( -19.25929423112888017, 9.818144317380269825, -216.1837936240308409 ) ) ;
#17194=CARTESIAN_POINT ( 'NONE',  ( 16.20395612672116314, -10.90071921976151081, -219.5016540749954856 ) ) ;
#17195=CARTESIAN_POINT ( 'NONE',  ( -28.42127686227592420, -0.6461176296494712812, -221.6028628238154567 ) ) ;
#17198=CARTESIAN_POINT ( 'NONE',  ( 16.07044873961816123, 22.39643131523411412, -226.8512752114033901 ) ) ;
#17200=CARTESIAN_POINT ( 'NONE',  ( 5.104697752190542559, 17.18208638613223016, -220.3923334988619445 ) ) ;
#17201=CARTESIAN_POINT ( 'NONE',  ( -3.424405916006480144, -18.03457810294644403, -219.2650390415759318 ) ) ;
#17202=CARTESIAN_POINT ( 'NONE',  ( 19.88636028791461641, -20.85574262981397453, -219.9907771812986823 ) ) ;
#17204=CARTESIAN_POINT ( 'NONE',  ( -18.94992041651601156, 14.87246523864368974, -232.0280096192260828 ) ) ;
#17205=CARTESIAN_POINT ( 'NONE',  ( -24.82235633397527508, 10.76243500821901300, -227.9886044494091948 ) ) ;
#17206=CARTESIAN_POINT ( 'NONE',  ( -18.09994298044773942, 1.383435435878707320, -215.7801353739235708 ) ) ;
#17207=CARTESIAN_POINT ( 'NONE',  ( -2.278185930139247084, -29.13041568434719863, -223.8160414879089046 ) ) ;
#17210=CARTESIAN_POINT ( 'NONE',  ( 25.70381634773192658, 10.55338509461953400, -230.3576492130207782 ) ) ;
#17211=CARTESIAN_POINT ( 'NONE',  ( 13.43173494629961517, -24.23096015178613172, -223.5315588962966160 ) ) ;
#17212=CARTESIAN_POINT ( 'NONE',  ( 2.837900457371055563, 25.11342719071438978, -232.9871906064174709 ) ) ;
#17213=CARTESIAN_POINT ( 'NONE',  ( -22.17339560624464312, 16.26550580028390769, -232.0582861498566274 ) ) ;
#17215=CARTESIAN_POINT ( 'NONE',  ( 10.90540179105271967, 5.382827416078996841, -224.1493061458977820 ) ) ;
#17216=CARTESIAN_POINT ( 'NONE',  ( 11.13678936984666912, 26.95732789089726111, -228.8350761760834757 ) ) ;
#17218=CARTESIAN_POINT ( 'NONE',  ( -1.489322793389167288, -21.37773154815333498, -215.8826219457350817 ) ) ;
#17219=CARTESIAN_POINT ( 'NONE',  ( 14.98777556431132219, -10.10815648641214004, -217.9795565018743844 ) ) ;
#17221=CARTESIAN_POINT ( 'NONE',  ( -3.400000000000003908, 0.000000000000000000, -224.9999999999999716 ) ) ;
#17222=CARTESIAN_POINT ( 'NONE',  ( 28.57344184061583192, 5.631897254180425527, -225.1192013637692355 ) ) ;
#17223=CARTESIAN_POINT ( 'NONE',  ( -13.57658210113775432, -10.11812981318216131, -221.5438341886276987 ) ) ;
#17224=CARTESIAN_POINT ( 'NONE',  ( 6.250374750423979719, -27.98416211894771521, -222.2453514702945085 ) ) ;
#17225=CARTESIAN_POINT ( 'NONE',  ( 15.14536540539411114, 2.907144070186200580, -217.8738854795238922 ) ) ;
#17226=CARTESIAN_POINT ( 'NONE',  ( 9.880827190695510964, 24.82036951119805579, -218.1633337467656020 ) ) ;
#17227=CARTESIAN_POINT ( 'NONE',  ( -7.352050649209116884, 10.05454564170545417, -223.7370967983176229 ) ) ;
#17229=CARTESIAN_POINT ( 'NONE',  ( -21.01940116658287749, -3.333607517048045032, -230.8803659671980597 ) ) ;
#17231=CARTESIAN_POINT ( 'NONE',  ( 22.02796522526679723, 16.41909032291435366, -220.1590600991317217 ) ) ;
#17233=CARTESIAN_POINT ( 'NONE',  ( -11.27928845652762213, 14.86256579634383002, -216.2427993537644966 ) ) ;
#17234=CARTESIAN_POINT ( 'NONE',  ( -15.12838653695630420, 3.161599240781852949, -225.7834014684609656 ) ) ;
#17235=CARTESIAN_POINT ( 'NONE',  ( -12.35609710479046441, -10.83622032031252758, -230.4552079900997228 ) ) ;
#17237=CARTESIAN_POINT ( 'NONE',  ( 27.69955354773053458, 12.81264626165819287, -221.7750850138309602 ) ) ;
#17238=CARTESIAN_POINT ( 'NONE',  ( -12.01777041390050726, 10.97692933293401474, -227.6853890888168053 ) ) ;
#17239=CARTESIAN_POINT ( 'NONE',  ( 11.75404126451729070, 5.688294280104953415, -229.3533586468489602 ) ) ;
#17240=CARTESIAN_POINT ( 'NONE',  ( 14.21126657910812874, 6.833562750302326627, -220.2783117037562874 ) ) ;
#17241=CARTESIAN_POINT ( 'NONE',  ( -10.76816654174163368, -5.786055782404167402, -221.6662823521482437 ) ) ;
#17243=CARTESIAN_POINT ( 'NONE',  ( -7.872599071444734697, -12.17161831996831367, -225.5779045487515191 ) ) ;
#17244=CARTESIAN_POINT ( 'NONE',  ( -16.89013823391154290, 26.38860451648245231, -225.6449744083545852 ) ) ;
#17245=CARTESIAN_POINT ( 'NONE',  ( 15.10937218716165020, -26.44221868192832758, -222.7999243300199907 ) ) ;
#17246=CARTESIAN_POINT ( 'NONE',  ( 1.773982976645536835, 19.12448993322812285, -233.2315972735944172 ) ) ;
#17247=CARTESIAN_POINT ( 'NONE',  ( 27.54866699188204748, -16.08959018098719085, -223.7550031907416326 ) ) ;
#17249=CARTESIAN_POINT ( 'NONE',  ( -25.44919589272258520, 4.740781954932180575, -232.0725131810460766 ) ) ;
#17251=CARTESIAN_POINT ( 'NONE',  ( -6.407569900110946293, 14.82357759665407215, -221.6203916094852957 ) ) ;
#17252=CARTESIAN_POINT ( 'NONE',  ( 14.19979467405507556, 6.351366891014061267, -230.8614099669030679 ) ) ;
#17253=CARTESIAN_POINT ( 'NONE',  ( 15.12287735332712835, 21.03907941686458116, -231.7894952627153202 ) ) ;
#17254=CARTESIAN_POINT ( 'NONE',  ( 12.89118769162836031, 6.140251663080722899, -228.8792332048833771 ) ) ;
#17255=CARTESIAN_POINT ( 'NONE',  ( 6.919598145955467849, -31.16410449029495311, -226.5345828574877487 ) ) ;
#17256=CARTESIAN_POINT ( 'NONE',  ( 10.86206282953156510, 30.27427353967719981, -226.0953027964478110 ) ) ;
#17257=CARTESIAN_POINT ( 'NONE',  ( 28.57344184061583192, 5.631897254180425527, -225.1192013637692355 ) ) ;
#17258=CARTESIAN_POINT ( 'NONE',  ( -0.3008257096753846893, -14.77709807386645480, -230.6673697011181048 ) ) ;
#17259=CARTESIAN_POINT ( 'NONE',  ( -10.32994309255856535, 16.55762392127841665, -218.3313395458419279 ) ) ;
#17260=CARTESIAN_POINT ( 'NONE',  ( -0.1881941282075867139, 17.37563936270229092, -230.9177995227891813 ) ) ;
#17261=CARTESIAN_POINT ( 'NONE',  ( -19.31342342724724759, -3.870051895940637365, -217.8584481481169348 ) ) ;
#17262=CARTESIAN_POINT ( 'NONE',  ( -19.72392517715239535, 13.50888179936880107, -230.7714862421596251 ) ) ;
#17264=CARTESIAN_POINT ( 'NONE',  ( -19.84402263676350131, 8.565754689849573111, -217.6561116767911983 ) ) ;
#17265=CARTESIAN_POINT ( 'NONE',  ( 15.46952826979347151, 3.173892190046953665, -221.7237849701489552 ) ) ;
#17267=CARTESIAN_POINT ( 'NONE',  ( 8.496844655769807630, 14.66037471857024599, -219.1631158796573118 ) ) ;
#17268=CARTESIAN_POINT ( 'NONE',  ( 14.78595257191855694, -4.705020206487795065, -221.9958499870062099 ) ) ;
#17269=CARTESIAN_POINT ( 'NONE',  ( 20.28526114930425450, -5.837089636085359245, -233.7994602772149051 ) ) ;
#17270=CARTESIAN_POINT ( 'NONE',  ( -2.612157044224189484, 27.88031182936952135, -224.5292183073761692 ) ) ;
#17272=CARTESIAN_POINT ( 'NONE',  ( 13.43730899468209294, 8.427513769504761498, -221.4030804848920297 ) ) ;
#17273=CARTESIAN_POINT ( 'NONE',  ( -13.21307282338718991, -4.958223064515467016, -219.4340824732878730 ) ) ;
#17274=CARTESIAN_POINT ( 'NONE',  ( -1.643553855084622928, -13.05119293000219294, -222.7191902239112551 ) ) ;
#17275=CARTESIAN_POINT ( 'NONE',  ( 21.53087031351596892, -21.03550532031109555, -227.1077645633325233 ) ) ;
#17276=CARTESIAN_POINT ( 'NONE',  ( 2.021807401899061496, 24.17554150923399092, -230.4042646614662146 ) ) ;
#17278=CARTESIAN_POINT ( 'NONE',  ( 14.73597170006453361, 7.272367905564328439, -221.0092474305599239 ) ) ;
#17279=CARTESIAN_POINT ( 'NONE',  ( -13.98136146596813845, 3.850743984385103680, -228.7620665878280590 ) ) ;
#17280=CARTESIAN_POINT ( 'NONE',  ( -15.05930145804884290, 24.78193219970826533, -223.0510781988847953 ) ) ;
#17281=CARTESIAN_POINT ( 'NONE',  ( 28.19769730429874599, -1.268543021275377658, -231.5188709829604363 ) ) ;
#17282=CARTESIAN_POINT ( 'NONE',  ( 2.630208337444488453, 16.40323635460054774, -219.2570070657488088 ) ) ;
#17283=CARTESIAN_POINT ( 'NONE',  ( -15.32935061426341861, 5.146212415319166844, -225.5669090095357774 ) ) ;
#17284=CARTESIAN_POINT ( 'NONE',  ( 7.359401564398577733, 15.81697286067417707, -215.8326977948377987 ) ) ;
#17285=CARTESIAN_POINT ( 'NONE',  ( 11.64632602964496044, -20.35392056169815689, -232.5450580586399383 ) ) ;
#17288=CARTESIAN_POINT ( 'NONE',  ( -2.735889804569492600, 12.71735652435744512, -225.1194195722198117 ) ) ;
#17289=CARTESIAN_POINT ( 'NONE',  ( -14.04855893775563125, -7.839533416607601168, -216.6740050463540115 ) ) ;
#17291=CARTESIAN_POINT ( 'NONE',  ( 20.23125423326388628, 7.836699765464857137, -217.8891354894872450 ) ) ;
#17292=CARTESIAN_POINT ( 'NONE',  ( -17.84981083811007707, 0.8485253248287054628, -231.8041300026935119 ) ) ;
#17293=CARTESIAN_POINT ( 'NONE',  ( 14.98777556431132219, -10.10815648641214004, -217.9795565018743844 ) ) ;
#17295=CARTESIAN_POINT ( 'NONE',  ( -9.716674560061926869, 27.56227806819028103, -219.4917914922789919 ) ) ;
#17296=CARTESIAN_POINT ( 'NONE',  ( -13.65925618638770800, 3.289586759644148817, -222.1579143493116533 ) ) ;
#17297=CARTESIAN_POINT ( 'NONE',  ( -4.253447013113726527, -22.64852647464574531, -232.0531923962242615 ) ) ;
#17300=CARTESIAN_POINT ( 'NONE',  ( -26.02440924314744919, 2.824604386891162111, -232.0644005296583430 ) ) ;
#17301=CARTESIAN_POINT ( 'NONE',  ( 14.02967383842077709, -23.07461891086659378, -219.7428183145782725 ) ) ;
#17302=CARTESIAN_POINT ( 'NONE',  ( 13.83657615971619848, -1.576202780126219949, -222.4470885262105639 ) ) ;
#17304=CARTESIAN_POINT ( 'NONE',  ( 17.02590609996173754, 6.796709046606974169, -230.8496778635019098 ) ) ;
#17305=CARTESIAN_POINT ( 'NONE',  ( -14.84124724799726991, 21.42277200659090042, -233.6300684249849553 ) ) ;
#17306=CARTESIAN_POINT ( 'NONE',  ( 14.66646255503707152, 18.43809875292740230, -219.3480462970252063 ) ) ;
#17307=CARTESIAN_POINT ( 'NONE',  ( -6.114698591673049854, -22.00309638965383030, -231.6969144128436540 ) ) ;
#17308=CARTESIAN_POINT ( 'NONE',  ( 16.48937362995332734, -6.768414299447169213, -233.6525893218997680 ) ) ;
#17311=CARTESIAN_POINT ( 'NONE',  ( 3.378648530876271039, 26.08525450992624428, -218.4319906442508454 ) ) ;
#17312=CARTESIAN_POINT ( 'NONE',  ( -20.21481434941064848, 7.972326285609216967, -230.8475376972877484 ) ) ;
#17313=CARTESIAN_POINT ( 'NONE',  ( -12.10179538005628963, 1.685214252672075030, -222.4835512146784424 ) ) ;
#17314=CARTESIAN_POINT ( 'NONE',  ( -14.04666385475200485, -11.54975518965215286, -229.4392169170632201 ) ) ;
#17317=CARTESIAN_POINT ( 'NONE',  ( 18.84307465506600465, 4.899879697440840509, -218.2189947030338715 ) ) ;
#17318=CARTESIAN_POINT ( 'NONE',  ( 18.63268865202281432, -19.94522792032704572, -227.6816033052257637 ) ) ;
#17319=CARTESIAN_POINT ( 'NONE',  ( 7.769483725421269860, 20.68783433326350263, -233.2348178266662728 ) ) ;
#17320=CARTESIAN_POINT ( 'NONE',  ( -11.98736441306973077, 11.45674391201457176, -217.8252237716743025 ) ) ;
#17322=CARTESIAN_POINT ( 'NONE',  ( 16.84354851290083133, 10.42424693870724361, -215.2582953371023109 ) ) ;
#17324=CARTESIAN_POINT ( 'NONE',  ( 10.85888002857596923, 15.81835858589122878, -232.3913150909872627 ) ) ;
#17326=CARTESIAN_POINT ( 'NONE',  ( 7.486336813247038258, -29.35413437595724773, -221.4114973598149447 ) ) ;
#17327=CARTESIAN_POINT ( 'NONE',  ( 21.05631363308661363, -21.50266115212419393, -222.6654548186096747 ) ) ;
#17330=CARTESIAN_POINT ( 'NONE',  ( -15.35982698007958724, 5.508237851081846159, -233.6994028941782631 ) ) ;
#17331=CARTESIAN_POINT ( 'NONE',  ( -27.59531865868800082, -2.367229732415436771, -222.8128998708299093 ) ) ;
#17332=CARTESIAN_POINT ( 'NONE',  ( -16.81936022032888545, 5.700806722825413786, -218.5726178058217215 ) ) ;
#17333=CARTESIAN_POINT ( 'NONE',  ( 1.656472371294090085, 27.29382523973669095, -230.4991099578876117 ) ) ;
#17334=CARTESIAN_POINT ( 'NONE',  ( 4.238595127209166868, 26.19205419861516404, -230.1142052665570077 ) ) ;
#17336=CARTESIAN_POINT ( 'NONE',  ( 31.06375291838557118, -1.327124779900562768, -220.7315133954257647 ) ) ;
#17338=CARTESIAN_POINT ( 'NONE',  ( 11.82943521288609823, 27.58963564415041247, -226.1180395413371400 ) ) ;
#17340=CARTESIAN_POINT ( 'NONE',  ( -13.48133478602219171, 10.24771958306113362, -218.3822527490931691 ) ) ;
#17341=CARTESIAN_POINT ( 'NONE',  ( -22.57859951143173660, 16.82392524473188899, -219.5628058978911383 ) ) ;
#17342=CARTESIAN_POINT ( 'NONE',  ( -24.09642229725868745, -17.04339013636034750, -228.1169379854252384 ) ) ;
#17346=CARTESIAN_POINT ( 'NONE',  ( 13.86459245677513330, 0.7513318449320793846, -221.1689395455950660 ) ) ;
#17347=CARTESIAN_POINT ( 'NONE',  ( -11.10144104376680652, 18.49675466419975578, -232.2931259015917647 ) ) ;
#17348=CARTESIAN_POINT ( 'NONE',  ( 18.99256614858759207, 26.22894869843687715, -224.5811130452664202 ) ) ;
#17349=CARTESIAN_POINT ( 'NONE',  ( -24.68906941503829700, 2.445024713909649705, -232.6803430500543755 ) ) ;
#17352=CARTESIAN_POINT ( 'NONE',  ( -23.71722460534674681, -17.39027245378339259, -231.9193655574418074 ) ) ;
#17354=CARTESIAN_POINT ( 'NONE',  ( -12.88620494227545343, -3.269292211592822461, -225.1464181993036391 ) ) ;
#17355=CARTESIAN_POINT ( 'NONE',  ( -8.523771322135640816, 24.09653697920728987, -233.1071395647740303 ) ) ;
#17356=CARTESIAN_POINT ( 'NONE',  ( -12.11864581566431553, -23.10742878804749978, -232.9192999331436909 ) ) ;
#17357=CARTESIAN_POINT ( 'NONE',  ( -6.282398543089500187, 12.01615879894893801, -228.5121145169883903 ) ) ;
#17358=CARTESIAN_POINT ( 'NONE',  ( 12.03076347463371398, -25.25364776008588308, -216.5688293904237298 ) ) ;
#17360=CARTESIAN_POINT ( 'NONE',  ( -17.43458823433387650, 2.804998135793385750, -231.8077100320880959 ) ) ;
#17362=CARTESIAN_POINT ( 'NONE',  ( -6.769588938507062004, 18.22485903270490937, -231.3660928915624879 ) ) ;
#17363=CARTESIAN_POINT ( 'NONE',  ( 25.30228294196351868, 7.987863777258004561, -233.0744943826964573 ) ) ;
#17364=CARTESIAN_POINT ( 'NONE',  ( 27.04607490430786854, 4.607450003618843049, -220.3758934308003461 ) ) ;
#17365=CARTESIAN_POINT ( 'NONE',  ( 25.30228294196351868, 7.987863777258004561, -233.0744943826964573 ) ) ;
#17366=CARTESIAN_POINT ( 'NONE',  ( 4.093437342195941575, -12.31737333437662940, -220.6844603446061512 ) ) ;
#17367=CARTESIAN_POINT ( 'NONE',  ( 11.13671218404335761, 30.21738803452449673, -224.2405745632392211 ) ) ;
#17370=CARTESIAN_POINT ( 'NONE',  ( 25.69300549816939494, 5.947472783069708946, -230.6131061331718115 ) ) ;
#17371=CARTESIAN_POINT ( 'NONE',  ( 0.3839640804239903837, -16.65388496721540790, -217.3312339551772823 ) ) ;
#17372=CARTESIAN_POINT ( 'NONE',  ( -11.16203726658389606, 26.27101666727781648, -227.8592829514190612 ) ) ;
#17373=CARTESIAN_POINT ( 'NONE',  ( 18.23116248274160256, 13.99874872632082123, -216.0593560670294835 ) ) ;
#17374=CARTESIAN_POINT ( 'NONE',  ( -25.95884575339096401, -1.972114683626720044, -231.2145524501483749 ) ) ;
#17375=CARTESIAN_POINT ( 'NONE',  ( -14.47418542577149836, 8.806675964858893479, -228.0010566307936699 ) ) ;
#17376=CARTESIAN_POINT ( 'NONE',  ( -0.8357710952364670876, 15.48480697989137234, -216.9118565312697910 ) ) ;
#17377=CARTESIAN_POINT ( 'NONE',  ( 15.33651282626308010, 7.807290788239344970, -218.6940806506825652 ) ) ;
#17380=CARTESIAN_POINT ( 'NONE',  ( 7.513872959756128012, -15.38293111518118295, -221.6143039513618760 ) ) ;
#17381=ORIENTED_EDGE ( 'NONE', *, *, #7048, .F. ) ;
#17382=CARTESIAN_POINT ( 'NONE',  ( 9.338484253624125486, -13.53666216847648052, -219.8958652322373837 ) ) ;
#17383=CARTESIAN_POINT ( 'NONE',  ( -8.791002657293931932, 17.82034842365333205, -218.5247019341474584 ) ) ;
#17386=CARTESIAN_POINT ( 'NONE',  ( 18.23324537670537993, 23.47692953258263771, -224.8333321331434433 ) ) ;
#17387=CARTESIAN_POINT ( 'NONE',  ( 25.54997870115619207, -2.097555195297153841, -218.7002440566220400 ) ) ;
#17388=CARTESIAN_POINT ( 'NONE',  ( -0.8413160509385254615, -28.71376977722865931, -218.8117683208458288 ) ) ;
#17390=CARTESIAN_POINT ( 'NONE',  ( -1.633632075387274840, -15.48245080501611071, -218.5193615163172751 ) ) ;
#17392=CARTESIAN_POINT ( 'NONE',  ( -7.928079932584687128, 26.12067226064367986, -221.2051195461628197 ) ) ;
#17394=CARTESIAN_POINT ( 'NONE',  ( 13.72034832542693827, 10.98995328009155692, -220.6189139471235592 ) ) ;
#17395=CARTESIAN_POINT ( 'NONE',  ( -19.25929423112888017, 9.818144317380269825, -216.1837936240308409 ) ) ;
#17396=CARTESIAN_POINT ( 'NONE',  ( -6.067446494494625142, 16.28408815813367028, -230.0786439517394513 ) ) ;
#17397=CARTESIAN_POINT ( 'NONE',  ( 2.893760225568064115, 14.39521026618305477, -227.6654023557511550 ) ) ;
#17398=CARTESIAN_POINT ( 'NONE',  ( -21.47149190714903710, 3.672831083387290363, -231.0833634068433469 ) ) ;
#17399=CARTESIAN_POINT ( 'NONE',  ( 9.168912942254459963, 16.03578711007639157, -234.6923200900793347 ) ) ;
#17401=CARTESIAN_POINT ( 'NONE',  ( 7.876378987416962296, -12.17572650474792617, -223.4643623724329018 ) ) ;
#17404=CARTESIAN_POINT ( 'NONE',  ( 0.9046320824004248085, 13.39785254849979701, -226.4815711199935890 ) ) ;
#17406=CARTESIAN_POINT ( 'NONE',  ( 18.18465861704851960, -5.084991117879029687, -230.0453011691623999 ) ) ;
#17407=CARTESIAN_POINT ( 'NONE',  ( 19.06763123184207487, -2.048228142369658666, -218.2337357994572073 ) ) ;
#17408=CARTESIAN_POINT ( 'NONE',  ( 28.02123297569005089, 5.903198806000402143, -227.5759114383273811 ) ) ;
#17411=CARTESIAN_POINT ( 'NONE',  ( 2.967317674205219191, -16.40215926535219282, -217.6245344443522924 ) ) ;
#17413=CARTESIAN_POINT ( 'NONE',  ( -9.171998067665157350, 9.395241133357435714, -226.3428046914542051 ) ) ;
#17416=CARTESIAN_POINT ( 'NONE',  ( -21.08008464085897060, -0.9048411197481797119, -217.0000000010748522 ) ) ;
#17417=CARTESIAN_POINT ( 'NONE',  ( -8.465333986790207987, -12.59497810381903982, -228.1424919783533198 ) ) ;
#17420=CARTESIAN_POINT ( 'NONE',  ( -14.70651859537745487, 4.211702956367679107, -230.0357207626005334 ) ) ;
#17421=CARTESIAN_POINT ( 'NONE',  ( 20.16749130626988773, -19.72590806003585229, -223.0880382675181579 ) ) ;
#17422=CARTESIAN_POINT ( 'NONE',  ( 14.88131340536105718, -1.788773220640928807, -222.5905533966261203 ) ) ;
#17424=CARTESIAN_POINT ( 'NONE',  ( 13.71585692689473213, 6.523039003617190801, -224.4540437369149402 ) ) ;
#17425=CARTESIAN_POINT ( 'NONE',  ( -9.722597143579921664, 7.159547510896417499, -227.5730737101346222 ) ) ;
#17427=CARTESIAN_POINT ( 'NONE',  ( 12.91443243054181700, 13.28840485332751875, -229.6651346406987955 ) ) ;
#17428=CARTESIAN_POINT ( 'NONE',  ( -0.6911605129178206575, -19.14003671809244267, -232.0914249810984131 ) ) ;
#17429=CARTESIAN_POINT ( 'NONE',  ( 15.45838063607522805, -1.173615160199915630, -230.4730353221563917 ) ) ;
#17431=CARTESIAN_POINT ( 'NONE',  ( -10.23029362138610843, 26.44342627367518617, -221.6879936327511871 ) ) ;
#17432=CARTESIAN_POINT ( 'NONE',  ( -22.53796032816233463, 16.84148256071415872, -226.0516062466300582 ) ) ;
#17433=CARTESIAN_POINT ( 'NONE',  ( -28.99982533490676317, 5.894721259135065949, -231.5937499788843468 ) ) ;
#17435=CARTESIAN_POINT ( 'NONE',  ( -15.55375487336196372, -9.676988738288478942, -219.9111427047364202 ) ) ;
#17438=CARTESIAN_POINT ( 'NONE',  ( 27.54521312182184545, 10.10774643363308023, -222.6232199463151744 ) ) ;
#17439=CARTESIAN_POINT ( 'NONE',  ( 2.435323595375026073, -28.08909517487921192, -228.1503986837488469 ) ) ;
#17440=CARTESIAN_POINT ( 'NONE',  ( 19.19288224840068935, 10.13059690604263174, -232.1906135022504998 ) ) ;
#17441=CARTESIAN_POINT ( 'NONE',  ( -22.04257564474043818, 18.72061943465525857, -219.1781831295219263 ) ) ;
#17442=CARTESIAN_POINT ( 'NONE',  ( 28.77543668145700195, 2.466904630248945907, -219.6646827587300947 ) ) ;
#17444=CARTESIAN_POINT ( 'NONE',  ( 4.559463107227270662, 13.27337529356814017, -226.9596205199204633 ) ) ;
#17447=CARTESIAN_POINT ( 'NONE',  ( -1.177898122437396333, -26.14463525305933445, -216.8677949074964033 ) ) ;
#17448=CARTESIAN_POINT ( 'NONE',  ( 16.85953475301105442, -7.801609028127129086, -231.9437213283852941 ) ) ;
#17451=CARTESIAN_POINT ( 'NONE',  ( -15.42311360645077301, 11.97619046995196079, -234.9244673706848801 ) ) ;
#17452=CARTESIAN_POINT ( 'NONE',  ( -26.74184309910812374, -3.166857098814535032, -228.4517881524372456 ) ) ;
#17453=CARTESIAN_POINT ( 'NONE',  ( 19.55931020704464274, 3.833820734573247346, -215.4549349108404783 ) ) ;
#17454=CARTESIAN_POINT ( 'NONE',  ( 6.040050017043670394, 13.67534390435379699, -220.4759402345340504 ) ) ;
#17455=CARTESIAN_POINT ( 'NONE',  ( 5.720314275582434327, 25.17872937134267630, -219.7530083620574430 ) ) ;
#17457=CARTESIAN_POINT ( 'NONE',  ( 9.097608097968041818, -8.678217757318975600, -221.4288273931462641 ) ) ;
#17459=CARTESIAN_POINT ( 'NONE',  ( 14.22574309452842733, 4.476723532073429546, -225.5862451792618231 ) ) ;
#17460=CARTESIAN_POINT ( 'NONE',  ( -9.747505956077446854, 15.39125695327449783, -233.2799778227147840 ) ) ;
#17461=CARTESIAN_POINT ( 'NONE',  ( -14.95675039876920032, 11.42095949000369259, -217.2220932760075129 ) ) ;
#17462=CARTESIAN_POINT ( 'NONE',  ( -9.225692202065292946, -15.38374647092247116, -218.6784895636799320 ) ) ;
#17463=CARTESIAN_POINT ( 'NONE',  ( -22.04257564474043818, 18.72061943465525857, -219.1781831295219263 ) ) ;
#17468=CARTESIAN_POINT ( 'NONE',  ( -9.679547659771646551, 14.60131434979866505, -230.4338124916943968 ) ) ;
#17469=CARTESIAN_POINT ( 'NONE',  ( 6.550054208186137039, 12.38618022562281595, -231.5087189857719068 ) ) ;
#17470=CARTESIAN_POINT ( 'NONE',  ( 18.79638869589749461, 0.4878066561304963966, -219.5712168927955759 ) ) ;
#17471=CARTESIAN_POINT ( 'NONE',  ( -24.34656557913400476, -15.24755813437383267, -217.2726941375463809 ) ) ;
#17472=CARTESIAN_POINT ( 'NONE',  ( -24.60063047153272819, -17.11178239752603858, -226.7032704813509554 ) ) ;
#17473=CARTESIAN_POINT ( 'NONE',  ( -7.626320092023432196, 21.25423560278784407, -233.8867968595558295 ) ) ;
#17474=CARTESIAN_POINT ( 'NONE',  ( -0.6367083786117293531, -29.73461014436635708, -220.1383336929387724 ) ) ;
#17475=CARTESIAN_POINT ( 'NONE',  ( 15.91295838535984331, 21.88410254487826379, -230.9583961155862823 ) ) ;
#17476=CARTESIAN_POINT ( 'NONE',  ( 8.727084366397900084, -11.39314604550613375, -218.1375774943401495 ) ) ;
#17480=CARTESIAN_POINT ( 'NONE',  ( 14.55590852435181226, 2.816890518231522034, -218.5131513550309990 ) ) ;
#17482=CARTESIAN_POINT ( 'NONE',  ( -2.426309470044460959, 27.69042070294474556, -223.4541227565655674 ) ) ;
#17483=CARTESIAN_POINT ( 'NONE',  ( 20.47387447818710271, 7.390772095927000684, -234.0991886097562258 ) ) ;
#17484=CARTESIAN_POINT ( 'NONE',  ( 14.73698509926073186, 4.443590625350892331, -227.4062002049096236 ) ) ;
#17485=CARTESIAN_POINT ( 'NONE',  ( 20.18206873099720156, 1.748383523995667987, -234.4526011791959661 ) ) ;
#17486=CARTESIAN_POINT ( 'NONE',  ( -7.442430984977708164, -13.68264719635657301, -220.8544524341123747 ) ) ;
#17487=CARTESIAN_POINT ( 'NONE',  ( 1.682843645364419993, 12.02583837823347679, -224.9288196625490457 ) ) ;
#17489=CARTESIAN_POINT ( 'NONE',  ( -3.316277044624852621, -11.89182204942354382, -222.3557635030381618 ) ) ;
#17490=CARTESIAN_POINT ( 'NONE',  ( -10.29720673141181209, 11.14783905173092649, -222.8560683878917530 ) ) ;
#17492=CARTESIAN_POINT ( 'NONE',  ( 11.09231067055629616, 7.417581979752235100, -227.5152062457793534 ) ) ;
#17493=CARTESIAN_POINT ( 'NONE',  ( -14.48876282330270016, -2.056064607042531911, -223.6537127325441361 ) ) ;
#17494=CARTESIAN_POINT ( 'NONE',  ( -20.29166677327761903, 16.18344358422343632, -220.0060062064338524 ) ) ;
#17495=CARTESIAN_POINT ( 'NONE',  ( 1.557078628722260438, 24.20011951319323273, -235.1441088220640268 ) ) ;
#17496=CARTESIAN_POINT ( 'NONE',  ( 22.05207439088920651, 1.190718621721708947, -218.4927357815377604 ) ) ;
#17498=CARTESIAN_POINT ( 'NONE',  ( 7.295492848317381984, -15.02116458630077034, -222.2946426130486941 ) ) ;
#17499=CARTESIAN_POINT ( 'NONE',  ( 19.33791609681259160, -22.44220124466257360, -223.0821732511882090 ) ) ;
#17500=CARTESIAN_POINT ( 'NONE',  ( -2.532949683519015949, 17.18298404079579100, -229.0924323441805086 ) ) ;
#17503=CARTESIAN_POINT ( 'NONE',  ( 12.10245006109274080, 26.02147364279441888, -220.6079829738538649 ) ) ;
#17504=CARTESIAN_POINT ( 'NONE',  ( -29.62561404221338890, 0.9211338879504321620, -221.2478075149841743 ) ) ;
#17505=CARTESIAN_POINT ( 'NONE',  ( -25.98129645912436914, -15.13773040547512139, -224.1390156429105787 ) ) ;
#17506=CARTESIAN_POINT ( 'NONE',  ( 6.427665535191954937, -16.40046818492683656, -232.5919299485929912 ) ) ;
#17507=CARTESIAN_POINT ( 'NONE',  ( -0.7879796667336372851, 21.22375955577181372, -219.1554080315090118 ) ) ;
#17509=CARTESIAN_POINT ( 'NONE',  ( 13.17424634425744046, 10.51488364724239588, -221.4616598107521099 ) ) ;
#17510=CARTESIAN_POINT ( 'NONE',  ( -13.83274569775339202, 16.20364235096346661, -234.0851861771356539 ) ) ;
#17511=CARTESIAN_POINT ( 'NONE',  ( -3.125843203957122896, 15.99774916147792680, -222.8808123721668721 ) ) ;
#17513=CARTESIAN_POINT ( 'NONE',  ( 3.378648530876271039, 26.08525450992624428, -218.4319906442508454 ) ) ;
#17514=CARTESIAN_POINT ( 'NONE',  ( -16.56270003954679382, 4.935922114544952777, -221.6503923146493378 ) ) ;
#17515=CARTESIAN_POINT ( 'NONE',  ( 25.70350299105564318, 4.008313962570879241, -233.1578316763087173 ) ) ;
#17516=CARTESIAN_POINT ( 'NONE',  ( 5.625090746907006611, -14.93184515622287201, -221.0486942310484721 ) ) ;
#17520=CARTESIAN_POINT ( 'NONE',  ( -9.716674560061926869, 27.56227806819028103, -219.4917914922789919 ) ) ;
#17521=CARTESIAN_POINT ( 'NONE',  ( 20.53331905177824979, -5.913034700419025569, -230.9395893631423462 ) ) ;
#17522=CARTESIAN_POINT ( 'NONE',  ( 28.52058947142581502, -1.755848367977142610, -221.9695116608532715 ) ) ;
#17523=CARTESIAN_POINT ( 'NONE',  ( 18.06016678184731461, 2.257982981100609354, -218.9983079406065940 ) ) ;
#17524=CARTESIAN_POINT ( 'NONE',  ( 1.780803752597676537, -13.83832444325970101, -229.2250779460899537 ) ) ;
#17526=CARTESIAN_POINT ( 'NONE',  ( -18.47334320050258327, 24.79293862780133040, -226.9986786077537317 ) ) ;
#17527=CARTESIAN_POINT ( 'NONE',  ( -12.99458409358603284, 11.56864380452031504, -232.0274663316965018 ) ) ;
#17528=CARTESIAN_POINT ( 'NONE',  ( -18.46722752239034193, 0.9784074152395518809, -232.1633353206286188 ) ) ;
#17529=CARTESIAN_POINT ( 'NONE',  ( -10.95598939193837928, -18.74794674280272488, -217.4432683290776538 ) ) ;
#17532=CARTESIAN_POINT ( 'NONE',  ( 20.58703255433590940, 0.4816031003617209372, -231.9427175861361263 ) ) ;
#17533=CARTESIAN_POINT ( 'NONE',  ( -22.04257564474043818, 18.72061943465525857, -219.1781831295219263 ) ) ;
#17534=CARTESIAN_POINT ( 'NONE',  ( 8.716925653960343467, -14.61958666771473858, -219.5525962724747444 ) ) ;
#17537=CARTESIAN_POINT ( 'NONE',  ( 15.08139719848974103, 12.15862464477973504, -219.3112749338812080 ) ) ;
#17538=CARTESIAN_POINT ( 'NONE',  ( -14.08083899843152231, 10.81596681319144970, -234.3239311387574446 ) ) ;
#17540=CARTESIAN_POINT ( 'NONE',  ( 21.68053922431529301, 13.05890675940072931, -230.5667798303363440 ) ) ;
#17541=CARTESIAN_POINT ( 'NONE',  ( 5.517988016436452980, -29.70724229459007759, -226.4438119151823514 ) ) ;
#17543=CARTESIAN_POINT ( 'NONE',  ( -0.9249541874382023465, 14.55235618511626328, -223.7321818898853962 ) ) ;
#17544=CARTESIAN_POINT ( 'NONE',  ( -13.92941769543345032, 11.48925904027772127, -219.8938199480626281 ) ) ;
#17545=CARTESIAN_POINT ( 'NONE',  ( -14.99655511003079233, 2.316638599135941945, -232.4215266639120046 ) ) ;
#17547=CARTESIAN_POINT ( 'NONE',  ( -17.56620462375804692, -17.71942105192161065, -219.9081625180047013 ) ) ;
#17550=CARTESIAN_POINT ( 'NONE',  ( 14.92135368508905202, 7.451356898669101447, -219.1823315336843621 ) ) ;
#17551=CARTESIAN_POINT ( 'NONE',  ( 4.568467666399979699, -17.52045581048442457, -219.7174082404806938 ) ) ;
#17552=CARTESIAN_POINT ( 'NONE',  ( 12.71450444683213021, 7.595266944807587350, -224.4213778964231665 ) ) ;
#17553=CARTESIAN_POINT ( 'NONE',  ( -23.52999999174766543, 19.39566142560855866, -221.9446938626390704 ) ) ;
#17554=CARTESIAN_POINT ( 'NONE',  ( 25.09997929702755926, 1.294103573351435221, -217.0485712200477906 ) ) ;
#17555=CARTESIAN_POINT ( 'NONE',  ( 4.389496648589924277, 14.47660514356954131, -220.6151178996808540 ) ) ;
#17557=CARTESIAN_POINT ( 'NONE',  ( -6.512931564893298386, -17.32529878264574563, -216.7284160531958719 ) ) ;
#17558=CARTESIAN_POINT ( 'NONE',  ( 21.30961698559626427, -20.48616475849644303, -228.5322376518520002 ) ) ;
#17561=CARTESIAN_POINT ( 'NONE',  ( -12.13319425917249283, 4.024026700415168634, -229.5243363405849095 ) ) ;
#17562=CARTESIAN_POINT ( 'NONE',  ( -22.35893676869521229, -6.243268429983856116, -219.2540196962538062 ) ) ;
#17563=CARTESIAN_POINT ( 'NONE',  ( -12.06153928353927540, 8.661506524875534296, -226.8425068572842349 ) ) ;
#17564=CARTESIAN_POINT ( 'NONE',  ( -2.692720963948733282, 24.67937284847025481, -218.0912907784291406 ) ) ;
#17565=CARTESIAN_POINT ( 'NONE',  ( 5.066530254613678785, 15.76189963344335254, -222.1234037505291781 ) ) ;
#17567=CARTESIAN_POINT ( 'NONE',  ( 18.59830189133340639, -20.05840858737748533, -233.4490516770458157 ) ) ;
#17569=CARTESIAN_POINT ( 'NONE',  ( 14.85123888640019452, 5.067529763532427012, -221.9058491819374979 ) ) ;
#17570=CARTESIAN_POINT ( 'NONE',  ( -15.23792247720107440, 7.806131751461257373, -230.3336101049160902 ) ) ;
#17571=CARTESIAN_POINT ( 'NONE',  ( -11.01414002179357610, 8.614420160880040811, -226.3770540798392972 ) ) ;
#17572=CARTESIAN_POINT ( 'NONE',  ( -13.44605823798860200, -7.860403065310468840, -219.7865185367595586 ) ) ;
#17573=CARTESIAN_POINT ( 'NONE',  ( -19.00318367631585659, 13.14621133775862916, -233.8403879275295765 ) ) ;
#17576=CARTESIAN_POINT ( 'NONE',  ( 14.94998080268256757, -2.571697545922924100, -223.4431372107500238 ) ) ;
#17577=CARTESIAN_POINT ( 'NONE',  ( 25.50289296650958448, 5.998088869914441901, -233.1161630295026157 ) ) ;
#17578=CARTESIAN_POINT ( 'NONE',  ( -22.03660207690921879, 17.07234836129451949, -222.7335359861421296 ) ) ;
#17579=CARTESIAN_POINT ( 'NONE',  ( 11.38520239593705163, 18.87760105923376486, -235.3435298574111130 ) ) ;
#17581=CARTESIAN_POINT ( 'NONE',  ( -16.74550766701807447, 3.787526820511904813, -217.9802846976114381 ) ) ;
#17582=CARTESIAN_POINT ( 'NONE',  ( -10.39490437715664228, -5.549361993742060406, -223.4983083630424403 ) ) ;
#17583=CARTESIAN_POINT ( 'NONE',  ( -30.78084016402396372, -2.501288241119758116, -224.5721874330603214 ) ) ;
#17584=CARTESIAN_POINT ( 'NONE',  ( -8.328662059352005542, 28.53523473722178139, -221.4280032538016201 ) ) ;
#17585=CARTESIAN_POINT ( 'NONE',  ( -8.379125946468517938, -29.31735857037017468, -221.8060643354269814 ) ) ;
#17586=CARTESIAN_POINT ( 'NONE',  ( 4.730976410881341465, 17.65764351829336931, -217.6025626048331674 ) ) ;
#17587=CARTESIAN_POINT ( 'NONE',  ( 10.16297913136807907, -22.49776018550796408, -215.0507767410722977 ) ) ;
#17589=CARTESIAN_POINT ( 'NONE',  ( 21.17011458613547248, 1.652544727609948527, -234.6098499860487152 ) ) ;
#17590=CARTESIAN_POINT ( 'NONE',  ( -3.015877970456246615, 27.27456613555083464, -227.6995284396757313 ) ) ;
#17591=CARTESIAN_POINT ( 'NONE',  ( 29.47107563651793427, 6.731311671946880182, -220.0565342412898815 ) ) ;
#17592=CARTESIAN_POINT ( 'NONE',  ( 16.91879448796214191, 0.8271603773820436212, -230.0510230802265710 ) ) ;
#17593=CARTESIAN_POINT ( 'NONE',  ( 12.54860906168727652, 6.077542143275485031, -228.1605930327268368 ) ) ;
#17594=CARTESIAN_POINT ( 'NONE',  ( -8.373128421490182660, -27.12459427582015792, -230.7938890564172709 ) ) ;
#17595=CARTESIAN_POINT ( 'NONE',  ( 5.773563157792669820, 21.63217468058455140, -235.0383461317610170 ) ) ;
#17597=CARTESIAN_POINT ( 'NONE',  ( -13.54879968420069503, -27.67624318860520916, -230.2549257473255579 ) ) ;
#17598=CARTESIAN_POINT ( 'NONE',  ( -4.334015487506815312, 18.19775486192265390, -231.4387392399519285 ) ) ;
#17599=CARTESIAN_POINT ( 'NONE',  ( 10.88376588832297287, 7.577514201227793400, -222.7215714477710833 ) ) ;
#17600=CARTESIAN_POINT ( 'NONE',  ( -16.54465188417290022, 6.134005835925411709, -228.8256222654843270 ) ) ;
#17602=CARTESIAN_POINT ( 'NONE',  ( -4.845359737286285551, 16.85396349487340117, -233.9229833851842670 ) ) ;
#17603=CARTESIAN_POINT ( 'NONE',  ( 25.60482246989237609, 8.614967517510873307, -219.3103232513597618 ) ) ;
#17604=CARTESIAN_POINT ( 'NONE',  ( 12.66847874168482591, -12.52481328540277161, -229.3043100997535646 ) ) ;
#17606=CARTESIAN_POINT ( 'NONE',  ( 11.63416633096549369, -11.60453582225250990, -230.7583135875248104 ) ) ;
#17607=CARTESIAN_POINT ( 'NONE',  ( -3.125843203957122896, 15.99774916147792680, -222.8808123721668721 ) ) ;
#17610=CARTESIAN_POINT ( 'NONE',  ( 7.743212835174657194, 11.90778931056080481, -226.0491028376908105 ) ) ;
#17611=CARTESIAN_POINT ( 'NONE',  ( 20.15756451863428111, -2.090604891399794774, -217.8900786001194945 ) ) ;
#17612=CARTESIAN_POINT ( 'NONE',  ( -13.67406442719345883, -9.319000780081536206, -231.1492214949047934 ) ) ;
#17613=CARTESIAN_POINT ( 'NONE',  ( 8.332496243628455090, -29.79192972398156769, -226.1452587264855367 ) ) ;
#17614=CARTESIAN_POINT ( 'NONE',  ( 1.030230143518703345, 18.27887886751213387, -229.5791973322770616 ) ) ;
#17616=CARTESIAN_POINT ( 'NONE',  ( 23.74723497152361062, 5.524508269105988134, -217.6012181427065002 ) ) ;
#17617=CARTESIAN_POINT ( 'NONE',  ( -9.171998067665157350, 9.395241133357435714, -226.3428046914542051 ) ) ;
#17618=CARTESIAN_POINT ( 'NONE',  ( -8.308618357598591686, 12.44656112581930785, -228.0014162119141474 ) ) ;
#17620=CARTESIAN_POINT ( 'NONE',  ( -2.435715273212520238, 23.41098772907853132, -217.6796576669356966 ) ) ;
#17621=CARTESIAN_POINT ( 'NONE',  ( 15.96089671440110713, 1.143943728337336374, -218.3532651118343892 ) ) ;
#17622=CARTESIAN_POINT ( 'NONE',  ( 13.40064012097826307, 2.532414129335418096, -221.5952957478750989 ) ) ;
#17623=CARTESIAN_POINT ( 'NONE',  ( 18.03651828442428595, -19.10816016050398147, -231.7458924702002037 ) ) ;
#17626=CARTESIAN_POINT ( 'NONE',  ( 11.67669251569587985, 24.04736029062789981, -218.5856804285192254 ) ) ;
#17627=CARTESIAN_POINT ( 'NONE',  ( 26.42227051273691885, -8.869064526452445918, -225.3570890864022260 ) ) ;
#17629=CARTESIAN_POINT ( 'NONE',  ( 16.07305932912010960, 0.9253679043337685872, -229.0409936706996064 ) ) ;
#17630=CARTESIAN_POINT ( 'NONE',  ( 1.292981098121811279, -26.53499626907933262, -232.9055005154886828 ) ) ;
#17631=CARTESIAN_POINT ( 'NONE',  ( -12.90983082593748676, 14.84936372681532823, -233.8009687022269532 ) ) ;
#17632=CARTESIAN_POINT ( 'NONE',  ( -10.01410430826631170, 16.10970239316000630, -233.6135099156378203 ) ) ;
#17634=CARTESIAN_POINT ( 'NONE',  ( -20.26851768784797869, -0.8260594303982465858, -217.1279713726092098 ) ) ;
#17635=CARTESIAN_POINT ( 'NONE',  ( -15.28220591200235390, -15.65475725988279443, -217.1155325995422913 ) ) ;
#17638=CARTESIAN_POINT ( 'NONE',  ( -11.46843428684449151, 6.508406145394057596, -225.7212143570321814 ) ) ;
#17639=CARTESIAN_POINT ( 'NONE',  ( 0.09627406729119250550, -13.23594471221713142, -227.7621942207877339 ) ) ;
#17640=CARTESIAN_POINT ( 'NONE',  ( 14.96415947227435339, -1.927366939720012606, -222.7010313878448358 ) ) ;
#17643=CARTESIAN_POINT ( 'NONE',  ( 21.07144422417032104, 18.33581350331571969, -223.6711752364813890 ) ) ;
#17644=CARTESIAN_POINT ( 'NONE',  ( -9.045741320599788082, 11.46901338045063312, -219.0588111342715365 ) ) ;
#17646=CARTESIAN_POINT ( 'NONE',  ( 18.30590144060498403, 15.06309558287673767, -219.0459394567220102 ) ) ;
#17647=CARTESIAN_POINT ( 'NONE',  ( 5.319567441806261066, -29.83260615907786573, -224.9444841741296841 ) ) ;
#17650=CARTESIAN_POINT ( 'NONE',  ( -2.692720963948733282, 24.67937284847025481, -218.0912907784291406 ) ) ;
#17651=CARTESIAN_POINT ( 'NONE',  ( -10.24168223636446662, 16.14271751156598356, -231.4847994864913971 ) ) ;
#17652=CARTESIAN_POINT ( 'NONE',  ( 18.39384604806649648, 2.566915855367216004, -231.7421336352533103 ) ) ;
#17653=CARTESIAN_POINT ( 'NONE',  ( -16.76407561856198214, -10.47882714055132070, -219.0733374248486598 ) ) ;
#17656=CARTESIAN_POINT ( 'NONE',  ( -21.08008464085897060, -0.9048411197481797119, -217.0000000010748522 ) ) ;
#17657=CARTESIAN_POINT ( 'NONE',  ( 0.8935217740153370558, -25.09083646304939919, -218.5222943608621335 ) ) ;
#17658=CARTESIAN_POINT ( 'NONE',  ( 14.95414693437772868, 8.262206471704862665, -230.1862972580043163 ) ) ;
#17659=CARTESIAN_POINT ( 'NONE',  ( -3.673551555920188783, 29.81207051619892923, -228.8770490300152005 ) ) ;
#17660=CARTESIAN_POINT ( 'NONE',  ( 17.85905871012913693, 8.463974683125162102, -234.6532732619751300 ) ) ;
#17661=CARTESIAN_POINT ( 'NONE',  ( 4.883314309504700468, 19.06839645569368358, -217.0171359871271193 ) ) ;
#17663=CARTESIAN_POINT ( 'NONE',  ( -13.60146639818222702, -25.11808310587244009, -230.9974232610874196 ) ) ;
#17664=CARTESIAN_POINT ( 'NONE',  ( 13.28406271702445274, -5.237238614233280742, -225.2640488721434622 ) ) ;
#17667=CARTESIAN_POINT ( 'NONE',  ( -28.76901170826145560, 13.32870333992657663, -228.6722616467874616 ) ) ;
#17668=CARTESIAN_POINT ( 'NONE',  ( -16.42300678490213883, -6.478264502461970054, -228.9348778629521064 ) ) ;
#17669=CARTESIAN_POINT ( 'NONE',  ( -11.94782396647286049, 8.456988817430419303, -225.5094493096559063 ) ) ;
#17670=CARTESIAN_POINT ( 'NONE',  ( 14.60728983664449387, 19.38727400458104455, -216.6381802409380555 ) ) ;
#17671=CARTESIAN_POINT ( 'NONE',  ( 5.646952844456516019, 23.06006924884521325, -218.8221376988549878 ) ) ;
#17673=CARTESIAN_POINT ( 'NONE',  ( 25.69865375807269459, -17.81673768310515626, -220.5381737609034474 ) ) ;
#17674=ORIENTED_EDGE ( 'NONE', *, *, #5134, .T. ) ;
#17675=CARTESIAN_POINT ( 'NONE',  ( 17.07668571305246985, 2.037405138410691485, -219.7626854147787867 ) ) ;
#17677=CARTESIAN_POINT ( 'NONE',  ( -13.24620988741752825, 28.78239319002125285, -225.3527830703614256 ) ) ;
#17678=CARTESIAN_POINT ( 'NONE',  ( -11.40916210110096962, 20.01996232974788725, -234.3205435716851923 ) ) ;
#17679=CARTESIAN_POINT ( 'NONE',  ( -28.09913862414779473, -9.456046895945956265, -221.0065986266286870 ) ) ;
#17681=CARTESIAN_POINT ( 'NONE',  ( -11.79584727357715934, 6.509288465425584036, -222.6080315736180921 ) ) ;
#17684=CARTESIAN_POINT ( 'NONE',  ( 28.78651053433536333, -0.9604905981993369091, -227.3547688931310233 ) ) ;
#17686=CARTESIAN_POINT ( 'NONE',  ( -13.58070052954164275, 11.19572749768420650, -220.2511552028196604 ) ) ;
#17687=CARTESIAN_POINT ( 'NONE',  ( 14.95834318372430083, -1.617016552789838801, -229.6306532055809271 ) ) ;
#17688=CARTESIAN_POINT ( 'NONE',  ( -22.47200958260654957, 4.697452857301940732, -216.5879371680706242 ) ) ;
#17689=CARTESIAN_POINT ( 'NONE',  ( 9.107417252317809186, 16.30291009569977234, -218.0131178633739921 ) ) ;
#17691=CARTESIAN_POINT ( 'NONE',  ( -26.47652094774193188, -8.527600130219385122, -218.5932275281782324 ) ) ;
#17692=CARTESIAN_POINT ( 'NONE',  ( -0.4548635697939061306, 27.30478022265488036, -219.8474162243132071 ) ) ;
#17693=CARTESIAN_POINT ( 'NONE',  ( -6.642805165258356404, -28.12267032419628521, -230.9452027245340560 ) ) ;
#17694=CARTESIAN_POINT ( 'NONE',  ( 5.331555957413248059, 27.50712867803999728, -219.0801070358024276 ) ) ;
#17695=CARTESIAN_POINT ( 'NONE',  ( 13.52447848812844100, -22.07588418332509050, -234.6412735253872484 ) ) ;
#17696=CARTESIAN_POINT ( 'NONE',  ( 14.73484710815641030, -0.3083309717192121435, -227.9841133479512223 ) ) ;
#17697=CARTESIAN_POINT ( 'NONE',  ( -12.33203608746942237, 8.428128317385924717, -222.9277009507565026 ) ) ;
#17699=CARTESIAN_POINT ( 'NONE',  ( 29.82766783012230505, -1.714217446056379934, -229.3564438616236316 ) ) ;
#17700=CARTESIAN_POINT ( 'NONE',  ( 3.786538429322381383, 16.06208591393598084, -226.9891439814428793 ) ) ;
#17701=CARTESIAN_POINT ( 'NONE',  ( -12.62195384480319582, 9.244619650382723819, -228.6283004876635516 ) ) ;
#17703=CARTESIAN_POINT ( 'NONE',  ( 25.18785298611088308, 3.974282393449815931, -218.7636041058819956 ) ) ;
#17704=CARTESIAN_POINT ( 'NONE',  ( -10.37556110177195023, -11.10057404503678846, -224.0577835142470349 ) ) ;
#17706=CARTESIAN_POINT ( 'NONE',  ( 12.08790845148079640, 6.355304031620478078, -220.0087475230167229 ) ) ;
#17708=CARTESIAN_POINT ( 'NONE',  ( -5.787689185779406387, -30.68964578337966387, -228.1462806397894383 ) ) ;
#17709=CARTESIAN_POINT ( 'NONE',  ( -10.16319438574952372, 11.71174522937666040, -227.8434026503654479 ) ) ;
#17711=CARTESIAN_POINT ( 'NONE',  ( 15.88043104796248528, 11.88135572392608807, -216.2525917828042168 ) ) ;
#17713=CARTESIAN_POINT ( 'NONE',  ( -14.59766675578715223, 7.926254675926275972, -222.3706877972550444 ) ) ;
#17714=CARTESIAN_POINT ( 'NONE',  ( 4.754245974719506940, 31.05377813473586102, -220.6166503949300193 ) ) ;
#17715=CARTESIAN_POINT ( 'NONE',  ( 27.16757474806794903, 2.676291341565463888, -220.8863403533574115 ) ) ;
#17717=CARTESIAN_POINT ( 'NONE',  ( 18.63268865202281432, -19.94522792032704572, -227.6816033052257637 ) ) ;
#17718=CARTESIAN_POINT ( 'NONE',  ( 8.767697218519710844, -14.65932909790238448, -230.8495237012982386 ) ) ;
#17719=CARTESIAN_POINT ( 'NONE',  ( -3.389634396460917465, 16.42708991135657115, -221.9057377485790994 ) ) ;
#17721=CARTESIAN_POINT ( 'NONE',  ( 19.20300624114736721, 0.6066039755357417462, -231.5046416827383950 ) ) ;
#17722=CARTESIAN_POINT ( 'NONE',  ( 27.02029988085337919, -0.4174685747284823112, -230.1188858631967378 ) ) ;
#17723=CARTESIAN_POINT ( 'NONE',  ( -13.52935284690462758, -5.503084506376929141, -222.3607690796775671 ) ) ;
#17724=CARTESIAN_POINT ( 'NONE',  ( -3.734153817218577309, -19.72686645808614614, -233.9207428641194610 ) ) ;
#17725=CARTESIAN_POINT ( 'NONE',  ( -9.175187729848801155, 26.50888816229029743, -227.9285554593684253 ) ) ;
#17727=CARTESIAN_POINT ( 'NONE',  ( -14.37318171526297483, 2.227741863946853140, -231.7654527934561202 ) ) ;
#17728=CARTESIAN_POINT ( 'NONE',  ( -2.934221234790329369, 15.07857928364152222, -230.9558365497803720 ) ) ;
#17729=CARTESIAN_POINT ( 'NONE',  ( -2.693916085894628942, 18.86613858709357672, -230.4911878356387263 ) ) ;
#17734=CARTESIAN_POINT ( 'NONE',  ( -0.1881941282075867139, 17.37563936270229092, -230.9177995227891813 ) ) ;
#17735=CARTESIAN_POINT ( 'NONE',  ( -27.32939371162572684, 5.861081283609568260, -224.9659309793921409 ) ) ;
#17736=CARTESIAN_POINT ( 'NONE',  ( 10.90540179105271967, 5.382827416078996841, -224.1493061458977820 ) ) ;
#17737=CARTESIAN_POINT ( 'NONE',  ( 8.767697218519710844, -14.65932909790238448, -230.8495237012982386 ) ) ;
#17740=CARTESIAN_POINT ( 'NONE',  ( 7.743212835174657194, 11.90778931056080481, -226.0491028376908105 ) ) ;
#17741=CARTESIAN_POINT ( 'NONE',  ( 18.57039993684838564, -7.499893981036622748, -219.4816775992414080 ) ) ;
#17743=CARTESIAN_POINT ( 'NONE',  ( 0.5120693878963755719, -30.63998626839889639, -227.9504769009175220 ) ) ;
#17745=CARTESIAN_POINT ( 'NONE',  ( -11.24282496690421596, 12.44430180464951086, -232.4405891940542404 ) ) ;
#17747=CARTESIAN_POINT ( 'NONE',  ( -7.752954785937490989, 10.21341112307795385, -225.5135920495299615 ) ) ;
#17749=CARTESIAN_POINT ( 'NONE',  ( -6.282398543089500187, 12.01615879894893801, -228.5121145169883903 ) ) ;
#17750=CARTESIAN_POINT ( 'NONE',  ( -10.22552941266963877, -9.699191453761107695, -225.4315674810442545 ) ) ;
#17754=CARTESIAN_POINT ( 'NONE',  ( -6.101488798441174310, 11.33371047077072369, -225.3616985956418546 ) ) ;
#17755=CARTESIAN_POINT ( 'NONE',  ( 4.072690587420734865, -13.44063513242216246, -222.4530508649998239 ) ) ;
#17757=CARTESIAN_POINT ( 'NONE',  ( -11.79584727357715934, 6.509288465425584036, -222.6080315736180921 ) ) ;
#17758=CARTESIAN_POINT ( 'NONE',  ( 13.38540196930496862, 9.639609424068478205, -227.8779021328794840 ) ) ;
#17759=CARTESIAN_POINT ( 'NONE',  ( -13.17897211815351000, 23.48099580033777301, -217.3415693533541173 ) ) ;
#17761=CARTESIAN_POINT ( 'NONE',  ( 16.53859560591101641, 22.24348416270211359, -223.7250258089275974 ) ) ;
#17762=CARTESIAN_POINT ( 'NONE',  ( -8.370291489323296474, -27.15533861588617981, -226.3382906634514597 ) ) ;
#17764=CARTESIAN_POINT ( 'NONE',  ( -4.073886805163430935, 14.35067061637828623, -226.4733297826468572 ) ) ;
#17765=CARTESIAN_POINT ( 'NONE',  ( -22.03660207690921879, 17.07234836129451949, -222.7335359861421296 ) ) ;
#17766=CARTESIAN_POINT ( 'NONE',  ( -16.90193019167508126, 18.45790510038867893, -217.5707532411249758 ) ) ;
#17767=CARTESIAN_POINT ( 'NONE',  ( -19.03657574603155567, -20.25511037490812782, -224.1171725289517269 ) ) ;
#17770=CARTESIAN_POINT ( 'NONE',  ( -21.89482327431018760, 1.733733432562314158, -233.1353281693111796 ) ) ;
#17771=CARTESIAN_POINT ( 'NONE',  ( 2.245945009347994237, -28.59251958642781233, -226.9771193766267743 ) ) ;
#17772=CARTESIAN_POINT ( 'NONE',  ( 15.42212722119060864, 5.401662248084913465, -220.8333402320903645 ) ) ;
#17774=CARTESIAN_POINT ( 'NONE',  ( -5.807479211365208727, 19.77444019604324410, -216.0778658752277863 ) ) ;
#17776=CARTESIAN_POINT ( 'NONE',  ( -17.91550223652134122, 4.809113705933536487, -230.6324822114035555 ) ) ;
#17777=CARTESIAN_POINT ( 'NONE',  ( 23.04342321161690776, 14.90264581583150694, -218.4777833225197412 ) ) ;
#17778=CARTESIAN_POINT ( 'NONE',  ( 15.85665641241444668, 18.24713744004561988, -217.7195292979064902 ) ) ;
#17780=CARTESIAN_POINT ( 'NONE',  ( -15.48425879135615446, -25.29886615046042309, -220.6886037686364261 ) ) ;
#17781=CARTESIAN_POINT ( 'NONE',  ( 15.60497028854143764, -26.39208911975253002, -225.8550158017044112 ) ) ;
#17785=CARTESIAN_POINT ( 'NONE',  ( -12.22073052649759184, 14.03927388329973525, -215.9097966823721606 ) ) ;
#17786=CARTESIAN_POINT ( 'NONE',  ( -23.46219451118877330, -13.03948552059806509, -221.3852197888554372 ) ) ;
#17787=CARTESIAN_POINT ( 'NONE',  ( -13.97943781666340790, 5.798109546139844639, -228.2992319913466019 ) ) ;
#17788=CARTESIAN_POINT ( 'NONE',  ( 23.44028133050380802, 19.87677100428751231, -223.1503774981096342 ) ) ;
#17789=CARTESIAN_POINT ( 'NONE',  ( -1.696080206444520844, 14.74162257415073540, -222.2455536759108838 ) ) ;
#17791=CARTESIAN_POINT ( 'NONE',  ( 20.52151979663716830, -23.02670487196117222, -229.5295066797569348 ) ) ;
#17792=CARTESIAN_POINT ( 'NONE',  ( 22.18132842682159733, 5.591149267797686839, -232.0584733989884114 ) ) ;
#17793=CARTESIAN_POINT ( 'NONE',  ( 2.660414182604129429, 28.99288898680367055, -232.5781547115647072 ) ) ;
#17794=CARTESIAN_POINT ( 'NONE',  ( -12.15711705271618470, 28.08001788883979799, -220.3431297925021681 ) ) ;
#17795=CARTESIAN_POINT ( 'NONE',  ( -27.10757994293576800, -10.52107906247675473, -229.7403242048749519 ) ) ;
#17796=CARTESIAN_POINT ( 'NONE',  ( -21.93900267957129557, 7.862893636934532360, -233.4951761057262161 ) ) ;
#17799=CARTESIAN_POINT ( 'NONE',  ( 14.56914850832129815, -2.041740472307377985, -224.7121590863160350 ) ) ;
#17800=CARTESIAN_POINT ( 'NONE',  ( -2.047892494109819328, 12.88402507277750786, -223.5104301352110951 ) ) ;
#17801=CARTESIAN_POINT ( 'NONE',  ( 13.21888801141564151, 2.135177519634172238, -228.0426311217386797 ) ) ;
#17802=CARTESIAN_POINT ( 'NONE',  ( 15.92396645628901020, -0.3225394686005420009, -223.0199929375764327 ) ) ;
#17803=CARTESIAN_POINT ( 'NONE',  ( 8.812073984913094904, 13.12649198322903210, -229.9172071780580495 ) ) ;
#17804=CARTESIAN_POINT ( 'NONE',  ( -19.98462433625633494, -12.30084073857678639, -216.8518508258974862 ) ) ;
#17807=CARTESIAN_POINT ( 'NONE',  ( -1.707778556226592581, 19.51307486516442680, -232.5708079709245055 ) ) ;
#17808=CARTESIAN_POINT ( 'NONE',  ( -1.489322793389167288, -21.37773154815333498, -215.8826219457350817 ) ) ;
#17809=CARTESIAN_POINT ( 'NONE',  ( 5.169766346882679997, 29.28517558595074988, -221.5178724947562614 ) ) ;
#17810=CARTESIAN_POINT ( 'NONE',  ( 8.134488596945347538, -11.59059696487595481, -231.6292735970982335 ) ) ;
#17812=CARTESIAN_POINT ( 'NONE',  ( -10.29720673141181209, 11.14783905173092649, -222.8560683878917530 ) ) ;
#17814=CARTESIAN_POINT ( 'NONE',  ( -28.53682043726378836, -3.412203979905605866, -221.0207037827091767 ) ) ;
#17815=CARTESIAN_POINT ( 'NONE',  ( 9.489894741926459432, 25.96007012349547338, -222.3210984495278524 ) ) ;
#17816=CARTESIAN_POINT ( 'NONE',  ( -21.66803296057637951, 19.04503900041684616, -222.6603677762044526 ) ) ;
#17817=CARTESIAN_POINT ( 'NONE',  ( 26.48990917286906921, 12.16675355942207659, -225.0153622588060216 ) ) ;
#17818=CARTESIAN_POINT ( 'NONE',  ( -12.60888841760081824, -15.87650330583304914, -218.3826098682522456 ) ) ;
#17821=CARTESIAN_POINT ( 'NONE',  ( 26.75877786246624623, 11.80320999550499117, -231.5572967531201414 ) ) ;
#17823=CARTESIAN_POINT ( 'NONE',  ( -7.876537541093066253, -10.96045937405908965, -230.9151686379251487 ) ) ;
#17824=CARTESIAN_POINT ( 'NONE',  ( -1.038524475621362075, 14.89017051181998141, -222.3948816610352139 ) ) ;
#17825=CARTESIAN_POINT ( 'NONE',  ( 16.96779410054824666, 23.69881408353223406, -220.2174342377987841 ) ) ;
#17826=CARTESIAN_POINT ( 'NONE',  ( -8.900302563431933933, 20.17395648083808268, -216.9116515890487733 ) ) ;
#17827=CARTESIAN_POINT ( 'NONE',  ( -4.155456637169709921, 11.30291311430030987, -225.2606024264729001 ) ) ;
#17828=CARTESIAN_POINT ( 'NONE',  ( -21.89065952084848021, -0.9940043559354364566, -216.9999999999999716 ) ) ;
#17830=CARTESIAN_POINT ( 'NONE',  ( 9.413533971304945069, -13.52850967935795623, -226.9656141048783695 ) ) ;
#17831=CARTESIAN_POINT ( 'NONE',  ( 7.640685522499278903, -12.22373526560700441, -226.1755943870604710 ) ) ;
#17833=CARTESIAN_POINT ( 'NONE',  ( 18.46552355142154411, 5.019711608606525211, -231.5099115070375433 ) ) ;
#17834=CARTESIAN_POINT ( 'NONE',  ( 19.06763123184207487, -2.048228142369658666, -218.2337357994572073 ) ) ;
#17835=CARTESIAN_POINT ( 'NONE',  ( -14.13781561609191328, -15.90667165809925621, -233.6615929499251649 ) ) ;
#17836=CARTESIAN_POINT ( 'NONE',  ( -1.489322793389167288, -21.37773154815333498, -215.8826219457350817 ) ) ;
#17837=CARTESIAN_POINT ( 'NONE',  ( 3.528957931946373971, 27.43889307663531696, -223.4805233499528185 ) ) ;
#17839=CARTESIAN_POINT ( 'NONE',  ( -12.13127060986278316, 5.971392262169284315, -229.0615017441034524 ) ) ;
#17840=CARTESIAN_POINT ( 'NONE',  ( -3.368164009525018265, 19.03203264544105622, -233.5986411977714567 ) ) ;
#17841=CARTESIAN_POINT ( 'NONE',  ( 3.060417506408009469, 27.46204888741655026, -226.6022202862033623 ) ) ;
#17842=CARTESIAN_POINT ( 'NONE',  ( 22.70267758588118312, -6.899298642777032420, -215.6456595153534863 ) ) ;
#17845=CARTESIAN_POINT ( 'NONE',  ( 22.73582563804385970, 20.20868311426415431, -227.8513184012435886 ) ) ;
#17846=CARTESIAN_POINT ( 'NONE',  ( -17.75632171729475317, 14.45153669854845901, -218.6240360064753929 ) ) ;
#17847=CARTESIAN_POINT ( 'NONE',  ( 14.95834318372430083, -1.617016552789838801, -229.6306532055809271 ) ) ;
#17848=CARTESIAN_POINT ( 'NONE',  ( -4.650330424930598561, -23.85841421069521928, -231.7493909980149454 ) ) ;
#17852=CARTESIAN_POINT ( 'NONE',  ( 15.91295838535984331, 21.88410254487826379, -230.9583961155862823 ) ) ;
#17853=CARTESIAN_POINT ( 'NONE',  ( 26.20608998270887469, -2.199599969171641689, -229.6935040011478009 ) ) ;
#17855=CARTESIAN_POINT ( 'NONE',  ( 6.427665535191954937, -16.40046818492683656, -232.5919299485929912 ) ) ;
#17857=CARTESIAN_POINT ( 'NONE',  ( 2.008896548638861024, 20.64812324442097591, -233.5818019448501843 ) ) ;
#17858=CARTESIAN_POINT ( 'NONE',  ( -24.30769394037691100, 17.48612956801762053, -223.4340414801748693 ) ) ;
#17860=CARTESIAN_POINT ( 'NONE',  ( -14.83974801774860630, 13.71714848582103485, -216.0935642439352762 ) ) ;
#17861=CARTESIAN_POINT ( 'NONE',  ( -18.38002254392888446, -21.81807606669838506, -229.0374583293157968 ) ) ;
#17865=CARTESIAN_POINT ( 'NONE',  ( -11.26857159993117996, 28.96895336474501192, -225.6039696848669678 ) ) ;
#17866=CARTESIAN_POINT ( 'NONE',  ( 2.697602325873029727, -29.85947730167685421, -229.1126320946688111 ) ) ;
#17867=CARTESIAN_POINT ( 'NONE',  ( 14.93094482340519846, -1.857544602713102400, -222.6424950236294364 ) ) ;
#17868=CARTESIAN_POINT ( 'NONE',  ( -23.49379658590067876, 11.46840048879614393, -217.2519070826072323 ) ) ;
#17869=CARTESIAN_POINT ( 'NONE',  ( -12.88152464663890306, 6.317716727793897924, -230.5294309895745073 ) ) ;
#17870=CARTESIAN_POINT ( 'NONE',  ( -1.268862717067444024, 15.25222216985846480, -229.0661283592426116 ) ) ;
#17872=CARTESIAN_POINT ( 'NONE',  ( 20.62963957373278134, 2.372686805184054837, -232.5966151263358483 ) ) ;
#17873=CARTESIAN_POINT ( 'NONE',  ( -19.03657574603155567, -20.25511037490812782, -224.1171725289517269 ) ) ;
#17875=CARTESIAN_POINT ( 'NONE',  ( 6.491278574642851851, 13.23281603069746382, -229.0355254242266767 ) ) ;
#17876=CARTESIAN_POINT ( 'NONE',  ( -12.01777041390050726, 10.97692933293401474, -227.6853890888168053 ) ) ;
#17877=CARTESIAN_POINT ( 'NONE',  ( -14.01966324001334385, 10.60695606488527964, -217.6333332521996340 ) ) ;
#17879=CARTESIAN_POINT ( 'NONE',  ( -22.16366393984728234, -4.852915104599624385, -232.2864540303542924 ) ) ;
#17882=CARTESIAN_POINT ( 'NONE',  ( -18.08305592660031991, 4.022743421239192152, -217.2335041149100050 ) ) ;
#17883=CARTESIAN_POINT ( 'NONE',  ( 7.295492848317381984, -15.02116458630077034, -222.2946426130486941 ) ) ;
#17884=CARTESIAN_POINT ( 'NONE',  ( 22.84140515590350518, 18.29101041979067332, -226.2334522600520472 ) ) ;
#17885=CARTESIAN_POINT ( 'NONE',  ( 4.354034006296288339, 14.09944204372416188, -221.2519525881239417 ) ) ;
#17886=CARTESIAN_POINT ( 'NONE',  ( -16.66921372850992000, 0.4301828684420727078, -227.8397539831347842 ) ) ;
#17887=CARTESIAN_POINT ( 'NONE',  ( 20.02669998934234741, 11.93441252203826508, -216.7824909737982182 ) ) ;
#17889=CARTESIAN_POINT ( 'NONE',  ( 17.99029889091409018, 9.613712288440757092, -232.0298403238024036 ) ) ;
#17891=CARTESIAN_POINT ( 'NONE',  ( -15.27057301462635408, -17.00912219741827514, -233.6288396447818627 ) ) ;
#17892=CARTESIAN_POINT ( 'NONE',  ( 5.668262076144046979, -25.28042871382391965, -216.8182873783340483 ) ) ;
#17895=CARTESIAN_POINT ( 'NONE',  ( -7.626320092023432196, 21.25423560278784407, -233.8867968595558295 ) ) ;
#17896=CARTESIAN_POINT ( 'NONE',  ( 11.91821674756695693, -1.593691010653677242, -227.2895864140137405 ) ) ;
#17897=CARTESIAN_POINT ( 'NONE',  ( 15.13105790938820228, -1.902449014147146178, -222.1588331224812407 ) ) ;
#17898=CARTESIAN_POINT ( 'NONE',  ( 14.20064147608437821, 14.63411858269657806, -233.6150408276221242 ) ) ;
#17899=CARTESIAN_POINT ( 'NONE',  ( 10.63406535173453271, 22.16595115341124256, -219.6461356279925781 ) ) ;
#17901=CARTESIAN_POINT ( 'NONE',  ( 26.97873870420736253, -17.71910932852193454, -225.8965020979516964 ) ) ;
#17903=CARTESIAN_POINT ( 'NONE',  ( -5.373457274256926652, 30.83572167890261184, -229.2199105909169532 ) ) ;
#17904=CARTESIAN_POINT ( 'NONE',  ( -5.568057711815838751, 28.69723585065299076, -232.1518503103610271 ) ) ;
#17905=CARTESIAN_POINT ( 'NONE',  ( 21.75737151495774313, -2.205713500382427750, -233.2756072794337285 ) ) ;
#17906=CARTESIAN_POINT ( 'NONE',  ( -24.02434186778878455, 18.57431834865475651, -228.2662945587547370 ) ) ;
#17908=CARTESIAN_POINT ( 'NONE',  ( 22.14341918773124362, -7.622004812940091689, -217.4502831791021720 ) ) ;
#17909=CARTESIAN_POINT ( 'NONE',  ( -6.593106361191484410, 26.27107262772703322, -231.8730401762632596 ) ) ;
#17910=CARTESIAN_POINT ( 'NONE',  ( 16.22460398937575121, -0.7285105026664867589, -219.3274985887512116 ) ) ;
#17911=CARTESIAN_POINT ( 'NONE',  ( -14.83974801774860630, 13.71714848582103485, -216.0935642439352762 ) ) ;
#17912=CARTESIAN_POINT ( 'NONE',  ( 26.48990917286906921, 12.16675355942207659, -225.0153622588060216 ) ) ;
#17913=CARTESIAN_POINT ( 'NONE',  ( 15.50884165284638705, 1.028647572718199843, -227.8181348745474679 ) ) ;
#17915=CARTESIAN_POINT ( 'NONE',  ( 5.585286719045844173, 27.51657303716567426, -222.4190945945824751 ) ) ;
#17916=CARTESIAN_POINT ( 'NONE',  ( -15.22366728182010043, -5.552021002219007961, -230.2511309519622671 ) ) ;
#17917=CARTESIAN_POINT ( 'NONE',  ( 5.623554730548537606, 15.65270319720736225, -231.3185741195121068 ) ) ;
#17918=CARTESIAN_POINT ( 'NONE',  ( -0.6614632862528592172, -26.57152937425246719, -233.3304277112415548 ) ) ;
#17921=CARTESIAN_POINT ( 'NONE',  ( -13.75208518020500748, 5.661250135068270239, -227.6647651141479685 ) ) ;
#17923=CARTESIAN_POINT ( 'NONE',  ( 13.37423534347618670, -3.100899090186935325, -222.2483675785374260 ) ) ;
#17924=CARTESIAN_POINT ( 'NONE',  ( 9.382249691333727881, 26.55946126407900820, -224.4468135941759215 ) ) ;
#17925=CARTESIAN_POINT ( 'NONE',  ( -13.96147744945181124, 5.260363697127891314, -222.3342733685200301 ) ) ;
#17926=CARTESIAN_POINT ( 'NONE',  ( -27.53108621362071773, 14.15137273650544536, -219.7961709676081625 ) ) ;
#17928=CARTESIAN_POINT ( 'NONE',  ( -10.89162261547930655, -11.18732543557264592, -227.7569336215896953 ) ) ;
#17929=CARTESIAN_POINT ( 'NONE',  ( 22.49659352743751128, 7.060662713609715979, -215.7089950799439180 ) ) ;
#17932=CARTESIAN_POINT ( 'NONE',  ( -13.21307282338718991, -4.958223064515467016, -219.4340824732878730 ) ) ;
#17933=CARTESIAN_POINT ( 'NONE',  ( -1.433739110790628102, 17.19322394474796667, -219.1420620387681879 ) ) ;
#17934=CARTESIAN_POINT ( 'NONE',  ( -19.67797246974518544, 1.229961341702398681, -219.4743747885323160 ) ) ;
#17935=CARTESIAN_POINT ( 'NONE',  ( -17.07311071032027172, 18.59516984069744794, -230.9440421721702137 ) ) ;
#17937=CARTESIAN_POINT ( 'NONE',  ( 4.952019330116582907, 28.88045068338265509, -217.6369327391592208 ) ) ;
#17938=CARTESIAN_POINT ( 'NONE',  ( -3.077342110593487945, -14.65776296416898816, -220.8866639047373610 ) ) ;
#17939=CARTESIAN_POINT ( 'NONE',  ( 1.525817648051120967, -14.82969601928396841, -225.8796824437346515 ) ) ;
#17941=CARTESIAN_POINT ( 'NONE',  ( 13.03557269046774714, 7.519834803053426775, -226.9490612297269081 ) ) ;
#17942=CARTESIAN_POINT ( 'NONE',  ( 22.14671607713456325, -14.13547298543019437, -218.1897693226341914 ) ) ;
#17943=CARTESIAN_POINT ( 'NONE',  ( -21.28605893225895684, -20.43870967537180050, -221.0356759888913700 ) ) ;
#17944=CARTESIAN_POINT ( 'NONE',  ( -5.902479482706956659, -14.78727544128710214, -218.5565286504736946 ) ) ;
#17945=CARTESIAN_POINT ( 'NONE',  ( 6.402706778685327116, 14.41397785959879307, -226.0127495172349086 ) ) ;
#17947=CARTESIAN_POINT ( 'NONE',  ( 17.32394486779715592, 4.028159306070694612, -218.4253989884176690 ) ) ;
#17948=CARTESIAN_POINT ( 'NONE',  ( 0.9046320824004248085, 13.39785254849979701, -226.4815711199935890 ) ) ;
#17949=CARTESIAN_POINT ( 'NONE',  ( 0.9458336400950161371, 17.49535648476021876, -228.8359568483051589 ) ) ;
#17950=CARTESIAN_POINT ( 'NONE',  ( 12.64197975508134597, -4.295353707277522304, -228.6481500018833799 ) ) ;
#17952=CARTESIAN_POINT ( 'NONE',  ( 9.774133712851615030, 11.09751083462123766, -229.6876724410067823 ) ) ;
#17953=CARTESIAN_POINT ( 'NONE',  ( -13.92941769543345032, 11.48925904027772127, -219.8938199480626281 ) ) ;
#17954=CARTESIAN_POINT ( 'NONE',  ( 11.21112214669106777, 5.418350954422431975, -227.6539796508718325 ) ) ;
#17955=CARTESIAN_POINT ( 'NONE',  ( -4.253447013113726527, -22.64852647464574531, -232.0531923962242615 ) ) ;
#17958=CARTESIAN_POINT ( 'NONE',  ( 10.50530447320976535, 20.19629329636330084, -217.1354359361034767 ) ) ;
#17959=CARTESIAN_POINT ( 'NONE',  ( 18.46162736253148395, -12.23454570505295358, -218.9425382959138062 ) ) ;
#17960=CARTESIAN_POINT ( 'NONE',  ( -16.32047052250102581, 2.570795953410685009, -230.9329235942756213 ) ) ;
#17962=CARTESIAN_POINT ( 'NONE',  ( -8.878187501988019648, -11.23476449186280846, -221.0271673637577123 ) ) ;
#17964=CARTESIAN_POINT ( 'NONE',  ( -0.1571923090946999446, 19.34188126963334398, -216.6893131123363787 ) ) ;
#17965=CARTESIAN_POINT ( 'NONE',  ( -0.4465333940385243228, 12.27026616490476485, -221.3722328744566425 ) ) ;
#17967=CARTESIAN_POINT ( 'NONE',  ( -18.09776816382430908, 23.50806826204562583, -229.9568677523880638 ) ) ;
#17968=CARTESIAN_POINT ( 'NONE',  ( 25.79934686323926840, -4.908228874239597417, -218.4849570602390543 ) ) ;
#17971=CARTESIAN_POINT ( 'NONE',  ( -11.33137429837660193, 27.25022425932026238, -230.1650924901870212 ) ) ;
#17972=CARTESIAN_POINT ( 'NONE',  ( 7.337960271553932046, -12.57654522398025065, -224.9099165242034530 ) ) ;
#17973=CARTESIAN_POINT ( 'NONE',  ( 27.32546652195855685, -7.354568365469916991, -229.0866163655393279 ) ) ;
#17974=CARTESIAN_POINT ( 'NONE',  ( -18.70100282803782576, 16.58357028540773115, -216.4425743468854080 ) ) ;
#17975=CARTESIAN_POINT ( 'NONE',  ( -16.36835685385702988, 8.002698209344293545, -233.7585018083067894 ) ) ;
#17977=CARTESIAN_POINT ( 'NONE',  ( -1.696080206444520844, 14.74162257415073540, -222.2455536759108838 ) ) ;
#17979=CARTESIAN_POINT ( 'NONE',  ( -20.05025075566126702, 1.207204931470905018, -215.1628017022767949 ) ) ;
#17980=CARTESIAN_POINT ( 'NONE',  ( -13.60885102855131201, -21.92822159330905762, -220.4851091041354607 ) ) ;
#17982=CARTESIAN_POINT ( 'NONE',  ( 13.82984244654956107, 22.51831320572884820, -232.1830460045772213 ) ) ;
#17983=CARTESIAN_POINT ( 'NONE',  ( -6.094651895680649467, 13.59752566126439177, -221.0608041154719103 ) ) ;
#17984=CARTESIAN_POINT ( 'NONE',  ( -14.98215928292561294, 22.79623052288931362, -230.3289734367122890 ) ) ;
#17985=CARTESIAN_POINT ( 'NONE',  ( -15.02851318684991000, -5.270497739200964205, -221.5518599052197146 ) ) ;
#17988=CARTESIAN_POINT ( 'NONE',  ( 19.30248206944178335, -1.297331563427565726, -230.8957665284791290 ) ) ;
#17989=CARTESIAN_POINT ( 'NONE',  ( -5.100309671427054603, -23.83006135775530510, -217.1425084463234612 ) ) ;
#17990=CARTESIAN_POINT ( 'NONE',  ( 14.23581535094758266, 1.730511134508401438, -227.4509761555696628 ) ) ;
#17991=CARTESIAN_POINT ( 'NONE',  ( 4.484811161826725900, 15.38298568785217313, -219.4617573400562662 ) ) ;
#17993=CARTESIAN_POINT ( 'NONE',  ( -22.32700334442577272, 3.978587747811427988, -218.4803616146862453 ) ) ;
#17994=CARTESIAN_POINT ( 'NONE',  ( 20.05374812456133782, 24.17492691056345677, -223.1494843338164458 ) ) ;
#17995=CARTESIAN_POINT ( 'NONE',  ( 13.69275646168278371, 8.674223198772375909, -220.8699857572541987 ) ) ;
#17997=CARTESIAN_POINT ( 'NONE',  ( -26.26363215285178043, -18.18116807333735352, -227.1727963224598739 ) ) ;
#17998=CARTESIAN_POINT ( 'NONE',  ( -7.349743644505656093, -15.31718010764164539, -232.4470764718129772 ) ) ;
#17999=CARTESIAN_POINT ( 'NONE',  ( 5.982950994121768673, -14.58086824529316594, -231.1438280359330975 ) ) ;
#18002=CARTESIAN_POINT ( 'NONE',  ( -1.837924626891132229, 29.27703531260187475, -227.2344808100871774 ) ) ;
#18003=CARTESIAN_POINT ( 'NONE',  ( 26.96734317869073294, -1.796611605495658681, -216.2358245450472509 ) ) ;
#18004=CARTESIAN_POINT ( 'NONE',  ( 28.22932473237819551, -8.039268142081398949, -226.6539694142420558 ) ) ;
#18005=CARTESIAN_POINT ( 'NONE',  ( -17.49393085256189906, 10.63366922396483361, -217.7502683347138657 ) ) ;
#18006=CARTESIAN_POINT ( 'NONE',  ( 16.96779410054824666, 23.69881408353223406, -220.2174342377987841 ) ) ;
#18007=CARTESIAN_POINT ( 'NONE',  ( 10.12648780932046755, 24.76571117977573522, -228.8499436907259792 ) ) ;
#18009=CARTESIAN_POINT ( 'NONE',  ( 4.375292991814291987, -28.67199747747994465, -220.8092881619367631 ) ) ;
#18011=CARTESIAN_POINT ( 'NONE',  ( -0.2758005215353623862, 11.79991891162212525, -226.8645588387054488 ) ) ;
#18012=CARTESIAN_POINT ( 'NONE',  ( -4.334570222994868161, 11.62786715207288601, -222.6396919303362267 ) ) ;
#18013=CARTESIAN_POINT ( 'NONE',  ( 18.84909589690502685, -4.856542942594316514, -217.9726137486037771 ) ) ;
#18014=CARTESIAN_POINT ( 'NONE',  ( -8.501641725227710111, 25.47064987787527102, -217.3358698761548737 ) ) ;
#18016=CARTESIAN_POINT ( 'NONE',  ( -5.974114889119001681, 17.52937113675171332, -232.3862906442651592 ) ) ;
#18017=CARTESIAN_POINT ( 'NONE',  ( 25.30941179858102430, 8.661697827793627624, -216.7530520919057722 ) ) ;
#18018=CARTESIAN_POINT ( 'NONE',  ( -17.88126539071149779, 5.766250685202066961, -232.9050303536861293 ) ) ;
#18019=CARTESIAN_POINT ( 'NONE',  ( 16.38151749656409351, 8.902090001712490874, -231.2955017965201989 ) ) ;
#18020=CARTESIAN_POINT ( 'NONE',  ( -29.74115761720981510, -1.844952462305729401, -220.6656484738778943 ) ) ;
#18022=CARTESIAN_POINT ( 'NONE',  ( -3.130305314451475418, 18.08417128930788209, -217.9058652980469333 ) ) ;
#18023=CARTESIAN_POINT ( 'NONE',  ( -13.33530847390368024, -5.065163879519744228, -226.5386329521395226 ) ) ;
#18024=CARTESIAN_POINT ( 'NONE',  ( 11.62313423782632782, 11.98467543564608029, -219.7293303032897995 ) ) ;
#18025=CARTESIAN_POINT ( 'NONE',  ( -7.928105003701093167, -26.09134507487772225, -231.8683635223868578 ) ) ;
#18027=CARTESIAN_POINT ( 'NONE',  ( -26.19327040236159831, 13.44417515682194875, -223.7810975255189874 ) ) ;
#18028=CARTESIAN_POINT ( 'NONE',  ( 0.000000000000000000, 0.000000000000000000, 0.000000000000000000 ) ) ;
#18029=CARTESIAN_POINT ( 'NONE',  ( 9.338484253624125486, -13.53666216847648052, -219.8958652322373837 ) ) ;
#18030=CARTESIAN_POINT ( 'NONE',  ( 3.635089269978064141, 27.05650967970794341, -222.4639105745756638 ) ) ;
#18031=CARTESIAN_POINT ( 'NONE',  ( -16.07193224038526580, 12.24477688577882439, -232.1409653212175499 ) ) ;
#18032=CARTESIAN_POINT ( 'NONE',  ( -16.85225081326727903, 6.237400186851330020, -234.5847093771173206 ) ) ;
#18033=CARTESIAN_POINT ( 'NONE',  ( -13.98007945013786291, -9.257046693524761949, -228.3752161438062842 ) ) ;
#18034=CARTESIAN_POINT ( 'NONE',  ( 19.13589083395335422, 16.69125564174534659, -234.7442498487877174 ) ) ;
#18037=CARTESIAN_POINT ( 'NONE',  ( -17.24073315697368969, -20.31883122441189826, -234.2947248507418863 ) ) ;
#18038=CARTESIAN_POINT ( 'NONE',  ( 5.359747511823000465, 20.14556701535824601, -232.9094821222151381 ) ) ;
#18039=CARTESIAN_POINT ( 'NONE',  ( 13.86383614057800884, 4.939477956453596441, -219.6543243356308324 ) ) ;
#18041=CARTESIAN_POINT ( 'NONE',  ( -5.727886109716582297, 15.25217619989539486, -230.5419623196804650 ) ) ;
#18042=CARTESIAN_POINT ( 'NONE',  ( 12.03015173539790617, 23.46358517874481109, -216.0611092640310744 ) ) ;
#18043=CARTESIAN_POINT ( 'NONE',  ( -5.100309671427054603, -23.83006135775530510, -217.1425084463234612 ) ) ;
#18044=CARTESIAN_POINT ( 'NONE',  ( 1.250172743705837641, -19.35180105203422940, -231.6553945523530729 ) ) ;
#18046=CARTESIAN_POINT ( 'NONE',  ( 14.98418162551161714, 4.450317369940187895, -227.9894155827521161 ) ) ;
#18047=CARTESIAN_POINT ( 'NONE',  ( 18.22947608839760747, -6.525328669204546905, -217.7409786913911205 ) ) ;
#18048=CARTESIAN_POINT ( 'NONE',  ( 13.78060503451313323, -0.3076571220309521904, -222.4352540772387101 ) ) ;
#18049=CARTESIAN_POINT ( 'NONE',  ( -13.05629324012484282, -10.24599397043673221, -218.7452066004821347 ) ) ;
#18050=CARTESIAN_POINT ( 'NONE',  ( 2.445562843591592372, 25.89340784564244657, -229.2671352353737859 ) ) ;
#18051=CARTESIAN_POINT ( 'NONE',  ( 20.62963957373278134, 2.372686805184054837, -232.5966151263358483 ) ) ;
#18052=CARTESIAN_POINT ( 'NONE',  ( 5.331555957413248059, 27.50712867803999728, -219.0801070358024276 ) ) ;
#18053=CARTESIAN_POINT ( 'NONE',  ( 3.755404788550845474, 24.96758616565139022, -220.0839658302907935 ) ) ;
#18054=CARTESIAN_POINT ( 'NONE',  ( 19.91550388961935525, -0.5333217442993671842, -216.6463151812154138 ) ) ;
#18056=CARTESIAN_POINT ( 'NONE',  ( 13.48097272627202159, 8.509510470709432894, -231.5257201610278059 ) ) ;
#18057=CARTESIAN_POINT ( 'NONE',  ( -21.26441444091935296, 10.69428164102106926, -219.3434466924981336 ) ) ;
#18058=CARTESIAN_POINT ( 'NONE',  ( -28.05279008194460744, 4.018900919424986284, -224.6698354068587662 ) ) ;
#18059=CARTESIAN_POINT ( 'NONE',  ( -0.3025942668150596315, -28.96010673020088788, -223.5534481764385646 ) ) ;
#18062=CARTESIAN_POINT ( 'NONE',  ( 23.04897566969193079, 17.95862962700741861, -223.6438515760422661 ) ) ;
#18063=CARTESIAN_POINT ( 'NONE',  ( 21.15565078817875388, -13.66792796406074295, -219.8984673185389624 ) ) ;
#18066=CARTESIAN_POINT ( 'NONE',  ( -6.870552667427666904, -18.85419487977974029, -216.2130481585807047 ) ) ;
#18068=CARTESIAN_POINT ( 'NONE',  ( 4.559463107227270662, 13.27337529356814017, -226.9596205199204633 ) ) ;
#18069=CARTESIAN_POINT ( 'NONE',  ( 2.660414182604129429, 28.99288898680367055, -232.5781547115647072 ) ) ;
#18071=CARTESIAN_POINT ( 'NONE',  ( -6.201839134465864767, 11.37481922992157379, -223.7040893475979146 ) ) ;
#18072=CARTESIAN_POINT ( 'NONE',  ( -29.05925532287432489, -3.238226816112620199, -230.1495230746535867 ) ) ;
#18073=CARTESIAN_POINT ( 'NONE',  ( 27.54201077264015396, -3.286392687948289648, -218.1575117614944190 ) ) ;
#18075=CARTESIAN_POINT ( 'NONE',  ( -8.823862513872974489, 14.92351368520778898, -217.1499513473673346 ) ) ;
#18076=CARTESIAN_POINT ( 'NONE',  ( -21.92622494339052608, -22.07770017127804962, -220.0303431275545165 ) ) ;
#18078=CARTESIAN_POINT ( 'NONE',  ( 26.54225689383817866, -6.924125931238839016, -230.1506921200174247 ) ) ;
#18079=CARTESIAN_POINT ( 'NONE',  ( -14.73016414256368911, 22.23431809695627237, -217.1425123644553707 ) ) ;
#18081=CARTESIAN_POINT ( 'NONE',  ( -15.64716994811699813, 6.210654946517923491, -217.0002936794128345 ) ) ;
#18083=CARTESIAN_POINT ( 'NONE',  ( 3.522445101072706475, 23.08420003150784439, -231.7850044194335055 ) ) ;
#18085=CARTESIAN_POINT ( 'NONE',  ( -12.10179538005628963, 1.685214252672075030, -222.4835512146784424 ) ) ;
#18086=CARTESIAN_POINT ( 'NONE',  ( -17.56620462375804692, -17.71942105192161065, -219.9081625180047013 ) ) ;
#18088=CARTESIAN_POINT ( 'NONE',  ( 16.96779410054824666, 23.69881408353223406, -220.2174342377987841 ) ) ;
#18089=CARTESIAN_POINT ( 'NONE',  ( 1.660345614755502686, 12.19060476922103931, -223.1112690039082906 ) ) ;
#18090=CARTESIAN_POINT ( 'NONE',  ( -19.94037810645588138, 20.40093185429846656, -220.0593903119159620 ) ) ;
#18091=CARTESIAN_POINT ( 'NONE',  ( -15.57180599510074437, -4.609960555941468918, -228.7341395176208323 ) ) ;
#18095=CARTESIAN_POINT ( 'NONE',  ( -18.46722752239034193, 0.9784074152395518809, -232.1633353206286188 ) ) ;
#18096=CARTESIAN_POINT ( 'NONE',  ( -13.04380155829002419, -28.08004287256819609, -224.7912146079995352 ) ) ;
#18097=CARTESIAN_POINT ( 'NONE',  ( 24.58316096239279602, 5.861425670879941485, -231.3104446318280623 ) ) ;
#18098=CARTESIAN_POINT ( 'NONE',  ( -3.060450601941519189, 13.29454208326677289, -222.0135664617158682 ) ) ;
#18102=CARTESIAN_POINT ( 'NONE',  ( -24.49083850720273148, 4.222094140707651100, -219.1543001448025905 ) ) ;
#18103=CARTESIAN_POINT ( 'NONE',  ( 10.82528077991200810, 8.849546035972329250, -221.2068619981234008 ) ) ;
#18105=CARTESIAN_POINT ( 'NONE',  ( 20.23125423326388628, 7.836699765464857137, -217.8891354894872450 ) ) ;
#18107=CARTESIAN_POINT ( 'NONE',  ( 20.39962514764921409, -3.647888038500222141, -219.1338420190236036 ) ) ;
#18108=CARTESIAN_POINT ( 'NONE',  ( -15.15819830826754355, -2.370657588173597841, -221.8013720140894236 ) ) ;
#18112=CARTESIAN_POINT ( 'NONE',  ( -16.13584396029534318, 23.78382729893626646, -231.6788043429177435 ) ) ;
#18113=CARTESIAN_POINT ( 'NONE',  ( 10.41909793732091494, -5.130961835214151279, -225.2553394319931783 ) ) ;
#18114=CIRCLE ( 'NONE', #15969, 1.000000000000013323 ) ;
#18115=CARTESIAN_POINT ( 'NONE',  ( 26.48152825632016061, -2.044474411990439666, -219.3412966555575565 ) ) ;
#18116=CARTESIAN_POINT ( 'NONE',  ( -13.31590776630363315, 5.340120742929252096, -225.6956515496373186 ) ) ;
#18117=CARTESIAN_POINT ( 'NONE',  ( 17.97920459523930958, 17.43922474653955490, -233.2737719749805763 ) ) ;
#18118=CARTESIAN_POINT ( 'NONE',  ( 7.497537106193371770, 19.52448593130572618, -231.1338690134634248 ) ) ;
#18120=CARTESIAN_POINT ( 'NONE',  ( 6.644147376113458847, -12.60537238651543923, -230.3381876225809037 ) ) ;
#18122=CARTESIAN_POINT ( 'NONE',  ( -5.467362224022371819, 23.92882567691090046, -234.7811165710531611 ) ) ;
#18123=CARTESIAN_POINT ( 'NONE',  ( -15.46752262371512820, 15.15798787883389487, -233.5981584775992701 ) ) ;
#18124=CARTESIAN_POINT ( 'NONE',  ( 17.03334375980016446, -6.184066897328505341, -231.2622903164569834 ) ) ;
#18125=CARTESIAN_POINT ( 'NONE',  ( -1.249406995060579062, 25.48934319316224162, -216.9406480707515072 ) ) ;
#18127=CARTESIAN_POINT ( 'NONE',  ( 2.987882271643250931, 28.57355997650491020, -217.8917278841813925 ) ) ;
#18128=CARTESIAN_POINT ( 'NONE',  ( 15.87399429023076003, -1.683916961781461552, -230.8621029165058758 ) ) ;
#18129=CARTESIAN_POINT ( 'NONE',  ( -17.39699619235753048, 15.64332637722790054, -216.0406373264262641 ) ) ;
#18131=CARTESIAN_POINT ( 'NONE',  ( 22.18132842682159733, 5.591149267797686839, -232.0584733989884114 ) ) ;
#18132=CARTESIAN_POINT ( 'NONE',  ( 9.214796078729456497, 26.59493510027307650, -225.5796848805584318 ) ) ;
#18135=CARTESIAN_POINT ( 'NONE',  ( 10.90137817157632227, 16.64712710991609868, -230.5401786220292593 ) ) ;
#18136=CARTESIAN_POINT ( 'NONE',  ( -15.27057301462635408, -17.00912219741827514, -233.6288396447818627 ) ) ;
#18137=CARTESIAN_POINT ( 'NONE',  ( 23.49048926389013658, 9.645778135078892035, -218.7307869890797463 ) ) ;
#18138=CARTESIAN_POINT ( 'NONE',  ( -7.007669255080013926, -23.60960382150139836, -233.3096631214588115 ) ) ;
#18140=CARTESIAN_POINT ( 'NONE',  ( -17.78731991475362406, 16.78509880370027929, -218.2387321183659310 ) ) ;
#18142=CARTESIAN_POINT ( 'NONE',  ( 20.07985072697885442, -15.33367264652052953, -217.4666949641080294 ) ) ;
#18143=CARTESIAN_POINT ( 'NONE',  ( 8.321021197036545303, 25.59447019508656140, -228.6184429848799482 ) ) ;
#18144=CARTESIAN_POINT ( 'NONE',  ( -11.94782396647286049, 8.456988817430419303, -225.5094493096559063 ) ) ;
#18145=CARTESIAN_POINT ( 'NONE',  ( -26.42613204384124259, 13.88327151024443395, -218.2510073314678323 ) ) ;
#18146=CARTESIAN_POINT ( 'NONE',  ( -25.33517302999029042, -8.734563104097837538, -228.3677567689655916 ) ) ;
#18147=CARTESIAN_POINT ( 'NONE',  ( 9.616550234602936342, 9.263684773868845923, -230.4827401731016607 ) ) ;
#18151=CARTESIAN_POINT ( 'NONE',  ( -9.601352586650603982, -12.91383303375239322, -233.5046259060385125 ) ) ;
#18152=CARTESIAN_POINT ( 'NONE',  ( 9.880827190695510964, 24.82036951119805579, -218.1633337467656020 ) ) ;
#18153=CARTESIAN_POINT ( 'NONE',  ( 26.91963614581376874, 6.107751173605064920, -232.2246916053503298 ) ) ;
#18154=CARTESIAN_POINT ( 'NONE',  ( -8.316505849089994129, 18.84563905716333210, -217.0138378867507640 ) ) ;
#18155=CARTESIAN_POINT ( 'NONE',  ( 12.99334571784053338, 27.47142594410712846, -219.5003755906066658 ) ) ;
#18156=CARTESIAN_POINT ( 'NONE',  ( 1.152695246012044095, -27.06931983241920747, -220.0193874843003528 ) ) ;
#18159=CARTESIAN_POINT ( 'NONE',  ( -1.981531036097845533, -15.05108582582333909, -227.0172948689592829 ) ) ;
#18160=CARTESIAN_POINT ( 'NONE',  ( 15.42212722119060864, 5.401662248084913465, -220.8333402320903645 ) ) ;
#18161=CARTESIAN_POINT ( 'NONE',  ( 13.38839277810360429, -5.174145297632733786, -223.8523798909600941 ) ) ;
#18162=CARTESIAN_POINT ( 'NONE',  ( -26.22594988380878789, -0.1068133454905619700, -219.1167922977186322 ) ) ;
#18164=CARTESIAN_POINT ( 'NONE',  ( -13.60146639818222702, -25.11808310587244009, -230.9974232610874196 ) ) ;
#18166=CARTESIAN_POINT ( 'NONE',  ( 12.11771628698343051, 17.56545729485151952, -218.0322663566023493 ) ) ;
#18168=CARTESIAN_POINT ( 'NONE',  ( -18.09994298044773942, 1.383435435878707320, -215.7801353739235708 ) ) ;
#18169=CARTESIAN_POINT ( 'NONE',  ( 4.484811161826725900, 15.38298568785217313, -219.4617573400562662 ) ) ;
#18170=CARTESIAN_POINT ( 'NONE',  ( -2.612157044224189484, 27.88031182936952135, -224.5292183073761692 ) ) ;
#18171=CARTESIAN_POINT ( 'NONE',  ( 15.13450096816097634, -26.20215934980152639, -231.3023426574493726 ) ) ;
#18172=CARTESIAN_POINT ( 'NONE',  ( 17.97920459523930958, 17.43922474653955490, -233.2737719749805763 ) ) ;
#18173=CARTESIAN_POINT ( 'NONE',  ( -12.69709334397052203, 10.59859500067950400, -221.6107941937004568 ) ) ;
#18174=CARTESIAN_POINT ( 'NONE',  ( -17.65933056022148762, 0.7424667221540405260, -229.0964312085266386 ) ) ;
#18175=CARTESIAN_POINT ( 'NONE',  ( -5.805911442544755552, -26.83424102279996504, -229.6222293353685302 ) ) ;
#18178=CARTESIAN_POINT ( 'NONE',  ( 14.39473142419577023, 15.98257177912839389, -217.4557725731239373 ) ) ;
#18179=CARTESIAN_POINT ( 'NONE',  ( 19.65870185572374140, -17.77243814521307641, -229.4329728153015253 ) ) ;
#18181=CARTESIAN_POINT ( 'NONE',  ( -6.163092920833200594, -27.00835405423771007, -232.1022292408408987 ) ) ;
#18183=CARTESIAN_POINT ( 'NONE',  ( -5.807479211365208727, 19.77444019604324410, -216.0778658752277863 ) ) ;
#18184=CARTESIAN_POINT ( 'NONE',  ( -4.531689447889125866, 14.11317536318881416, -231.6806015375303502 ) ) ;
#18186=CARTESIAN_POINT ( 'NONE',  ( -11.24282496690421596, 12.44430180464951086, -232.4405891940542404 ) ) ;
#18187=CARTESIAN_POINT ( 'NONE',  ( -26.09107693309126574, -10.38942742183557399, -230.9365759677854442 ) ) ;
#18190=CARTESIAN_POINT ( 'NONE',  ( -7.825349071214003693, 24.14595706726266755, -216.5959661901539732 ) ) ;
#18191=CARTESIAN_POINT ( 'NONE',  ( -9.601352586650603982, -12.91383303375239322, -233.5046259060385125 ) ) ;
#18192=CARTESIAN_POINT ( 'NONE',  ( 20.25084204406298127, -10.11176871144018818, -232.7817218064674591 ) ) ;
#18193=CARTESIAN_POINT ( 'NONE',  ( -24.02434186778878455, 18.57431834865475651, -228.2662945587547370 ) ) ;
#18194=CARTESIAN_POINT ( 'NONE',  ( -26.41026844077819291, 5.012316129610852933, -233.8406020309487872 ) ) ;
#18195=CARTESIAN_POINT ( 'NONE',  ( 5.563568780623874943, 21.86458082533069103, -218.6474243140849012 ) ) ;
#18197=CARTESIAN_POINT ( 'NONE',  ( -17.17143024911216287, 2.756036084795755681, -233.9491886983466316 ) ) ;
#18198=CARTESIAN_POINT ( 'NONE',  ( -6.911745780724915633, -15.37483479843349699, -221.7918796665217656 ) ) ;
#18200=EDGE_CURVE ( 'NONE', #161, #15629, #2312, .T. ) ;
#18202=CARTESIAN_POINT ( 'NONE',  ( -14.24491355791863612, 5.286533920242113105, -221.7104936369346433 ) ) ;
#18203=CARTESIAN_POINT ( 'NONE',  ( 10.40160332990717151, 27.59713857063802323, -221.5374724512453213 ) ) ;
#18204=CARTESIAN_POINT ( 'NONE',  ( -3.162425552858488143, 20.40327580806445695, -216.0004724541873316 ) ) ;
#18206=CARTESIAN_POINT ( 'NONE',  ( 19.75516891782859474, -3.344025276999063934, -216.3638920815759263 ) ) ;
#18209=CARTESIAN_POINT ( 'NONE',  ( -11.67631226053870996, 6.737291529340801333, -227.3110382950315227 ) ) ;
#18210=CARTESIAN_POINT ( 'NONE',  ( -5.579930056231209967, -28.86398153493815144, -221.8494056429758814 ) ) ;
#18212=CARTESIAN_POINT ( 'NONE',  ( 7.168644370073567806, 19.32044210858112265, -233.1278450877711634 ) ) ;
#18213=CARTESIAN_POINT ( 'NONE',  ( 14.72896495958249830, -2.932656333180209796, -224.3388645783988125 ) ) ;
#18215=CARTESIAN_POINT ( 'NONE',  ( -21.28804099221702018, -0.9277163183344186992, -219.0000000002572733 ) ) ;
#18216=CARTESIAN_POINT ( 'NONE',  ( 25.02650711521362936, 17.58144575069911042, -223.6165279156031431 ) ) ;
#18218=CARTESIAN_POINT ( 'NONE',  ( 15.48014850427786548, 1.347595008492685320, -222.3163328437614723 ) ) ;
#18219=CARTESIAN_POINT ( 'NONE',  ( 17.97843143658897347, 22.12221935793617078, -220.9346589834416079 ) ) ;
#18221=CARTESIAN_POINT ( 'NONE',  ( 16.44812011099018889, -8.334251478664654655, -229.6488175962812761 ) ) ;
#18222=CARTESIAN_POINT ( 'NONE',  ( -21.08965452150356867, -10.66825825602615296, -217.1903588586143314 ) ) ;
#18225=CARTESIAN_POINT ( 'NONE',  ( -6.331039912586185814, 17.62337457105953220, -233.2305561356360499 ) ) ;
#18226=CARTESIAN_POINT ( 'NONE',  ( 12.82249318900957391, -5.922664226158099510, -218.4318038749311768 ) ) ;
#18227=CARTESIAN_POINT ( 'NONE',  ( 16.06750045776299629, -1.909440863493336860, -220.4398626676318713 ) ) ;
#18228=CARTESIAN_POINT ( 'NONE',  ( -14.94667331530454213, 6.325011500478772142, -230.0242139990887154 ) ) ;
#18229=CARTESIAN_POINT ( 'NONE',  ( 12.93042813863272755, 0.4488092930645843914, -225.5263188864764174 ) ) ;
#18230=CARTESIAN_POINT ( 'NONE',  ( 19.67070349224072956, 16.44307963282299312, -220.0378483479504439 ) ) ;
#18232=CARTESIAN_POINT ( 'NONE',  ( 9.588041944343061118, -18.04984130968639633, -234.4334306750605776 ) ) ;
#18234=CARTESIAN_POINT ( 'NONE',  ( -31.84745724608465522, 5.474219582435353004, -224.7210333253351564 ) ) ;
#18235=CARTESIAN_POINT ( 'NONE',  ( 3.641537757978871248, 12.43698445400491437, -220.3805014257186485 ) ) ;
#18236=CARTESIAN_POINT ( 'NONE',  ( -0.8357710952364670876, 15.48480697989137234, -216.9118565312697910 ) ) ;
#18237=CARTESIAN_POINT ( 'NONE',  ( 26.09199240421564880, -11.03603815124446186, -222.0211821522591435 ) ) ;
#18238=CARTESIAN_POINT ( 'NONE',  ( -7.189383125363055349, 14.28512618638020548, -231.7475838278701303 ) ) ;
#18241=CARTESIAN_POINT ( 'NONE',  ( 2.804048525646705148, 30.59371477727813726, -220.6614663749232363 ) ) ;
#18242=CARTESIAN_POINT ( 'NONE',  ( -16.88427011841620029, 9.219900108593305887, -231.9155403335099948 ) ) ;
#18243=CARTESIAN_POINT ( 'NONE',  ( -9.540790481621398200, 9.981116473660406996, -228.6478862620407995 ) ) ;
#18244=CARTESIAN_POINT ( 'NONE',  ( 14.73698509926073186, 4.443590625350892331, -227.4062002049096236 ) ) ;
#18245=CARTESIAN_POINT ( 'NONE',  ( 9.382249691333727881, 26.55946126407900820, -224.4468135941759215 ) ) ;
#18248=CARTESIAN_POINT ( 'NONE',  ( 10.32480721127626033, 15.84468581819879773, -230.0799086455579072 ) ) ;
#18249=CARTESIAN_POINT ( 'NONE',  ( -21.08965452150356867, -10.66825825602615296, -217.1903588586143314 ) ) ;
#18250=CARTESIAN_POINT ( 'NONE',  ( 16.00819137755116373, 4.595691552992191120, -229.5669508871464757 ) ) ;
#18251=CARTESIAN_POINT ( 'NONE',  ( -3.642659482353215239, -13.10753628101701018, -222.6432544668793980 ) ) ;
#18253=CARTESIAN_POINT ( 'NONE',  ( -7.284474494690100776, 13.60812129561547046, -227.7414351104868331 ) ) ;
#18254=CARTESIAN_POINT ( 'NONE',  ( 14.68951511424354273, -18.85605729411972575, -217.5026406474102885 ) ) ;
#18255=CARTESIAN_POINT ( 'NONE',  ( 11.75069299018312208, 6.043853022588032253, -224.2604610870103841 ) ) ;
#18256=CARTESIAN_POINT ( 'NONE',  ( -16.57767831947938575, 23.50485984366324388, -222.7977068309636763 ) ) ;
#18257=CARTESIAN_POINT ( 'NONE',  ( -27.68973657932738064, 5.930811633061950694, -216.7842770206311513 ) ) ;
#18258=CARTESIAN_POINT ( 'NONE',  ( -13.57658210113775432, -10.11812981318216131, -221.5438341886276987 ) ) ;
#18259=CARTESIAN_POINT ( 'NONE',  ( 16.53896178738450828, 2.691624496798088462, -232.5974196329879078 ) ) ;
#18261=CARTESIAN_POINT ( 'NONE',  ( -20.50691009226094863, -22.90269851828495007, -230.6242067303112435 ) ) ;
#18262=CARTESIAN_POINT ( 'NONE',  ( 0.3632086708616291126, 21.06287758167331958, -232.5112839711303820 ) ) ;
#18263=CARTESIAN_POINT ( 'NONE',  ( -17.72669652144150376, 1.460525322529694581, -220.6883622781615202 ) ) ;
#18264=CARTESIAN_POINT ( 'NONE',  ( -15.77374768176864173, 20.07639682234129097, -218.6858893794192795 ) ) ;
#18265=CARTESIAN_POINT ( 'NONE',  ( 7.393167209263542539, 10.77319710117329699, -221.1179833906701049 ) ) ;
#18266=EDGE_LOOP ( 'NONE', ( #14653, #7522, #5932, #6771, #1569, #15987, #10227 ) ) ;
#18267=CARTESIAN_POINT ( 'NONE',  ( -5.474373895759362618, -29.29005893717160092, -223.2371403555430334 ) ) ;
#18269=CARTESIAN_POINT ( 'NONE',  ( 5.191785474240024456, -25.78595846473334419, -219.2330600099714673 ) ) ;
#18271=CARTESIAN_POINT ( 'NONE',  ( -21.73153953336191790, 8.758376218440917071, -235.2971293019126051 ) ) ;
#18272=CARTESIAN_POINT ( 'NONE',  ( 21.30961698559626427, -20.48616475849644303, -228.5322376518520002 ) ) ;
#18273=CARTESIAN_POINT ( 'NONE',  ( -23.10791503177032880, -5.282985115830100220, -217.6364121950018671 ) ) ;
#18274=CARTESIAN_POINT ( 'NONE',  ( -8.514447835183077018, -10.26590951297754195, -225.5321622820681569 ) ) ;
#18275=CARTESIAN_POINT ( 'NONE',  ( 14.87635807518583775, 11.13002414557121789, -232.1789382499626981 ) ) ;
#18277=CARTESIAN_POINT ( 'NONE',  ( -12.33997807949817904, 15.01940705987184188, -217.6798968600957380 ) ) ;
#18278=CARTESIAN_POINT ( 'NONE',  ( 1.773982976645536835, 19.12448993322812285, -233.2315972735944172 ) ) ;
#18279=CARTESIAN_POINT ( 'NONE',  ( 11.39755372583812587, 20.40856199875060639, -231.2895618162029621 ) ) ;
#18280=CARTESIAN_POINT ( 'NONE',  ( 22.52555938611480002, -22.70209057424856525, -227.7033606670069332 ) ) ;
#18281=CARTESIAN_POINT ( 'NONE',  ( 10.12956299421491302, 11.38773431477224385, -230.3175791991728829 ) ) ;
#18282=CARTESIAN_POINT ( 'NONE',  ( -16.58624905143161143, 8.715293938925766426, -220.0618460037763384 ) ) ;
#18283=CARTESIAN_POINT ( 'NONE',  ( 1.366658787427950772, -15.59113167952139456, -228.2894046839634257 ) ) ;
#18284=CARTESIAN_POINT ( 'NONE',  ( -16.20072894238734307, 0.5024448614660336210, -230.4554067149722130 ) ) ;
#18286=CARTESIAN_POINT ( 'NONE',  ( 21.25094435758043332, 17.68230636442804027, -229.7964888993842010 ) ) ;
#18287=CARTESIAN_POINT ( 'NONE',  ( 12.89329787743523070, -9.350464391519500040, -225.0861735818250224 ) ) ;
#18291=CARTESIAN_POINT ( 'NONE',  ( -9.606889355748592152, -11.26588727105406385, -229.9123324032181586 ) ) ;
#18292=CARTESIAN_POINT ( 'NONE',  ( 0.2389779871941385414, 16.64595486589868045, -218.1658233406367629 ) ) ;
#18293=CARTESIAN_POINT ( 'NONE',  ( 3.764125772070460396, 11.78312483992801596, -228.3484643988637970 ) ) ;
#18295=CARTESIAN_POINT ( 'NONE',  ( -0.9414827276148034496, 23.96885519606619752, -216.4491898092606164 ) ) ;
#18296=CARTESIAN_POINT ( 'NONE',  ( -28.57583275380518018, -9.842401781236429059, -222.4643230566485386 ) ) ;
#18299=CARTESIAN_POINT ( 'NONE',  ( -2.208416658185406334, 29.10348627872611615, -219.8480645685746424 ) ) ;
#18300=CARTESIAN_POINT ( 'NONE',  ( -4.398080837965281376, -27.92536303359771566, -232.3360949592949112 ) ) ;
#18301=CARTESIAN_POINT ( 'NONE',  ( 24.80560757033128993, -15.22139526172250079, -221.3338856610240271 ) ) ;
#18302=CARTESIAN_POINT ( 'NONE',  ( -3.755296588130283553, 23.77975947300719284, -233.7323173085780752 ) ) ;
#18303=CARTESIAN_POINT ( 'NONE',  ( -24.79170285622992509, 4.551775110860766915, -234.5907228154019322 ) ) ;
#18304=CARTESIAN_POINT ( 'NONE',  ( 3.755480357635514022, 24.23367984900377436, -231.4105847235276201 ) ) ;
#18306=CARTESIAN_POINT ( 'NONE',  ( 14.32363442937021425, 2.978337679677412808, -227.0386046113487453 ) ) ;
#18307=CARTESIAN_POINT ( 'NONE',  ( -21.61315260466662380, -9.974349528768403417, -231.2583083768228960 ) ) ;
#18309=CARTESIAN_POINT ( 'NONE',  ( -14.94640692938030746, 5.382918922058764544, -220.5478552936960455 ) ) ;
#18310=CARTESIAN_POINT ( 'NONE',  ( 2.471164685565028662, 14.01327037412690935, -223.4905256513065410 ) ) ;
#18311=CARTESIAN_POINT ( 'NONE',  ( -5.562203253303141359, 12.75725363875033302, -225.3078268727488478 ) ) ;
#18312=CARTESIAN_POINT ( 'NONE',  ( -14.97948828349161232, -4.621108923465524931, -227.6270126398174796 ) ) ;
#18315=CARTESIAN_POINT ( 'NONE',  ( -13.83274569775339202, 16.20364235096346661, -234.0851861771356539 ) ) ;
#18316=CARTESIAN_POINT ( 'NONE',  ( -19.49800774256867086, -24.03546784425654792, -228.3621204403185061 ) ) ;
#18317=CARTESIAN_POINT ( 'NONE',  ( 14.80138866163881772, 1.641909370019589032, -227.5118825796487272 ) ) ;
#18318=CARTESIAN_POINT ( 'NONE',  ( 13.43170911749896490, 19.07691563292472026, -232.7497845103644636 ) ) ;
#18321=CARTESIAN_POINT ( 'NONE',  ( -13.01696012539752445, 9.878799299062107409, -218.8446158128127195 ) ) ;
#18322=EDGE_CURVE ( 'NONE', #4932, #2027, #16832, .T. ) ;
#18323=CARTESIAN_POINT ( 'NONE',  ( 13.14260364752544596, 5.866423290307341887, -222.7705901084601408 ) ) ;
#18325=CARTESIAN_POINT ( 'NONE',  ( 15.61962121506769385, 4.525360868525488911, -229.0684696061408090 ) ) ;
#18327=CARTESIAN_POINT ( 'NONE',  ( 16.03897629125586377, -3.546747291816754633, -223.1229430630804700 ) ) ;
#18328=CARTESIAN_POINT ( 'NONE',  ( -22.53818779203657741, -7.663114047788936567, -232.6164956747681458 ) ) ;
#18331=CARTESIAN_POINT ( 'NONE',  ( -4.558896566524145655, 13.01459016691503301, -228.3167740496058684 ) ) ;
#18332=CARTESIAN_POINT ( 'NONE',  ( 30.90240445905660138, -9.617167762261830788, -225.5262352394493064 ) ) ;
#18333=CARTESIAN_POINT ( 'NONE',  ( 28.36095019830170472, -8.296631283839911220, -225.2861439608085448 ) ) ;
#18334=CARTESIAN_POINT ( 'NONE',  ( -15.82622499106666325, 9.895986579907866343, -218.5115209877527604 ) ) ;
#18335=CARTESIAN_POINT ( 'NONE',  ( 13.19406830060760605, 4.163358546877222288, -228.8532745215267425 ) ) ;
#18336=CARTESIAN_POINT ( 'NONE',  ( 24.93482953594869755, 13.13888391581411241, -222.4369546851285691 ) ) ;
#18337=CARTESIAN_POINT ( 'NONE',  ( 3.813635332914135923, -14.61080527247722927, -220.2619188551939828 ) ) ;
#18338=CARTESIAN_POINT ( 'NONE',  ( 18.54610009393809023, 0.6523581019769808531, -231.1787333216317677 ) ) ;
#18339=CARTESIAN_POINT ( 'NONE',  ( -10.54177647804913320, 7.401649028325941515, -220.3980514230326264 ) ) ;
#18340=CARTESIAN_POINT ( 'NONE',  ( 12.90536070039565963, 17.66816134723717724, -234.8562535614228750 ) ) ;
#18341=CARTESIAN_POINT ( 'NONE',  ( 2.660414182604129429, 28.99288898680367055, -232.5781547115647072 ) ) ;
#18342=CARTESIAN_POINT ( 'NONE',  ( 14.50342097185254353, -4.720444175079822280, -222.5922120714632513 ) ) ;
#18343=CARTESIAN_POINT ( 'NONE',  ( -1.881996891245037995, 28.05344686410985489, -218.6379207300106202 ) ) ;
#18344=CARTESIAN_POINT ( 'NONE',  ( -21.93900267957129557, 7.862893636934532360, -233.4951761057262161 ) ) ;
#18345=CARTESIAN_POINT ( 'NONE',  ( 18.15173157547545557, 23.32481284044927961, -217.8532150843729482 ) ) ;
#18346=CARTESIAN_POINT ( 'NONE',  ( -18.88344489807484905, 1.071113352238720617, -230.0966926586188208 ) ) ;
#18347=CARTESIAN_POINT ( 'NONE',  ( -13.55591840520136770, 8.363404288414606924, -231.2690188357804857 ) ) ;
#18348=CARTESIAN_POINT ( 'NONE',  ( 27.75679124201660741, 4.911524026080384075, -221.4430403652340829 ) ) ;
#18349=CARTESIAN_POINT ( 'NONE',  ( 7.804112641607792611, 19.76858558208418515, -218.6463059509973164 ) ) ;
#18350=CARTESIAN_POINT ( 'NONE',  ( 15.58663895521930876, 0.3114376099562851108, -227.9849797934280957 ) ) ;
#18352=CARTESIAN_POINT ( 'NONE',  ( 10.89019654021101857, 23.08162452736882031, -220.1893104909416934 ) ) ;
#18353=CARTESIAN_POINT ( 'NONE',  ( -21.28605893225895684, -20.43870967537180050, -221.0356759888913700 ) ) ;
#18354=CARTESIAN_POINT ( 'NONE',  ( 14.19800769603076240, 4.587407146151301518, -224.2928935459285071 ) ) ;
#18355=CARTESIAN_POINT ( 'NONE',  ( -8.609577223708431148, -18.69066821291321290, -217.1995118692595099 ) ) ;
#18357=CARTESIAN_POINT ( 'NONE',  ( -4.490213599459100813, 14.55066867058898694, -222.6488251579668827 ) ) ;
#18359=CARTESIAN_POINT ( 'NONE',  ( 15.50624253654579654, -15.96056326703506478, -233.0338314371582840 ) ) ;
#18361=CARTESIAN_POINT ( 'NONE',  ( 12.14863411169100971, 10.95505907656739097, -219.3725293661985063 ) ) ;
#18362=CARTESIAN_POINT ( 'NONE',  ( -10.91003322996498071, 12.84665145358222382, -229.9786893781767958 ) ) ;
#18363=CARTESIAN_POINT ( 'NONE',  ( -20.06846544527470400, 7.877362284741439069, -235.3910773253824402 ) ) ;
#18364=CARTESIAN_POINT ( 'NONE',  ( -14.79915263310685347, -6.493660518011266092, -224.0818296219458716 ) ) ;
#18366=CARTESIAN_POINT ( 'NONE',  ( -24.49083850720273148, 4.222094140707651100, -219.1543001448025905 ) ) ;
#18368=CARTESIAN_POINT ( 'NONE',  ( -24.78158512205813224, 1.917202307505101455, -217.2232489266994833 ) ) ;
#18369=CARTESIAN_POINT ( 'NONE',  ( 14.63115627273841923, 9.024791562541032874, -232.5054678133655841 ) ) ;
#18370=CARTESIAN_POINT ( 'NONE',  ( -16.03353370602922467, 4.897644413504528060, -222.5335369890782999 ) ) ;
#18371=CARTESIAN_POINT ( 'NONE',  ( 2.987882271643250931, 28.57355997650491020, -217.8917278841813925 ) ) ;
#18372=CARTESIAN_POINT ( 'NONE',  ( 20.05374812456133782, 24.17492691056345677, -223.1494843338164458 ) ) ;
#18373=CARTESIAN_POINT ( 'NONE',  ( -11.90549671174648694, -23.44716645851259784, -216.8989558407570257 ) ) ;
#18375=CARTESIAN_POINT ( 'NONE',  ( 6.930886114109415352, -28.33506752827666020, -226.0544877841801110 ) ) ;
#18376=CARTESIAN_POINT ( 'NONE',  ( -16.85225081326727903, 6.237400186851330020, -234.5847093771173206 ) ) ;
#18377=CARTESIAN_POINT ( 'NONE',  ( 19.06212547406409641, -9.287000003594721775, -232.7453815625877667 ) ) ;
#18378=CARTESIAN_POINT ( 'NONE',  ( 29.31647908907816102, 0.9594737942742700421, -228.5782466420670858 ) ) ;
#18380=CARTESIAN_POINT ( 'NONE',  ( -15.48425879135615446, -25.29886615046042309, -220.6886037686364261 ) ) ;
#18381=CARTESIAN_POINT ( 'NONE',  ( 10.49810582199713416, 9.357428619962972149, -224.5466107281195605 ) ) ;
#18383=CARTESIAN_POINT ( 'NONE',  ( -8.112279890008961658, 11.99566605360304727, -225.9834628568286519 ) ) ;
#18384=CARTESIAN_POINT ( 'NONE',  ( 11.41090957555148222, 16.52772439454343711, -218.2458222691329013 ) ) ;
#18385=CARTESIAN_POINT ( 'NONE',  ( 4.907833106823921376, 13.98151846258800290, -229.0190609869640923 ) ) ;
#18386=CARTESIAN_POINT ( 'NONE',  ( 19.61276001257277102, 19.97122404150989894, -229.5162757829903342 ) ) ;
#18387=CARTESIAN_POINT ( 'NONE',  ( 26.60633779560760459, -14.33430814915920593, -230.5388497754989885 ) ) ;
#18388=CARTESIAN_POINT ( 'NONE',  ( 20.05202556141620107, 8.012988804822112954, -215.8722494878839200 ) ) ;
#18389=CARTESIAN_POINT ( 'NONE',  ( -9.007976471255481954, 12.60968992764439633, -227.9367755778692981 ) ) ;
#18390=CARTESIAN_POINT ( 'NONE',  ( -10.06927776881013514, -17.00317020600589402, -217.8513858272130790 ) ) ;
#18394=CARTESIAN_POINT ( 'NONE',  ( 13.43730899468209294, 8.427513769504761498, -221.4030804848920297 ) ) ;
#18395=CARTESIAN_POINT ( 'NONE',  ( 9.552164729858477088, -28.54380927792562872, -224.2925619065192677 ) ) ;
#18396=CARTESIAN_POINT ( 'NONE',  ( -14.24491355791863612, 5.286533920242113105, -221.7104936369346433 ) ) ;
#18397=CARTESIAN_POINT ( 'NONE',  ( -14.24095617957673632, -25.86326826095433162, -229.7068514753157160 ) ) ;
#18399=CARTESIAN_POINT ( 'NONE',  ( 15.96089671440110713, 1.143943728337336374, -218.3532651118343892 ) ) ;
#18402=CARTESIAN_POINT ( 'NONE',  ( -4.619644865335168049, 14.75104250038670450, -232.3086264397671812 ) ) ;
#18404=CARTESIAN_POINT ( 'NONE',  ( -2.808235066048971440, 30.42019778760651150, -222.6481917607299295 ) ) ;
#18405=CARTESIAN_POINT ( 'NONE',  ( -18.41550138691291139, -5.273244084890690075, -216.7348800533310964 ) ) ;
#18408=CARTESIAN_POINT ( 'NONE',  ( -3.368164009525018265, 19.03203264544105622, -233.5986411977714567 ) ) ;
#18409=CARTESIAN_POINT ( 'NONE',  ( -6.645226799955220365, -27.24439832571371767, -217.1032720093393493 ) ) ;
#18410=CARTESIAN_POINT ( 'NONE',  ( 8.332496243628455090, -29.79192972398156769, -226.1452587264855367 ) ) ;
#18413=CARTESIAN_POINT ( 'NONE',  ( -11.11821474075380678, 16.53100589793018926, -232.3736596382188395 ) ) ;
#18414=CARTESIAN_POINT ( 'NONE',  ( 8.162622027327667951, 13.88735946031204094, -224.7165241036068153 ) ) ;
#18415=CARTESIAN_POINT ( 'NONE',  ( -18.46722752239034193, 0.9784074152395518809, -232.1633353206286188 ) ) ;
#18416=CARTESIAN_POINT ( 'NONE',  ( -17.07051451008491938, 15.19890664381897949, -233.6014043774825666 ) ) ;
#18417=CARTESIAN_POINT ( 'NONE',  ( -26.24201160508392761, -9.884581200937399004, -221.6903139798603206 ) ) ;
#18418=CARTESIAN_POINT ( 'NONE',  ( -14.22255565734842619, 21.32307452572284134, -218.8849463683180261 ) ) ;
#18419=CARTESIAN_POINT ( 'NONE',  ( 20.05202556141620107, 8.012988804822112954, -215.8722494878839200 ) ) ;
#18420=CARTESIAN_POINT ( 'NONE',  ( 2.631948090663005946, 31.21493676147814611, -222.3107766067421380 ) ) ;
#18421=CARTESIAN_POINT ( 'NONE',  ( 11.81564506561547390, -6.597897255275705142, -225.1493936678799628 ) ) ;
#18424=CARTESIAN_POINT ( 'NONE',  ( -9.540790481621398200, 9.981116473660406996, -228.6478862620407995 ) ) ;
#18425=CARTESIAN_POINT ( 'NONE',  ( -12.75534255189586652, -28.05386989040209400, -226.4018635127162327 ) ) ;
#18426=CARTESIAN_POINT ( 'NONE',  ( 17.34727976380017722, 4.822939981779328811, -230.8836217450937909 ) ) ;
#18427=CARTESIAN_POINT ( 'NONE',  ( 7.743212835174657194, 11.90778931056080481, -226.0491028376908105 ) ) ;
#18431=CARTESIAN_POINT ( 'NONE',  ( -22.57859951143173660, 16.82392524473188899, -219.5628058978911383 ) ) ;
#18434=CARTESIAN_POINT ( 'NONE',  ( 15.07212457412616224, 2.472408313530222390, -227.3472192494155024 ) ) ;
#18436=CARTESIAN_POINT ( 'NONE',  ( 14.86622134549281427, 0.1848946639127413416, -222.0051228238385477 ) ) ;
#18437=CARTESIAN_POINT ( 'NONE',  ( 19.20300624114736721, 0.6066039755357417462, -231.5046416827383950 ) ) ;
#18438=CARTESIAN_POINT ( 'NONE',  ( -17.96792326766206926, -0.6237852504629022299, -217.9759415197746932 ) ) ;
#18439=CARTESIAN_POINT ( 'NONE',  ( 19.48258831087540344, -3.612136468958778934, -219.4255404790470436 ) ) ;
#18440=CARTESIAN_POINT ( 'NONE',  ( -14.37894460687751597, -1.926260335694933268, -225.0161641904981593 ) ) ;
#18443=CARTESIAN_POINT ( 'NONE',  ( 6.685304925496912354, 17.61973327427626046, -230.4152170797364931 ) ) ;
#18444=CARTESIAN_POINT ( 'NONE',  ( 8.773758653197093693, -22.96626044227292951, -216.4280442219689178 ) ) ;
#18445=CARTESIAN_POINT ( 'NONE',  ( 12.84024077373997841, -14.50125846907313054, -216.8496453050001946 ) ) ;
#18446=CARTESIAN_POINT ( 'NONE',  ( -15.83178333309709629, 2.467763724635483324, -230.4064772870105458 ) ) ;
#18447=CARTESIAN_POINT ( 'NONE',  ( 13.16746181015946959, 0.3897807143096829741, -227.1676274388083243 ) ) ;
#18448=CARTESIAN_POINT ( 'NONE',  ( 17.42772712443221650, 11.35756022693713341, -231.2166398222404382 ) ) ;
#18449=CARTESIAN_POINT ( 'NONE',  ( 2.859576749041432553, -13.55982619688326984, -227.5954719880151345 ) ) ;
#18452=CARTESIAN_POINT ( 'NONE',  ( -24.77996431573922820, 10.49354383977773786, -234.1655613096203581 ) ) ;
#18454=CARTESIAN_POINT ( 'NONE',  ( 11.84598249547323690, 10.36127485500543699, -218.5481300776139904 ) ) ;
#18455=CARTESIAN_POINT ( 'NONE',  ( 3.744112528862662881, 31.76296354843916703, -227.8872370379487506 ) ) ;
#18456=CARTESIAN_POINT ( 'NONE',  ( 16.71284463105542883, -8.832875790685479345, -219.1937169315102949 ) ) ;
#18457=CARTESIAN_POINT ( 'NONE',  ( -8.966714183099560032, 19.05224306381768073, -234.0879867025980445 ) ) ;
#18458=CARTESIAN_POINT ( 'NONE',  ( -25.80904414196669450, 12.19501778665756220, -219.1732313092283846 ) ) ;
#18459=CARTESIAN_POINT ( 'NONE',  ( 9.986779374595107228, 29.47523823012521049, -229.5287702428778687 ) ) ;
#18460=CARTESIAN_POINT ( 'NONE',  ( -20.95553895916151177, 12.88782924195037438, -232.2493899712447956 ) ) ;
#18461=CARTESIAN_POINT ( 'NONE',  ( -3.205260335674071648, 17.52234722004434531, -232.9754319808710363 ) ) ;
#18464=CARTESIAN_POINT ( 'NONE',  ( 3.174664235197445006, 17.30896320251298448, -221.0803896709622620 ) ) ;
#18466=CARTESIAN_POINT ( 'NONE',  ( 27.92729748684602598, -8.572309054117944527, -222.6487661343338686 ) ) ;
#18469=CARTESIAN_POINT ( 'NONE',  ( 20.34032485158648029, 2.741617426884598530, -217.9827731991294968 ) ) ;
#18470=CARTESIAN_POINT ( 'NONE',  ( -10.89162261547930655, -11.18732543557264592, -227.7569336215896953 ) ) ;
#18472=CARTESIAN_POINT ( 'NONE',  ( -4.073886805163430935, 14.35067061637828623, -226.4733297826468572 ) ) ;
#18473=CARTESIAN_POINT ( 'NONE',  ( 14.46917091355089902, -8.493370822347547033, -231.7163745456035997 ) ) ;
#18474=CARTESIAN_POINT ( 'NONE',  ( 21.24820809707834357, 20.59746639607275398, -225.8540969741923732 ) ) ;
#18475=CARTESIAN_POINT ( 'NONE',  ( -16.50467377682197423, 21.56569464670658220, -229.9175202103629374 ) ) ;
#18476=CARTESIAN_POINT ( 'NONE',  ( -9.045741320599788082, 11.46901338045063312, -219.0588111342715365 ) ) ;
#18478=CARTESIAN_POINT ( 'NONE',  ( -13.39502153392024475, -9.880902914596246589, -222.0112808355889342 ) ) ;
#18480=CARTESIAN_POINT ( 'NONE',  ( -17.59913672443795463, -0.5356773789333074687, -220.7342471185320960 ) ) ;
#18482=CARTESIAN_POINT ( 'NONE',  ( -22.30463520409893263, -0.6981587008078518064, -233.9491726243120127 ) ) ;
#18483=CARTESIAN_POINT ( 'NONE',  ( 21.38922145650625239, 17.10616209967719215, -217.8354246241890451 ) ) ;
#18485=CARTESIAN_POINT ( 'NONE',  ( -17.64438593497130370, 2.824953307685432069, -229.4443205246391813 ) ) ;
#18486=CARTESIAN_POINT ( 'NONE',  ( 11.20713200305815427, 28.28922876448651635, -219.1239564724620834 ) ) ;
#18488=CARTESIAN_POINT ( 'NONE',  ( 25.60482246989237609, 8.614967517510873307, -219.3103232513597618 ) ) ;
#18490=CARTESIAN_POINT ( 'NONE',  ( -8.763358281418030415, -9.103836352148345412, -222.0692104753270257 ) ) ;
#18492=CARTESIAN_POINT ( 'NONE',  ( -16.87231408860552051, -20.68405295654727993, -231.0270656955280515 ) ) ;
#18493=CARTESIAN_POINT ( 'NONE',  ( -31.04415783139704388, 5.868882651865275690, -221.1472518903637194 ) ) ;
#18494=CARTESIAN_POINT ( 'NONE',  ( 10.10435529162921853, -13.32996982371095918, -231.5224098423250894 ) ) ;
#18495=CARTESIAN_POINT ( 'NONE',  ( 22.47485217157460724, -0.5904823501021798648, -216.4383471256914220 ) ) ;
#18496=CARTESIAN_POINT ( 'NONE',  ( -15.46216926290318305, -2.495270579625169738, -221.2150947962298631 ) ) ;
#18497=CARTESIAN_POINT ( 'NONE',  ( 19.70286159681817750, 17.87637900817293612, -218.6154571368943493 ) ) ;
#18499=CARTESIAN_POINT ( 'NONE',  ( -12.89119823113977503, 10.10140484475961564, -218.5945808114896636 ) ) ;
#18500=CARTESIAN_POINT ( 'NONE',  ( 16.73391517716289911, 11.95167056011791828, -233.0268722588312755 ) ) ;
#18502=CARTESIAN_POINT ( 'NONE',  ( 16.84848658399567611, 11.39632653812981644, -217.9589513831453473 ) ) ;
#18503=CARTESIAN_POINT ( 'NONE',  ( 6.295505112925526170, 15.36201163567862693, -221.5772643759389098 ) ) ;
#18504=CARTESIAN_POINT ( 'NONE',  ( 18.17041142304332624, -16.27896884253082987, -234.9734867155044356 ) ) ;
#18505=CARTESIAN_POINT ( 'NONE',  ( -8.316505849089994129, 18.84563905716333210, -217.0138378867507640 ) ) ;
#18506=CARTESIAN_POINT ( 'NONE',  ( -21.08008464085897060, -0.9048411197481797119, -217.0000000010748522 ) ) ;
#18508=CARTESIAN_POINT ( 'NONE',  ( 17.43816562714825125, 15.15720016074785903, -232.3748236813696906 ) ) ;
#18509=CARTESIAN_POINT ( 'NONE',  ( 7.470327549107519616, -12.61959153319410909, -223.5186783388273568 ) ) ;
#18510=CARTESIAN_POINT ( 'NONE',  ( -15.82622499106666325, 9.895986579907866343, -218.5115209877527604 ) ) ;
#18511=CARTESIAN_POINT ( 'NONE',  ( -4.715783688792956063, 28.29821729825949816, -228.0423900005874600 ) ) ;
#18512=CARTESIAN_POINT ( 'NONE',  ( -14.78079095050690661, -5.416970230978240153, -229.7193632018645246 ) ) ;
#18513=CARTESIAN_POINT ( 'NONE',  ( 17.57135037026572277, 0.09191994211922807634, -232.8447871904542410 ) ) ;
#18515=CARTESIAN_POINT ( 'NONE',  ( 9.818699534354031755, 13.69084898312510390, -233.4870046949650089 ) ) ;
#18516=CARTESIAN_POINT ( 'NONE',  ( 4.340445191644851874, 29.86837761166362881, -227.4879512554873315 ) ) ;
#18517=CARTESIAN_POINT ( 'NONE',  ( 22.90686649137879627, -15.60507238429272192, -227.8443525802422585 ) ) ;
#18521=CARTESIAN_POINT ( 'NONE',  ( 4.484811161826725900, 15.38298568785217313, -219.4617573400562662 ) ) ;
#18522=CARTESIAN_POINT ( 'NONE',  ( -14.25383187134801588, -24.74900029534085633, -216.9920501705437630 ) ) ;
#18523=CARTESIAN_POINT ( 'NONE',  ( 7.958080982411646076, -16.12895853103474408, -217.0903302464454612 ) ) ;
#18524=CARTESIAN_POINT ( 'NONE',  ( 11.32394539683753720, -15.63383003174572572, -233.0723040138117881 ) ) ;
#18525=CARTESIAN_POINT ( 'NONE',  ( -8.548213857283494477, 12.07277636836182211, -222.5354997492170241 ) ) ;
#18526=CARTESIAN_POINT ( 'NONE',  ( 12.00334754111224100, 12.62951371569041115, -228.5814949098771649 ) ) ;
#18528=CARTESIAN_POINT ( 'NONE',  ( -16.36835685385702988, 8.002698209344293545, -233.7585018083067894 ) ) ;
#18529=CARTESIAN_POINT ( 'NONE',  ( -20.35224420216377439, -13.00389602580315085, -219.1266045330881980 ) ) ;
#18530=CARTESIAN_POINT ( 'NONE',  ( -9.661739055621840322, 20.41227307912577871, -232.0920144483423257 ) ) ;
#18531=CARTESIAN_POINT ( 'NONE',  ( 26.59731715018858011, 13.56210517473685329, -229.5787264587298466 ) ) ;
#18532=CARTESIAN_POINT ( 'NONE',  ( -6.388048297418547961, 21.92257289597608150, -233.3290245341164848 ) ) ;
#18533=CARTESIAN_POINT ( 'NONE',  ( 24.68599888815047194, -16.20242508705913309, -228.6174911781957633 ) ) ;
#18538=CARTESIAN_POINT ( 'NONE',  ( -18.47334320050258327, 24.79293862780133040, -226.9986786077537317 ) ) ;
#18539=CARTESIAN_POINT ( 'NONE',  ( -20.48546531633906298, -12.23885716989380157, -214.8851912114337210 ) ) ;
#18541=CARTESIAN_POINT ( 'NONE',  ( 7.769483725421269860, 20.68783433326350263, -233.2348178266662728 ) ) ;
#18543=CARTESIAN_POINT ( 'NONE',  ( 22.14671607713456325, -14.13547298543019437, -218.1897693226341914 ) ) ;
#18545=CARTESIAN_POINT ( 'NONE',  ( -17.88126539071149779, 5.766250685202066961, -232.9050303536861293 ) ) ;
#18547=CARTESIAN_POINT ( 'NONE',  ( -24.33894786102607455, 16.69464852328507831, -227.6320542475859554 ) ) ;
#18548=CARTESIAN_POINT ( 'NONE',  ( 18.84307465506600465, 4.899879697440840509, -218.2189947030338715 ) ) ;
#18549=CARTESIAN_POINT ( 'NONE',  ( -5.218961787268129093, -16.18493974670746027, -219.8229902141834771 ) ) ;
#18551=CARTESIAN_POINT ( 'NONE',  ( 14.22574309452842733, 4.476723532073429546, -225.5862451792618231 ) ) ;
#18553=CARTESIAN_POINT ( 'NONE',  ( 21.83031488338151149, -1.542591969257156803, -231.3901500139511427 ) ) ;
#18555=CARTESIAN_POINT ( 'NONE',  ( -16.21268175593173311, -5.852138355245464219, -231.1837890105803410 ) ) ;
#18558=CARTESIAN_POINT ( 'NONE',  ( 5.365126951644291431, 19.60085171667039816, -218.9155869426879519 ) ) ;
#18559=CARTESIAN_POINT ( 'NONE',  ( 9.097608097968041818, -8.678217757318975600, -221.4288273931462641 ) ) ;
#18560=CARTESIAN_POINT ( 'NONE',  ( 21.53087031351596892, -21.03550532031109555, -227.1077645633325233 ) ) ;
#18562=CARTESIAN_POINT ( 'NONE',  ( -12.67219131930435694, 19.52425521811199971, -218.0046184995277372 ) ) ;
#18563=CARTESIAN_POINT ( 'NONE',  ( -18.46822229429615447, 3.027586163204024405, -230.1002726880134333 ) ) ;
#18564=CARTESIAN_POINT ( 'NONE',  ( 18.14488609917747652, 6.993670804558928644, -231.4804853770579882 ) ) ;
#18565=CARTESIAN_POINT ( 'NONE',  ( -13.27091111731893847, -21.09541201825366841, -219.8810390191036106 ) ) ;
#18567=CARTESIAN_POINT ( 'NONE',  ( -14.63872435137796302, 9.306825831109410530, -216.0000338566471214 ) ) ;
#18568=ORIENTED_EDGE ( 'NONE', *, *, #70, .F. ) ;
#18569=CARTESIAN_POINT ( 'NONE',  ( 11.41911493375616260, 8.796695304819765582, -229.7440655656592412 ) ) ;
#18570=CARTESIAN_POINT ( 'NONE',  ( 10.59565547865383728, -13.75865772189005476, -221.5384683668846435 ) ) ;
#18571=CARTESIAN_POINT ( 'NONE',  ( 4.301648988406530094, 13.23079486486395240, -223.2766268961034655 ) ) ;
#18572=CARTESIAN_POINT ( 'NONE',  ( -11.46843428684449151, 6.508406145394057596, -225.7212143570321814 ) ) ;
#18575=CARTESIAN_POINT ( 'NONE',  ( 10.93653298376230687, 10.42959444671468106, -232.5920418140667039 ) ) ;
#18576=CARTESIAN_POINT ( 'NONE',  ( -24.05551141223569545, 2.266836731622281498, -230.7594878221277384 ) ) ;
#18577=CARTESIAN_POINT ( 'NONE',  ( -12.74846050492543625, 19.93509882904884734, -216.0172840992881049 ) ) ;
#18579=CARTESIAN_POINT ( 'NONE',  ( 6.136979247480394584, 21.37054498543370684, -230.9985475420231467 ) ) ;
#18583=CARTESIAN_POINT ( 'NONE',  ( -16.81617677814535128, 0.6259372974186930838, -233.5115673467681745 ) ) ;
#18584=CARTESIAN_POINT ( 'NONE',  ( -14.02540557227298024, -18.71004003062420651, -218.0769645724313932 ) ) ;
#18586=CARTESIAN_POINT ( 'NONE',  ( -11.85645341316062051, 18.51497629668490674, -217.8828067666886454 ) ) ;
#18587=CARTESIAN_POINT ( 'NONE',  ( 2.179383121900682951, -16.00498718933496889, -221.0566978482307832 ) ) ;
#18588=CARTESIAN_POINT ( 'NONE',  ( 22.22999428328319382, 14.15012104770485557, -232.1858878619060249 ) ) ;
#18589=CARTESIAN_POINT ( 'NONE',  ( -4.784012432433236484, 23.31984772163034947, -232.0554186943449508 ) ) ;
#18590=CARTESIAN_POINT ( 'NONE',  ( -21.64120863631820413, 17.87363223393748868, -233.1390268986752119 ) ) ;
#18592=CARTESIAN_POINT ( 'NONE',  ( -23.72332483825893235, -1.495203899552344007, -219.0564715008207770 ) ) ;
#18593=CARTESIAN_POINT ( 'NONE',  ( 13.61707622192329481, 14.84143455326118932, -217.6958999636067063 ) ) ;
#18594=CARTESIAN_POINT ( 'NONE',  ( -15.12838653695630420, 3.161599240781852949, -225.7834014684609656 ) ) ;
#18595=CARTESIAN_POINT ( 'NONE',  ( -27.56397725925346975, 4.259055856374357241, -222.4951663284069241 ) ) ;
#18597=CARTESIAN_POINT ( 'NONE',  ( -30.62445638522240188, 0.2907099072661952222, -224.9999970559163387 ) ) ;
#18598=CARTESIAN_POINT ( 'NONE',  ( 6.566035546683759883, 15.06745272174450712, -218.8330720708048034 ) ) ;
#18599=CARTESIAN_POINT ( 'NONE',  ( -14.67397018911906770, 9.031553917454052893, -228.4349422195089119 ) ) ;
#18600=CARTESIAN_POINT ( 'NONE',  ( 2.469769522101480597, 18.85781121334172639, -215.5372409425634430 ) ) ;
#18601=CARTESIAN_POINT ( 'NONE',  ( 19.87150736056128864, 8.436445599727830924, -233.0166429845654932 ) ) ;
#18604=CARTESIAN_POINT ( 'NONE',  ( -10.60443131906876246, -11.12562719024938396, -217.6076818590567257 ) ) ;
#18606=CARTESIAN_POINT ( 'NONE',  ( -15.95714424191699266, -19.90201571590360885, -231.7641511196865451 ) ) ;
#18607=CARTESIAN_POINT ( 'NONE',  ( -30.66857674073067130, 4.440060741118782239, -229.9901150862898476 ) ) ;
#18608=CARTESIAN_POINT ( 'NONE',  ( 5.569356713096689226, -12.06902110579006226, -223.1407905962607003 ) ) ;
#18609=CARTESIAN_POINT ( 'NONE',  ( 15.24707275637840453, -5.950922448839978784, -232.7034617680506869 ) ) ;
#18610=CARTESIAN_POINT ( 'NONE',  ( -22.51170993270524789, -14.32174306031543054, -231.7292175355062795 ) ) ;
#18611=CARTESIAN_POINT ( 'NONE',  ( 13.60311248493089131, 7.003372205918751092, -219.1738832909067867 ) ) ;
#18613=CARTESIAN_POINT ( 'NONE',  ( -14.83806045519817829, 13.18806197935771074, -233.4179411789645542 ) ) ;
#18614=CARTESIAN_POINT ( 'NONE',  ( 24.49559427486850893, 14.86117239466233642, -230.3058416388274736 ) ) ;
#18615=CARTESIAN_POINT ( 'NONE',  ( 12.53674998645855787, 17.96979015029927851, -232.8843215672231679 ) ) ;
#18616=CARTESIAN_POINT ( 'NONE',  ( 12.83388873239664996, 22.07510045760132655, -230.4740059944613222 ) ) ;
#18617=CARTESIAN_POINT ( 'NONE',  ( 23.13778136609039038, -14.60301800679963335, -216.4810713267295341 ) ) ;
#18618=CARTESIAN_POINT ( 'NONE',  ( -4.021035526861677312, 25.02763064454595110, -216.6167103172201678 ) ) ;
#18619=CARTESIAN_POINT ( 'NONE',  ( -15.15110768032078070, 3.517015312212880218, -219.5479300368539270 ) ) ;
#18622=CARTESIAN_POINT ( 'NONE',  ( 3.737366178615106893, -15.16223317163647621, -230.3303395318446292 ) ) ;
#18623=CARTESIAN_POINT ( 'NONE',  ( -12.33203608746942237, 8.428128317385924717, -222.9277009507565026 ) ) ;
#18624=CARTESIAN_POINT ( 'NONE',  ( 7.772443558932104146, 25.24620711463332157, -231.7813173736589931 ) ) ;
#18625=CARTESIAN_POINT ( 'NONE',  ( -12.44777057840899559, -8.577008958641105352, -229.4809580173677830 ) ) ;
#18626=CARTESIAN_POINT ( 'NONE',  ( 20.10109416526603709, 2.018147939476731434, -216.1034161917718848 ) ) ;
#18627=CARTESIAN_POINT ( 'NONE',  ( 9.533850545951205291, 16.09136358716069637, -215.9093469876620475 ) ) ;
#18629=CARTESIAN_POINT ( 'NONE',  ( 5.141746912158045468, 22.01688500372448232, -216.6678693612369386 ) ) ;
#18630=CARTESIAN_POINT ( 'NONE',  ( 14.72885890443278889, -12.34426796497947620, -219.7005447341389868 ) ) ;
#18631=CARTESIAN_POINT ( 'NONE',  ( 17.56598174185312899, -13.96259959359126768, -216.8519506175684626 ) ) ;
#18633=CARTESIAN_POINT ( 'NONE',  ( 7.769483725421269860, 20.68783433326350263, -233.2348178266662728 ) ) ;
#18634=CARTESIAN_POINT ( 'NONE',  ( -28.63642022368215478, -8.327690832987633129, -230.6787490302224057 ) ) ;
#18635=CARTESIAN_POINT ( 'NONE',  ( -6.722478243781921492, -14.20656108661463612, -231.4169491518476889 ) ) ;
#18636=CARTESIAN_POINT ( 'NONE',  ( 14.65870393774896030, -26.09170264574407838, -221.2973805112574723 ) ) ;
#18637=CARTESIAN_POINT ( 'NONE',  ( -10.76972226383489506, 9.682563335906554158, -229.2555443445334333 ) ) ;
#18638=CARTESIAN_POINT ( 'NONE',  ( 10.32480721127626033, 15.84468581819879773, -230.0799086455579072 ) ) ;
#18639=CARTESIAN_POINT ( 'NONE',  ( -16.63766460830045091, 5.158675778507696208, -232.1659425527909093 ) ) ;
#18640=CARTESIAN_POINT ( 'NONE',  ( -19.01002492504315811, 19.85266905124972681, -219.0021410556803687 ) ) ;
#18641=CARTESIAN_POINT ( 'NONE',  ( -14.27379873579015879, -4.865929470441826332, -223.9216412988620561 ) ) ;
#18643=CARTESIAN_POINT ( 'NONE',  ( -7.375127652145912371, 13.01042140126078195, -223.9959097520547004 ) ) ;
#18644=CARTESIAN_POINT ( 'NONE',  ( 11.64932556965463561, 7.668732705389711413, -229.0406978839571366 ) ) ;
#18645=CARTESIAN_POINT ( 'NONE',  ( 8.463901354249619757, 8.457277735286822917, -222.5555366599873821 ) ) ;
#18648=CARTESIAN_POINT ( 'NONE',  ( 28.96372477351199137, -10.18960100487436904, -225.5971803650229504 ) ) ;
#18651=CARTESIAN_POINT ( 'NONE',  ( -26.74045434827795020, 12.41518252455047744, -220.4617428697642652 ) ) ;
#18652=CARTESIAN_POINT ( 'NONE',  ( -11.54310632260721903, -10.65784888458977697, -232.4489430773787149 ) ) ;
#18654=CARTESIAN_POINT ( 'NONE',  ( 18.29617186523616468, 23.20920553663278341, -223.4372550713720216 ) ) ;
#18656=CARTESIAN_POINT ( 'NONE',  ( 25.69672030403964769, -15.30292110028031338, -224.0206579222720791 ) ) ;
#18658=CARTESIAN_POINT ( 'NONE',  ( -25.61997837663875188, 10.01664178086244483, -231.6711741719404074 ) ) ;
#18659=CARTESIAN_POINT ( 'NONE',  ( -8.005900519654911562, 11.01772743098285545, -228.7074549843708269 ) ) ;
#18660=CARTESIAN_POINT ( 'NONE',  ( 18.78616100366561881, 3.045752412654093355, -231.5393376370170699 ) ) ;
#18661=CARTESIAN_POINT ( 'NONE',  ( -2.389036117848273300, -16.12222041688038132, -229.2542492100865559 ) ) ;
#18665=CARTESIAN_POINT ( 'NONE',  ( 12.71657619101469194, -13.18628128886902040, -219.4305778833985414 ) ) ;
#18666=CARTESIAN_POINT ( 'NONE',  ( 12.85638490943064660, -2.799177453791098280, -223.9042890815753424 ) ) ;
#18668=CARTESIAN_POINT ( 'NONE',  ( 8.162622027327667951, 13.88735946031204094, -224.7165241036068153 ) ) ;
#18669=CARTESIAN_POINT ( 'NONE',  ( 16.03771109128167538, -13.01076189404929195, -214.9179096003404084 ) ) ;
#18670=CARTESIAN_POINT ( 'NONE',  ( 15.65513449100897780, -26.00057195821942457, -227.4103383097017570 ) ) ;
#18672=CARTESIAN_POINT ( 'NONE',  ( -10.16319438574952372, 11.71174522937666040, -227.8434026503654479 ) ) ;
#18673=CARTESIAN_POINT ( 'NONE',  ( 17.66525298603349370, 4.919957226727790456, -233.3736646485340032 ) ) ;
#18674=CARTESIAN_POINT ( 'NONE',  ( 13.17424634425744046, 10.51488364724239588, -221.4616598107521099 ) ) ;
#18676=CARTESIAN_POINT ( 'NONE',  ( -3.542274070161974375, -15.57207032904040389, -222.0010230139451437 ) ) ;
#18678=CARTESIAN_POINT ( 'NONE',  ( -16.99821283087967672, -0.5135051709387361552, -216.2173766440975555 ) ) ;
#18679=CARTESIAN_POINT ( 'NONE',  ( 12.58577552758108986, 11.40439409249366420, -217.4478085440898951 ) ) ;
#18680=CARTESIAN_POINT ( 'NONE',  ( 9.923626285694149729, -13.24753681723166210, -222.8613851586638361 ) ) ;
#18681=CARTESIAN_POINT ( 'NONE',  ( 1.773982976645536835, 19.12448993322812285, -233.2315972735944172 ) ) ;
#18682=CARTESIAN_POINT ( 'NONE',  ( -17.79285498209129202, 9.187865686019035749, -216.3798185811636756 ) ) ;
#18683=CARTESIAN_POINT ( 'NONE',  ( 10.02118533929671074, 10.65166262057242008, -217.7534731326719566 ) ) ;
#18684=CARTESIAN_POINT ( 'NONE',  ( -21.01482965301294925, 6.368220028842532798, -231.7530032521518990 ) ) ;
#18685=CARTESIAN_POINT ( 'NONE',  ( -1.881996891245037995, 28.05344686410985489, -218.6379207300106202 ) ) ;
#18686=DIRECTION ( 'NONE',  ( -0.9940043559354229119, 0.1093404791529896669, -4.060016141862974029E-14 ) ) ;
#18687=CARTESIAN_POINT ( 'NONE',  ( 6.166782020495575445, -26.61202787628535660, -217.6604608484729795 ) ) ;
#18688=CARTESIAN_POINT ( 'NONE',  ( 15.13105790938820228, -1.902449014147146178, -222.1588331224812407 ) ) ;
#18691=CARTESIAN_POINT ( 'NONE',  ( -17.22166590524039265, 4.587137274468266135, -215.4863060638890033 ) ) ;
#18692=CARTESIAN_POINT ( 'NONE',  ( -10.96310611394154755, -12.59072721579616605, -220.6792497830813318 ) ) ;
#18695=CARTESIAN_POINT ( 'NONE',  ( 5.719431426348611680, -15.09047950350996281, -220.7788505835459318 ) ) ;
#18696=CARTESIAN_POINT ( 'NONE',  ( 11.35656094503625901, 14.01405796444069018, -230.6944611846958537 ) ) ;
#18697=CARTESIAN_POINT ( 'NONE',  ( -11.48592899399814726, 13.65854631785387774, -230.8311022452805616 ) ) ;
#18698=CARTESIAN_POINT ( 'NONE',  ( -21.50655177804914686, 20.61731362457859973, -218.7935603611527426 ) ) ;
#18700=CARTESIAN_POINT ( 'NONE',  ( 31.90367160121947876, -0.9372977198352894224, -223.6547426844143445 ) ) ;
#18702=CARTESIAN_POINT ( 'NONE',  ( 9.586902571418640662, 24.43292817174309661, -231.9968623198229807 ) ) ;
#18703=CARTESIAN_POINT ( 'NONE',  ( -26.70018640714903668, 3.110792036746048428, -228.8761207540193823 ) ) ;
#18704=CARTESIAN_POINT ( 'NONE',  ( -21.89065952084834166, -0.9940043559354216907, -218.9999999999999716 ) ) ;
#18706=CARTESIAN_POINT ( 'NONE',  ( 11.63337745479824292, 8.229076005436313679, -220.5472098800687206 ) ) ;
#18707=CARTESIAN_POINT ( 'NONE',  ( -17.55809605150417951, 6.636094600389130349, -229.8856864643722986 ) ) ;
#18708=CARTESIAN_POINT ( 'NONE',  ( 6.812728368504421539, 14.35307019806973194, -216.7766581591129977 ) ) ;
#18709=CARTESIAN_POINT ( 'NONE',  ( 24.60354977307301283, 7.993510024274534942, -218.5358880819990759 ) ) ;
#18710=CARTESIAN_POINT ( 'NONE',  ( -3.294080042861979862, -13.96442541267666826, -227.2909938985368683 ) ) ;
#18711=ORIENTED_EDGE ( 'NONE', *, *, #7214, .T. ) ;
#18712=CARTESIAN_POINT ( 'NONE',  ( -10.95598939193837928, -18.74794674280272488, -217.4432683290776538 ) ) ;
#18713=CARTESIAN_POINT ( 'NONE',  ( -14.63872435137796302, 9.306825831109410530, -216.0000338566471214 ) ) ;
#18714=CARTESIAN_POINT ( 'NONE',  ( 5.451525948382545117, -12.45300865616632713, -227.8545162512558306 ) ) ;
#18715=CARTESIAN_POINT ( 'NONE',  ( -7.825349071214003693, 24.14595706726266755, -216.5959661901539732 ) ) ;
#18716=CARTESIAN_POINT ( 'NONE',  ( 9.867031390707305505, -6.965612358230354850, -226.9368589251366188 ) ) ;
#18717=CARTESIAN_POINT ( 'NONE',  ( -18.75993824683981970, -9.028840681436806292, -217.1556094966459227 ) ) ;
#18718=CARTESIAN_POINT ( 'NONE',  ( 26.72610819325501907, 14.97064052581051108, -224.6384473985499426 ) ) ;
#18720=CARTESIAN_POINT ( 'NONE',  ( -21.72273972318264867, 21.08396222359856864, -224.0477214759881690 ) ) ;
#18721=CARTESIAN_POINT ( 'NONE',  ( 11.75069299018312208, 6.043853022588032253, -224.2604610870103841 ) ) ;
#18722=CARTESIAN_POINT ( 'NONE',  ( 12.58590500897257947, 11.38573988265384607, -230.4867078522624695 ) ) ;
#18723=CARTESIAN_POINT ( 'NONE',  ( 8.179023008129211902, 20.84698146175953681, -218.6376653143925921 ) ) ;
#18724=CARTESIAN_POINT ( 'NONE',  ( -3.600307272616782406, -16.89541809348436630, -217.5924753110707570 ) ) ;
#18725=CARTESIAN_POINT ( 'NONE',  ( -4.651113456395510326, 27.58151660986499110, -218.3072938287727141 ) ) ;
#18726=CARTESIAN_POINT ( 'NONE',  ( 13.54927135793711557, 0.6749664302445949060, -222.0769159577524192 ) ) ;
#18727=CARTESIAN_POINT ( 'NONE',  ( 4.072690587420734865, -13.44063513242216246, -222.4530508649998239 ) ) ;
#18728=CARTESIAN_POINT ( 'NONE',  ( -16.07193224038526580, 12.24477688577882439, -232.1409653212175499 ) ) ;
#18729=CARTESIAN_POINT ( 'NONE',  ( 0.1556102272723409452, 19.71550568250159685, -232.1993058477363547 ) ) ;
#18730=CARTESIAN_POINT ( 'NONE',  ( -18.64257584594551531, -16.66392856591270899, -217.1407738418131999 ) ) ;
#18731=CARTESIAN_POINT ( 'NONE',  ( 17.66525298603349370, 4.919957226727790456, -233.3736646485340032 ) ) ;
#18732=CARTESIAN_POINT ( 'NONE',  ( 19.20222574149634909, 21.83532798770326266, -218.6913543321078919 ) ) ;
#18734=CARTESIAN_POINT ( 'NONE',  ( -3.501680520304516264, 14.31538576447642264, -219.8967178229432307 ) ) ;
#18735=CARTESIAN_POINT ( 'NONE',  ( 14.50342097185254353, -4.720444175079822280, -222.5922120714632513 ) ) ;
#18736=CARTESIAN_POINT ( 'NONE',  ( 19.75516891782859474, -3.344025276999063934, -216.3638920815759263 ) ) ;
#18738=CARTESIAN_POINT ( 'NONE',  ( -3.843007962268670585, 27.94983497691806917, -231.4302614368887703 ) ) ;
#18739=CARTESIAN_POINT ( 'NONE',  ( -24.74482344071061135, -7.641957171360318490, -233.9284114646162891 ) ) ;
#18740=CARTESIAN_POINT ( 'NONE',  ( -7.349743644505656093, -15.31718010764164539, -232.4470764718129772 ) ) ;
#18741=CARTESIAN_POINT ( 'NONE',  ( 16.07085865561684201, -17.65509622858733252, -216.6880805489183501 ) ) ;
#18742=CARTESIAN_POINT ( 'NONE',  ( -9.115411286166651195, 13.66191091052436235, -230.3338332872444312 ) ) ;
#18743=CARTESIAN_POINT ( 'NONE',  ( 16.48099188159542194, 16.04875567542346815, -230.8408106201084706 ) ) ;
#18744=CARTESIAN_POINT ( 'NONE',  ( -25.80904414196669450, 12.19501778665756220, -219.1732313092283846 ) ) ;
#18745=CARTESIAN_POINT ( 'NONE',  ( -25.00745438246740804, 14.90779342625281778, -219.2410538611701156 ) ) ;
#18746=CARTESIAN_POINT ( 'NONE',  ( -12.38412712796990434, -11.70129718676926878, -221.8135637406489025 ) ) ;
#18747=CARTESIAN_POINT ( 'NONE',  ( -7.464187997994982560, 14.20693289415472016, -228.8865298551900764 ) ) ;
#18748=CARTESIAN_POINT ( 'NONE',  ( 13.20340559785743828, 9.575208899273587093, -218.1210831379648312 ) ) ;
#18749=CARTESIAN_POINT ( 'NONE',  ( 6.550054208186137039, 12.38618022562281595, -231.5087189857719068 ) ) ;
#18750=CARTESIAN_POINT ( 'NONE',  ( 20.28526114930425450, -5.837089636085359245, -233.7994602772149051 ) ) ;
#18754=CARTESIAN_POINT ( 'NONE',  ( -3.843007962268670585, 27.94983497691806917, -231.4302614368887703 ) ) ;
#18755=CARTESIAN_POINT ( 'NONE',  ( -23.71722460534674681, -17.39027245378339259, -231.9193655574418074 ) ) ;
#18758=CARTESIAN_POINT ( 'NONE',  ( 14.54149994592679107, 8.070685273005897997, -229.7292930672863349 ) ) ;
#18759=CARTESIAN_POINT ( 'NONE',  ( 21.53087031351596892, -21.03550532031109555, -227.1077645633325233 ) ) ;
#18760=CARTESIAN_POINT ( 'NONE',  ( -12.78558550453068854, 7.693178343823584342, -230.0800953344970878 ) ) ;
#18762=CARTESIAN_POINT ( 'NONE',  ( 18.55287065739596031, 7.869864349944380777, -232.8430408253643691 ) ) ;
#18763=CARTESIAN_POINT ( 'NONE',  ( -5.429593058350183910, -25.95961553913046416, -230.5291520159703111 ) ) ;
#18769=CARTESIAN_POINT ( 'NONE',  ( 11.44298997664856721, -19.26084286805135193, -217.6324489131326914 ) ) ;
#18772=CARTESIAN_POINT ( 'NONE',  ( 12.84032013659066251, 19.10303921738740485, -230.8110334357214128 ) ) ;
#18774=CARTESIAN_POINT ( 'NONE',  ( 11.16964468591631920, 25.71443501674299981, -224.7497461878887464 ) ) ;
#18775=ADVANCED_FACE ( 'NONE', ( #11709 ), #6872, .F. ) ;
#18776=CARTESIAN_POINT ( 'NONE',  ( 12.00030915192824565, -12.23229153226815313, -233.8665814532129730 ) ) ;
#18777=CARTESIAN_POINT ( 'NONE',  ( 13.96958060839473958, -9.488587112651741151, -218.7731372952745232 ) ) ;
#18779=CARTESIAN_POINT ( 'NONE',  ( -8.407534899841293097, 16.91942258446019665, -231.3029992963236339 ) ) ;
#18780=CARTESIAN_POINT ( 'NONE',  ( -14.20363567091065349, 7.857660128015216294, -223.4151327167956822 ) ) ;
#18781=CARTESIAN_POINT ( 'NONE',  ( 17.24423567610276109, 8.542587572837451404, -218.6562240232607621 ) ) ;
#18783=CARTESIAN_POINT ( 'NONE',  ( -2.076897692258683925, -29.27639190819841275, -225.1343076284445601 ) ) ;
#18786=CARTESIAN_POINT ( 'NONE',  ( 16.77055746703809191, 7.081497542956901370, -232.0295235404293521 ) ) ;
#18787=CARTESIAN_POINT ( 'NONE',  ( 17.47473467751515486, -18.15791173363047051, -230.0427332633545632 ) ) ;
#18788=CARTESIAN_POINT ( 'NONE',  ( 2.008896548638861024, 20.64812324442097591, -233.5818019448501843 ) ) ;
#18789=CARTESIAN_POINT ( 'NONE',  ( -18.08305592660031991, 4.022743421239192152, -217.2335041149100050 ) ) ;
#18792=CARTESIAN_POINT ( 'NONE',  ( 6.812728368504421539, 14.35307019806973194, -216.7766581591129977 ) ) ;
#18793=CARTESIAN_POINT ( 'NONE',  ( -24.53276002501160136, 17.12571705644413811, -226.2419685911331442 ) ) ;
#18794=CARTESIAN_POINT ( 'NONE',  ( 0.2389779871941385414, 16.64595486589868045, -218.1658233406367629 ) ) ;
#18796=CARTESIAN_POINT ( 'NONE',  ( -2.576162127940193169, -15.57202066281789321, -231.6911579627040396 ) ) ;
#18797=CARTESIAN_POINT ( 'NONE',  ( 27.36047156164216787, -8.591464759722228450, -221.3690063136810977 ) ) ;
#18799=CARTESIAN_POINT ( 'NONE',  ( -15.57331739480619248, 4.297375044201914740, -216.4079605712025511 ) ) ;
#18800=CARTESIAN_POINT ( 'NONE',  ( -20.83288780491947279, -19.75659621676223665, -225.4831129403879117 ) ) ;
#18802=CARTESIAN_POINT ( 'NONE',  ( 4.999282783285113219, -13.99249059192112021, -223.3817383379047214 ) ) ;
#18803=CARTESIAN_POINT ( 'NONE',  ( -18.88895772509644644, 1.306698388790553444, -217.6272550812279292 ) ) ;
#18804=CARTESIAN_POINT ( 'NONE',  ( 3.080453011304693511, 29.32691491905673331, -222.8956499783474499 ) ) ;
#18805=CARTESIAN_POINT ( 'NONE',  ( -8.523771322135640816, 24.09653697920728987, -233.1071395647740303 ) ) ;
#18806=ORIENTED_EDGE ( 'NONE', *, *, #7092, .T. ) ;
#18807=CARTESIAN_POINT ( 'NONE',  ( 13.85225051576513700, -1.547701942753643145, -218.6451083988944788 ) ) ;
#18808=CARTESIAN_POINT ( 'NONE',  ( 12.18657022793382794, 26.76558097653315471, -221.8882195427397335 ) ) ;
#18809=CARTESIAN_POINT ( 'NONE',  ( -15.82952867276381603, 3.677461268355039170, -227.9997968350711801 ) ) ;
#18810=CARTESIAN_POINT ( 'NONE',  ( -13.66744685701839046, 5.938820276054873837, -223.0954633396572149 ) ) ;
#18811=CARTESIAN_POINT ( 'NONE',  ( -13.53581065110708970, -26.13331550560631555, -224.9773145811678887 ) ) ;
#18813=CARTESIAN_POINT ( 'NONE',  ( 10.95881707662767290, 12.06788758096456782, -231.4359029166177208 ) ) ;
#18815=CARTESIAN_POINT ( 'NONE',  ( -23.99493126334580850, 6.052326449358573335, -219.7958990219547672 ) ) ;
#18816=CARTESIAN_POINT ( 'NONE',  ( 1.867752180833619713, 31.25122076096762669, -227.4007918511463231 ) ) ;
#18817=CARTESIAN_POINT ( 'NONE',  ( 26.53121369294028042, 10.74560293343441586, -229.2288136770759195 ) ) ;
#18818=CARTESIAN_POINT ( 'NONE',  ( -12.16163208632051784, -17.84934472108236747, -234.2417547270719638 ) ) ;
#18820=CARTESIAN_POINT ( 'NONE',  ( -11.57846532275044460, -10.37575015818511304, -229.3776965522603462 ) ) ;
#18821=CARTESIAN_POINT ( 'NONE',  ( -14.12265793148702464, 24.49085167151569919, -218.3312790639385241 ) ) ;
#18822=CARTESIAN_POINT ( 'NONE',  ( 1.729916699924999746, -18.64927252049523432, -233.5000329212076906 ) ) ;
#18823=CARTESIAN_POINT ( 'NONE',  ( 0.7245137624042983227, 13.44764381486384330, -223.4043886706536455 ) ) ;
#18824=CARTESIAN_POINT ( 'NONE',  ( 9.734612854996214537, -6.789898087979761243, -225.0934417779699004 ) ) ;
#18825=CARTESIAN_POINT ( 'NONE',  ( -15.19144047750087267, -10.24270553329939304, -232.4311702607364793 ) ) ;
#18826=CARTESIAN_POINT ( 'NONE',  ( 22.16968511661519869, 1.542591969257184337, -234.6098499860488573 ) ) ;
#18828=CARTESIAN_POINT ( 'NONE',  ( -5.125319492185865577, 20.53749879880200524, -218.7557759432853288 ) ) ;
#18829=CARTESIAN_POINT ( 'NONE',  ( 9.931717191100288389, 12.93133689537362940, -228.8926047089119038 ) ) ;
#18830=CARTESIAN_POINT ( 'NONE',  ( 13.61707622192329481, 14.84143455326118932, -217.6958999636067063 ) ) ;
#18831=CARTESIAN_POINT ( 'NONE',  ( 17.34461553379066601, 6.893916422670210764, -233.3442385185644525 ) ) ;
#18832=CARTESIAN_POINT ( 'NONE',  ( -0.1378336831626507664, -14.33879523207274964, -230.9095596798049144 ) ) ;
#18834=CARTESIAN_POINT ( 'NONE',  ( -9.969679877803788060, 12.84542071557917176, -220.4758784541224657 ) ) ;
#18835=CARTESIAN_POINT ( 'NONE',  ( 18.60971343765040942, 2.368090295052050820, -218.6871071987073094 ) ) ;
#18836=CARTESIAN_POINT ( 'NONE',  ( 10.12607331509846986, -17.07097861414113638, -217.9029769802564545 ) ) ;
#18837=CARTESIAN_POINT ( 'NONE',  ( -17.39737143130126285, 7.531548707695031375, -232.0788227848755696 ) ) ;
#18838=CARTESIAN_POINT ( 'NONE',  ( 8.674175678922351196, 20.85307874897338110, -216.6688793998777101 ) ) ;
#18840=CARTESIAN_POINT ( 'NONE',  ( -28.18501077041064562, -8.523171531337160545, -227.0531053546762337 ) ) ;
#18841=CARTESIAN_POINT ( 'NONE',  ( 25.50289296650958448, 5.998088869914441901, -233.1161630295026157 ) ) ;
#18842=CARTESIAN_POINT ( 'NONE',  ( 20.02669998934234741, 11.93441252203826508, -216.7824909737982182 ) ) ;
#18843=CARTESIAN_POINT ( 'NONE',  ( 18.29617186523616468, 23.20920553663278341, -223.4372550713720216 ) ) ;
#18844=CARTESIAN_POINT ( 'NONE',  ( 22.40610909459028122, -16.32493987272327018, -222.3848458449739951 ) ) ;
#18845=CARTESIAN_POINT ( 'NONE',  ( 13.09169075717699293, -6.869491136113572871, -220.8313809912125691 ) ) ;
#18847=CARTESIAN_POINT ( 'NONE',  ( 10.07175337281514871, 14.76776740066196325, -231.7834566702614723 ) ) ;
#18848=CARTESIAN_POINT ( 'NONE',  ( -26.65136949509196640, -16.37772123076025466, -229.1931346627563073 ) ) ;
#18849=CARTESIAN_POINT ( 'NONE',  ( -14.24095617957673632, -25.86326826095433162, -229.7068514753157160 ) ) ;
#18850=CARTESIAN_POINT ( 'NONE',  ( 12.84024077373997841, -14.50125846907313054, -216.8496453050001946 ) ) ;
#18851=CARTESIAN_POINT ( 'NONE',  ( -21.29946384424354733, 21.01772963953914442, -222.5871995662667757 ) ) ;
#18852=CARTESIAN_POINT ( 'NONE',  ( 8.647507700742417924, 16.42978512283924175, -220.3082116258600536 ) ) ;
#18853=CARTESIAN_POINT ( 'NONE',  ( -13.93333636822611155, 3.327141996558931947, -221.4468162587888287 ) ) ;
#18854=CARTESIAN_POINT ( 'NONE',  ( -6.407569900110946293, 14.82357759665407215, -221.6203916094852957 ) ) ;
#18855=CARTESIAN_POINT ( 'NONE',  ( -24.12156516248416693, -2.505154625461648799, -217.3585533157102248 ) ) ;
#18857=CARTESIAN_POINT ( 'NONE',  ( -17.14223598032838325, 23.31797360549976261, -226.5771676936548431 ) ) ;
#18858=CARTESIAN_POINT ( 'NONE',  ( 18.23116248274160256, 13.99874872632082123, -216.0593560670294835 ) ) ;
#18859=CARTESIAN_POINT ( 'NONE',  ( 25.17176037151762813, 18.95054595444721102, -221.3490360113488862 ) ) ;
#18860=CARTESIAN_POINT ( 'NONE',  ( 18.79106389458910442, -5.302521403133691358, -233.5021979784848440 ) ) ;
#18863=CARTESIAN_POINT ( 'NONE',  ( -2.208416658185406334, 29.10348627872611615, -219.8480645685746424 ) ) ;
#18864=CARTESIAN_POINT ( 'NONE',  ( -16.01199461824852932, -9.140529685459805265, -215.3147469429904106 ) ) ;
#18867=CARTESIAN_POINT ( 'NONE',  ( 24.57222455393806015, 12.08236629421828212, -229.7319216558644541 ) ) ;
#18868=CARTESIAN_POINT ( 'NONE',  ( -14.29986196492902550, 0.06805469746732484282, -227.4167624117703213 ) ) ;
#18869=CARTESIAN_POINT ( 'NONE',  ( 23.44296991241933981, -12.51566675729016964, -231.4065378011870564 ) ) ;
#18870=CARTESIAN_POINT ( 'NONE',  ( -15.48255455842386219, 10.01793346089237069, -233.1197357361336913 ) ) ;
#18872=CARTESIAN_POINT ( 'NONE',  ( -13.93333636822611155, 3.327141996558931947, -221.4468162587888287 ) ) ;
#18873=CARTESIAN_POINT ( 'NONE',  ( 1.268102448827562068, -18.18084990330622830, -231.0699201170278911 ) ) ;
#18877=CARTESIAN_POINT ( 'NONE',  ( 10.54788747927062964, -11.30141756528536412, -223.8337882627521651 ) ) ;
#18878=CARTESIAN_POINT ( 'NONE',  ( 12.81768984168529357, -2.998094226192216549, -225.2178905539254004 ) ) ;
#18881=CARTESIAN_POINT ( 'NONE',  ( 5.112468059216026539, 15.05346046978967856, -223.6558835435016590 ) ) ;
#18882=CARTESIAN_POINT ( 'NONE',  ( 0.7903203334012884884, 21.30772501796948859, -217.9064416298261619 ) ) ;
#18883=CARTESIAN_POINT ( 'NONE',  ( 9.478576170506354259, -9.424747406754709900, -230.1309108789951949 ) ) ;
#18885=CARTESIAN_POINT ( 'NONE',  ( 17.28140336138120858, -11.48510652344925020, -216.9852223368602893 ) ) ;
#18888=CARTESIAN_POINT ( 'NONE',  ( -10.70754874174748039, 23.84972878377777405, -230.7991598016655246 ) ) ;
#18889=CARTESIAN_POINT ( 'NONE',  ( -17.00819119081011266, 8.904695857470725784, -219.7915043529501133 ) ) ;
#18890=CARTESIAN_POINT ( 'NONE',  ( -16.36835685385702988, 8.002698209344293545, -233.7585018083067894 ) ) ;
#18891=CARTESIAN_POINT ( 'NONE',  ( -14.04270955969662360, -23.25437626513260980, -222.0989702864435174 ) ) ;
#18894=CARTESIAN_POINT ( 'NONE',  ( 14.21126657910812874, 6.833562750302326627, -220.2783117037562874 ) ) ;
#18895=CARTESIAN_POINT ( 'NONE',  ( 15.57652300565637482, -15.79620443381692496, -231.0117242343698081 ) ) ;
#18897=CARTESIAN_POINT ( 'NONE',  ( 7.168644370073567806, 19.32044210858112265, -233.1278450877711634 ) ) ;
#18898=CARTESIAN_POINT ( 'NONE',  ( -14.83974801774860630, 13.71714848582103485, -216.0935642439352762 ) ) ;
#18899=CARTESIAN_POINT ( 'NONE',  ( 16.22460398937575121, -0.7285105026664867589, -219.3274985887512116 ) ) ;
#18900=CARTESIAN_POINT ( 'NONE',  ( -18.39892766464214446, 25.11039525536027739, -225.3444503920457294 ) ) ;
#18901=CARTESIAN_POINT ( 'NONE',  ( -22.10934047915427314, 0.9940043559354312386, -216.9999999999999716 ) ) ;
#18902=CARTESIAN_POINT ( 'NONE',  ( 1.780803752597676537, -13.83832444325970101, -229.2250779460899537 ) ) ;
#18903=CARTESIAN_POINT ( 'NONE',  ( 19.06763123184207487, -2.048228142369658666, -218.2337357994572073 ) ) ;
#18905=CARTESIAN_POINT ( 'NONE',  ( -19.31342342724724759, -3.870051895940637365, -217.8584481481169348 ) ) ;
#18906=CARTESIAN_POINT ( 'NONE',  ( -17.58289524052909414, 0.7988212499981205417, -233.9567931471624149 ) ) ;
#18907=CARTESIAN_POINT ( 'NONE',  ( -13.44952714103469305, -17.53057434768947331, -217.9956016333683237 ) ) ;
#18908=CARTESIAN_POINT ( 'NONE',  ( 4.823266655078461085, -13.86048651889774241, -224.7145696108100026 ) ) ;
#18909=CARTESIAN_POINT ( 'NONE',  ( -28.61025869263052712, 6.891613135096296361, -222.2489362813765013 ) ) ;
#18910=CARTESIAN_POINT ( 'NONE',  ( 0.8374361358884788720, 23.73768315274483953, -232.4065959030912154 ) ) ;
#18911=CARTESIAN_POINT ( 'NONE',  ( -7.903959818038710061, 11.02445096303677552, -229.5951168968472871 ) ) ;
#18913=CARTESIAN_POINT ( 'NONE',  ( 30.30402220111207612, -9.997565949388443229, -221.8870099070453250 ) ) ;
#18916=CARTESIAN_POINT ( 'NONE',  ( 12.53674998645855787, 17.96979015029927851, -232.8843215672231679 ) ) ;
#18917=CARTESIAN_POINT ( 'NONE',  ( -14.30586181932858914, 18.69563132175512266, -215.8217153853723573 ) ) ;
#18918=CARTESIAN_POINT ( 'NONE',  ( -22.18165477997343871, 9.502253276305026475, -218.0070055737419636 ) ) ;
#18919=CARTESIAN_POINT ( 'NONE',  ( -11.24961133108761935, -10.18645864713539950, -228.7780882195199013 ) ) ;
#18922=CARTESIAN_POINT ( 'NONE',  ( 21.77183241683778547, 12.04504704525620085, -233.6005549158834640 ) ) ;
#18923=CARTESIAN_POINT ( 'NONE',  ( -16.45414350258782221, 17.57852913985137988, -231.3969631806205598 ) ) ;
#18924=CARTESIAN_POINT ( 'NONE',  ( 21.77779027533950540, 18.43917590911969029, -232.9503911151153659 ) ) ;
#18925=CARTESIAN_POINT ( 'NONE',  ( 24.81668481317358399, 17.11438712655213124, -222.1096362285750274 ) ) ;
#18926=CARTESIAN_POINT ( 'NONE',  ( -25.31373219958254595, -16.11658482301340811, -218.6250613297025609 ) ) ;
#18928=CARTESIAN_POINT ( 'NONE',  ( -8.652743106909156268, -19.89692808811530966, -232.3032230114403376 ) ) ;
#18929=CARTESIAN_POINT ( 'NONE',  ( -7.686214453470440411, 10.71593237010305444, -228.8058998235944159 ) ) ;
#18930=CARTESIAN_POINT ( 'NONE',  ( 13.36656406724190305, -19.73987914515934960, -233.3798509643240209 ) ) ;
#18931=CARTESIAN_POINT ( 'NONE',  ( -2.934221234790329369, 15.07857928364152222, -230.9558365497803720 ) ) ;
#18932=CARTESIAN_POINT ( 'NONE',  ( 10.88145840916109819, -7.482884786208209960, -219.8679920012262414 ) ) ;
#18933=CARTESIAN_POINT ( 'NONE',  ( -18.89430729770302975, -12.42271633246521212, -233.2230176520695295 ) ) ;
#18934=CARTESIAN_POINT ( 'NONE',  ( 12.15450584778660570, 2.288537795953278220, -225.7049340319972828 ) ) ;
#18936=CARTESIAN_POINT ( 'NONE',  ( -8.881241380679488984, 27.18697625135247975, -224.4474391433207927 ) ) ;
#18937=CARTESIAN_POINT ( 'NONE',  ( -14.58575946311604277, 2.190332613129932327, -228.6717927865686590 ) ) ;
#18938=CARTESIAN_POINT ( 'NONE',  ( 11.87982377808925527, 10.85265283465803421, -229.5027252913499183 ) ) ;
#18939=CARTESIAN_POINT ( 'NONE',  ( 10.97349919442152810, 9.416813005082010690, -227.3764328406868742 ) ) ;
#18940=CARTESIAN_POINT ( 'NONE',  ( 3.979505144402133876, -26.19079129315300491, -216.2323960841296469 ) ) ;
#18941=CARTESIAN_POINT ( 'NONE',  ( 12.75306435971521068, 14.56583715532477186, -214.9711136650476533 ) ) ;
#18942=CARTESIAN_POINT ( 'NONE',  ( 15.52719855059926424, 1.633696074270991172, -221.7349885876216433 ) ) ;
#18943=CARTESIAN_POINT ( 'NONE',  ( -5.856318878364832337, -22.45395696943396402, -215.0711972856051943 ) ) ;
#18944=CARTESIAN_POINT ( 'NONE',  ( -16.12870690754239078, 23.19263481078822053, -221.6099859194323471 ) ) ;
#18945=CARTESIAN_POINT ( 'NONE',  ( -4.224287562409271501, 29.03635716824519264, -224.1823526280761882 ) ) ;
#18946=CARTESIAN_POINT ( 'NONE',  ( -13.05629324012484282, -10.24599397043673221, -218.7452066004821347 ) ) ;
#18947=CARTESIAN_POINT ( 'NONE',  ( -22.19349712985372491, 11.03542788991621748, -219.7744882786627443 ) ) ;
#18948=CARTESIAN_POINT ( 'NONE',  ( 11.20580770355584299, 27.81589616365139150, -231.3138133330081132 ) ) ;
#18950=CARTESIAN_POINT ( 'NONE',  ( 16.54345861550681107, 19.37554510112122230, -218.2240151908141002 ) ) ;
#18951=CARTESIAN_POINT ( 'NONE',  ( 21.29805123434030634, -10.14609140759417905, -218.4136040999194108 ) ) ;
#18953=CARTESIAN_POINT ( 'NONE',  ( 17.93010821528303822, -10.80507700282924688, -233.3968735006674251 ) ) ;
#18955=CARTESIAN_POINT ( 'NONE',  ( 16.84848658399567611, 11.39632653812981644, -217.9589513831453473 ) ) ;
#18956=CARTESIAN_POINT ( 'NONE',  ( -24.71505016400469756, -15.67489082254766508, -232.1683526798342143 ) ) ;
#18957=CARTESIAN_POINT ( 'NONE',  ( 0.5120693878963755719, -30.63998626839889639, -227.9504769009175220 ) ) ;
#18958=CARTESIAN_POINT ( 'NONE',  ( 11.14834367153813233, -21.42845646353120870, -216.4520112529555718 ) ) ;
#18959=CARTESIAN_POINT ( 'NONE',  ( 1.820119372073704112, 23.17972341190215246, -230.7270437017659503 ) ) ;
#18961=CARTESIAN_POINT ( 'NONE',  ( 15.70179827786738969, 6.572001003133339125, -229.5476218741844434 ) ) ;
#18962=CARTESIAN_POINT ( 'NONE',  ( -27.29953305526601426, 11.21644211419729054, -229.3676346105362995 ) ) ;
#18963=CARTESIAN_POINT ( 'NONE',  ( -11.88513743913613752, 17.65694776598872195, -232.6054623148957035 ) ) ;
#18964=CARTESIAN_POINT ( 'NONE',  ( 28.96372477351199137, -10.18960100487436904, -225.5971803650229504 ) ) ;
#18965=CARTESIAN_POINT ( 'NONE',  ( 2.579827969572558111, 15.91317371615649101, -219.7652087782269916 ) ) ;
#18967=CARTESIAN_POINT ( 'NONE',  ( -21.99356461413155728, 5.827088221545293045, -219.1725956997024127 ) ) ;
#18968=CARTESIAN_POINT ( 'NONE',  ( 12.58033168766476528, 20.35631482982274676, -235.1670639654690547 ) ) ;
#18969=CARTESIAN_POINT ( 'NONE',  ( 10.44758276073090109, -14.65753298717242714, -218.5965683461722904 ) ) ;
#18971=CARTESIAN_POINT ( 'NONE',  ( -8.966714183099560032, 19.05224306381768073, -234.0879867025980445 ) ) ;
#18972=CARTESIAN_POINT ( 'NONE',  ( -10.60443131906876246, -11.12562719024938396, -217.6076818590567257 ) ) ;
#18974=CARTESIAN_POINT ( 'NONE',  ( 15.76910524310159900, 5.601482066865847820, -220.3440822020379528 ) ) ;
#18975=CARTESIAN_POINT ( 'NONE',  ( -27.82842955277035202, 11.70195273568964112, -227.9294339757464911 ) ) ;
#18976=CARTESIAN_POINT ( 'NONE',  ( 19.06212547406409641, -9.287000003594721775, -232.7453815625877667 ) ) ;
#18978=CARTESIAN_POINT ( 'NONE',  ( -15.20262116893801974, 8.038155052917188570, -217.6767387945475036 ) ) ;
#18979=CARTESIAN_POINT ( 'NONE',  ( -14.29986196492902550, 0.06805469746732484282, -227.4167624117703213 ) ) ;
#18980=CARTESIAN_POINT ( 'NONE',  ( -4.650330424930598561, -23.85841421069521928, -231.7493909980149454 ) ) ;
#18982=CARTESIAN_POINT ( 'NONE',  ( 15.53193985890930406, 1.024324097469592187, -227.8693888979224198 ) ) ;
#18983=CARTESIAN_POINT ( 'NONE',  ( -15.82069055112642353, 8.315535108674763976, -217.2800172218543935 ) ) ;
#18984=CARTESIAN_POINT ( 'NONE',  ( 17.50516624540364319, -11.67908417450482794, -218.9956384138364740 ) ) ;
#18985=CARTESIAN_POINT ( 'NONE',  ( 14.59755125472582016, -2.008934638541916229, -227.2287433509217465 ) ) ;
#18987=CARTESIAN_POINT ( 'NONE',  ( 14.40184562439531213, 6.414772937171507650, -227.4651811604036595 ) ) ;
#18988=CARTESIAN_POINT ( 'NONE',  ( -7.399925907206128528, 10.29859031525428037, -227.1614041762800298 ) ) ;
#18990=CARTESIAN_POINT ( 'NONE',  ( 16.48099188159542194, 16.04875567542346815, -230.8408106201084706 ) ) ;
#18991=CARTESIAN_POINT ( 'NONE',  ( -5.110696651857618455, -18.61886646437566384, -231.2604145522360000 ) ) ;
#18992=CARTESIAN_POINT ( 'NONE',  ( 14.51690190576628048, -4.522004643715366257, -218.3468014590714859 ) ) ;
#18993=CARTESIAN_POINT ( 'NONE',  ( -22.04240660558204823, 19.10355008918698871, -223.9524535985323723 ) ) ;
#18994=CARTESIAN_POINT ( 'NONE',  ( -17.30580402557236752, 11.30149179219993982, -230.8639894634705172 ) ) ;
#18995=CARTESIAN_POINT ( 'NONE',  ( -27.40681729237160269, 15.04232492504307572, -225.3323746796125704 ) ) ;
#18997=CARTESIAN_POINT ( 'NONE',  ( -8.182256202386261279, -21.48229377488409497, -218.8195705044138606 ) ) ;
#19000=CARTESIAN_POINT ( 'NONE',  ( 27.58248235015124550, 10.80791576765187934, -226.6933256641281389 ) ) ;
#19001=CARTESIAN_POINT ( 'NONE',  ( 14.72885890443278889, -12.34426796497947620, -219.7005447341389868 ) ) ;
#19002=CARTESIAN_POINT ( 'NONE',  ( 11.67669251569587985, 24.04736029062789981, -218.5856804285192254 ) ) ;
#19003=CARTESIAN_POINT ( 'NONE',  ( -11.33137429837660193, 27.25022425932026238, -230.1650924901870212 ) ) ;
#19006=CARTESIAN_POINT ( 'NONE',  ( 21.06229272850552547, 3.434461253538921621, -234.1452885155528918 ) ) ;
#19007=CARTESIAN_POINT ( 'NONE',  ( 10.07175337281514871, 14.76776740066196325, -231.7834566702614723 ) ) ;
#19009=CARTESIAN_POINT ( 'NONE',  ( 0.04660897052267574947, -31.13860575300111577, -224.7746869833732717 ) ) ;
#19010=CARTESIAN_POINT ( 'NONE',  ( 20.38902395782249144, -18.95772103455488633, -230.9098670703349967 ) ) ;
#19013=CARTESIAN_POINT ( 'NONE',  ( -23.68377094563794572, 13.02263794644603578, -215.9752901280847652 ) ) ;
#19014=CARTESIAN_POINT ( 'NONE',  ( -24.64494147011371084, -8.645298684267959999, -229.1812397229770113 ) ) ;
#19015=CARTESIAN_POINT ( 'NONE',  ( -20.45797657813638182, 1.164962349958370336, -217.1306074022350572 ) ) ;
#19016=CARTESIAN_POINT ( 'NONE',  ( 7.163080459435270164, 24.05253566895842354, -232.4475987112033408 ) ) ;
#19017=CARTESIAN_POINT ( 'NONE',  ( 2.914696262605396715, 19.49933023975583879, -231.6035545612375017 ) ) ;
#19019=CARTESIAN_POINT ( 'NONE',  ( -22.78589867900506150, -1.373495078166624861, -218.8339345403132370 ) ) ;
#19020=CARTESIAN_POINT ( 'NONE',  ( 5.623554730548537606, 15.65270319720736225, -231.3185741195121068 ) ) ;
#19021=CARTESIAN_POINT ( 'NONE',  ( -15.61959985466312872, 8.133362592386543355, -230.7826037412100106 ) ) ;
#19022=CARTESIAN_POINT ( 'NONE',  ( -22.14646582578067679, 6.967411055428133437, -231.6932229095398270 ) ) ;
#19023=CARTESIAN_POINT ( 'NONE',  ( -21.50522087930578152, -16.03150550247721640, -231.4768288373508369 ) ) ;
#19024=CARTESIAN_POINT ( 'NONE',  ( 15.37450427861381286, -5.898921106289613847E-14, -228.0000000000000853 ) ) ;
#19027=CARTESIAN_POINT ( 'NONE',  ( 26.28575214971901630, 3.591103948354015696, -217.0994821834097763 ) ) ;
#19028=CARTESIAN_POINT ( 'NONE',  ( -21.01242583983345469, 16.60754347445175227, -220.8286358486543293 ) ) ;
#19029=CARTESIAN_POINT ( 'NONE',  ( 8.373295497769937867, 8.203271496719947820, -226.1884629658694053 ) ) ;
#19030=CARTESIAN_POINT ( 'NONE',  ( -17.96792326766206926, -0.6237852504629022299, -217.9759415197746932 ) ) ;
#19031=CARTESIAN_POINT ( 'NONE',  ( -11.10256751292636324, -5.696117445562730808, -228.9287437256430451 ) ) ;
#19032=CARTESIAN_POINT ( 'NONE',  ( -17.04082806826102470, -4.797954729550726327, -217.3726213297937306 ) ) ;
#19034=CARTESIAN_POINT ( 'NONE',  ( -5.298027976154672025, 13.43376398981453157, -220.6333279128949982 ) ) ;
#19035=CARTESIAN_POINT ( 'NONE',  ( -6.722478243781921492, -14.20656108661463612, -231.4169491518476889 ) ) ;
#19036=CARTESIAN_POINT ( 'NONE',  ( -11.02345917017863464, 29.02019856777526741, -223.9475008740665771 ) ) ;
#19037=CARTESIAN_POINT ( 'NONE',  ( 23.13778136609039038, -14.60301800679963335, -216.4810713267295341 ) ) ;
#19038=CARTESIAN_POINT ( 'NONE',  ( 15.14614948138922657, -0.1777235777276532369, -227.9951794835837973 ) ) ;
#19040=CARTESIAN_POINT ( 'NONE',  ( 30.55431851955342282, 7.682798326916945975, -224.9061577511691610 ) ) ;
#19042=CARTESIAN_POINT ( 'NONE',  ( -9.175187729848801155, 26.50888816229029743, -227.9285554593684253 ) ) ;
#19043=CARTESIAN_POINT ( 'NONE',  ( -15.30864812529618391, 1.596444765892653717, -220.3859421844601627 ) ) ;
#19044=CARTESIAN_POINT ( 'NONE',  ( 14.80394259695730064, 1.224172658189580432, -225.4564070658925061 ) ) ;
#19045=CARTESIAN_POINT ( 'NONE',  ( 14.19979467405507556, 6.351366891014061267, -230.8614099669030679 ) ) ;
#19046=CARTESIAN_POINT ( 'NONE',  ( -2.827720241434194648, -28.87017495157254743, -218.9856045314649577 ) ) ;
#19048=CARTESIAN_POINT ( 'NONE',  ( 9.986779374595107228, 29.47523823012521049, -229.5287702428778687 ) ) ;
#19050=CARTESIAN_POINT ( 'NONE',  ( -2.809719670556939608, -23.45209095268191390, -234.3886352793013543 ) ) ;
#19051=CARTESIAN_POINT ( 'NONE',  ( -12.67219131930435694, 19.52425521811199971, -218.0046184995277372 ) ) ;
#19052=CARTESIAN_POINT ( 'NONE',  ( 17.31940731551425827, 24.90170669671083914, -222.9868986272316533 ) ) ;
#19053=CARTESIAN_POINT ( 'NONE',  ( -25.42089018817326007, -6.263968923056941307, -218.6542964065910439 ) ) ;
#19054=CARTESIAN_POINT ( 'NONE',  ( -25.36936018126600345, 11.57160208538938306, -224.9662154788713622 ) ) ;
#19055=CARTESIAN_POINT ( 'NONE',  ( -5.582510911615395699, 27.25430150734737111, -233.3200100877314469 ) ) ;
#19056=CARTESIAN_POINT ( 'NONE',  ( 22.44730228620155899, 3.608729811217749717, -232.0798239124179645 ) ) ;
#19058=CARTESIAN_POINT ( 'NONE',  ( 17.97642781552999836, -18.85565020944788373, -229.3765379620127760 ) ) ;
#19059=CARTESIAN_POINT ( 'NONE',  ( 5.719431426348611680, -15.09047950350996281, -220.7788505835459318 ) ) ;
#19061=CARTESIAN_POINT ( 'NONE',  ( -2.543684969149407227, 16.28137730373167713, -227.6987697727321915 ) ) ;
#19062=CARTESIAN_POINT ( 'NONE',  ( 10.78187269046063435, 10.73871010366167944, -221.9206544238666368 ) ) ;
#19063=CARTESIAN_POINT ( 'NONE',  ( 27.96460686140487084, -1.872811165202790340, -220.9791906660856000 ) ) ;
#19064=CARTESIAN_POINT ( 'NONE',  ( -11.28700884291539630, -21.85791790461604478, -233.5354093188319951 ) ) ;
#19065=CARTESIAN_POINT ( 'NONE',  ( 7.088126259304779353, -19.25156530781288566, -233.7785425911077937 ) ) ;
#19066=CARTESIAN_POINT ( 'NONE',  ( -6.407569900110946293, 14.82357759665407215, -221.6203916094852957 ) ) ;
#19068=CARTESIAN_POINT ( 'NONE',  ( 26.92457506054779515, 6.538608665672222209, -219.8654465082432807 ) ) ;
#19069=CARTESIAN_POINT ( 'NONE',  ( -22.17339560624464312, 16.26550580028390769, -232.0582861498566274 ) ) ;
#19070=CARTESIAN_POINT ( 'NONE',  ( -8.221702953833418093, 11.87876791566348800, -223.9138461338794741 ) ) ;
#19071=CARTESIAN_POINT ( 'NONE',  ( -1.772400894765090662, 19.49811434610897010, -217.8797837662441168 ) ) ;
#19072=CARTESIAN_POINT ( 'NONE',  ( -26.04932551096112192, 5.001193774903864409, -228.9498367494266802 ) ) ;
#19073=CARTESIAN_POINT ( 'NONE',  ( 12.48419387172699579, 6.663456953110941328, -219.2717027540951165 ) ) ;
#19074=CARTESIAN_POINT ( 'NONE',  ( 8.339826811406878093, -13.81198187275966660, -229.8741491687588621 ) ) ;
#19077=CARTESIAN_POINT ( 'NONE',  ( -5.807479211365208727, 19.77444019604324410, -216.0778658752277863 ) ) ;
#19078=CARTESIAN_POINT ( 'NONE',  ( 28.08231343014353243, -2.974470402155979354, -225.4253119135968291 ) ) ;
#19080=CARTESIAN_POINT ( 'NONE',  ( 19.72515656911863147, 14.02277373989196541, -218.0718040828188009 ) ) ;
#19081=CARTESIAN_POINT ( 'NONE',  ( -18.08305592660031991, 4.022743421239192152, -217.2335041149100050 ) ) ;
#19082=CARTESIAN_POINT ( 'NONE',  ( 14.65870393774896030, -26.09170264574407838, -221.2973805112574723 ) ) ;
#19084=CARTESIAN_POINT ( 'NONE',  ( -17.65835845419170624, 22.55329142274348442, -231.2673511165784532 ) ) ;
#19085=CARTESIAN_POINT ( 'NONE',  ( -13.11494368899652052, 3.355507568391938200, -225.9121440085824304 ) ) ;
#19086=CARTESIAN_POINT ( 'NONE',  ( -11.82217545354207644, -11.78227988727524966, -219.0934395369134506 ) ) ;
#19089=CARTESIAN_POINT ( 'NONE',  ( -22.17339560624464312, 16.26550580028390769, -232.0582861498566274 ) ) ;
#19090=CARTESIAN_POINT ( 'NONE',  ( 14.94445598564424493, -12.06760924077967090, -230.4366326412025785 ) ) ;
#19091=CARTESIAN_POINT ( 'NONE',  ( -23.14980455159086503, 0.3541108476526578785, -217.8785187302087536 ) ) ;
#19093=CARTESIAN_POINT ( 'NONE',  ( 12.91676121433235913, 9.519065828383201477, -226.8102878246443765 ) ) ;
#19094=CARTESIAN_POINT ( 'NONE',  ( -9.491065840222427497, 13.31995980477872266, -232.8537120564120073 ) ) ;
#19096=CARTESIAN_POINT ( 'NONE',  ( 24.52860916307685457, 12.75391509163817361, -221.3604763108436941 ) ) ;
#19097=CARTESIAN_POINT ( 'NONE',  ( 3.099569060413221333, -25.61866983817578713, -217.9657659276338677 ) ) ;
#19098=CARTESIAN_POINT ( 'NONE',  ( 21.26068545928058384, -3.181857413669367141, -233.8217025890263585 ) ) ;
#19100=CARTESIAN_POINT ( 'NONE',  ( -1.301562195391901877, 16.19210386685474390, -220.0867867038183192 ) ) ;
#19101=CARTESIAN_POINT ( 'NONE',  ( -19.72392517715239535, 13.50888179936880107, -230.7714862421596251 ) ) ;
#19102=CARTESIAN_POINT ( 'NONE',  ( -17.17143024911216287, 2.756036084795755681, -233.9491886983466316 ) ) ;
#19103=CARTESIAN_POINT ( 'NONE',  ( -21.38043581477633026, -15.61850963832630335, -229.1016256230698502 ) ) ;
#19106=CARTESIAN_POINT ( 'NONE',  ( 15.46952826979347151, 3.173892190046953665, -221.7237849701489552 ) ) ;
#19107=CARTESIAN_POINT ( 'NONE',  ( 1.152695246012044095, -27.06931983241920747, -220.0193874843003528 ) ) ;
#19108=CARTESIAN_POINT ( 'NONE',  ( 10.83706092800007781, 10.12544885278926543, -227.1716144446442343 ) ) ;
#19109=CARTESIAN_POINT ( 'NONE',  ( -11.42613629117093765, 28.09170287990588832, -228.7150250545069241 ) ) ;
#19111=CARTESIAN_POINT ( 'NONE',  ( 16.53896178738450828, 2.691624496798088462, -232.5974196329879078 ) ) ;
#19113=CARTESIAN_POINT ( 'NONE',  ( 5.343558017910363667, 26.29639771561252459, -218.1010331760174665 ) ) ;
#19115=CARTESIAN_POINT ( 'NONE',  ( -8.258403559667634397, -29.80786866836635696, -223.3983869762195127 ) ) ;
#19116=CARTESIAN_POINT ( 'NONE',  ( 8.649266908999912573, -10.50942778440553482, -226.4415026780416440 ) ) ;
#19119=CARTESIAN_POINT ( 'NONE',  ( -20.38637754046084183, 19.95723714148678241, -217.5201383746364172 ) ) ;
#19120=CARTESIAN_POINT ( 'NONE',  ( -17.95722789764597849, -8.907256384892455969, -219.4045086951509518 ) ) ;
#19121=CARTESIAN_POINT ( 'NONE',  ( 21.27683256847563698, 4.223177115764435108, -215.2584548172064842 ) ) ;
#19122=CARTESIAN_POINT ( 'NONE',  ( 7.213476267053916757, 16.78447451494783138, -217.5857052077849687 ) ) ;
#19123=CARTESIAN_POINT ( 'NONE',  ( 1.430961520682887400, 16.89318350835024063, -220.3256763723340157 ) ) ;
#19125=CARTESIAN_POINT ( 'NONE',  ( 11.27265965248755819, -10.15440342946296148, -217.7707216267749573 ) ) ;
#19126=CARTESIAN_POINT ( 'NONE',  ( 14.73698509926073186, 4.443590625350892331, -227.4062002049096236 ) ) ;
#19128=CARTESIAN_POINT ( 'NONE',  ( -8.413706464639300719, 10.92140547936800843, -220.6417935981040728 ) ) ;
#19129=CARTESIAN_POINT ( 'NONE',  ( -15.60078324628501356, 3.527872497691606934, -227.4630248446626695 ) ) ;
#19130=CARTESIAN_POINT ( 'NONE',  ( -5.534391910549205207, -14.54353160188980709, -228.1022699408985943 ) ) ;
#19131=CARTESIAN_POINT ( 'NONE',  ( -14.83974801774860630, 13.71714848582103485, -216.0935642439352762 ) ) ;
#19133=CARTESIAN_POINT ( 'NONE',  ( 14.99379536286055625, -2.466525803139443695, -223.2806853455627731 ) ) ;
#19134=CARTESIAN_POINT ( 'NONE',  ( 30.60340911705754863, 5.703403611927857497, -225.1938343315648297 ) ) ;
#19135=CARTESIAN_POINT ( 'NONE',  ( -22.38528940623734798, 16.50235888036280230, -227.1443357386333162 ) ) ;
#19136=CARTESIAN_POINT ( 'NONE',  ( 13.70863938672594529, 6.616599615120571265, -232.1343637516268643 ) ) ;
#19137=CARTESIAN_POINT ( 'NONE',  ( -21.89482327431018760, 1.733733432562314158, -233.1353281693111796 ) ) ;
#19139=CARTESIAN_POINT ( 'NONE',  ( -29.11561446909439965, 0.2226424683783513325, -217.8829860219008765 ) ) ;
#19141=CARTESIAN_POINT ( 'NONE',  ( -17.66047203424674450, -3.377913611064220056, -232.7782090104293786 ) ) ;
#19142=CARTESIAN_POINT ( 'NONE',  ( -22.56222084847001597, 18.89892770556097901, -231.8972396388394088 ) ) ;
#19143=CARTESIAN_POINT ( 'NONE',  ( -13.13432812001650341, -19.42279346457301514, -216.4126494286626610 ) ) ;
#19144=CARTESIAN_POINT ( 'NONE',  ( 12.53674998645855787, 17.96979015029927851, -232.8843215672231679 ) ) ;
#19146=CARTESIAN_POINT ( 'NONE',  ( 4.093437342195941575, -12.31737333437662940, -220.6844603446061512 ) ) ;
#19148=ADVANCED_FACE ( 'NONE', ( #10696 ), #7101, .F. ) ;
#19149=CARTESIAN_POINT ( 'NONE',  ( 15.14859676485869500, 2.119979922547468032, -231.9009926880791284 ) ) ;
#19151=CARTESIAN_POINT ( 'NONE',  ( -1.796846813493219619, 26.08418332695505271, -220.7262848173578504 ) ) ;
#19152=CARTESIAN_POINT ( 'NONE',  ( -27.52457542293397097, 5.447957517019466067, -230.2717933641555135 ) ) ;
#19153=CARTESIAN_POINT ( 'NONE',  ( 18.06016678184731461, 2.257982981100609354, -218.9983079406065940 ) ) ;
#19154=CARTESIAN_POINT ( 'NONE',  ( 30.55431851955342282, 7.682798326916945975, -224.9061577511691610 ) ) ;
#19155=CARTESIAN_POINT ( 'NONE',  ( 4.772350409791505932, -16.13531085440822466, -233.6884202312745344 ) ) ;
#19156=CARTESIAN_POINT ( 'NONE',  ( 17.60070748514786132, 25.68479983175475567, -229.9331108608050158 ) ) ;
#19160=CARTESIAN_POINT ( 'NONE',  ( -6.646164377397596468, -30.92684034042379437, -222.9942643485979374 ) ) ;
#19161=CARTESIAN_POINT ( 'NONE',  ( -13.51991436508781597, 16.61129329384914755, -232.1184346153593197 ) ) ;
#19163=CARTESIAN_POINT ( 'NONE',  ( 6.491278574642851851, 13.23281603069746382, -229.0355254242266767 ) ) ;
#19164=CARTESIAN_POINT ( 'NONE',  ( -29.22168435891936156, -1.352755938724206519, -225.9547066689444250 ) ) ;
#19165=CARTESIAN_POINT ( 'NONE',  ( -17.30580402557236752, 11.30149179219993982, -230.8639894634705172 ) ) ;
#19166=CARTESIAN_POINT ( 'NONE',  ( -1.302381543002304687, 18.65968181418110206, -215.1730913991678449 ) ) ;
#19167=CARTESIAN_POINT ( 'NONE',  ( 15.57986488780344736, -0.6155558446892130942, -225.2777919203616932 ) ) ;
#19169=CARTESIAN_POINT ( 'NONE',  ( 11.72806877847873253, -14.77654346318461975, -220.1368134445341695 ) ) ;
#19170=CARTESIAN_POINT ( 'NONE',  ( 18.24334571313621467, -21.83696521683136282, -220.5798317591433886 ) ) ;
#19171=CARTESIAN_POINT ( 'NONE',  ( -6.573387563318148885, 17.69612765735440973, -231.1211991061559274 ) ) ;
#19174=CARTESIAN_POINT ( 'NONE',  ( 12.58590500897257947, 11.38573988265384607, -230.4867078522624695 ) ) ;
#19175=CARTESIAN_POINT ( 'NONE',  ( -28.08095947817005822, 1.343466879924336999, -219.1986237337335695 ) ) ;
#19176=CARTESIAN_POINT ( 'NONE',  ( -23.54665576872953636, -14.78900941482413067, -230.7594827126482073 ) ) ;
#19178=CARTESIAN_POINT ( 'NONE',  ( 8.510712203779903007, -27.79691582975998898, -230.5316902582456180 ) ) ;
#19179=CARTESIAN_POINT ( 'NONE',  ( -2.543684969149407227, 16.28137730373167713, -227.6987697727321915 ) ) ;
#19181=CARTESIAN_POINT ( 'NONE',  ( 13.71585692689473213, 6.523039003617190801, -224.4540437369149402 ) ) ;
#19182=CARTESIAN_POINT ( 'NONE',  ( -17.17400284685640344, 24.63223427531467280, -220.6313524368512162 ) ) ;
#19183=CARTESIAN_POINT ( 'NONE',  ( -6.564517230509238743, 23.65597541655194647, -219.1225629381441991 ) ) ;
#19185=CARTESIAN_POINT ( 'NONE',  ( 8.674175678922351196, 20.85307874897338110, -216.6688793998777101 ) ) ;
#19186=CARTESIAN_POINT ( 'NONE',  ( -15.99768154740552717, 2.245235659047613908, -226.7015216759272107 ) ) ;
#19187=CARTESIAN_POINT ( 'NONE',  ( 24.19672885113291727, 10.99915907690374439, -233.6834417629405891 ) ) ;
#19188=CARTESIAN_POINT ( 'NONE',  ( 11.12240951639491549, -23.90857633046665853, -218.9373339142375130 ) ) ;
#19191=CARTESIAN_POINT ( 'NONE',  ( -9.517741096562200909, 20.63709896626785678, -234.1036702156204967 ) ) ;
#19192=CARTESIAN_POINT ( 'NONE',  ( -30.94549479715584539, -0.2777009447058255143, -220.3105931650466118 ) ) ;
#19193=CARTESIAN_POINT ( 'NONE',  ( 22.03647168421188596, 0.3315607655626346961, -232.0572713672587213 ) ) ;
#19194=CARTESIAN_POINT ( 'NONE',  ( 25.80927844399814930, 11.21489550116160316, -221.3538377621514996 ) ) ;
#19195=CARTESIAN_POINT ( 'NONE',  ( -24.68906941503829700, 2.445024713909649705, -232.6803430500543755 ) ) ;
#19196=CARTESIAN_POINT ( 'NONE',  ( 1.836136847161299990, -12.84546502099244591, -226.1727064218434293 ) ) ;
#19197=CARTESIAN_POINT ( 'NONE',  ( -17.39699619235753048, 15.64332637722790054, -216.0406373264262641 ) ) ;
#19199=CARTESIAN_POINT ( 'NONE',  ( -13.01696012539752445, 9.878799299062107409, -218.8446158128127195 ) ) ;
#19201=CARTESIAN_POINT ( 'NONE',  ( -18.08305592660031991, 4.022743421239192152, -217.2335041149100050 ) ) ;
#19202=CARTESIAN_POINT ( 'NONE',  ( -22.54883021006152433, -16.50439104605484530, -230.5104955902558004 ) ) ;
#19204=CARTESIAN_POINT ( 'NONE',  ( -14.00380962569832199, 8.747390586476997854, -231.7950903513155936 ) ) ;
#19205=CARTESIAN_POINT ( 'NONE',  ( 0.3839640804239903837, -16.65388496721540790, -217.3312339551772823 ) ) ;
#19208=CARTESIAN_POINT ( 'NONE',  ( 20.41968681625622040, 10.18377600976054076, -218.1989382652844256 ) ) ;
#19209=CARTESIAN_POINT ( 'NONE',  ( -4.558896566524145655, 13.01459016691503301, -228.3167740496058684 ) ) ;
#19211=CARTESIAN_POINT ( 'NONE',  ( 12.56556766396551872, 9.776144415819011613, -223.4791766911294815 ) ) ;
#19212=CARTESIAN_POINT ( 'NONE',  ( 3.878020530997904114, -17.84699472038997214, -232.6985457136631794 ) ) ;
#19214=CARTESIAN_POINT ( 'NONE',  ( -4.490213599459100813, 14.55066867058898694, -222.6488251579668827 ) ) ;
#19215=CARTESIAN_POINT ( 'NONE',  ( -15.82760502346409304, 5.624826830110399634, -227.5369622385896946 ) ) ;
#19216=CARTESIAN_POINT ( 'NONE',  ( -24.79170285622992509, 4.551775110860766915, -234.5907228154019322 ) ) ;
#19218=CARTESIAN_POINT ( 'NONE',  ( -16.83358080157556103, -19.16169236771116857, -229.6922051654298116 ) ) ;
#19222=CARTESIAN_POINT ( 'NONE',  ( 24.34047711160105720, 17.90454708687460794, -228.1939002122307159 ) ) ;
#19223=CARTESIAN_POINT ( 'NONE',  ( 7.436546160899932367, -15.25288503996851475, -221.8354696069030467 ) ) ;
#19224=CARTESIAN_POINT ( 'NONE',  ( 12.23063869552301242, 12.84118223717021934, -218.8273164334868284 ) ) ;
#19226=CARTESIAN_POINT ( 'NONE',  ( -11.02345917017863464, 29.02019856777526741, -223.9475008740665771 ) ) ;
#19227=CARTESIAN_POINT ( 'NONE',  ( 29.96674103997387206, 4.060923908484647349, -228.5323681967686298 ) ) ;
#19228=CARTESIAN_POINT ( 'NONE',  ( 7.995304978256253747, 13.28024228361502779, -220.6535174700288451 ) ) ;
#19230=CARTESIAN_POINT ( 'NONE',  ( -8.376153411442972541, -27.59911039556260448, -219.0729038785590888 ) ) ;
#19231=CARTESIAN_POINT ( 'NONE',  ( 9.104026917753444081, -10.66572815660443041, -221.9193219976906448 ) ) ;
#19234=CARTESIAN_POINT ( 'NONE',  ( -20.06846544527470400, 7.877362284741439069, -235.3910773253824402 ) ) ;
#19235=CARTESIAN_POINT ( 'NONE',  ( -20.58881354142085485, -10.73024182470851606, -219.1570184730780397 ) ) ;
#19236=CARTESIAN_POINT ( 'NONE',  ( 13.98152565379061052, 2.156981915107639036, -230.5667344709999611 ) ) ;
#19237=CARTESIAN_POINT ( 'NONE',  ( 2.630208337444488453, 16.40323635460054774, -219.2570070657488088 ) ) ;
#19238=CARTESIAN_POINT ( 'NONE',  ( -1.316322971969275502, 14.13179993441458215, -224.9782367179667233 ) ) ;
#19240=CARTESIAN_POINT ( 'NONE',  ( 14.43570356028121893, -19.75277720499002498, -215.7015347705405759 ) ) ;
#19242=CARTESIAN_POINT ( 'NONE',  ( 26.24002132888527328, 11.62331517472360964, -222.5300873157218859 ) ) ;
#19243=CARTESIAN_POINT ( 'NONE',  ( -8.995433708001568718, 13.44373928221519243, -231.9251680978426577 ) ) ;
#19245=CARTESIAN_POINT ( 'NONE',  ( -15.51814470728089645, 2.949994979016113739, -222.8331727603033130 ) ) ;
#19246=CARTESIAN_POINT ( 'NONE',  ( -14.33274213004767716, -3.240524307521291725, -229.5155949954044559 ) ) ;
#19247=CARTESIAN_POINT ( 'NONE',  ( -17.39699619235753048, 15.64332637722790054, -216.0406373264262641 ) ) ;
#19250=CARTESIAN_POINT ( 'NONE',  ( 14.68028918641733149, -3.003797161868758447, -225.1263072288626006 ) ) ;
#19252=CARTESIAN_POINT ( 'NONE',  ( -17.75632171729475317, 14.45153669854845901, -218.6240360064753929 ) ) ;
#19253=CARTESIAN_POINT ( 'NONE',  ( 17.85905871012913693, 8.463974683125162102, -234.6532732619751300 ) ) ;
#19254=CARTESIAN_POINT ( 'NONE',  ( 16.40130693394614525, -0.1574073183566240264, -221.9481963320051534 ) ) ;
#19255=CARTESIAN_POINT ( 'NONE',  ( -17.53163374842703703, -10.16025041587072764, -214.8411325589202647 ) ) ;
#19256=CARTESIAN_POINT ( 'NONE',  ( -21.27082149447729620, -6.316573346028001801, -216.2864220516500779 ) ) ;
#19257=CARTESIAN_POINT ( 'NONE',  ( -7.903959818038710061, 11.02445096303677552, -229.5951168968472871 ) ) ;
#19258=CARTESIAN_POINT ( 'NONE',  ( -14.24095617957673632, -25.86326826095433162, -229.7068514753157160 ) ) ;
#19259=CARTESIAN_POINT ( 'NONE',  ( 4.656903975822286768, 13.45000048768594780, -227.6722060245555497 ) ) ;
#19260=CARTESIAN_POINT ( 'NONE',  ( 6.571750410407496190, -24.62545695199335682, -234.5391748598602248 ) ) ;
#19263=CARTESIAN_POINT ( 'NONE',  ( 28.53243699394185384, 6.329221954355706004, -218.6437889135959267 ) ) ;
#19265=CARTESIAN_POINT ( 'NONE',  ( -2.618694198633108261, 15.69630225547860825, -226.1451761977223498 ) ) ;
#19266=CARTESIAN_POINT ( 'NONE',  ( -24.79507334250576278, 6.844873424762779379, -218.1074956078844878 ) ) ;
#19267=CARTESIAN_POINT ( 'NONE',  ( 27.40550551777678123, 5.967061366481472895, -228.7463788799179554 ) ) ;
#19268=CARTESIAN_POINT ( 'NONE',  ( 29.81944548462877975, 8.043843257819576209, -228.1755181449411793 ) ) ;
#19269=CARTESIAN_POINT ( 'NONE',  ( -15.00281653375496127, -15.21317112889928858, -231.9690514080965613 ) ) ;
#19271=CARTESIAN_POINT ( 'NONE',  ( 16.71363093372661979, 20.70203100498337179, -215.6856694095356488 ) ) ;
#19273=CARTESIAN_POINT ( 'NONE',  ( -14.25383187134801588, -24.74900029534085633, -216.9920501705437630 ) ) ;
#19274=CARTESIAN_POINT ( 'NONE',  ( -4.386767007475907754, 14.39570986262862107, -223.2690175027443615 ) ) ;
#19276=CARTESIAN_POINT ( 'NONE',  ( 10.12956299421491302, 11.38773431477224385, -230.3175791991728829 ) ) ;
#19278=CARTESIAN_POINT ( 'NONE',  ( -21.26441444091935296, 10.69428164102106926, -219.3434466924981336 ) ) ;
#19279=CARTESIAN_POINT ( 'NONE',  ( -11.59874896804548250, 27.28969409813203484, -218.8626241359735332 ) ) ;
#19280=CARTESIAN_POINT ( 'NONE',  ( 14.64440749032966593, 2.523901497798496596, -225.4572725674553340 ) ) ;
#19281=CARTESIAN_POINT ( 'NONE',  ( 7.724698117049915602, -20.76727510557136469, -231.0612438369181518 ) ) ;
#19283=CARTESIAN_POINT ( 'NONE',  ( 6.025688374458400887, -15.61258154445926749, -220.0079782759978002 ) ) ;
#19284=CARTESIAN_POINT ( 'NONE',  ( -2.015708574708954259, 26.78900769828807782, -221.5371848586876808 ) ) ;
#19287=CARTESIAN_POINT ( 'NONE',  ( 7.639528166734322667, 11.92751229241157596, -224.6077814063189635 ) ) ;
#19288=CARTESIAN_POINT ( 'NONE',  ( 25.69761320619099720, -8.403105518750903613, -219.2599777650661110 ) ) ;
#19289=CARTESIAN_POINT ( 'NONE',  ( -11.49803752765619258, -8.459563989871591971, -222.4296168992866853 ) ) ;
#19290=CARTESIAN_POINT ( 'NONE',  ( 0.5120693878963755719, -30.63998626839889639, -227.9504769009175220 ) ) ;
#19291=CARTESIAN_POINT ( 'NONE',  ( 0.9458336400950161371, 17.49535648476021876, -228.8359568483051589 ) ) ;
#19293=CARTESIAN_POINT ( 'NONE',  ( 25.53003411612920459, 7.940385729200389875, -230.5495695598654322 ) ) ;
#19294=CARTESIAN_POINT ( 'NONE',  ( -7.395406416482832590, 12.93623984139929739, -219.2606224730616873 ) ) ;
#19295=CARTESIAN_POINT ( 'NONE',  ( -2.618694198633108261, 15.69630225547860825, -226.1451761977223498 ) ) ;
#19297=CARTESIAN_POINT ( 'NONE',  ( 0.3632086708616291126, 21.06287758167331958, -232.5112839711303820 ) ) ;
#19298=CARTESIAN_POINT ( 'NONE',  ( -15.65611835717891687, 5.486779671999271635, -227.0554626315911264 ) ) ;
#19299=CARTESIAN_POINT ( 'NONE',  ( 29.33969601628096768, 11.98971187598327504, -225.2039690377576733 ) ) ;
#19300=CARTESIAN_POINT ( 'NONE',  ( 7.092430827040528740, -27.48041265710635628, -228.4891580147104548 ) ) ;
#19303=CARTESIAN_POINT ( 'NONE',  ( 12.10245006109274080, 26.02147364279441888, -220.6079829738538649 ) ) ;
#19304=CARTESIAN_POINT ( 'NONE',  ( 25.61231557635624156, -8.129803667132245337, -228.3450084804328242 ) ) ;
#19306=CARTESIAN_POINT ( 'NONE',  ( 19.20300624114736721, 0.6066039755357417462, -231.5046416827383950 ) ) ;
#19307=CARTESIAN_POINT ( 'NONE',  ( 8.709470447750865318, -17.43408031369701661, -216.5121658579468829 ) ) ;
#19309=CARTESIAN_POINT ( 'NONE',  ( -6.201839134465864767, 11.37481922992157379, -223.7040893475979146 ) ) ;
#19310=CARTESIAN_POINT ( 'NONE',  ( -19.61183938075907918, 22.25855138946451106, -229.5731876748794207 ) ) ;
#19312=CARTESIAN_POINT ( 'NONE',  ( 21.83031488337932657, -1.542591969257240070, -231.3901500139511427 ) ) ;
#19313=CARTESIAN_POINT ( 'NONE',  ( -11.18311023676720062, -15.30649302686804347, -231.8766562234714002 ) ) ;
#19316=CARTESIAN_POINT ( 'NONE',  ( -29.88125065636863198, 4.504452993877526623, -226.2048141718237275 ) ) ;
#19317=CARTESIAN_POINT ( 'NONE',  ( 0.4504461526642338232, -19.62726417856956473, -215.9916429883993487 ) ) ;
#19319=CARTESIAN_POINT ( 'NONE',  ( 19.67070349224072956, 16.44307963282299312, -220.0378483479504439 ) ) ;
#19321=CARTESIAN_POINT ( 'NONE',  ( -16.13584396029534318, 23.78382729893626646, -231.6788043429177435 ) ) ;
#19323=CARTESIAN_POINT ( 'NONE',  ( 11.73428189025226942, 12.46434742632455084, -228.1539301014595083 ) ) ;
#19324=CARTESIAN_POINT ( 'NONE',  ( -3.821460206879919941, -14.75247343660110921, -225.5705290259156470 ) ) ;
#19327=CARTESIAN_POINT ( 'NONE',  ( -4.142636420702924482, 14.17169704882741321, -225.1666440184957310 ) ) ;
#19328=CARTESIAN_POINT ( 'NONE',  ( -9.679547659771646551, 14.60131434979866505, -230.4338124916943968 ) ) ;
#19329=CARTESIAN_POINT ( 'NONE',  ( 19.10353041285295816, 2.510539514498965730, -232.1135168369976896 ) ) ;
#19330=CARTESIAN_POINT ( 'NONE',  ( -16.75383819933101748, -8.593015344009392820, -230.3978590765929084 ) ) ;
#19333=CARTESIAN_POINT ( 'NONE',  ( 20.88210880980788531, 0.9259446317980322139, -218.6312544800709929 ) ) ;
#19334=CARTESIAN_POINT ( 'NONE',  ( 3.191506000329551007, -19.56356538597602679, -231.2193641236077326 ) ) ;
#19335=CARTESIAN_POINT ( 'NONE',  ( 12.58590500897257947, 11.38573988265384607, -230.4867078522624695 ) ) ;
#19336=CARTESIAN_POINT ( 'NONE',  ( -3.514547081416551588, 30.38636916157537016, -227.3529586180979436 ) ) ;
#19337=CARTESIAN_POINT ( 'NONE',  ( 13.12946830070648652, 6.370976456471619365, -231.5124810213676483 ) ) ;
#19338=CARTESIAN_POINT ( 'NONE',  ( 12.18657022793382794, 26.76558097653315471, -221.8882195427397335 ) ) ;
#19339=CARTESIAN_POINT ( 'NONE',  ( 13.45723858497841618, 1.555143580403207659, -222.4309038978887543 ) ) ;
#19340=CARTESIAN_POINT ( 'NONE',  ( -21.52428768452188734, -21.65989873160339840, -225.4304055049964006 ) ) ;
#19341=CARTESIAN_POINT ( 'NONE',  ( 19.06435866915521515, -20.24829071055443563, -218.8318535520223804 ) ) ;
#19344=CARTESIAN_POINT ( 'NONE',  ( -29.15345109632842124, 14.07532767497844262, -225.0972140442887621 ) ) ;
#19345=CARTESIAN_POINT ( 'NONE',  ( -25.33517302999029042, -8.734563104097837538, -228.3677567689655916 ) ) ;
#19346=CARTESIAN_POINT ( 'NONE',  ( -22.38347148959098121, 12.58966534755613687, -218.4978713241202399 ) ) ;
#19347=CARTESIAN_POINT ( 'NONE',  ( 14.63115627273841923, 9.024791562541032874, -232.5054678133655841 ) ) ;
#19348=CARTESIAN_POINT ( 'NONE',  ( 5.104697752190542559, 17.18208638613223016, -220.3923334988619445 ) ) ;
#19350=CARTESIAN_POINT ( 'NONE',  ( 13.82710435306955432, -11.68840971183345800, -215.7775723145259974 ) ) ;
#19352=CARTESIAN_POINT ( 'NONE',  ( 20.34032485158648029, 2.741617426884598530, -217.9827731991294968 ) ) ;
#19353=CARTESIAN_POINT ( 'NONE',  ( -13.66744685701839046, 5.938820276054873837, -223.0954633396572149 ) ) ;
#19354=CARTESIAN_POINT ( 'NONE',  ( -10.01410430826631170, 16.10970239316000630, -233.6135099156378203 ) ) ;
#19355=CARTESIAN_POINT ( 'NONE',  ( -13.83093441725390704, -7.146379636134302160, -230.0501880019394605 ) ) ;
#19356=CARTESIAN_POINT ( 'NONE',  ( -15.20262116893801974, 8.038155052917188570, -217.6767387945475036 ) ) ;
#19359=CARTESIAN_POINT ( 'NONE',  ( 14.62702828724412285, -1.994068170757606673, -224.0552340365271959 ) ) ;
#19360=CARTESIAN_POINT ( 'NONE',  ( -11.82020046940938407, 10.16362659047642758, -224.3364193436540575 ) ) ;
#19361=CARTESIAN_POINT ( 'NONE',  ( 13.34963947135311102, 7.416462695144936390, -217.9359469527792044 ) ) ;
#19362=CARTESIAN_POINT ( 'NONE',  ( 16.56146809408446430, -0.9616313295950813522, -228.5729530379900609 ) ) ;
#19363=CARTESIAN_POINT ( 'NONE',  ( 10.55627441269396094, 10.31758739525044888, -223.1990319438957613 ) ) ;
#19364=CARTESIAN_POINT ( 'NONE',  ( -14.80115690555879659, -8.758261077448048937, -218.2925738755452016 ) ) ;
#19365=CARTESIAN_POINT ( 'NONE',  ( -2.125813515909480866, 15.68152656492264363, -220.3943115937447317 ) ) ;
#19366=CARTESIAN_POINT ( 'NONE',  ( -1.633632075387274840, -15.48245080501611071, -218.5193615163172751 ) ) ;
#19367=CARTESIAN_POINT ( 'NONE',  ( 7.168644370073567806, 19.32044210858112265, -233.1278450877711634 ) ) ;
#19368=CARTESIAN_POINT ( 'NONE',  ( 5.917072789534883803, -21.18442853552521754, -235.1867574136372525 ) ) ;
#19370=CARTESIAN_POINT ( 'NONE',  ( -10.02095171162140019, 11.02119725306997111, -224.1251327387667516 ) ) ;
#19371=SURFACE_SIDE_STYLE ('',( #10940 ) ) ;
#19372=CARTESIAN_POINT ( 'NONE',  ( 27.12528000378512871, -1.050705938820645224, -232.4139529590446784 ) ) ;
#19373=CARTESIAN_POINT ( 'NONE',  ( 3.614175329767659761, 21.98488100320606264, -219.0898850257099753 ) ) ;
#19374=CARTESIAN_POINT ( 'NONE',  ( 14.55590852435181226, 2.816890518231522034, -218.5131513550309990 ) ) ;
#19375=CARTESIAN_POINT ( 'NONE',  ( 17.34727976380017722, 4.822939981779328811, -230.8836217450937909 ) ) ;
#19376=CARTESIAN_POINT ( 'NONE',  ( -7.753256282497156704, -15.05334625439219565, -219.2728364670455221 ) ) ;
#19377=CARTESIAN_POINT ( 'NONE',  ( 10.66732316618037402, 25.78610527446713263, -216.5597036843431624 ) ) ;
#19379=CARTESIAN_POINT ( 'NONE',  ( -6.154316005079235374, -31.08134634390615503, -226.4265589226172892 ) ) ;
#19380=CARTESIAN_POINT ( 'NONE',  ( -11.03778527004271659, 26.96286968643956428, -225.4057095641571209 ) ) ;
#19381=CARTESIAN_POINT ( 'NONE',  ( 22.73582563804385970, 20.20868311426415431, -227.8513184012435886 ) ) ;
#19382=CARTESIAN_POINT ( 'NONE',  ( -24.82235633397527508, 10.76243500821901300, -227.9886044494091948 ) ) ;
#19383=CARTESIAN_POINT ( 'NONE',  ( 4.569118550756183339, 31.72363458735121000, -222.3920438419263519 ) ) ;
#19384=CARTESIAN_POINT ( 'NONE',  ( 27.84414217501293010, 2.965433895642837214, -221.8999927093654492 ) ) ;
#19385=CARTESIAN_POINT ( 'NONE',  ( 6.592356972974974916, -14.93599889844929862, -226.9608163220883625 ) ) ;
#19387=CARTESIAN_POINT ( 'NONE',  ( 9.835929410207317147, -16.71508016877321268, -232.2716196330763694 ) ) ;
#19388=CARTESIAN_POINT ( 'NONE',  ( -10.30040261405712698, 19.75576125044891285, -218.0811964201226658 ) ) ;
#19390=CARTESIAN_POINT ( 'NONE',  ( 15.87442104186276381, 8.674488492264579520, -230.9702037640878416 ) ) ;
#19391=CARTESIAN_POINT ( 'NONE',  ( 14.56914850832129815, -2.041740472307377985, -224.7121590863160350 ) ) ;
#19392=CARTESIAN_POINT ( 'NONE',  ( -22.23616899077527975, -11.51447210886970751, -217.5950109096934568 ) ) ;
#19393=CARTESIAN_POINT ( 'NONE',  ( -7.460068573003235670, -29.58770008691625364, -228.1902472473001637 ) ) ;
#19394=CARTESIAN_POINT ( 'NONE',  ( -3.010752168931037698, 15.84372070116375575, -223.4060793985500482 ) ) ;
#19396=CARTESIAN_POINT ( 'NONE',  ( 24.52860916307685457, 12.75391509163817361, -221.3604763108436941 ) ) ;
#19397=CARTESIAN_POINT ( 'NONE',  ( -4.104500432947460808, 15.73223271406093460, -218.0734292856946297 ) ) ;
#19398=CARTESIAN_POINT ( 'NONE',  ( 3.689800395305025127, 23.07294874520714956, -219.2515233573129478 ) ) ;
#19400=CARTESIAN_POINT ( 'NONE',  ( 10.31623634631035991, 26.83927646318382898, -220.2315638557092541 ) ) ;
#19401=CARTESIAN_POINT ( 'NONE',  ( 13.30790133003807441, 0.6370684082013071681, -222.3495379725305270 ) ) ;
#19402=CARTESIAN_POINT ( 'NONE',  ( 15.65443801613259467, 7.488839228060037989, -233.6469817377710569 ) ) ;
#19403=CARTESIAN_POINT ( 'NONE',  ( 10.05661706967825353, -14.25456047934742365, -218.9909083857680230 ) ) ;
#19404=CARTESIAN_POINT ( 'NONE',  ( 21.96352831578809273, -0.3315607655629317918, -233.9427286327412503 ) ) ;
#19406=CARTESIAN_POINT ( 'NONE',  ( 10.66614775643814994, 26.29080367171353672, -230.0818785118670178 ) ) ;
#19407=CARTESIAN_POINT ( 'NONE',  ( 21.58416078958130413, -8.344710983103166058, -219.2549068428508861 ) ) ;
#19409=CARTESIAN_POINT ( 'NONE',  ( 13.47054497134856277, -24.75371201277411615, -218.7687119198782000 ) ) ;
#19410=CARTESIAN_POINT ( 'NONE',  ( -10.84997096467605182, 25.01800101807719301, -232.4518260228253155 ) ) ;
#19411=CARTESIAN_POINT ( 'NONE',  ( -11.94727018630768178, 9.025563988971828877, -220.6148682757971358 ) ) ;
#19413=CARTESIAN_POINT ( 'NONE',  ( -17.17400284685640344, 24.63223427531467280, -220.6313524368512162 ) ) ;
#19414=CARTESIAN_POINT ( 'NONE',  ( -21.50522087930578152, -16.03150550247721640, -231.4768288373508369 ) ) ;
#19417=CARTESIAN_POINT ( 'NONE',  ( -15.15110768032078070, 3.517015312212880218, -219.5479300368539270 ) ) ;
#19418=CARTESIAN_POINT ( 'NONE',  ( 9.471595414968767557, -23.22249338881061931, -232.1368331642201497 ) ) ;
#19419=CARTESIAN_POINT ( 'NONE',  ( -18.47334320050258327, 24.79293862780133040, -226.9986786077537317 ) ) ;
#19420=CARTESIAN_POINT ( 'NONE',  ( 25.18311526135610734, 13.65721788432563955, -224.7326014392022273 ) ) ;
#19421=CARTESIAN_POINT ( 'NONE',  ( -7.903959818038710061, 11.02445096303677552, -229.5951168968472871 ) ) ;
#19423=CARTESIAN_POINT ( 'NONE',  ( 14.12692363916921146, 20.59586666873830296, -230.0804552526094540 ) ) ;
#19424=CARTESIAN_POINT ( 'NONE',  ( -3.088421015035204498, -25.33386621341791667, -218.8172537214380498 ) ) ;
#19428=CARTESIAN_POINT ( 'NONE',  ( -10.84440549681320221, 27.00404139634608214, -224.0969657459751261 ) ) ;
#19429=CARTESIAN_POINT ( 'NONE',  ( -9.852301241816233457, 15.10013604187968461, -230.8124578431014697 ) ) ;
#19430=CARTESIAN_POINT ( 'NONE',  ( -15.72555926117677139, 17.60926865496976745, -217.2114552733360142 ) ) ;
#19431=CARTESIAN_POINT ( 'NONE',  ( -12.22799442060091657, -11.48557521842085372, -222.2662941369099201 ) ) ;
#19434=CARTESIAN_POINT ( 'NONE',  ( -13.65925618638770800, 3.289586759644148817, -222.1579143493116533 ) ) ;
#19435=CARTESIAN_POINT ( 'NONE',  ( 3.849154133940814848, -15.34907234289524958, -223.0340372416051196 ) ) ;
#19436=CARTESIAN_POINT ( 'NONE',  ( 25.33562512631297281, 12.25422971834577268, -228.6777356031426791 ) ) ;
#19437=CARTESIAN_POINT ( 'NONE',  ( -4.620781219515533778, 16.99182040716223696, -217.1278208835672672 ) ) ;
#19439=CARTESIAN_POINT ( 'NONE',  ( -18.91027996815576628, 5.295101183552822555, -231.2253513302548527 ) ) ;
#19440=CARTESIAN_POINT ( 'NONE',  ( 7.393167209263542539, 10.77319710117329699, -221.1179833906701049 ) ) ;
#19441=CARTESIAN_POINT ( 'NONE',  ( 14.32085100525799248, 9.220655089380342062, -219.9006227404039464 ) ) ;
#19442=CARTESIAN_POINT ( 'NONE',  ( 13.54927135793711557, 0.6749664302445949060, -222.0769159577524192 ) ) ;
#19443=CARTESIAN_POINT ( 'NONE',  ( -21.63546480557098306, -21.44004028177477750, -223.8762611443524122 ) ) ;
#19444=CARTESIAN_POINT ( 'NONE',  ( 8.257114973007913861, -25.39836461225790742, -232.6217252414676295 ) ) ;
#19447=CARTESIAN_POINT ( 'NONE',  ( -24.77996431573922820, 10.49354383977773786, -234.1655613096203581 ) ) ;
#19448=CARTESIAN_POINT ( 'NONE',  ( -15.58915292315067802, -7.289217648355976742, -221.6802381019405175 ) ) ;
#19449=CARTESIAN_POINT ( 'NONE',  ( -26.19327040236159831, 13.44417515682194875, -223.7810975255189874 ) ) ;
#19450=CARTESIAN_POINT ( 'NONE',  ( 11.98894270675143225, 20.38243841428667835, -233.2283128908360084 ) ) ;
#19451=CARTESIAN_POINT ( 'NONE',  ( -1.973645837583506424, 28.78841935349527503, -228.5341874691134763 ) ) ;
#19453=CARTESIAN_POINT ( 'NONE',  ( 22.53017539111736411, -13.33152463597901516, -234.4848520764015518 ) ) ;
#19454=CARTESIAN_POINT ( 'NONE',  ( 16.64225601860865211, 1.926018578292457928, -220.2177910260893725 ) ) ;
#19456=CARTESIAN_POINT ( 'NONE',  ( 0.1645309800062008665, 15.56029994314186382, -233.1129172884685943 ) ) ;
#19457=CARTESIAN_POINT ( 'NONE',  ( -19.98042543492610079, 23.51949599776966693, -226.6701036947414138 ) ) ;
#19458=CARTESIAN_POINT ( 'NONE',  ( -26.76734473129764069, -3.453818734898710829, -232.3222361544058003 ) ) ;
#19459=CARTESIAN_POINT ( 'NONE',  ( -28.13472254077564116, 12.33996625515159629, -224.9141344439281909 ) ) ;
#19461=CARTESIAN_POINT ( 'NONE',  ( 26.54225689383817866, -6.924125931238839016, -230.1506921200174247 ) ) ;
#19463=CARTESIAN_POINT ( 'NONE',  ( 3.001892273201697048, 27.20292285420111966, -216.7800154582108689 ) ) ;
#19464=CARTESIAN_POINT ( 'NONE',  ( 13.40064012097826307, 2.532414129335418096, -221.5952957478750989 ) ) ;
#19465=CARTESIAN_POINT ( 'NONE',  ( 15.57986488780344736, -0.6155558446892130942, -225.2777919203616932 ) ) ;
#19466=CARTESIAN_POINT ( 'NONE',  ( 12.99034161053428349, 11.71468708507361889, -230.9043293568357740 ) ) ;
#19468=CARTESIAN_POINT ( 'NONE',  ( -15.33992272861872763, -7.600289318192222865, -231.6130094852651951 ) ) ;
#19470=CARTESIAN_POINT ( 'NONE',  ( 5.563568780623874943, 21.86458082533069103, -218.6474243140849012 ) ) ;
#19471=CARTESIAN_POINT ( 'NONE',  ( -5.178973235464019886, -24.35492185057628944, -233.6431870320687381 ) ) ;
#19472=CARTESIAN_POINT ( 'NONE',  ( 4.389496648589924277, 14.47660514356954131, -220.6151178996808540 ) ) ;
#19473=CARTESIAN_POINT ( 'NONE',  ( 6.679393088666140343, -31.31585170264869689, -224.7195491891107793 ) ) ;
#19474=CARTESIAN_POINT ( 'NONE',  ( 14.30360180157784988, -0.2838691938953850080, -227.9870050950131315 ) ) ;
#19475=CARTESIAN_POINT ( 'NONE',  ( -16.74094048923576494, 16.03040267675914521, -217.9177456399057178 ) ) ;
#19477=CARTESIAN_POINT ( 'NONE',  ( 30.87761267810551757, -2.376991648450896388, -225.4116222034606949 ) ) ;
#19478=CARTESIAN_POINT ( 'NONE',  ( 14.61121792518381390, 23.81825453963186590, -227.9329146581663110 ) ) ;
#19479=CARTESIAN_POINT ( 'NONE',  ( -14.94640692938030746, 5.382918922058764544, -220.5478552936960455 ) ) ;
#19481=CARTESIAN_POINT ( 'NONE',  ( 16.00819137755116373, 4.595691552992191120, -229.5669508871464757 ) ) ;
#19482=CARTESIAN_POINT ( 'NONE',  ( -18.40842514464981861, -18.33793064768350334, -230.6214457472987931 ) ) ;
#19484=CARTESIAN_POINT ( 'NONE',  ( 28.41961022423218353, 10.76616830294286409, -220.2698681100053193 ) ) ;
#19485=CARTESIAN_POINT ( 'NONE',  ( -21.59049550158629316, -10.60627468734379164, -215.2236992441505663 ) ) ;
#19486=CARTESIAN_POINT ( 'NONE',  ( -0.3197916200495275474, 16.38897215927557482, -229.9606066735827028 ) ) ;
#19489=CARTESIAN_POINT ( 'NONE',  ( 23.44028133050380802, 19.87677100428751231, -223.1503774981096342 ) ) ;
#19491=CARTESIAN_POINT ( 'NONE',  ( -12.14452111807825041, 26.21581784948545035, -221.1455569020914140 ) ) ;
#19492=CARTESIAN_POINT ( 'NONE',  ( -5.191169535941942748, 31.49570301054888688, -227.4714364261087098 ) ) ;
#19493=CARTESIAN_POINT ( 'NONE',  ( 15.90795275983908574, 2.546196724714939297, -229.0855319561646297 ) ) ;
#19494=CARTESIAN_POINT ( 'NONE',  ( 10.22171596740309418, -15.66339630224980972, -229.7686180632486810 ) ) ;
#19495=CARTESIAN_POINT ( 'NONE',  ( 18.70674991763376482, -20.04093309878971496, -230.8534322170362714 ) ) ;
#19497=CARTESIAN_POINT ( 'NONE',  ( 16.64225601860865211, 1.926018578292457928, -220.2177910260893725 ) ) ;
#19498=CARTESIAN_POINT ( 'NONE',  ( -29.78324924674133456, -0.2661018803894699136, -229.0431670511964057 ) ) ;
#19499=CARTESIAN_POINT ( 'NONE',  ( -16.21268175593173311, -5.852138355245464219, -231.1837890105803410 ) ) ;
#19500=CARTESIAN_POINT ( 'NONE',  ( 2.178520447619924472, -13.56847537563065487, -221.4085897031499428 ) ) ;
#19501=CARTESIAN_POINT ( 'NONE',  ( 6.225744896574323839, 14.38227537199079720, -224.8391693295998266 ) ) ;
#19503=CARTESIAN_POINT ( 'NONE',  ( -11.84805200323110164, 5.835720598137266180, -228.2740675967047537 ) ) ;
#19504=CARTESIAN_POINT ( 'NONE',  ( -6.101488798441174310, 11.33371047077072369, -225.3616985956418546 ) ) ;
#19505=CARTESIAN_POINT ( 'NONE',  ( -3.139695637132168038, 25.12735071829084177, -230.1469660918596389 ) ) ;
#19506=CARTESIAN_POINT ( 'NONE',  ( 16.37256825621668099, -5.086412116083368851, -216.7246661941694867 ) ) ;
#19510=CARTESIAN_POINT ( 'NONE',  ( 15.26539804565921621, 9.309431686815628382, -232.9129599938668207 ) ) ;
#19511=CARTESIAN_POINT ( 'NONE',  ( -22.53796032816233463, 16.84148256071415872, -226.0516062466300582 ) ) ;
#19512=CARTESIAN_POINT ( 'NONE',  ( 22.49659352743751128, 7.060662713609715979, -215.7089950799439180 ) ) ;
#19513=CARTESIAN_POINT ( 'NONE',  ( 1.250172743705837641, -19.35180105203422940, -231.6553945523530729 ) ) ;
#19517=CARTESIAN_POINT ( 'NONE',  ( 11.33210854356620523, 22.81476816607802149, -217.8536224460118262 ) ) ;
#19518=CARTESIAN_POINT ( 'NONE',  ( -31.13345889576667247, -1.683779982087686422, -229.5421043233184264 ) ) ;
#19519=CARTESIAN_POINT ( 'NONE',  ( -15.83178333309709629, 2.467763724635483324, -230.4064772870105458 ) ) ;
#19520=CARTESIAN_POINT ( 'NONE',  ( 13.99926435381047618, -21.11851526759364006, -232.9234173943665951 ) ) ;
#19522=CARTESIAN_POINT ( 'NONE',  ( 0.6364901924797052857, 13.89978473517355617, -221.8840706290426397 ) ) ;
#19524=CARTESIAN_POINT ( 'NONE',  ( -18.41237742040652847, 14.06446039901721790, -216.7469276929859632 ) ) ;
#19525=CARTESIAN_POINT ( 'NONE',  ( -11.67631226053870996, 6.737291529340801333, -227.3110382950315227 ) ) ;
#19526=CARTESIAN_POINT ( 'NONE',  ( -8.011291865669539547, -12.94570094964118923, -221.6322823144945744 ) ) ;
#19530=CARTESIAN_POINT ( 'NONE',  ( -9.517741096562200909, 20.63709896626785678, -234.1036702156204967 ) ) ;
#19531=CARTESIAN_POINT ( 'NONE',  ( 9.903783394593444811, -26.64562852513063973, -229.6560785209296682 ) ) ;
#19532=CARTESIAN_POINT ( 'NONE',  ( -10.30050448363967419, 10.07750059423401190, -220.1837019037183723 ) ) ;
#19533=CARTESIAN_POINT ( 'NONE',  ( -14.37318171526297483, 2.227741863946853140, -231.7654527934561202 ) ) ;
#19534=CARTESIAN_POINT ( 'NONE',  ( 2.914696262605396715, 19.49933023975583879, -231.6035545612375017 ) ) ;
#19536=CARTESIAN_POINT ( 'NONE',  ( 16.55609572527610851, 2.729108819536508967, -230.5704679660131831 ) ) ;
#19537=CARTESIAN_POINT ( 'NONE',  ( -16.95213199947759009, -16.93177456301608785, -219.4409135693619817 ) ) ;
#19539=CARTESIAN_POINT ( 'NONE',  ( 8.674175678922351196, 20.85307874897338110, -216.6688793998777101 ) ) ;
#19540=CARTESIAN_POINT ( 'NONE',  ( -11.10144104376680652, 18.49675466419975578, -232.2931259015917647 ) ) ;
#19541=CARTESIAN_POINT ( 'NONE',  ( -8.137644474477026435, 12.10064032984799098, -226.6735072060122036 ) ) ;
#19542=CARTESIAN_POINT ( 'NONE',  ( -12.38412712796990434, -11.70129718676926878, -221.8135637406489025 ) ) ;
#19545=CARTESIAN_POINT ( 'NONE',  ( -16.74550766701807447, 3.787526820511904813, -217.9802846976114381 ) ) ;
#19546=CARTESIAN_POINT ( 'NONE',  ( 3.940243381406264511, -15.52098910442465041, -222.4744391328516144 ) ) ;
#19547=CARTESIAN_POINT ( 'NONE',  ( 21.35706335192880445, 15.67286272432725092, -219.2578158352350783 ) ) ;
#19549=CARTESIAN_POINT ( 'NONE',  ( 2.539761864897490007, 23.64215977235053501, -233.4645566207487661 ) ) ;
#19551=CARTESIAN_POINT ( 'NONE',  ( -16.75232826114664775, 4.232868982398014346, -229.4158550594996200 ) ) ;
#19553=CARTESIAN_POINT ( 'NONE',  ( 12.03015173539790617, 23.46358517874481109, -216.0611092640310744 ) ) ;
#19554=CARTESIAN_POINT ( 'NONE',  ( 13.61707622192329481, 14.84143455326118932, -217.6958999636067063 ) ) ;
#19556=CARTESIAN_POINT ( 'NONE',  ( -11.88525712185471050, -8.925198460467992589, -221.0951487055306472 ) ) ;
#19557=CARTESIAN_POINT ( 'NONE',  ( 9.584731462935641488, -12.36622837314704348, -230.4796538097028531 ) ) ;
#19561=CARTESIAN_POINT ( 'NONE',  ( -10.14083745617744547, 19.87482866967577877, -216.0596634563153486 ) ) ;
#19562=CARTESIAN_POINT ( 'NONE',  ( 11.78812147976811175, -1.482036947660514636, -224.5790252820172270 ) ) ;
#19563=CARTESIAN_POINT ( 'NONE',  ( 27.36047156164216787, -8.591464759722228450, -221.3690063136810977 ) ) ;
#19564=CARTESIAN_POINT ( 'NONE',  ( 12.98364502352995942, 13.67380631913144029, -233.1535077318696096 ) ) ;
#19565=CARTESIAN_POINT ( 'NONE',  ( 8.132753622789847370, 14.44084924206385701, -222.7013822740049704 ) ) ;
#19567=CARTESIAN_POINT ( 'NONE',  ( 6.114261689233397412, -11.26162238963769369, -223.0577857700231164 ) ) ;
#19568=CARTESIAN_POINT ( 'NONE',  ( 15.76910524310159900, 5.601482066865847820, -220.3440822020379528 ) ) ;
#19569=CARTESIAN_POINT ( 'NONE',  ( -4.619644865335168049, 14.75104250038670450, -232.3086264397671812 ) ) ;
#19570=CARTESIAN_POINT ( 'NONE',  ( -10.30034651166687887, 25.05454868506992838, -216.5587736482213188 ) ) ;
#19571=CARTESIAN_POINT ( 'NONE',  ( -30.71739798481564421, -2.702902032605977389, -225.9472362185736642 ) ) ;
#19572=CARTESIAN_POINT ( 'NONE',  ( -15.82069055112642353, 8.315535108674763976, -217.2800172218543935 ) ) ;
#19574=CARTESIAN_POINT ( 'NONE',  ( 26.16486877413895584, -0.2437668799822691745, -230.8325409000573814 ) ) ;
#19576=CARTESIAN_POINT ( 'NONE',  ( -0.7286890422672397394, 21.00519367000705273, -234.2149015821977969 ) ) ;
#19577=CARTESIAN_POINT ( 'NONE',  ( 29.21307215008108216, 4.139194015751272104, -229.9658791484231699 ) ) ;
#19578=CARTESIAN_POINT ( 'NONE',  ( -18.70100282803782576, 16.58357028540773115, -216.4425743468854080 ) ) ;
#19579=CARTESIAN_POINT ( 'NONE',  ( 7.639528166734322667, 11.92751229241157596, -224.6077814063189635 ) ) ;
#19582=CARTESIAN_POINT ( 'NONE',  ( -2.117958212721558375, 27.20243410318316535, -230.7086725634165418 ) ) ;
#19583=CARTESIAN_POINT ( 'NONE',  ( -13.52935284690462758, -5.503084506376929141, -222.3607690796775671 ) ) ;
#19584=CARTESIAN_POINT ( 'NONE',  ( 9.333020543840051531, 16.91085096921651143, -217.7308990335875762 ) ) ;
#19585=CARTESIAN_POINT ( 'NONE',  ( 10.30964016151751750, -15.48526446506176413, -234.8200832677974859 ) ) ;
#19587=CARTESIAN_POINT ( 'NONE',  ( -21.19360951076126653, 12.15251088906093457, -217.9482185194656552 ) ) ;
#19589=CARTESIAN_POINT ( 'NONE',  ( 28.81324478616323148, -9.895151559995404966, -227.1624192579662918 ) ) ;
#19591=CARTESIAN_POINT ( 'NONE',  ( 8.632180352507942800, 16.83956698119041917, -230.4752415867875186 ) ) ;
#19592=CARTESIAN_POINT ( 'NONE',  ( -13.70798801564395752, 13.71024986321384809, -218.3360451569033955 ) ) ;
#19593=CARTESIAN_POINT ( 'NONE',  ( -11.79271689233719478, 3.876813423829604144, -228.6816298097564299 ) ) ;
#19594=CARTESIAN_POINT ( 'NONE',  ( -20.64589292112740537, -18.79971917946562598, -222.0410088502282520 ) ) ;
#19597=CARTESIAN_POINT ( 'NONE',  ( 22.66015888791822519, 10.43487984001084534, -234.3950629709119937 ) ) ;
#19599=CARTESIAN_POINT ( 'NONE',  ( -17.20514689733751368, -7.568958929800959190, -215.6459182133127115 ) ) ;
#19600=CARTESIAN_POINT ( 'NONE',  ( -4.583529401292260275, 28.77615850237956607, -226.7744741901706504 ) ) ;
#19601=CARTESIAN_POINT ( 'NONE',  ( 15.51129552754472307, 0.2180314803830030457, -231.3815478022924879 ) ) ;
#19602=CARTESIAN_POINT ( 'NONE',  ( -10.24168223636446662, 16.14271751156598356, -231.4847994864913971 ) ) ;
#19603=CARTESIAN_POINT ( 'NONE',  ( 12.90536070039565963, 17.66816134723717724, -234.8562535614228750 ) ) ;
#19605=CARTESIAN_POINT ( 'NONE',  ( -16.15126510923403202, -0.4755054218165427615, -219.3066569788202571 ) ) ;
#19606=CARTESIAN_POINT ( 'NONE',  ( -3.496415903701482808, -16.44974864882642152, -218.6042005240371111 ) ) ;
#19607=( GEOMETRIC_REPRESENTATION_CONTEXT ( 3 ) GLOBAL_UNCERTAINTY_ASSIGNED_CONTEXT ( ( #13029 ) ) GLOBAL_UNIT_ASSIGNED_CONTEXT ( ( #16011, #9262, #3844 ) ) REPRESENTATION_CONTEXT ( 'NONE', 'WORKASPACE' ) );
#19608=CARTESIAN_POINT ( 'NONE',  ( 0.2799207934783670693, -28.72270877262613453, -227.3216717588132667 ) ) ;
#19610=CARTESIAN_POINT ( 'NONE',  ( 20.23125423326388628, 7.836699765464857137, -217.8891354894872450 ) ) ;
#19611=CARTESIAN_POINT ( 'NONE',  ( 11.39114332821395692, -8.257479203742953189, -226.5648397932267528 ) ) ;
#19612=CARTESIAN_POINT ( 'NONE',  ( -21.63546480557098306, -21.44004028177477750, -223.8762611443524122 ) ) ;
#19613=CARTESIAN_POINT ( 'NONE',  ( -13.13432812001650341, -19.42279346457301514, -216.4126494286626610 ) ) ;
#19614=CARTESIAN_POINT ( 'NONE',  ( 9.489894741926459432, 25.96007012349547338, -222.3210984495278524 ) ) ;
#19616=CARTESIAN_POINT ( 'NONE',  ( -13.84508897751235246, 5.904954704487344941, -218.7722818424232401 ) ) ;
#19617=CARTESIAN_POINT ( 'NONE',  ( -9.151299407007059017, 9.196974979111923076, -223.9483834032048719 ) ) ;
#19618=CARTESIAN_POINT ( 'NONE',  ( -1.364406401035816785, 24.33111505239456918, -219.5658712396381418 ) ) ;
#19619=CARTESIAN_POINT ( 'NONE',  ( 13.95236037140391261, -4.360547358326352096, -218.9684814425422132 ) ) ;
#19621=CARTESIAN_POINT ( 'NONE',  ( 23.18902850759750933, 20.27908137164207147, -226.2847847834817117 ) ) ;
#19622=CARTESIAN_POINT ( 'NONE',  ( -21.10507617219916199, 14.90539259013048756, -229.7677326419877488 ) ) ;
#19623=CARTESIAN_POINT ( 'NONE',  ( 27.79290571682592770, 12.05347838982552666, -230.1298045326732051 ) ) ;
#19624=CARTESIAN_POINT ( 'NONE',  ( -0.8337089444836248697, -27.22572500676309559, -220.1932236949194532 ) ) ;
#19628=CARTESIAN_POINT ( 'NONE',  ( 18.29617186523616468, 23.20920553663278341, -223.4372550713720216 ) ) ;
#19629=CARTESIAN_POINT ( 'NONE',  ( 20.43533161254376296, -19.75510188685668567, -224.2614117135439074 ) ) ;
#19631=CARTESIAN_POINT ( 'NONE',  ( -14.84823930505322132, -23.35465403802561823, -218.3226235040776260 ) ) ;
#19632=CARTESIAN_POINT ( 'NONE',  ( 1.382955251742491898, 16.46353944795171032, -231.7743150979565030 ) ) ;
#19633=CARTESIAN_POINT ( 'NONE',  ( -5.340143745732740754, 22.10628181454592678, -235.0476201740528097 ) ) ;
#19635=CARTESIAN_POINT ( 'NONE',  ( -13.56774755469388616, 7.311522441667196226, -219.1912666243428021 ) ) ;
#19636=CARTESIAN_POINT ( 'NONE',  ( -24.65069530437947876, -0.7989515219415058711, -216.4419420286324112 ) ) ;
#19639=CARTESIAN_POINT ( 'NONE',  ( -9.540790481621398200, 9.981116473660406996, -228.6478862620407995 ) ) ;
#19640=CARTESIAN_POINT ( 'NONE',  ( 8.072455080350884771, -13.51419333260225741, -221.0758372092125228 ) ) ;
#19642=CARTESIAN_POINT ( 'NONE',  ( -12.90983082593748676, 14.84936372681532823, -233.8009687022269532 ) ) ;
#19643=CARTESIAN_POINT ( 'NONE',  ( 18.39384604806649648, 2.566915855367216004, -231.7421336352533103 ) ) ;
#19644=CARTESIAN_POINT ( 'NONE',  ( -8.328662059352005542, 28.53523473722178139, -221.4280032538016201 ) ) ;
#19646=CARTESIAN_POINT ( 'NONE',  ( 17.92683513449900445, 4.153309877386362814, -218.0960491240478234 ) ) ;
#19647=CARTESIAN_POINT ( 'NONE',  ( -10.06242375715308945, -19.11710762076843295, -231.0938065448402199 ) ) ;
#19649=CARTESIAN_POINT ( 'NONE',  ( 12.95792863868717149, 16.83236386576623644, -216.3406066345214356 ) ) ;
#19650=CARTESIAN_POINT ( 'NONE',  ( -10.45265333418718612, 16.71118685480038479, -231.7490466715443631 ) ) ;
#19651=CARTESIAN_POINT ( 'NONE',  ( -9.746008880186941781, 12.96562886885531896, -220.1990846131056401 ) ) ;
#19652=CARTESIAN_POINT ( 'NONE',  ( 27.54201077264015396, -3.286392687948289648, -218.1575117614944190 ) ) ;
#19655=CARTESIAN_POINT ( 'NONE',  ( -29.95012366401462955, 4.746560250930182967, -224.6954343660969471 ) ) ;
#19656=CARTESIAN_POINT ( 'NONE',  ( -4.451292041429703694, -15.86428280493796628, -231.0943874731633798 ) ) ;
#19657=CARTESIAN_POINT ( 'NONE',  ( 14.66712853512338732, 1.689060028942728442, -227.4794820723986390 ) ) ;
#19658=CARTESIAN_POINT ( 'NONE',  ( -2.735889804569492600, 12.71735652435744512, -225.1194195722198117 ) ) ;
#19660=CARTESIAN_POINT ( 'NONE',  ( 21.75737151495493649, -2.205713500382455283, -233.2756072794337285 ) ) ;
#19661=CARTESIAN_POINT ( 'NONE',  ( 15.23494377589453919, 15.24947835004434538, -215.7641128510430519 ) ) ;
#19662=CARTESIAN_POINT ( 'NONE',  ( 22.46220731426537043, 18.23201731183003460, -227.5436199598787539 ) ) ;
#19664=CARTESIAN_POINT ( 'NONE',  ( -27.99742768613627319, -7.906662303124995184, -217.4094589651611216 ) ) ;
#19665=CARTESIAN_POINT ( 'NONE',  ( -5.519971913460887336, -12.21762732219001713, -227.2962593638428359 ) ) ;
#19666=CARTESIAN_POINT ( 'NONE',  ( 14.99336262864975211, -23.54026314425397004, -231.3018640253376361 ) ) ;
#19669=CARTESIAN_POINT ( 'NONE',  ( -4.211886032913159106, 20.62037006687756602, -216.9488349035050305 ) ) ;
#19670=CARTESIAN_POINT ( 'NONE',  ( 30.80938026993025503, 0.02210899415489638725, -229.5596456628577187 ) ) ;
#19671=CARTESIAN_POINT ( 'NONE',  ( 14.02668320743028119, -5.282748560960272677, -221.9001732195871739 ) ) ;
#19672=CARTESIAN_POINT ( 'NONE',  ( -20.97727766418175932, 9.381545086430262970, -232.5968905491617420 ) ) ;
#19673=CARTESIAN_POINT ( 'NONE',  ( 21.26803326031697949, 19.54255073453192892, -230.5813148908474659 ) ) ;
#19674=CARTESIAN_POINT ( 'NONE',  ( 12.16813927252146144, 18.27141895336136912, -230.9123895730235745 ) ) ;
#19676=CARTESIAN_POINT ( 'NONE',  ( 4.354371064427007276, -19.91633591276652382, -233.4790676556106348 ) ) ;
#19677=CARTESIAN_POINT ( 'NONE',  ( 16.07305932912010960, 0.9253679043337685872, -229.0409936706996064 ) ) ;
#19679=CARTESIAN_POINT ( 'NONE',  ( -7.403072389817287657, 18.92851032520892929, -215.2068968469505137 ) ) ;
#19680=CARTESIAN_POINT ( 'NONE',  ( -7.752954785937490989, 10.21341112307795385, -225.5135920495299615 ) ) ;
#19681=CARTESIAN_POINT ( 'NONE',  ( -28.57583275380518018, -9.842401781236429059, -222.4643230566485386 ) ) ;
#19682=CARTESIAN_POINT ( 'NONE',  ( -9.716674560061926869, 27.56227806819028103, -219.4917914922789919 ) ) ;
#19683=CARTESIAN_POINT ( 'NONE',  ( -20.26851768784797869, -0.8260594303982465858, -217.1279713726092098 ) ) ;
#19684=CARTESIAN_POINT ( 'NONE',  ( 17.00614511541963836, -1.958782916976874233, -219.4638360731791806 ) ) ;
#19685=CARTESIAN_POINT ( 'NONE',  ( -3.162425552858488143, 20.40327580806445695, -216.0004724541873316 ) ) ;
#19686=CARTESIAN_POINT ( 'NONE',  ( 27.79290571682592770, 12.05347838982552666, -230.1298045326732051 ) ) ;
#19687=CARTESIAN_POINT ( 'NONE',  ( -25.61997837663875188, 10.01664178086244483, -231.6711741719404074 ) ) ;
#19688=CARTESIAN_POINT ( 'NONE',  ( 12.71450444683213021, 7.595266944807587350, -224.4213778964231665 ) ) ;
#19690=CARTESIAN_POINT ( 'NONE',  ( 0.07890756785233743464, 25.14108539708653822, -218.4152285319504756 ) ) ;
#19691=CARTESIAN_POINT ( 'NONE',  ( -25.98129645912436914, -15.13773040547512139, -224.1390156429105787 ) ) ;
#19692=CARTESIAN_POINT ( 'NONE',  ( 21.25094435758043332, 17.68230636442804027, -229.7964888993842010 ) ) ;
#19693=CARTESIAN_POINT ( 'NONE',  ( -0.8305687497496098137, -27.95880702065288759, -232.3543905114424888 ) ) ;
#19695=CARTESIAN_POINT ( 'NONE',  ( -14.24491355791863612, 5.286533920242113105, -221.7104936369346433 ) ) ;
#19696=CARTESIAN_POINT ( 'NONE',  ( 18.03651828442428595, -19.10816016050398147, -231.7458924702002037 ) ) ;
#19697=CARTESIAN_POINT ( 'NONE',  ( 8.829458998963966465, 22.90677303676718779, -219.2026791561175685 ) ) ;
#19698=CARTESIAN_POINT ( 'NONE',  ( -24.18895665211001500, 11.26087434487096139, -231.0040666710689550 ) ) ;
#19699=CARTESIAN_POINT ( 'NONE',  ( -26.12939716039095117, 11.33146045174629357, -233.1192402782019997 ) ) ;
#19701=CARTESIAN_POINT ( 'NONE',  ( -9.481788909210624894, -22.96916533494018253, -217.3969400264330716 ) ) ;
#19703=CARTESIAN_POINT ( 'NONE',  ( 13.40064012097826307, 2.532414129335418096, -221.5952957478750989 ) ) ;
#19705=CARTESIAN_POINT ( 'NONE',  ( -11.65988442122670676, -3.998659314375652141, -223.4258670541443621 ) ) ;
#19706=CARTESIAN_POINT ( 'NONE',  ( 2.579827969572558111, 15.91317371615649101, -219.7652087782269916 ) ) ;
#19707=CARTESIAN_POINT ( 'NONE',  ( 20.13946171159960841, -0.1427001808266660232, -233.7987036390019853 ) ) ;
#19708=CARTESIAN_POINT ( 'NONE',  ( -5.590964611773372894, 13.92546790642523113, -228.7941110425196882 ) ) ;
#19711=CARTESIAN_POINT ( 'NONE',  ( 12.58577552758108986, 11.40439409249366420, -217.4478085440898951 ) ) ;
#19712=CARTESIAN_POINT ( 'NONE',  ( 3.050495372378628112, -23.18092737088175781, -231.5841725462776992 ) ) ;
#19714=CARTESIAN_POINT ( 'NONE',  ( 6.755953262402430326, -28.44658494672641424, -224.7309905328439754 ) ) ;
#19716=CARTESIAN_POINT ( 'NONE',  ( 20.89184612657454920, 5.404957034965973683, -232.0952743654565609 ) ) ;
#19717=CARTESIAN_POINT ( 'NONE',  ( 14.34945462593695531, -6.128426910066905542, -229.1128190117150041 ) ) ;
#19719=CARTESIAN_POINT ( 'NONE',  ( 18.65267415280877117, -0.4843198157805662651, -217.0419311198673711 ) ) ;
#19720=CARTESIAN_POINT ( 'NONE',  ( -10.42804209284631156, -14.08702332024887305, -217.7386024361820489 ) ) ;
#19721=CARTESIAN_POINT ( 'NONE',  ( 3.635089269978064141, 27.05650967970794341, -222.4639105745756638 ) ) ;
#19723=CARTESIAN_POINT ( 'NONE',  ( -22.28357709049062407, 7.264818440526320309, -215.3877468064711707 ) ) ;
#19724=CARTESIAN_POINT ( 'NONE',  ( -0.3969026096611234511, 20.89748314411456676, -216.3289738411752978 ) ) ;
#19725=CARTESIAN_POINT ( 'NONE',  ( 3.191455400233187412, 17.67480163422566619, -220.7055581859663107 ) ) ;
#19726=CARTESIAN_POINT ( 'NONE',  ( -22.05223281125446633, 0.4748437386657422543, -217.8785187290425256 ) ) ;
#19728=CARTESIAN_POINT ( 'NONE',  ( 18.81274554574540403, 10.85963742466947224, -234.0446454529665345 ) ) ;
#19729=CARTESIAN_POINT ( 'NONE',  ( -22.36207348798144778, 17.12313795477538036, -223.8571857210765472 ) ) ;
#19730=CARTESIAN_POINT ( 'NONE',  ( -22.14646582578067679, 6.967411055428133437, -231.6932229095398270 ) ) ;
#19731=CARTESIAN_POINT ( 'NONE',  ( -5.249799428260828904, -14.16826377401270065, -226.9124264195330056 ) ) ;
#19734=CARTESIAN_POINT ( 'NONE',  ( 4.656903975822286768, 13.45000048768594780, -227.6722060245555497 ) ) ;
#19735=CARTESIAN_POINT ( 'NONE',  ( 17.22969587606878505, -8.834803756807117381, -230.2348533348707917 ) ) ;
#19736=CARTESIAN_POINT ( 'NONE',  ( 14.83290459615719215, -2.296615622475745688, -226.9301701175285757 ) ) ;
#19737=CARTESIAN_POINT ( 'NONE',  ( -7.349743644505656093, -15.31718010764164539, -232.4470764718129772 ) ) ;
#19739=CARTESIAN_POINT ( 'NONE',  ( -2.772442535524381579, 13.75675912271027457, -228.9770533867650215 ) ) ;
#19740=CARTESIAN_POINT ( 'NONE',  ( -3.687581766460184429, 30.01855770642711718, -218.8323691868875187 ) ) ;
#19742=CARTESIAN_POINT ( 'NONE',  ( -12.44873260470819787, 7.411970124596155785, -229.4214091473984070 ) ) ;
#19743=CARTESIAN_POINT ( 'NONE',  ( -25.32486352395475393, -3.505876693931964549, -233.0869506614649822 ) ) ;
#19746=CARTESIAN_POINT ( 'NONE',  ( -11.69688825528096388, 18.63404371591177622, -215.8612738028812714 ) ) ;
#19747=CARTESIAN_POINT ( 'NONE',  ( -6.773088999562194346, -28.54379939428971369, -218.3283227997898450 ) ) ;
#19748=CARTESIAN_POINT ( 'NONE',  ( 14.34945462593695531, -6.128426910066905542, -229.1128190117150041 ) ) ;
#19749=CARTESIAN_POINT ( 'NONE',  ( -9.740348021262962064, 16.12529029871877384, -216.4361617420699702 ) ) ;
#19750=CARTESIAN_POINT ( 'NONE',  ( -12.10258892854866275, 5.599955477755926836, -221.6590149575334010 ) ) ;
#19751=CARTESIAN_POINT ( 'NONE',  ( -2.117958212721558375, 27.20243410318316535, -230.7086725634165418 ) ) ;
#19753=CARTESIAN_POINT ( 'NONE',  ( 22.24262848503957812, 2.205713500382371794, -232.7243927205662430 ) ) ;
#19754=CARTESIAN_POINT ( 'NONE',  ( -18.95931133506032040, -20.40484553783743138, -225.1835090426186525 ) ) ;
#19756=CARTESIAN_POINT ( 'NONE',  ( 6.771176146757415637, 15.60014285904435027, -218.3493856697694753 ) ) ;
#19757=CARTESIAN_POINT ( 'NONE',  ( -16.45414350258782221, 17.57852913985137988, -231.3969631806205598 ) ) ;
#19758=CARTESIAN_POINT ( 'NONE',  ( -15.05930145804884290, 24.78193219970826533, -223.0510781988847953 ) ) ;
#19759=CARTESIAN_POINT ( 'NONE',  ( -24.76242154467160717, -4.839146110080178254, -231.6857664014047202 ) ) ;
#19762=CARTESIAN_POINT ( 'NONE',  ( 21.19180206786061405, -1.472355559550188264, -231.3901500139509722 ) ) ;
#19763=CARTESIAN_POINT ( 'NONE',  ( -8.861553082841476581, -17.08180233781500590, -216.2529452235939402 ) ) ;
#19764=CARTESIAN_POINT ( 'NONE',  ( 18.46552355142154411, 5.019711608606525211, -231.5099115070375433 ) ) ;
#19765=CARTESIAN_POINT ( 'NONE',  ( 5.169766346882679997, 29.28517558595074988, -221.5178724947562614 ) ) ;
#19767=CARTESIAN_POINT ( 'NONE',  ( -17.91769793922991028, 3.277678596821882007, -219.5526088240203819 ) ) ;
#19768=CARTESIAN_POINT ( 'NONE',  ( 10.46530733675539793, 8.351728317179080818, -222.7431177495969621 ) ) ;
#19771=CARTESIAN_POINT ( 'NONE',  ( 24.42567939027770407, 10.22651298688739097, -219.4562066833365748 ) ) ;
#19773=CARTESIAN_POINT ( 'NONE',  ( 25.75976839005050323, -3.608312289253767347, -220.3697909415571417 ) ) ;
#19774=CARTESIAN_POINT ( 'NONE',  ( -27.88251101234890328, -7.575382714962081820, -221.6715981084135478 ) ) ;
#19777=CARTESIAN_POINT ( 'NONE',  ( -1.946052076048385482, 22.23149728939677061, -232.8927760318659068 ) ) ;
#19778=CARTESIAN_POINT ( 'NONE',  ( 29.48160760559006732, -8.328447718542550504, -230.7159994440206390 ) ) ;
#19779=CARTESIAN_POINT ( 'NONE',  ( 19.06763123184207487, -2.048228142369658666, -218.2337357994572073 ) ) ;
#19780=CARTESIAN_POINT ( 'NONE',  ( -15.36327147092456791, 5.453733681707060299, -220.0043800961136355 ) ) ;
#19781=CARTESIAN_POINT ( 'NONE',  ( 17.24952650401854370, 25.19767938110938843, -224.5319471861414797 ) ) ;
#19782=CARTESIAN_POINT ( 'NONE',  ( 14.78510113471881304, 14.77128235908076803, -230.8056908117964383 ) ) ;
#19784=CARTESIAN_POINT ( 'NONE',  ( 0.7148793108008648645, -17.78534256477599840, -218.6573294195452775 ) ) ;
#19785=CARTESIAN_POINT ( 'NONE',  ( 4.401501667365108617, 18.53594119471695123, -215.1186850315663150 ) ) ;
#19786=CARTESIAN_POINT ( 'NONE',  ( -10.33514150881494942, 13.62639309082336503, -216.9544063991933172 ) ) ;
#19787=CARTESIAN_POINT ( 'NONE',  ( 28.44445586451508845, -4.662230540760189612, -220.9797193573593290 ) ) ;
#19788=CARTESIAN_POINT ( 'NONE',  ( -3.855805549595750392, 26.68244055262801950, -232.4569730455296508 ) ) ;
#19791=CARTESIAN_POINT ( 'NONE',  ( -5.836418080594380164, 30.19240250712089590, -223.8354869487762357 ) ) ;
#19792=CARTESIAN_POINT ( 'NONE',  ( 12.66989206167516357, 2.082990619159506007, -225.6419847029432901 ) ) ;
#19793=CARTESIAN_POINT ( 'NONE',  ( -24.24202834850560606, 19.05981756344202438, -226.6980666352953335 ) ) ;
#19794=CARTESIAN_POINT ( 'NONE',  ( 14.32085100525799248, 9.220655089380342062, -219.9006227404039464 ) ) ;
#19795=CARTESIAN_POINT ( 'NONE',  ( 3.198229568054530070, 16.42319727383711481, -222.3960047798183552 ) ) ;
#19797=CARTESIAN_POINT ( 'NONE',  ( -4.824452364631481416, 22.01523768541901305, -216.8350837474290245 ) ) ;
#19798=CARTESIAN_POINT ( 'NONE',  ( -8.514447835183077018, -10.26590951297754195, -225.5321622820681569 ) ) ;
#19799=CARTESIAN_POINT ( 'NONE',  ( 17.99029889091409018, 9.613712288440757092, -232.0298403238024036 ) ) ;
#19800=CARTESIAN_POINT ( 'NONE',  ( -9.981957700435337699, -28.23530775694580441, -222.3321348641582347 ) ) ;
#19802=CARTESIAN_POINT ( 'NONE',  ( -22.07068341299880743, 18.38202870573248049, -227.7785760498121306 ) ) ;
#19804=CARTESIAN_POINT ( 'NONE',  ( 8.339826811406878093, -13.81198187275966660, -229.8741491687588621 ) ) ;
#19805=CARTESIAN_POINT ( 'NONE',  ( 7.042184411928968935, 23.28260216771182556, -230.5707103145148267 ) ) ;
#19806=CARTESIAN_POINT ( 'NONE',  ( -10.16319438574952372, 11.71174522937666040, -227.8434026503654479 ) ) ;
#19807=CARTESIAN_POINT ( 'NONE',  ( -30.17036082276531772, 5.959165309317525860, -219.4883053239162791 ) ) ;
#19808=CARTESIAN_POINT ( 'NONE',  ( -16.80743794350546594, -8.145538706591455735, -220.2004866397506078 ) ) ;
#19809=CARTESIAN_POINT ( 'NONE',  ( 14.29548763234129538, 2.320071712424730315, -230.2610858871018422 ) ) ;
#19812=CARTESIAN_POINT ( 'NONE',  ( -10.37549270978917448, -7.969494006339708392, -220.1790165754723603 ) ) ;
#19813=CARTESIAN_POINT ( 'NONE',  ( 2.485733319737138736, 14.76073968410796056, -221.5245536174130905 ) ) ;
#19814=CARTESIAN_POINT ( 'NONE',  ( 12.88374853655145458, 4.106359831454843068, -228.1016120772327440 ) ) ;
#19816=CARTESIAN_POINT ( 'NONE',  ( -16.48883219358909713, 20.84100960965193394, -219.4392138569792507 ) ) ;
#19817=CARTESIAN_POINT ( 'NONE',  ( 10.82528077991200810, 8.849546035972329250, -221.2068619981234008 ) ) ;
#19819=CARTESIAN_POINT ( 'NONE',  ( 3.208289162541382300, -18.46136333555241293, -230.6641274008648850 ) ) ;
#19820=CARTESIAN_POINT ( 'NONE',  ( -1.198425787605166715, -24.00698511249634137, -218.1862405767648170 ) ) ;
#19822=CARTESIAN_POINT ( 'NONE',  ( 26.29894631880581812, 12.29609390142961090, -226.3100047295820332 ) ) ;
#19823=CARTESIAN_POINT ( 'NONE',  ( 24.96294718070021901, -13.86220829677249178, -229.4442241490162075 ) ) ;
#19824=CARTESIAN_POINT ( 'NONE',  ( -24.76115377241536208, -2.015397159694146456, -231.8500816169410825 ) ) ;
#19825=CARTESIAN_POINT ( 'NONE',  ( -12.11864581566431553, -23.10742878804749978, -232.9192999331436909 ) ) ;
#19826=CARTESIAN_POINT ( 'NONE',  ( 14.96080648943632241, 22.28365808184747721, -220.1237743409445216 ) ) ;
#19827=CARTESIAN_POINT ( 'NONE',  ( -12.10258892854866275, 5.599955477755926836, -221.6590149575334010 ) ) ;
#19828=CARTESIAN_POINT ( 'NONE',  ( 2.539761864897490007, 23.64215977235053501, -233.4645566207487661 ) ) ;
#19829=CARTESIAN_POINT ( 'NONE',  ( -2.426309470044460959, 27.69042070294474556, -223.4541227565655674 ) ) ;
#19830=CARTESIAN_POINT ( 'NONE',  ( 13.42973690470193837, -10.83953015014330035, -233.9990574442320224 ) ) ;
#19831=CARTESIAN_POINT ( 'NONE',  ( 12.08198696763335178, 15.54678077493410981, -216.6084679670902631 ) ) ;
#19832=CARTESIAN_POINT ( 'NONE',  ( -21.67128887413246119, 15.53484693247673043, -229.0088198863946900 ) ) ;
#19833=CARTESIAN_POINT ( 'NONE',  ( -18.93763370444446181, -0.7340653299870684156, -219.7345063954518594 ) ) ;
#19835=CARTESIAN_POINT ( 'NONE',  ( 1.967796959512672306, -15.42100964229427085, -222.1538042820122314 ) ) ;
#19839=CARTESIAN_POINT ( 'NONE',  ( 25.33562512631297281, 12.25422971834577268, -228.6777356031426791 ) ) ;
#19840=CARTESIAN_POINT ( 'NONE',  ( 12.71657619101469194, -13.18628128886902040, -219.4305778833985414 ) ) ;
#19842=CARTESIAN_POINT ( 'NONE',  ( -5.519971913460887336, -12.21762732219001713, -227.2962593638428359 ) ) ;
#19844=CARTESIAN_POINT ( 'NONE',  ( -2.208416658185406334, 29.10348627872611615, -219.8480645685746424 ) ) ;
#19845=CARTESIAN_POINT ( 'NONE',  ( -1.584125552723561592, 20.48724127025963782, -214.7515060525244621 ) ) ;
#19847=CARTESIAN_POINT ( 'NONE',  ( -16.65698539163286540, 11.03290537638306112, -233.6474915129378758 ) ) ;
#19848=CARTESIAN_POINT ( 'NONE',  ( 27.38348740615853316, -3.050674415727137045, -231.0934891209028876 ) ) ;
#19851=CARTESIAN_POINT ( 'NONE',  ( -12.74846050492543625, 19.93509882904884734, -216.0172840992881049 ) ) ;
#19852=CARTESIAN_POINT ( 'NONE',  ( -3.265885032814331623, -11.59335615597398217, -224.1764024733101053 ) ) ;
#19855=CARTESIAN_POINT ( 'NONE',  ( -15.20262116893801974, 8.038155052917188570, -217.6767387945475036 ) ) ;
#19857=CARTESIAN_POINT ( 'NONE',  ( 15.58465056415575312, 2.812367138262562349, -229.5090343034091234 ) ) ;
#19858=CARTESIAN_POINT ( 'NONE',  ( 3.100794261777709782, 20.70580715608724276, -231.8781843337728219 ) ) ;
#19860=CARTESIAN_POINT ( 'NONE',  ( 14.73597170006453361, 7.272367905564328439, -221.0092474305599239 ) ) ;
#19861=CARTESIAN_POINT ( 'NONE',  ( -13.03991958801536555, -12.43893258430110471, -220.5791972147702040 ) ) ;
#19863=CARTESIAN_POINT ( 'NONE',  ( -11.35482716595652875, 11.86850131893102223, -220.6599844941370350 ) ) ;
#19864=CARTESIAN_POINT ( 'NONE',  ( 7.018811797190238622, 13.93862807232938472, -230.2855929063610176 ) ) ;
#19865=CARTESIAN_POINT ( 'NONE',  ( -1.406618399933933006, 16.47239985789244443, -232.2564017133012726 ) ) ;
#19868=CARTESIAN_POINT ( 'NONE',  ( 29.37495210618232022, -3.074218464324032229, -220.1817713028459025 ) ) ;
#19871=CARTESIAN_POINT ( 'NONE',  ( -11.79584727357715934, 6.509288465425584036, -222.6080315736180921 ) ) ;
#19872=CARTESIAN_POINT ( 'NONE',  ( -18.76818401764774080, -23.60322278862490109, -229.9112526505913365 ) ) ;
#19873=CARTESIAN_POINT ( 'NONE',  ( 18.60971343765040942, 2.368090295052050820, -218.6871071987073094 ) ) ;
#19874=CARTESIAN_POINT ( 'NONE',  ( 10.83706092800007781, 10.12544885278926543, -227.1716144446442343 ) ) ;
#19875=CARTESIAN_POINT ( 'NONE',  ( 15.02951300086239428, -2.213105892075448278, -222.9721716646413086 ) ) ;
#19878=CARTESIAN_POINT ( 'NONE',  ( -28.05279008194460744, 4.018900919424986284, -224.6698354068587662 ) ) ;
#19879=CARTESIAN_POINT ( 'NONE',  ( 10.81638188557560731, 14.98959006186633403, -234.2424515599453514 ) ) ;
#19881=CARTESIAN_POINT ( 'NONE',  ( 14.95414693437772868, 8.262206471704862665, -230.1862972580043163 ) ) ;
#19883=CARTESIAN_POINT ( 'NONE',  ( 17.64863983146639015, -7.217312291206318342, -219.9249463058993399 ) ) ;
#19884=CARTESIAN_POINT ( 'NONE',  ( -14.76273180397945772, -6.370707202906876532, -220.0066229284273334 ) ) ;
#19887=CARTESIAN_POINT ( 'NONE',  ( -8.523771322135640816, 24.09653697920728987, -233.1071395647740303 ) ) ;
#19888=CARTESIAN_POINT ( 'NONE',  ( 15.43677305580571435, -6.701975615562529853, -215.9934368197604897 ) ) ;
#19890=CARTESIAN_POINT ( 'NONE',  ( 20.89700225552940793, -4.547446057044195911, -232.3806459760843666 ) ) ;
#19891=CARTESIAN_POINT ( 'NONE',  ( -18.05576253097465766, 2.935622250037499104, -232.1557308718028594 ) ) ;
#19892=CARTESIAN_POINT ( 'NONE',  ( 13.93840998928060415, 0.7705246578886114639, -220.8158265847476116 ) ) ;
#19893=CARTESIAN_POINT ( 'NONE',  ( 14.72046356508972309, 21.23077830076469041, -229.4562045376679578 ) ) ;
#19896=CARTESIAN_POINT ( 'NONE',  ( 3.878020530997904114, -17.84699472038997214, -232.6985457136631794 ) ) ;
#19898=CARTESIAN_POINT ( 'NONE',  ( -28.88770769694534479, 14.24820799418726480, -223.2044777450442155 ) ) ;
#19899=CARTESIAN_POINT ( 'NONE',  ( -4.678665819194652187, 12.50541869316310262, -220.1509054161798247 ) ) ;
#19900=CARTESIAN_POINT ( 'NONE',  ( 6.839751633953758514, 19.11639828585652623, -235.1218211620789873 ) ) ;
#19901=CARTESIAN_POINT ( 'NONE',  ( 18.69377297094946755, -6.763382089143314957, -232.1160126380615338 ) ) ;
#19902=CARTESIAN_POINT ( 'NONE',  ( -10.24288955603410933, 28.30762631303078791, -220.8855665231519083 ) ) ;
#19904=CARTESIAN_POINT ( 'NONE',  ( -6.094651895680649467, 13.59752566126439177, -221.0608041154719103 ) ) ;
#19905=CARTESIAN_POINT ( 'NONE',  ( -15.82952867276381603, 3.677461268355039170, -227.9997968350711801 ) ) ;
#19907=CARTESIAN_POINT ( 'NONE',  ( -10.30050448363967419, 10.07750059423401190, -220.1837019037183723 ) ) ;
#19908=CARTESIAN_POINT ( 'NONE',  ( 25.69300549816939494, 5.947472783069708946, -230.6131061331718115 ) ) ;
#19909=CARTESIAN_POINT ( 'NONE',  ( 6.402706778685327116, 14.41397785959879307, -226.0127495172349086 ) ) ;
#19911=CARTESIAN_POINT ( 'NONE',  ( 13.55451907249704213, 16.71566520821242818, -219.1474322952048226 ) ) ;
#19912=CARTESIAN_POINT ( 'NONE',  ( -24.92024473536680773, -13.74570206812420103, -220.1598944320903115 ) ) ;
#19913=CARTESIAN_POINT ( 'NONE',  ( 22.66390650824515873, 11.48342577402021725, -231.3155567808436217 ) ) ;
#19914=CARTESIAN_POINT ( 'NONE',  ( 0.1236778125412633655, -13.14499247612405775, -221.8775184276742323 ) ) ;
#19916=CARTESIAN_POINT ( 'NONE',  ( -7.965409144353247761, 13.56739834143082213, -221.6246244520798712 ) ) ;
#19918=CARTESIAN_POINT ( 'NONE',  ( 13.09169075717699293, -6.869491136113572871, -220.8313809912125691 ) ) ;
#19919=CARTESIAN_POINT ( 'NONE',  ( 20.54489901492447501, 10.52141067440427591, -216.2005526543161693 ) ) ;
#19920=CARTESIAN_POINT ( 'NONE',  ( -16.12870690754239078, 23.19263481078822053, -221.6099859194323471 ) ) ;
#19921=CARTESIAN_POINT ( 'NONE',  ( -15.42311360645077301, 11.97619046995196079, -234.9244673706848801 ) ) ;
#19922=CARTESIAN_POINT ( 'NONE',  ( -18.83136555461844708, -9.493528738360442532, -219.1308048892593945 ) ) ;
#19923=CARTESIAN_POINT ( 'NONE',  ( -15.94549496081242346, -0.04271059606100771622, -224.7066567765017169 ) ) ;
#19927=CARTESIAN_POINT ( 'NONE',  ( -23.12176686270140991, -7.251528982847554872, -234.5139663548038413 ) ) ;
#19928=CARTESIAN_POINT ( 'NONE',  ( 2.471164685565028662, 14.01327037412690935, -223.4905256513065410 ) ) ;
#19929=CARTESIAN_POINT ( 'NONE',  ( 25.62718606866737403, 13.33219119508369310, -230.9315691959737933 ) ) ;
#19930=CARTESIAN_POINT ( 'NONE',  ( -18.09605518090995702, 22.22778748761825085, -222.5443354630425290 ) ) ;
#19931=CARTESIAN_POINT ( 'NONE',  ( 11.20580770355584299, 27.81589616365139150, -231.3138133330081132 ) ) ;
#19933=CARTESIAN_POINT ( 'NONE',  ( 8.192339082998598698, -27.06056373437490947, -224.5174968915583236 ) ) ;
#19935=CARTESIAN_POINT ( 'NONE',  ( 1.632321987819951969, -14.78074153629778387, -224.5834756332612301 ) ) ;
#19936=CARTESIAN_POINT ( 'NONE',  ( -31.76239872120898511, 5.177298019713663990, -226.5714959923072342 ) ) ;
#19937=CARTESIAN_POINT ( 'NONE',  ( 15.54083024098960486, -10.44392130763852222, -217.6620978190037476 ) ) ;
#19938=CARTESIAN_POINT ( 'NONE',  ( 26.86542643433637423, 1.561297562127881511, -231.3515426572852505 ) ) ;
#19940=CARTESIAN_POINT ( 'NONE',  ( -21.63546480557098306, -21.44004028177477750, -223.8762611443524122 ) ) ;
#19942=CARTESIAN_POINT ( 'NONE',  ( 3.174664235197445006, 17.30896320251298448, -221.0803896709622620 ) ) ;
#19943=CARTESIAN_POINT ( 'NONE',  ( -14.98215928292561294, 22.79623052288931362, -230.3289734367122890 ) ) ;
#19944=CARTESIAN_POINT ( 'NONE',  ( 11.82943521288609823, 27.58963564415041247, -226.1180395413371400 ) ) ;
#19945=CARTESIAN_POINT ( 'NONE',  ( 7.487569386194327770, 15.49107591903592862, -229.0624668269501001 ) ) ;
#19946=CARTESIAN_POINT ( 'NONE',  ( 19.49551695935633688, -21.73806820219217428, -217.5227155576580742 ) ) ;
#19947=CARTESIAN_POINT ( 'NONE',  ( 8.379126514044342500, 15.76264856365358646, -232.1787896114811360 ) ) ;
#19948=CARTESIAN_POINT ( 'NONE',  ( -12.70465517376339193, 12.03139199664008530, -229.6235454691090752 ) ) ;
#19949=CARTESIAN_POINT ( 'NONE',  ( -15.72195651633673208, 2.938252489821347346, -222.2698596109374023 ) ) ;
#19950=CARTESIAN_POINT ( 'NONE',  ( -1.981531036097845533, -15.05108582582333909, -227.0172948689592829 ) ) ;
#19954=CARTESIAN_POINT ( 'NONE',  ( 12.58590500897257947, 11.38573988265384607, -230.4867078522624695 ) ) ;
#19955=CARTESIAN_POINT ( 'NONE',  ( 10.38773686668317531, -11.52324865342443516, -226.2052026729718932 ) ) ;
#19958=CARTESIAN_POINT ( 'NONE',  ( -8.258403559667634397, -29.80786866836635696, -223.3983869762195127 ) ) ;
#19960=CARTESIAN_POINT ( 'NONE',  ( -2.958555384449997661, 13.07587799061801093, -222.7767538261418565 ) ) ;
#19961=CARTESIAN_POINT ( 'NONE',  ( 3.889974896201825239, 13.98719620150063214, -218.1465764473210527 ) ) ;
#19963=CARTESIAN_POINT ( 'NONE',  ( -3.843007962268670585, 27.94983497691806917, -231.4302614368887703 ) ) ;
#19964=CARTESIAN_POINT ( 'NONE',  ( -23.30703516638871875, -0.6243632158918477337, -216.1214812734271220 ) ) ;
#19967=CARTESIAN_POINT ( 'NONE',  ( -11.49049084071896409, 11.06834963248926940, -218.3354249205727058 ) ) ;
#19968=CARTESIAN_POINT ( 'NONE',  ( -21.30077981517617047, -23.37245693150986270, -228.9371924788557351 ) ) ;
#19969=CARTESIAN_POINT ( 'NONE',  ( 14.68556740487494849, -6.365102927765655672, -229.6664356779805587 ) ) ;
#19970=CARTESIAN_POINT ( 'NONE',  ( -8.966714183099560032, 19.05224306381768073, -234.0879867025980445 ) ) ;
#19971=CARTESIAN_POINT ( 'NONE',  ( 19.10353041285295816, 2.510539514498965730, -232.1135168369976896 ) ) ;
#19972=CARTESIAN_POINT ( 'NONE',  ( 1.430961520682887400, 16.89318350835024063, -220.3256763723340157 ) ) ;
#19974=CARTESIAN_POINT ( 'NONE',  ( 18.14488609917747652, 6.993670804558928644, -231.4804853770579882 ) ) ;
#19975=CARTESIAN_POINT ( 'NONE',  ( -8.698852260299409167, -27.05211559305675451, -224.0453856107860986 ) ) ;
#19978=CARTESIAN_POINT ( 'NONE',  ( -10.16319438574952372, 11.71174522937666040, -227.8434026503654479 ) ) ;
#19979=CARTESIAN_POINT ( 'NONE',  ( 21.26803326031697949, 19.54255073453192892, -230.5813148908474659 ) ) ;
#19980=CARTESIAN_POINT ( 'NONE',  ( -5.786930954831501772, 15.78543306641166311, -231.0475152612371517 ) ) ;
#19981=CARTESIAN_POINT ( 'NONE',  ( -25.99367553232993799, -4.794975032520305547, -231.0351783075731191 ) ) ;
#19984=CARTESIAN_POINT ( 'NONE',  ( -9.171998067665157350, 9.395241133357435714, -226.3428046914542051 ) ) ;
#19985=CARTESIAN_POINT ( 'NONE',  ( -5.577337716965932835, -27.36628652700976971, -219.4670492756933413 ) ) ;
#19986=CARTESIAN_POINT ( 'NONE',  ( 15.50884165284638705, 1.028647572718199843, -227.8181348745474679 ) ) ;
#19987=CARTESIAN_POINT ( 'NONE',  ( 11.82943521288609823, 27.58963564415041247, -226.1180395413371400 ) ) ;
#19990=CARTESIAN_POINT ( 'NONE',  ( -15.46752262371512820, 15.15798787883389487, -233.5981584775992701 ) ) ;
#19991=CARTESIAN_POINT ( 'NONE',  ( 21.18605525173251891, 3.426801613781890854, -232.1183243183448894 ) ) ;
#19992=CARTESIAN_POINT ( 'NONE',  ( 15.34286276367735979, 1.557318373440422565, -222.4358706187587416 ) ) ;
#19994=CARTESIAN_POINT ( 'NONE',  ( 16.07305932912010960, 0.9253679043337685872, -229.0409936706996064 ) ) ;
#19996=CARTESIAN_POINT ( 'NONE',  ( 26.20608998270887469, -2.199599969171641689, -229.6935040011478009 ) ) ;
#19997=CARTESIAN_POINT ( 'NONE',  ( -21.80830016239255897, -4.781675611938959847, -217.4666014280278148 ) ) ;
#20001=CARTESIAN_POINT ( 'NONE',  ( -1.565160934061885500, 18.19073094521525391, -232.0278805765578909 ) ) ;
#20002=CARTESIAN_POINT ( 'NONE',  ( 20.64894435305043174, -4.471500992710556233, -235.2405168901568686 ) ) ;
#20003=CARTESIAN_POINT ( 'NONE',  ( 23.48720700658024896, -2.145453947144424500, -217.8824464111000054 ) ) ;
#20004=CARTESIAN_POINT ( 'NONE',  ( -24.39036648059286350, 13.21953970265592027, -220.1632778389106591 ) ) ;
#20005=CARTESIAN_POINT ( 'NONE',  ( -19.11923763334766946, 1.257783214997954202, -219.7591028439344711 ) ) ;
#20006=CARTESIAN_POINT ( 'NONE',  ( 9.322595869360968734, 23.38184458253662967, -230.2763482547081821 ) ) ;
#20007=CARTESIAN_POINT ( 'NONE',  ( -0.3443283949127196042, -14.50397496964243516, -224.4114361181996458 ) ) ;
#20009=CARTESIAN_POINT ( 'NONE',  ( -13.06407726305387307, 3.888674610242962348, -219.0371145420960204 ) ) ;
#20010=CARTESIAN_POINT ( 'NONE',  ( 19.29971334243027314, 24.42889259816135095, -228.2141526116784291 ) ) ;
#20011=CARTESIAN_POINT ( 'NONE',  ( 0.6332696906856497554, 18.74964962670039625, -234.8596399859513042 ) ) ;
#20012=CARTESIAN_POINT ( 'NONE',  ( 18.71980393303116230, -12.14054210360577457, -231.5113610204687120 ) ) ;
#20013=CARTESIAN_POINT ( 'NONE',  ( -2.958555384449997661, 13.07587799061801093, -222.7767538261418565 ) ) ;
#20014=CARTESIAN_POINT ( 'NONE',  ( -14.70651859537745487, 4.211702956367679107, -230.0357207626005334 ) ) ;
#20016=CARTESIAN_POINT ( 'NONE',  ( 19.07698357483942786, 25.86742807064150895, -222.6991278896559834 ) ) ;
#20017=CARTESIAN_POINT ( 'NONE',  ( -24.49083850720273148, 4.222094140707651100, -219.1543001448025905 ) ) ;
#20018=CARTESIAN_POINT ( 'NONE',  ( -12.78558550453068854, 7.693178343823584342, -230.0800953344970878 ) ) ;
#20019=CARTESIAN_POINT ( 'NONE',  ( 27.40550551777678123, 5.967061366481472895, -228.7463788799179554 ) ) ;
#20020=CARTESIAN_POINT ( 'NONE',  ( 3.191455400233187412, 17.67480163422566619, -220.7055581859663107 ) ) ;
#20023=CARTESIAN_POINT ( 'NONE',  ( 16.29563576379945999, 21.41235115595959826, -221.8114656550040991 ) ) ;
#20024=CARTESIAN_POINT ( 'NONE',  ( -9.078153229956912540, -10.71731945587431056, -228.5228069477245469 ) ) ;
#20025=CARTESIAN_POINT ( 'NONE',  ( 22.86997486125673618, 17.56009411325475966, -222.3578648042903296 ) ) ;
#20026=CARTESIAN_POINT ( 'NONE',  ( -0.1378336831626507664, -14.33879523207274964, -230.9095596798049144 ) ) ;
#20028=CARTESIAN_POINT ( 'NONE',  ( -15.51982305277792307, 19.76957551617798359, -231.4018974401358832 ) ) ;
#20030=CARTESIAN_POINT ( 'NONE',  ( 12.85536293311005451, -7.423602990911125410, -229.4216632760384300 ) ) ;
#20031=CARTESIAN_POINT ( 'NONE',  ( 20.88350594575732799, 13.65521425050155813, -232.8060468608549911 ) ) ;
#20032=CARTESIAN_POINT ( 'NONE',  ( -4.879985665934096772, 15.33285679834440174, -220.9402849574511833 ) ) ;
#20033=CARTESIAN_POINT ( 'NONE',  ( -12.13319425917249283, 4.024026700415168634, -229.5243363405849095 ) ) ;
#20034=CARTESIAN_POINT ( 'NONE',  ( -26.46950597041758968, -8.633348373924491170, -225.4226425040951085 ) ) ;
#20035=CARTESIAN_POINT ( 'NONE',  ( -25.48569860171343748, 4.299098795181173216, -219.7804659532078801 ) ) ;
#20038=CARTESIAN_POINT ( 'NONE',  ( -27.95235446785429545, -6.124178816625678756, -218.3296603670965226 ) ) ;
#20039=CARTESIAN_POINT ( 'NONE',  ( 10.88376588832297287, 7.577514201227793400, -222.7215714477710833 ) ) ;
#20040=CARTESIAN_POINT ( 'NONE',  ( 18.81274554574540403, 10.85963742466947224, -234.0446454529665345 ) ) ;
#20041=CARTESIAN_POINT ( 'NONE',  ( -2.121548062149551495, 13.26065194155116345, -221.8830439064491884 ) ) ;
#20042=CARTESIAN_POINT ( 'NONE',  ( 7.739849882373770917, 11.59357455229016409, -219.5521933286238720 ) ) ;
#20043=CARTESIAN_POINT ( 'NONE',  ( 0.5565384680698680642, -16.73444667301361122, -219.8404036742738015 ) ) ;
#20045=CARTESIAN_POINT ( 'NONE',  ( 0.7797512750231831991, -26.58197935702783354, -230.4407411870234625 ) ) ;
#20047=CARTESIAN_POINT ( 'NONE',  ( -10.54177647804913320, 7.401649028325941515, -220.3980514230326264 ) ) ;
#20048=CARTESIAN_POINT ( 'NONE',  ( 20.25084204406298127, -10.11176871144018818, -232.7817218064674591 ) ) ;
#20049=CARTESIAN_POINT ( 'NONE',  ( -27.09167109716269550, -0.2825935922571593539, -219.8389404328913486 ) ) ;
#20050=CARTESIAN_POINT ( 'NONE',  ( -6.012234575298915473, -13.00555924700598709, -229.4955436083688483 ) ) ;
#20051=CARTESIAN_POINT ( 'NONE',  ( 17.98704291748025952, 16.14142602298251461, -217.3684083235702644 ) ) ;
#20053=CARTESIAN_POINT ( 'NONE',  ( -22.57344584932824105, 14.14390280519600473, -217.2212543695777924 ) ) ;
#20054=CARTESIAN_POINT ( 'NONE',  ( 8.645835506124264214, 12.38899589144949687, -223.4673650485651990 ) ) ;
#20055=CARTESIAN_POINT ( 'NONE',  ( 10.02513374692848913, 18.81568788741115128, -217.1505009242214612 ) ) ;
#20056=CARTESIAN_POINT ( 'NONE',  ( 14.91731358302415877, 13.33846450914490056, -217.2468882285060658 ) ) ;
#20057=CARTESIAN_POINT ( 'NONE',  ( 14.18953136290653205, -9.569333121228954298, -216.2179364387266389 ) ) ;
#20058=CARTESIAN_POINT ( 'NONE',  ( 13.10956039622986324, 4.581323766968698585, -221.0328522389722252 ) ) ;
#20059=CARTESIAN_POINT ( 'NONE',  ( -11.69222874857179484, 25.57550432052970280, -219.9467848335519591 ) ) ;
#20060=CARTESIAN_POINT ( 'NONE',  ( -13.02663300398358892, -17.15584419188240162, -232.5492131852532793 ) ) ;
#20063=CARTESIAN_POINT ( 'NONE',  ( 24.42567939027770407, 10.22651298688739097, -219.4562066833365748 ) ) ;
#20064=CARTESIAN_POINT ( 'NONE',  ( 22.17529396115045870, -12.37645153867399195, -229.8268438261158906 ) ) ;
#20065=CARTESIAN_POINT ( 'NONE',  ( -13.51406939156936104, 10.04301168678160749, -230.1761202643687056 ) ) ;
#20067=CARTESIAN_POINT ( 'NONE',  ( -5.902479482706956659, -14.78727544128710214, -218.5565286504736946 ) ) ;
#20068=CARTESIAN_POINT ( 'NONE',  ( 29.55842656951424985, 4.785221541509360854, -220.5134865854112718 ) ) ;
#20069=CARTESIAN_POINT ( 'NONE',  ( 4.569118550756183339, 31.72363458735121000, -222.3920438419263519 ) ) ;
#20071=CARTESIAN_POINT ( 'NONE',  ( 3.449504654906655254, 27.59247159270940841, -231.3461799890608859 ) ) ;
#20072=CARTESIAN_POINT ( 'NONE',  ( -15.34124043857492303, -4.213426711746545372, -218.8308339851419078 ) ) ;
#20075=CARTESIAN_POINT ( 'NONE',  ( 4.301648988406530094, 13.23079486486395240, -223.2766268961034655 ) ) ;
#20076=CARTESIAN_POINT ( 'NONE',  ( -6.608244874605412100, -9.640126028631323507, -223.8427097396816805 ) ) ;
#20077=CARTESIAN_POINT ( 'NONE',  ( 6.427665535191954937, -16.40046818492683656, -232.5919299485929912 ) ) ;
#20078=CARTESIAN_POINT ( 'NONE',  ( 13.49882595795384255, -9.201056071450322449, -219.2439763087855908 ) ) ;
#20079=CARTESIAN_POINT ( 'NONE',  ( -14.64425879132321384, 10.88727730234500868, -217.2315376225554644 ) ) ;
#20080=CARTESIAN_POINT ( 'NONE',  ( 10.12648780932046755, 24.76571117977573522, -228.8499436907259792 ) ) ;
#20082=CARTESIAN_POINT ( 'NONE',  ( -10.10782416658048710, 9.083762506436128703, -227.1045422723873344 ) ) ;
#20083=CARTESIAN_POINT ( 'NONE',  ( -13.53417258903678722, -8.044363197357762729, -224.1542709308240546 ) ) ;
#20084=CARTESIAN_POINT ( 'NONE',  ( -21.66803296057637951, 19.04503900041684616, -222.6603677762044526 ) ) ;
#20085=CARTESIAN_POINT ( 'NONE',  ( 17.23498165643884761, 6.576565757823654934, -216.5785374982484655 ) ) ;
#20086=CARTESIAN_POINT ( 'NONE',  ( 2.000982021813747291, 12.72833461843010205, -228.3416607300594308 ) ) ;
#20087=CARTESIAN_POINT ( 'NONE',  ( -17.40151406155100844, -6.170051014037699844, -218.8120118016391871 ) ) ;
#20090=CARTESIAN_POINT ( 'NONE',  ( -14.07917727715460821, 7.534853284453274291, -218.6337090155677458 ) ) ;
#20091=CARTESIAN_POINT ( 'NONE',  ( -13.20345004609422723, -27.40577205094947644, -221.7016714442654290 ) ) ;
#20092=CARTESIAN_POINT ( 'NONE',  ( 15.88514075556662242, 1.727533893982488244, -221.2479562541981011 ) ) ;
#20093=CARTESIAN_POINT ( 'NONE',  ( 15.85665641241444668, 18.24713744004561988, -217.7195292979064902 ) ) ;
#20095=CARTESIAN_POINT ( 'NONE',  ( 22.03647168421188240, 0.3315607655626218175, -232.0572713672587213 ) ) ;
#20096=CARTESIAN_POINT ( 'NONE',  ( -11.19223248830523332, 8.463078350427430507, -222.6400917074981578 ) ) ;
#20097=CARTESIAN_POINT ( 'NONE',  ( 14.70646826691583975, 6.155951851203820269, -230.2899142379868920 ) ) ;
#20098=CARTESIAN_POINT ( 'NONE',  ( 15.23010956230245228, 0.3844360911890600807, -222.0229298927499713 ) ) ;
#20100=CARTESIAN_POINT ( 'NONE',  ( -21.89065952084848021, -0.9940043559354364566, -216.9999999999999716 ) ) ;
#20101=CARTESIAN_POINT ( 'NONE',  ( 18.18465861704851960, -5.084991117879029687, -230.0453011691623999 ) ) ;
#20102=CARTESIAN_POINT ( 'NONE',  ( -26.98579662683621194, -8.531126968542736222, -229.5232528995939845 ) ) ;
#20106=CARTESIAN_POINT ( 'NONE',  ( 9.322595869360968734, 23.38184458253662967, -230.2763482547081821 ) ) ;
#20107=CARTESIAN_POINT ( 'NONE',  ( 12.92460608403495037, -28.21656386930617089, -223.0937501850342812 ) ) ;
#20108=CARTESIAN_POINT ( 'NONE',  ( 12.02378739738799140, -16.98783239109716092, -233.4545636224233931 ) ) ;
#20109=CARTESIAN_POINT ( 'NONE',  ( -22.13857085231108712, 6.545953331035805789, -217.2801712530867633 ) ) ;
#20110=CARTESIAN_POINT ( 'NONE',  ( 16.21758812354607215, 4.665393561625732488, -232.5634757513959983 ) ) ;
#20111=CARTESIAN_POINT ( 'NONE',  ( 15.04029996350473830, 7.457450192165341107, -220.5007084872782173 ) ) ;
#20112=CARTESIAN_POINT ( 'NONE',  ( 2.920206608988989760, -13.21961856575012639, -224.5557534934820865 ) ) ;
#20113=CARTESIAN_POINT ( 'NONE',  ( -13.09048442463468120, -0.002406630494250819839, -229.7150300986316438 ) ) ;
#20114=CARTESIAN_POINT ( 'NONE',  ( 3.889974896201825239, 13.98719620150063214, -218.1465764473210527 ) ) ;
#20115=CARTESIAN_POINT ( 'NONE',  ( 3.889974896201825239, 13.98719620150063214, -218.1465764473210527 ) ) ;
#20116=CARTESIAN_POINT ( 'NONE',  ( 22.50501984129641286, -15.15275112778533284, -228.8333022290248664 ) ) ;
#20118=CARTESIAN_POINT ( 'NONE',  ( -9.517741096562200909, 20.63709896626785678, -234.1036702156204967 ) ) ;
#20119=CARTESIAN_POINT ( 'NONE',  ( -17.96792326766206926, -0.6237852504629022299, -217.9759415197746932 ) ) ;
#20120=CARTESIAN_POINT ( 'NONE',  ( 8.126072675580726212, 14.68573014611672534, -233.8823376361746966 ) ) ;
#20121=CARTESIAN_POINT ( 'NONE',  ( -15.10945752141584464, 6.470132813599071220, -220.1568141593501764 ) ) ;
#20122=CARTESIAN_POINT ( 'NONE',  ( -3.003186468682855104, 15.63968344752823469, -231.5301608670590667 ) ) ;
#20124=CARTESIAN_POINT ( 'NONE',  ( 7.042184411928968935, 23.28260216771182556, -230.5707103145148267 ) ) ;
#20127=CARTESIAN_POINT ( 'NONE',  ( -24.25245498015852874, 0.2109992039763788352, -218.1398602137601301 ) ) ;
#20128=CARTESIAN_POINT ( 'NONE',  ( 24.57222455393806015, 12.08236629421828212, -229.7319216558644541 ) ) ;
#20129=CARTESIAN_POINT ( 'NONE',  ( -11.33724117040414647, -11.57131516804904159, -228.9094961685112537 ) ) ;
#20130=CARTESIAN_POINT ( 'NONE',  ( -9.810154340578240095, 25.84808829058669488, -220.5759521898573610 ) ) ;
#20132=CARTESIAN_POINT ( 'NONE',  ( 12.74640035234706659, -6.767230903810586895, -221.4971111014800726 ) ) ;
#20133=CARTESIAN_POINT ( 'NONE',  ( 14.29768887814754663, 10.87030385293788548, -231.8067013864770161 ) ) ;
#20134=CARTESIAN_POINT ( 'NONE',  ( -4.130417896617784912, 16.21758012034559826, -229.8171973319304584 ) ) ;
#20135=CARTESIAN_POINT ( 'NONE',  ( -14.00980274651940682, 20.05588230486321066, -234.2453272803952586 ) ) ;
#20137=CARTESIAN_POINT ( 'NONE',  ( -16.09622215267033596, -6.362375831002168525, -228.5323951500822943 ) ) ;
#20138=CARTESIAN_POINT ( 'NONE',  ( 14.81251837262747983, -1.020578734748967209, -221.0290343291311785 ) ) ;
#20140=CARTESIAN_POINT ( 'NONE',  ( -26.73251495235368225, -0.6309583860051256599, -232.5016102969711085 ) ) ;
#20141=CARTESIAN_POINT ( 'NONE',  ( 9.211411085256067111, 16.86455563410128633, -232.8411836211112700 ) ) ;
#20142=CARTESIAN_POINT ( 'NONE',  ( -15.47996233766743934, 8.203483081506188768, -221.0931279926996353 ) ) ;
#20143=CARTESIAN_POINT ( 'NONE',  ( -3.712761995161701911, 23.50704853188985766, -216.1220552374512067 ) ) ;
#20144=CARTESIAN_POINT ( 'NONE',  ( 14.70646826691583975, 6.155951851203820269, -230.2899142379868920 ) ) ;
#20146=CARTESIAN_POINT ( 'NONE',  ( -19.56933409648781108, -21.97186532644649759, -218.6835957583845982 ) ) ;
#20148=CARTESIAN_POINT ( 'NONE',  ( -8.326748185965973548, -13.59788789161040512, -220.4531618457016862 ) ) ;
#20149=CARTESIAN_POINT ( 'NONE',  ( -26.98548179121306845, 3.096138561569834913, -233.8324893795610251 ) ) ;
#20150=CARTESIAN_POINT ( 'NONE',  ( 6.053458391837899910, -12.85229775019162268, -220.9645494416007523 ) ) ;
#20151=CARTESIAN_POINT ( 'NONE',  ( -15.89118508636071958, -1.798691612803976492, -229.3605869667087234 ) ) ;
#20152=CARTESIAN_POINT ( 'NONE',  ( -26.98579662683621194, -8.531126968542736222, -229.5232528995939845 ) ) ;
#20153=CARTESIAN_POINT ( 'NONE',  ( 11.35656094503625901, 14.01405796444069018, -230.6944611846958537 ) ) ;
#20155=CARTESIAN_POINT ( 'NONE',  ( -8.308618357598591686, 12.44656112581930785, -228.0014162119141474 ) ) ;
#20156=CARTESIAN_POINT ( 'NONE',  ( 11.44717363687632528, 10.34477785005100969, -220.4550508611108341 ) ) ;
#20157=CARTESIAN_POINT ( 'NONE',  ( -2.208416658185406334, 29.10348627872611615, -219.8480645685746424 ) ) ;
#20158=CARTESIAN_POINT ( 'NONE',  ( 6.729623925010410623, 16.84721552001897038, -219.9221131804260381 ) ) ;
#20159=CARTESIAN_POINT ( 'NONE',  ( 9.622280932921700725, -12.40415793303572300, -216.8820201732712860 ) ) ;
#20160=CARTESIAN_POINT ( 'NONE',  ( 0.1866476013601106043, 25.93503619265524307, -233.5574764272258790 ) ) ;
#20162=CARTESIAN_POINT ( 'NONE',  ( -10.46545893407769157, -9.768586176915025732, -226.8636372813723199 ) ) ;
#20163=CARTESIAN_POINT ( 'NONE',  ( -13.93333636822611155, 3.327141996558931947, -221.4468162587888287 ) ) ;
#20164=DIRECTION ( 'NONE',  ( -0.9940043559354330149, -0.1093404791528966163, -6.737719923507020479E-14 ) ) ;
#20166=CARTESIAN_POINT ( 'NONE',  ( 14.19800769603076240, 4.587407146151301518, -224.2928935459285071 ) ) ;
#20167=CARTESIAN_POINT ( 'NONE',  ( 15.80653577316150837, -24.09293983082412893, -226.7583346419201575 ) ) ;
#20168=CARTESIAN_POINT ( 'NONE',  ( -12.87285471141929172, 9.485162256560764504, -229.1865421006261840 ) ) ;
#20169=CARTESIAN_POINT ( 'NONE',  ( 1.656472371294090085, 27.29382523973669095, -230.4991099578876117 ) ) ;
#20170=CARTESIAN_POINT ( 'NONE',  ( -13.52935284690462758, -5.503084506376929141, -222.3607690796775671 ) ) ;
#20171=CARTESIAN_POINT ( 'NONE',  ( 12.88374853655145458, 4.106359831454843068, -228.1016120772327440 ) ) ;
#20173=CARTESIAN_POINT ( 'NONE',  ( 12.90536070039565963, 17.66816134723717724, -234.8562535614228750 ) ) ;
#20175=CARTESIAN_POINT ( 'NONE',  ( -3.003186468682855104, 15.63968344752823469, -231.5301608670590667 ) ) ;
#20176=CARTESIAN_POINT ( 'NONE',  ( 20.08508968036338871, -9.819972662663129626, -218.2881406113160381 ) ) ;
#20177=CARTESIAN_POINT ( 'NONE',  ( 23.33467929415965614, -0.4823873731835089940, -233.9427286327415629 ) ) ;
#20179=CARTESIAN_POINT ( 'NONE',  ( -0.9414827276148034496, 23.96885519606619752, -216.4491898092606164 ) ) ;
#20180=CARTESIAN_POINT ( 'NONE',  ( -15.15491452760745439, -27.84330619910961957, -221.4571841043341180 ) ) ;
#20181=CARTESIAN_POINT ( 'NONE',  ( 12.73130673999417795, -23.76414828096303467, -217.7386337832039942 ) ) ;
#20182=CARTESIAN_POINT ( 'NONE',  ( 19.06435866915521515, -20.24829071055443563, -218.8318535520223804 ) ) ;
#20183=CARTESIAN_POINT ( 'NONE',  ( -11.83206531956964902, 10.60028422373495260, -231.1115289952381033 ) ) ;
#20184=CARTESIAN_POINT ( 'NONE',  ( 6.685304925496912354, 17.61973327427626046, -230.4152170797364931 ) ) ;
#20185=CARTESIAN_POINT ( 'NONE',  ( -16.20072894238734307, 0.5024448614660336210, -230.4554067149722130 ) ) ;
#20186=CARTESIAN_POINT ( 'NONE',  ( -13.84508897751235246, 5.904954704487344941, -218.7722818424232401 ) ) ;
#20187=CARTESIAN_POINT ( 'NONE',  ( -14.78201816772319077, -5.155518158621814173, -222.1275223803717154 ) ) ;
#20190=CARTESIAN_POINT ( 'NONE',  ( -9.810154340578240095, 25.84808829058669488, -220.5759521898573610 ) ) ;
#20191=CARTESIAN_POINT ( 'NONE',  ( 17.66525298603349370, 4.919957226727790456, -233.3736646485340032 ) ) ;
#20192=CARTESIAN_POINT ( 'NONE',  ( 9.400341091271927851, 28.64465517894215196, -231.0823126271420165 ) ) ;
#20193=CARTESIAN_POINT ( 'NONE',  ( 27.76845665997775114, -9.103683020204879739, -229.9743915588940979 ) ) ;
#20196=CARTESIAN_POINT ( 'NONE',  ( -27.29953305526601426, 11.21644211419729054, -229.3676346105362995 ) ) ;
#20197=CARTESIAN_POINT ( 'NONE',  ( -13.08850661186922260, -6.354795836388488439, -231.9371199848366984 ) ) ;
#20199=CARTESIAN_POINT ( 'NONE',  ( 4.559463107227270662, 13.27337529356814017, -226.9596205199204633 ) ) ;
#20201=CARTESIAN_POINT ( 'NONE',  ( 8.818493748348606331, -10.89961555176610375, -227.9481955143288303 ) ) ;
#20203=CARTESIAN_POINT ( 'NONE',  ( -15.15434969228324924, 4.423874646950748613, -230.6144467931089821 ) ) ;
#20204=CARTESIAN_POINT ( 'NONE',  ( -18.63458318964815774, 8.046101765467303935, -217.8151248213926863 ) ) ;
#20206=CARTESIAN_POINT ( 'NONE',  ( 25.70381634773192658, 10.55338509461953400, -230.3576492130207782 ) ) ;
#20211=CARTESIAN_POINT ( 'NONE',  ( -25.17982544627478703, 0.9072515815786372784, -215.5253307415545692 ) ) ;
#20212=CARTESIAN_POINT ( 'NONE',  ( -13.67406442719345883, -9.319000780081536206, -231.1492214949047934 ) ) ;
#20215=CARTESIAN_POINT ( 'NONE',  ( 4.936777854427027989, 27.97379167488809060, -227.0886654730259124 ) ) ;
#20216=CARTESIAN_POINT ( 'NONE',  ( 7.898002370961310525, -21.57266348603731387, -216.1546105971396798 ) ) ;
#20217=CARTESIAN_POINT ( 'NONE',  ( 10.40291689048662782, -13.87512507945592333, -231.9656913702303029 ) ) ;
#20218=CARTESIAN_POINT ( 'NONE',  ( -16.50467377682197423, 21.56569464670658220, -229.9175202103629374 ) ) ;
#20219=CARTESIAN_POINT ( 'NONE',  ( 25.50289296650958448, 5.998088869914441901, -233.1161630295026157 ) ) ;
#20220=CARTESIAN_POINT ( 'NONE',  ( 15.99247752609008444, 10.72268246046808216, -230.5614800526110173 ) ) ;
#20222=CARTESIAN_POINT ( 'NONE',  ( -12.75670220164522384, -23.12103459569904373, -229.1084755445707799 ) ) ;
#20225=CARTESIAN_POINT ( 'NONE',  ( -11.79271689233719478, 3.876813423829604144, -228.6816298097564299 ) ) ;
#20227=CARTESIAN_POINT ( 'NONE',  ( 16.11883106748507188, 21.48229216499086291, -233.4985352728212433 ) ) ;
#20228=CARTESIAN_POINT ( 'NONE',  ( 29.34815638429084927, -3.655059647784748122, -228.0165508611016207 ) ) ;
#20229=CARTESIAN_POINT ( 'NONE',  ( 12.10245006109274080, 26.02147364279441888, -220.6079829738538649 ) ) ;
#20230=CARTESIAN_POINT ( 'NONE',  ( -11.67631226053870996, 6.737291529340801333, -227.3110382950315227 ) ) ;
#20232=CARTESIAN_POINT ( 'NONE',  ( 17.60070748514786132, 25.68479983175475567, -229.9331108608050158 ) ) ;
#20233=CARTESIAN_POINT ( 'NONE',  ( -25.06333669508177309, 2.553070212212491530, -230.2963116797556893 ) ) ;
#20234=CARTESIAN_POINT ( 'NONE',  ( -4.104500432947460808, 15.73223271406093460, -218.0734292856946297 ) ) ;
#20237=CARTESIAN_POINT ( 'NONE',  ( 3.614175329767659761, 21.98488100320606264, -219.0898850257099753 ) ) ;
#20239=CARTESIAN_POINT ( 'NONE',  ( 28.22932473237819551, -8.039268142081398949, -226.6539694142420558 ) ) ;
#20240=CARTESIAN_POINT ( 'NONE',  ( -3.400000000000003908, 0.000000000000000000, -224.9999999999999716 ) ) ;
#20241=CARTESIAN_POINT ( 'NONE',  ( -28.46519324992292965, -8.397260794665152517, -225.6705986409035347 ) ) ;
#20242=CARTESIAN_POINT ( 'NONE',  ( -13.56011990957801139, -0.3895158544032599202, -219.3211261236655218 ) ) ;
#20243=CARTESIAN_POINT ( 'NONE',  ( -13.72723917162997154, -9.146515947596070006, -227.8820830806802746 ) ) ;
#20245=CARTESIAN_POINT ( 'NONE',  ( -4.170472558179216804, 16.67407401355319152, -230.2690496885289804 ) ) ;
#20246=CARTESIAN_POINT ( 'NONE',  ( 6.930886114109415352, -28.33506752827666020, -226.0544877841801110 ) ) ;
#20247=CARTESIAN_POINT ( 'NONE',  ( 19.70286159681817750, 17.87637900817293612, -218.6154571368943493 ) ) ;
#20248=CARTESIAN_POINT ( 'NONE',  ( -4.855966894080006035, 26.75753167227873064, -230.1547293463117114 ) ) ;
#20249=CARTESIAN_POINT ( 'NONE',  ( -7.329856113536736828, 10.17606210583481818, -226.3085553030691415 ) ) ;
#20251=CARTESIAN_POINT ( 'NONE',  ( -27.33303184979533285, -3.055344081261842870, -227.4850045670461043 ) ) ;
#20252=CARTESIAN_POINT ( 'NONE',  ( 17.68508104102419409, 23.41266195669770767, -227.5327139115408954 ) ) ;
#20253=CARTESIAN_POINT ( 'NONE',  ( -28.05279008194460744, 4.018900919424986284, -224.6698354068587662 ) ) ;
#20255=CARTESIAN_POINT ( 'NONE',  ( -28.96081738894762125, -0.4213479615504204800, -230.3891733152809707 ) ) ;
#20256=CARTESIAN_POINT ( 'NONE',  ( 8.379126514044342500, 15.76264856365358646, -232.1787896114811360 ) ) ;
#20258=CARTESIAN_POINT ( 'NONE',  ( -16.58624905143161143, 8.715293938925766426, -220.0618460037763384 ) ) ;
#20259=CARTESIAN_POINT ( 'NONE',  ( -1.806671251568986669, 13.52068930966770388, -228.3567401718105430 ) ) ;
#20260=CARTESIAN_POINT ( 'NONE',  ( 16.71272566993619080, 8.989703107375911273, -217.4612081447889125 ) ) ;
#20262=CARTESIAN_POINT ( 'NONE',  ( -20.07469464351956390, -22.83895492621963896, -220.1373730632280967 ) ) ;
#20264=CARTESIAN_POINT ( 'NONE',  ( -7.786003226018990198, -12.23758553950863082, -224.1954257758910671 ) ) ;
#20266=CARTESIAN_POINT ( 'NONE',  ( -13.06407726305387307, 3.888674610242962348, -219.0371145420960204 ) ) ;
#20267=CARTESIAN_POINT ( 'NONE',  ( 6.166782020495575445, -26.61202787628535660, -217.6604608484729795 ) ) ;
#20268=CARTESIAN_POINT ( 'NONE',  ( 12.70896864779121316, -3.955665148817821386, -221.1719243096075900 ) ) ;
#20269=CARTESIAN_POINT ( 'NONE',  ( -25.98129645912436914, -15.13773040547512139, -224.1390156429105787 ) ) ;
#20270=CARTESIAN_POINT ( 'NONE',  ( 15.15306935214909778, 7.771180183537883757, -217.5526096523957165 ) ) ;
#20272=CARTESIAN_POINT ( 'NONE',  ( -11.11479000491124047, 20.76372272540567110, -218.2001872134434564 ) ) ;
#20273=CARTESIAN_POINT ( 'NONE',  ( 10.97349919442152810, 9.416813005082010690, -227.3764328406868742 ) ) ;
#20275=CARTESIAN_POINT ( 'NONE',  ( 22.84140515590350518, 18.29101041979067332, -226.2334522600520472 ) ) ;
#20276=CARTESIAN_POINT ( 'NONE',  ( 10.25308675723727347, 13.16459519580956972, -229.3963488176951273 ) ) ;
#20277=CARTESIAN_POINT ( 'NONE',  ( 20.49803729918260942, -22.47924998572259980, -218.9346008044765028 ) ) ;
#20278=CARTESIAN_POINT ( 'NONE',  ( -6.127117917506272882, 18.94558806480136681, -232.9763641438055117 ) ) ;
#20279=CARTESIAN_POINT ( 'NONE',  ( -17.84981083811007707, 0.8485253248287054628, -231.8041300026935119 ) ) ;
#20281=CARTESIAN_POINT ( 'NONE',  ( 21.35706335192880445, 15.67286272432725092, -219.2578158352350783 ) ) ;
#20282=CARTESIAN_POINT ( 'NONE',  ( 3.810076078852552950, -13.18001539772800612, -226.2402971015400510 ) ) ;
#20283=CARTESIAN_POINT ( 'NONE',  ( -14.69827142695382527, 14.49176359921644597, -217.9600391472806109 ) ) ;
#20284=CARTESIAN_POINT ( 'NONE',  ( -0.3197916200495275474, 16.38897215927557482, -229.9606066735827028 ) ) ;
#20285=CARTESIAN_POINT ( 'NONE',  ( -11.49803752765619258, -8.459563989871591971, -222.4296168992866853 ) ) ;
#20286=CARTESIAN_POINT ( 'NONE',  ( -27.28038240442402440, 5.683827137705129040, -226.0726697751923382 ) ) ;
#20288=CARTESIAN_POINT ( 'NONE',  ( 24.34047711160105720, 17.90454708687460794, -228.1939002122307159 ) ) ;
#20290=CARTESIAN_POINT ( 'NONE',  ( -3.755296588130283553, 23.77975947300719284, -233.7323173085780752 ) ) ;
#20291=CARTESIAN_POINT ( 'NONE',  ( 15.74534598441689504, -4.714293076379259873, -220.2687296774407173 ) ) ;
#20292=CARTESIAN_POINT ( 'NONE',  ( 21.28562020585086501, -15.94148943779260819, -218.1725164024425396 ) ) ;
#20294=CARTESIAN_POINT ( 'NONE',  ( -2.808235066048971440, 30.42019778760651150, -222.6481917607299295 ) ) ;
#20295=CARTESIAN_POINT ( 'NONE',  ( -19.75796449794633602, -18.82837501718038453, -216.0857152239166794 ) ) ;
#20296=CARTESIAN_POINT ( 'NONE',  ( -8.803769170443210612, -17.82266517633203406, -233.6972128408098683 ) ) ;
#20297=CARTESIAN_POINT ( 'NONE',  ( 20.38902395782249144, -18.95772103455488633, -230.9098670703349967 ) ) ;
#20298=CARTESIAN_POINT ( 'NONE',  ( -8.137644474477026435, 12.10064032984799098, -226.6735072060122036 ) ) ;
#20299=CARTESIAN_POINT ( 'NONE',  ( 11.16964468591631920, 25.71443501674299981, -224.7497461878887464 ) ) ;
#20300=CARTESIAN_POINT ( 'NONE',  ( -16.74550766701807447, 3.787526820511904813, -217.9802846976114381 ) ) ;
#20301=CARTESIAN_POINT ( 'NONE',  ( -14.64425879132321384, 10.88727730234500868, -217.2315376225554644 ) ) ;
#20302=CARTESIAN_POINT ( 'NONE',  ( -17.87876569233342749, -13.82805272504658944, -230.9569051913176168 ) ) ;
#20303=CARTESIAN_POINT ( 'NONE',  ( -10.32994309255856535, 16.55762392127841665, -218.3313395458419279 ) ) ;
#20304=CARTESIAN_POINT ( 'NONE',  ( 15.26539804565921621, 9.309431686815628382, -232.9129599938668207 ) ) ;
#20305=CARTESIAN_POINT ( 'NONE',  ( 8.126072675580726212, 14.68573014611672534, -233.8823376361746966 ) ) ;
#20306=CARTESIAN_POINT ( 'NONE',  ( 14.41459438711767760, -7.262430563887544821, -219.0449948566021021 ) ) ;
#20310=CARTESIAN_POINT ( 'NONE',  ( -17.75316132689678383, 25.03468689048078843, -222.1645193425721061 ) ) ;
#20311=CARTESIAN_POINT ( 'NONE',  ( -13.44328839870790837, -7.440897691988615392, -217.2299511873609106 ) ) ;
#20314=CARTESIAN_POINT ( 'NONE',  ( 16.54345861550681107, 19.37554510112122230, -218.2240151908141002 ) ) ;
#20316=CARTESIAN_POINT ( 'NONE',  ( 17.02763684969102798, -14.67205317233652195, -233.2001291093645818 ) ) ;
#20317=CARTESIAN_POINT ( 'NONE',  ( -15.15110768032078070, 3.517015312212880218, -219.5479300368539270 ) ) ;
#20318=CARTESIAN_POINT ( 'NONE',  ( -11.27928845652762213, 14.86256579634383002, -216.2427993537644966 ) ) ;
#20319=CARTESIAN_POINT ( 'NONE',  ( 27.50364976068844669, 3.973406265104437729, -228.8805639113908228 ) ) ;
#20320=CARTESIAN_POINT ( 'NONE',  ( -10.73077095140340376, -23.14408218571897891, -231.4559151628563995 ) ) ;
#20322=CARTESIAN_POINT ( 'NONE',  ( 15.52719855059926424, 1.633696074270991172, -221.7349885876216433 ) ) ;
#20324=CARTESIAN_POINT ( 'NONE',  ( 14.07866085257239419, -11.11077054092157645, -229.4139412770749971 ) ) ;
#20326=CARTESIAN_POINT ( 'NONE',  ( 12.96537118559348478, -2.410286924380323104, -226.7941485364539460 ) ) ;
#20329=CARTESIAN_POINT ( 'NONE',  ( 2.085064686336211892, 14.99578618537741548, -226.0985834012817861 ) ) ;
#20330=CARTESIAN_POINT ( 'NONE',  ( 6.065954396161110651, -11.55577711821250553, -228.1182208427093485 ) ) ;
#20331=CARTESIAN_POINT ( 'NONE',  ( 8.818493748348606331, -10.89961555176610375, -227.9481955143288303 ) ) ;
#20333=CARTESIAN_POINT ( 'NONE',  ( -21.66803296057637951, 19.04503900041684616, -222.6603677762044526 ) ) ;
#20334=CARTESIAN_POINT ( 'NONE',  ( 20.76808360334631232, 5.412616674732960931, -234.1222385626545304 ) ) ;
#20335=CARTESIAN_POINT ( 'NONE',  ( 15.33128967029630729, 6.504525012335983902, -229.0514072561169883 ) ) ;
#20337=CARTESIAN_POINT ( 'NONE',  ( -8.370291489323296474, -27.15533861588617981, -226.3382906634514597 ) ) ;
#20339=CARTESIAN_POINT ( 'NONE',  ( -12.13319425917249283, 4.024026700415168634, -229.5243363405849095 ) ) ;
#20340=CARTESIAN_POINT ( 'NONE',  ( 14.02309809840729393, 19.05079204846204277, -234.6885355850075143 ) ) ;
#20341=CARTESIAN_POINT ( 'NONE',  ( 10.22171596740309418, -15.66339630224980972, -229.7686180632486810 ) ) ;
#20342=CARTESIAN_POINT ( 'NONE',  ( 4.656903975822286768, 13.45000048768594780, -227.6722060245555497 ) ) ;
#20343=CARTESIAN_POINT ( 'NONE',  ( -23.49379658590067876, 11.46840048879614393, -217.2519070826072323 ) ) ;
#20345=CARTESIAN_POINT ( 'NONE',  ( 9.400341091271927851, 28.64465517894215196, -231.0823126271420165 ) ) ;
#20346=CARTESIAN_POINT ( 'NONE',  ( -17.00265675087485917, 7.324244386240115645, -218.5600005870616656 ) ) ;
#20348=CARTESIAN_POINT ( 'NONE',  ( -5.807479211365208727, 19.77444019604324410, -216.0778658752277863 ) ) ;
#20349=CARTESIAN_POINT ( 'NONE',  ( 16.91879448796214191, 0.8271603773820436212, -230.0510230802265710 ) ) ;
#20350=CARTESIAN_POINT ( 'NONE',  ( 2.098184199980985376, -13.29281380427311099, -222.1652846463370281 ) ) ;
#20351=CARTESIAN_POINT ( 'NONE',  ( 29.12543877365354916, -1.475122899492763873, -224.0746120762670444 ) ) ;
#20355=CARTESIAN_POINT ( 'NONE',  ( 22.03647168420945590, 0.3315607655625663064, -232.0572713672586644 ) ) ;
#20356=CARTESIAN_POINT ( 'NONE',  ( -10.33268794075157082, -17.24452578398873115, -232.5240627438851959 ) ) ;
#20360=CARTESIAN_POINT ( 'NONE',  ( 6.260833139380572732, -16.02228513277848876, -219.5457089733663736 ) ) ;
#20361=CARTESIAN_POINT ( 'NONE',  ( 10.59524789654300925, 9.532374763983630928, -223.0758647391057821 ) ) ;
#20362=CARTESIAN_POINT ( 'NONE',  ( -4.715783688792956063, 28.29821729825949816, -228.0423900005874600 ) ) ;
#20363=CARTESIAN_POINT ( 'NONE',  ( -4.813101935419741295, 13.68373293383429434, -229.7840611589179503 ) ) ;
#20365=CARTESIAN_POINT ( 'NONE',  ( -21.86011749369748713, -1.271659148212478385, -218.8339345395071689 ) ) ;
#20367=CARTESIAN_POINT ( 'NONE',  ( 15.12287735332712835, 21.03907941686458116, -231.7894952627153202 ) ) ;
#20368=CARTESIAN_POINT ( 'NONE',  ( 21.75737151495493649, -2.205713500382455283, -233.2756072794337285 ) ) ;
#20369=CARTESIAN_POINT ( 'NONE',  ( 20.92846067405557520, -2.114533307883533109, -233.2756072794335580 ) ) ;
#20371=CARTESIAN_POINT ( 'NONE',  ( -13.00301829581513857, -0.4478114825397079279, -224.9470972339195214 ) ) ;
#20372=CARTESIAN_POINT ( 'NONE',  ( 23.44028133050380802, 19.87677100428751231, -223.1503774981096342 ) ) ;
#20373=CARTESIAN_POINT ( 'NONE',  ( -23.77327857871830830, 11.53128597905896768, -221.0855018166512025 ) ) ;
#20374=CARTESIAN_POINT ( 'NONE',  ( 9.986779374595107228, 29.47523823012521049, -229.5287702428778687 ) ) ;
#20375=CARTESIAN_POINT ( 'NONE',  ( 23.64727379217503866, 9.907944788639682088, -232.0643337313508709 ) ) ;
#20376=CARTESIAN_POINT ( 'NONE',  ( -14.84991717770350661, -12.66914290363892270, -234.6513150936106626 ) ) ;
#20378=CARTESIAN_POINT ( 'NONE',  ( -12.60959727102843786, -12.64039607560028600, -218.2377899390859284 ) ) ;
#20379=CARTESIAN_POINT ( 'NONE',  ( -19.86079186537285324, -0.7838168488858909821, -215.1601656726509475 ) ) ;
#20380=CARTESIAN_POINT ( 'NONE',  ( 9.584731462935641488, -12.36622837314704348, -230.4796538097028531 ) ) ;
#20381=CARTESIAN_POINT ( 'NONE',  ( 0.2389779871941385414, 16.64595486589868045, -218.1658233406367629 ) ) ;
#20382=CARTESIAN_POINT ( 'NONE',  ( 30.29962988386644085, -7.724198041227372080, -225.2151988352147782 ) ) ;
#20383=CARTESIAN_POINT ( 'NONE',  ( -27.88251101234890328, -7.575382714962081820, -221.6715981084135478 ) ) ;
#20385=CARTESIAN_POINT ( 'NONE',  ( 10.14297843322460402, 14.69845403004500639, -219.2805000163441207 ) ) ;
#20387=CARTESIAN_POINT ( 'NONE',  ( -20.80338291456855870, 18.97067006663518995, -230.9007617602332516 ) ) ;
#20388=CARTESIAN_POINT ( 'NONE',  ( 13.17768061945195157, 6.810183613937965674, -219.8302315341053657 ) ) ;
#20389=CARTESIAN_POINT ( 'NONE',  ( 9.107417252317809186, 16.30291009569977234, -218.0131178633739921 ) ) ;
#20390=CARTESIAN_POINT ( 'NONE',  ( 6.608541902967795423, 16.43938546752961116, -220.2982508316308952 ) ) ;
#20391=CARTESIAN_POINT ( 'NONE',  ( 0.1236778125412633655, -13.14499247612405775, -221.8775184276742323 ) ) ;
#20392=CARTESIAN_POINT ( 'NONE',  ( -5.762781846020777365, 12.94769902409342777, -223.1319556069387886 ) ) ;
#20393=CARTESIAN_POINT ( 'NONE',  ( -13.98136146596813845, 3.850743984385103680, -228.7620665878280590 ) ) ;
#20395=CARTESIAN_POINT ( 'NONE',  ( 18.06016678184731461, 2.257982981100609354, -218.9983079406065940 ) ) ;
#20396=CARTESIAN_POINT ( 'NONE',  ( 3.489817674839083228, -23.52381883976217836, -233.5393804659674117 ) ) ;
#20397=CARTESIAN_POINT ( 'NONE',  ( -20.71192633727912380, 6.339941255257877550, -217.2401662359725094 ) ) ;
#20399=CARTESIAN_POINT ( 'NONE',  ( 3.219568897812384645, 28.82511222849302257, -221.5626884747494216 ) ) ;
#20400=CARTESIAN_POINT ( 'NONE',  ( -15.27057301462635408, -17.00912219741827514, -233.6288396447818627 ) ) ;
#20401=CARTESIAN_POINT ( 'NONE',  ( -27.32939371162572684, 5.861081283609568260, -224.9659309793921409 ) ) ;
#20403=CARTESIAN_POINT ( 'NONE',  ( 7.174260007897984792, 9.971262771497068300, -226.2872513832048469 ) ) ;
#20405=CARTESIAN_POINT ( 'NONE',  ( -4.104500432947460808, 15.73223271406093460, -218.0734292856946297 ) ) ;
#20406=CARTESIAN_POINT ( 'NONE',  ( 14.29170853205465264, -5.149528714972483989, -227.7869631675187350 ) ) ;
#20407=CARTESIAN_POINT ( 'NONE',  ( 19.19076252585518105, -11.68002947460017715, -233.4322573972352188 ) ) ;
#20409=CARTESIAN_POINT ( 'NONE',  ( 11.82943521288609823, 27.58963564415041247, -226.1180395413371400 ) ) ;
#20410=CARTESIAN_POINT ( 'NONE',  ( -21.59049550158629316, -10.60627468734379164, -215.2236992441505663 ) ) ;
#20411=CARTESIAN_POINT ( 'NONE',  ( -7.832594822155400927, -23.57318293858060088, -216.4298491688572028 ) ) ;
#20412=CARTESIAN_POINT ( 'NONE',  ( 11.31395536621571019, -8.070181239749643964, -225.0898076798974614 ) ) ;
#20413=CARTESIAN_POINT ( 'NONE',  ( -14.01966324001334385, 10.60695606488527964, -217.6333332521996340 ) ) ;
#20414=CARTESIAN_POINT ( 'NONE',  ( 10.64724148863252395, 12.28344647332184181, -223.6549461381946173 ) ) ;
#20415=CARTESIAN_POINT ( 'NONE',  ( -18.70100282803782576, 16.58357028540773115, -216.4425743468854080 ) ) ;
#20416=CARTESIAN_POINT ( 'NONE',  ( -10.76972226383489506, 9.682563335906554158, -229.2555443445334333 ) ) ;
#20417=CARTESIAN_POINT ( 'NONE',  ( -15.91852731338648752, -4.625608912867816613, -229.2691880628015895 ) ) ;
#20419=CARTESIAN_POINT ( 'NONE',  ( -14.94618804342693075, 22.09718979644185666, -219.6454806548149463 ) ) ;
#20420=CARTESIAN_POINT ( 'NONE',  ( 17.29648694364601980, 10.20782262162153842, -233.8400727604031317 ) ) ;
#20421=CARTESIAN_POINT ( 'NONE',  ( 13.79814099039094089, 16.09927043668092850, -214.6489469124405502 ) ) ;
#20423=CARTESIAN_POINT ( 'NONE',  ( 23.27685575300125720, -16.81362096763192326, -220.1650456318757563 ) ) ;
#20427=CARTESIAN_POINT ( 'NONE',  ( -11.33137429837660193, 27.25022425932026238, -230.1650924901870212 ) ) ;
#20428=CARTESIAN_POINT ( 'NONE',  ( -28.75820353979175081, -10.31764292692039753, -230.8958203355234389 ) ) ;
#20430=CARTESIAN_POINT ( 'NONE',  ( 24.58316096239279602, 5.861425670879941485, -231.3104446318280623 ) ) ;
#20432=CARTESIAN_POINT ( 'NONE',  ( 19.68037530048075112, -17.97179847169212508, -231.8517058357153076 ) ) ;
#20433=CARTESIAN_POINT ( 'NONE',  ( -17.79285498209129202, 9.187865686019035749, -216.3798185811636756 ) ) ;
#20434=CARTESIAN_POINT ( 'NONE',  ( 19.87150736056128864, 8.436445599727830924, -233.0166429845654932 ) ) ;
#20435=CARTESIAN_POINT ( 'NONE',  ( -12.58820391453271093, -22.27128923838312247, -218.3899974299303324 ) ) ;
#20439=CARTESIAN_POINT ( 'NONE',  ( 15.27128302093890255, -22.10320814337061535, -229.9052109820655119 ) ) ;
#20440=CARTESIAN_POINT ( 'NONE',  ( 12.90388673151985977, -2.516900468902075083, -226.6432736121070661 ) ) ;
#20442=CARTESIAN_POINT ( 'NONE',  ( 12.91443243054181700, 13.28840485332751875, -229.6651346406987955 ) ) ;
#20443=CARTESIAN_POINT ( 'NONE',  ( 5.066530254613678785, 15.76189963344335254, -222.1234037505291781 ) ) ;
#20444=CARTESIAN_POINT ( 'NONE',  ( 8.679960083554519201, -14.04048791834972398, -217.5462328905347249 ) ) ;
#20445=CARTESIAN_POINT ( 'NONE',  ( 17.02763684969102798, -14.67205317233652195, -233.2001291093645818 ) ) ;
#20447=CARTESIAN_POINT ( 'NONE',  ( -7.464187997994982560, 14.20693289415472016, -228.8865298551900764 ) ) ;
#20448=CARTESIAN_POINT ( 'NONE',  ( -18.42638600874552424, 7.060399206045774534, -230.3991437614443214 ) ) ;
#20449=CARTESIAN_POINT ( 'NONE',  ( 14.18323607655884722, 3.286047475533308226, -222.8710065128477140 ) ) ;
#20451=CARTESIAN_POINT ( 'NONE',  ( -6.479026444546563290, -23.11309618162032820, -231.4158670874050756 ) ) ;
#20455=CARTESIAN_POINT ( 'NONE',  ( 3.490829917597003895, 11.40812925993816229, -222.8973702487053004 ) ) ;
#20456=CARTESIAN_POINT ( 'NONE',  ( 10.85678324124089755, -13.97331853324622131, -221.1336851750754420 ) ) ;
#20457=CARTESIAN_POINT ( 'NONE',  ( 5.248230734842167955, 23.54336384919183445, -216.8914391693808739 ) ) ;
#20458=CARTESIAN_POINT ( 'NONE',  ( -14.29986196492902550, 0.06805469746732484282, -227.4167624117703213 ) ) ;
#20459=CARTESIAN_POINT ( 'NONE',  ( 9.168912942254459963, 16.03578711007639157, -234.6923200900793347 ) ) ;
#20460=CARTESIAN_POINT ( 'NONE',  ( -14.58084844870496966, 13.85720943031455832, -233.3219724312919254 ) ) ;
#20461=CARTESIAN_POINT ( 'NONE',  ( -3.855805549595750392, 26.68244055262801950, -232.4569730455296508 ) ) ;
#20462=CARTESIAN_POINT ( 'NONE',  ( 22.00000000000000711, 0.000000000000000000, -233.0000000000000284 ) ) ;
#20463=CARTESIAN_POINT ( 'NONE',  ( 1.292981098121811279, -26.53499626907933262, -232.9055005154886828 ) ) ;
#20464=CARTESIAN_POINT ( 'NONE',  ( 16.50235023187294203, -3.000022380394500310, -230.0447763498268614 ) ) ;
#20466=CARTESIAN_POINT ( 'NONE',  ( 27.75679124201660741, 4.911524026080384075, -221.4430403652340829 ) ) ;
#20467=CARTESIAN_POINT ( 'NONE',  ( -15.95469971785872332, -24.72796590591627464, -225.3946449442874211 ) ) ;
#20469=CARTESIAN_POINT ( 'NONE',  ( 6.755953262402430326, -28.44658494672641424, -224.7309905328439754 ) ) ;
#20470=CARTESIAN_POINT ( 'NONE',  ( -18.05576253097465766, 2.935622250037499104, -232.1557308718028594 ) ) ;
#20471=CARTESIAN_POINT ( 'NONE',  ( -3.996294969088721505, 28.80481464818193515, -222.8623509149411746 ) ) ;
#20472=CARTESIAN_POINT ( 'NONE',  ( -22.56222084847001597, 18.89892770556097901, -231.8972396388394088 ) ) ;
#20474=CARTESIAN_POINT ( 'NONE',  ( -26.74184309910812374, -3.166857098814535032, -228.4517881524372456 ) ) ;
#20476=CARTESIAN_POINT ( 'NONE',  ( 11.57669841200422134, 10.63052136557218574, -228.9489978335593889 ) ) ;
#20478=CARTESIAN_POINT ( 'NONE',  ( -24.05551141223569545, 2.266836731622281498, -230.7594878221277384 ) ) ;
#20479=CARTESIAN_POINT ( 'NONE',  ( -24.53276002501160136, 17.12571705644413811, -226.2419685911331442 ) ) ;
#20480=CARTESIAN_POINT ( 'NONE',  ( -3.400000000000003908, 0.000000000000000000, -227.9999999999999716 ) ) ;
#20481=CARTESIAN_POINT ( 'NONE',  ( 5.833753951408669813, 12.47745132051510453, -226.2508980627489450 ) ) ;
#20482=CARTESIAN_POINT ( 'NONE',  ( -15.82068653568960137, 8.372322471091806051, -220.7139663195713979 ) ) ;
#20483=CARTESIAN_POINT ( 'NONE',  ( 7.283976506941576723, 24.82246917020504284, -234.3244871078919402 ) ) ;
#20484=CARTESIAN_POINT ( 'NONE',  ( 18.78616100366561881, 3.045752412654093355, -231.5393376370170699 ) ) ;
#20485=CARTESIAN_POINT ( 'NONE',  ( -9.899145469884247817, -15.57979392722981693, -233.4163339629578786 ) ) ;
#20487=CARTESIAN_POINT ( 'NONE',  ( -13.55429797312971374, -24.97278848321653300, -221.1627755146857908 ) ) ;
#20488=CARTESIAN_POINT ( 'NONE',  ( -14.00980274651940682, 20.05588230486321066, -234.2453272803952586 ) ) ;
#20489=CARTESIAN_POINT ( 'NONE',  ( 1.799766247726228174, -14.75051420185460849, -230.6199496058247291 ) ) ;
#20490=CARTESIAN_POINT ( 'NONE',  ( -7.429838964355703901, 14.87322129099639234, -232.2632863647814077 ) ) ;
#20491=CARTESIAN_POINT ( 'NONE',  ( 25.51806929334465934, -15.64550748320022144, -218.8629450469393589 ) ) ;
#20493=CARTESIAN_POINT ( 'NONE',  ( -15.15819830826754355, -2.370657588173597841, -221.8013720140894236 ) ) ;
#20494=CARTESIAN_POINT ( 'NONE',  ( 11.17884645811568944, 10.10284797925214662, -221.0856722371208036 ) ) ;
#20496=CARTESIAN_POINT ( 'NONE',  ( -6.901278853520646628, 15.41233971300566807, -220.5972764307651346 ) ) ;
#20497=CARTESIAN_POINT ( 'NONE',  ( 26.72610819325501907, 14.97064052581051108, -224.6384473985499426 ) ) ;
#20498=CARTESIAN_POINT ( 'NONE',  ( 13.03557269046774714, 7.519834803053426775, -226.9490612297269081 ) ) ;
#20499=CARTESIAN_POINT ( 'NONE',  ( 23.08329078023534109, 11.96623404944238978, -217.1428499060670845 ) ) ;
#20500=CARTESIAN_POINT ( 'NONE',  ( 0.2060740257213805326, -13.46849591350090947, -221.0879548523055860 ) ) ;
#20501=CARTESIAN_POINT ( 'NONE',  ( -10.07004052286948337, 22.64471483900350179, -217.4645417110143626 ) ) ;
#20502=CARTESIAN_POINT ( 'NONE',  ( 27.75679124201660741, 4.911524026080384075, -221.4430403652340829 ) ) ;
#20503=CARTESIAN_POINT ( 'NONE',  ( 7.434033643350927534, -13.76500825175950027, -228.7793665183827159 ) ) ;
#20504=CARTESIAN_POINT ( 'NONE',  ( -13.93825237094548619, 9.044872709574327985, -220.1275804576921757 ) ) ;
#20505=CARTESIAN_POINT ( 'NONE',  ( 9.527502190795640757, 23.55559004943647139, -217.4101659741468211 ) ) ;
#20507=CARTESIAN_POINT ( 'NONE',  ( -23.84209965496292227, -7.976777114481962805, -232.1458837748831456 ) ) ;
#20509=CARTESIAN_POINT ( 'NONE',  ( -21.47149190714903710, 3.672831083387290363, -231.0833634068433469 ) ) ;
#20510=CARTESIAN_POINT ( 'NONE',  ( 10.61539692146153691, 8.157890242340682718, -227.5705019877536301 ) ) ;
#20511=EDGE_LOOP ( 'NONE', ( #8888, #15771, #5895, #17674 ) ) ;
#20512=CARTESIAN_POINT ( 'NONE',  ( 17.19674704922021391, 23.07334190050143974, -228.8256488842130238 ) ) ;
#20513=CARTESIAN_POINT ( 'NONE',  ( 20.48752708986941329, -13.44209471493726937, -230.9762584513030106 ) ) ;
#20514=CARTESIAN_POINT ( 'NONE',  ( 11.81564506561547390, -6.597897255275705142, -225.1493936678799628 ) ) ;
#20515=CARTESIAN_POINT ( 'NONE',  ( 15.85665641241444668, 18.24713744004561988, -217.7195292979064902 ) ) ;
#20516=CARTESIAN_POINT ( 'NONE',  ( -26.70887854271809658, -5.532318215328999145, -217.2738835169348306 ) ) ;
#20517=CARTESIAN_POINT ( 'NONE',  ( -8.257247207528708444, -26.39349301559143512, -217.9383130379005138 ) ) ;
#20518=CARTESIAN_POINT ( 'NONE',  ( 5.569356713096689226, -12.06902110579006226, -223.1407905962607003 ) ) ;
#20519=CARTESIAN_POINT ( 'NONE',  ( -17.07051451008491938, 15.19890664381897949, -233.6014043774825666 ) ) ;
#20521=CARTESIAN_POINT ( 'NONE',  ( 16.53859560591101641, 22.24348416270211359, -223.7250258089275974 ) ) ;
#20522=CARTESIAN_POINT ( 'NONE',  ( -24.24202834850560606, 19.05981756344202438, -226.6980666352953335 ) ) ;
#20523=CARTESIAN_POINT ( 'NONE',  ( -11.36937006530106586, 5.486019310970209339, -224.0742584078730033 ) ) ;
#20524=CARTESIAN_POINT ( 'NONE',  ( 30.05917755080113096, -2.930701380670650114, -221.3976229872638726 ) ) ;
#20527=CARTESIAN_POINT ( 'NONE',  ( -3.996294969088721505, 28.80481464818193515, -222.8623509149411746 ) ) ;
#20528=CARTESIAN_POINT ( 'NONE',  ( 29.11492790716816614, 6.132849117128307270, -229.8316941169402412 ) ) ;
#20529=CARTESIAN_POINT ( 'NONE',  ( 8.681721411120292942, 8.442847255497570202, -228.0516816418615065 ) ) ;
#20530=CARTESIAN_POINT ( 'NONE',  ( 14.46917091355089902, -8.493370822347547033, -231.7163745456035997 ) ) ;
#20532=ORIENTED_EDGE ( 'NONE', *, *, #16914, .F. ) ;
#20533=CARTESIAN_POINT ( 'NONE',  ( -10.24288955603410933, 28.30762631303078791, -220.8855665231519083 ) ) ;
#20534=CARTESIAN_POINT ( 'NONE',  ( -13.37406041957185110, -11.77244451953823834, -233.9958171493936732 ) ) ;
#20537=CARTESIAN_POINT ( 'NONE',  ( 18.04365516558436866, 6.721233635139160612, -218.4376093631473168 ) ) ;
#20539=CARTESIAN_POINT ( 'NONE',  ( 12.70477135646371281, -9.814387909761604689, -230.3443492180780652 ) ) ;
#20541=CARTESIAN_POINT ( 'NONE',  ( -14.70651859537745487, 4.211702956367679107, -230.0357207626005334 ) ) ;
#20543=CARTESIAN_POINT ( 'NONE',  ( -16.74550766701807447, 3.787526820511904813, -217.9802846976114381 ) ) ;
#20544=CARTESIAN_POINT ( 'NONE',  ( -7.086613078029399659, -28.17108726511417771, -223.6412629831645233 ) ) ;
#20549=CARTESIAN_POINT ( 'NONE',  ( 17.83206265427627457, -15.38023228143295640, -231.0294926223175480 ) ) ;
#20552=CARTESIAN_POINT ( 'NONE',  ( 17.35243190875273811, 16.67741344734974263, -230.5744436858935558 ) ) ;
#20555=CARTESIAN_POINT ( 'NONE',  ( 5.791579991237209235, 15.48299465423324861, -228.0203551130359472 ) ) ;
#20556=CARTESIAN_POINT ( 'NONE',  ( 6.644147376113458847, -12.60537238651543923, -230.3381876225809037 ) ) ;
#20557=CARTESIAN_POINT ( 'NONE',  ( 5.569356713096689226, -12.06902110579006226, -223.1407905962607003 ) ) ;
#20559=CARTESIAN_POINT ( 'NONE',  ( -9.233762381136051189, 19.18161952504991419, -232.0796851897838451 ) ) ;
#20560=CARTESIAN_POINT ( 'NONE',  ( -25.17056316833229701, 11.10725809642625705, -227.0225660235207386 ) ) ;
#20561=CARTESIAN_POINT ( 'NONE',  ( 20.41968681625622040, 10.18377600976054076, -218.1989382652844256 ) ) ;
#20563=CARTESIAN_POINT ( 'NONE',  ( -3.088421015035204498, -25.33386621341791667, -218.8172537214380498 ) ) ;
#20566=CARTESIAN_POINT ( 'NONE',  ( 27.08994772491946890, 9.675875910685000747, -221.3471992134593336 ) ) ;
#20567=CARTESIAN_POINT ( 'NONE',  ( 11.82295278175540787, -22.41907685134884076, -220.1071383070178342 ) ) ;
#20568=CARTESIAN_POINT ( 'NONE',  ( 11.33210854356620523, 22.81476816607802149, -217.8536224460118262 ) ) ;
#20569=CARTESIAN_POINT ( 'NONE',  ( -6.855867220396999251, 12.17758473459128332, -220.6375607554995213 ) ) ;
#20571=CARTESIAN_POINT ( 'NONE',  ( 28.41961022423218353, 10.76616830294286409, -220.2698681100053193 ) ) ;
#20572=CARTESIAN_POINT ( 'NONE',  ( -4.620781219515533778, 16.99182040716223696, -217.1278208835672672 ) ) ;
#20574=CARTESIAN_POINT ( 'NONE',  ( 8.257114973007913861, -25.39836461225790742, -232.6217252414676295 ) ) ;
#20575=CARTESIAN_POINT ( 'NONE',  ( 26.16486877413895584, -0.2437668799822691745, -230.8325409000573814 ) ) ;
#20577=CARTESIAN_POINT ( 'NONE',  ( -15.46216926290318305, -2.495270579625169738, -221.2150947962298631 ) ) ;
#20578=CARTESIAN_POINT ( 'NONE',  ( 15.05360126642391450, 1.481754003466396963, -222.9454997252120734 ) ) ;
#20579=CARTESIAN_POINT ( 'NONE',  ( -17.12341639776428437, -14.09197680242149886, -218.6048700820433339 ) ) ;
#20583=CARTESIAN_POINT ( 'NONE',  ( 13.38323588254664642, -24.59169381177348157, -229.6955247737395780 ) ) ;
#20584=CARTESIAN_POINT ( 'NONE',  ( 29.01678366425524658, 8.126504218505314014, -229.6975090854573125 ) ) ;
#20585=CARTESIAN_POINT ( 'NONE',  ( 3.291078285693179950, 23.55624334554876498, -217.3208248278388623 ) ) ;
#20586=CARTESIAN_POINT ( 'NONE',  ( -8.716816145717144693, 12.22834664005217675, -231.7124508691059646 ) ) ;
#20588=CARTESIAN_POINT ( 'NONE',  ( 25.69869100782391413, -6.466588899411362057, -234.2905747065633193 ) ) ;
#20590=CARTESIAN_POINT ( 'NONE',  ( 12.23063869552301242, 12.84118223717021934, -218.8273164334868284 ) ) ;
#20591=CARTESIAN_POINT ( 'NONE',  ( -23.43012680803641956, 15.46310457140252304, -230.0052977649806962 ) ) ;
#20592=CARTESIAN_POINT ( 'NONE',  ( -23.43012680803641956, 15.46310457140252304, -230.0052977649806962 ) ) ;
#20593=CARTESIAN_POINT ( 'NONE',  ( -8.652743106909156268, -19.89692808811530966, -232.3032230114403376 ) ) ;
#20595=CARTESIAN_POINT ( 'NONE',  ( 25.38325563848796662, 11.05100313887457553, -217.8685524735130628 ) ) ;
#20596=CARTESIAN_POINT ( 'NONE',  ( -16.37512411505367282, 2.406627362596846620, -227.7341547288202719 ) ) ;
#20598=CARTESIAN_POINT ( 'NONE',  ( 10.85325209735074559, 11.82487774067193342, -216.5214842375702062 ) ) ;
#20599=CARTESIAN_POINT ( 'NONE',  ( 19.66580438618080251, 15.18147523775131624, -233.5153994334876586 ) ) ;
#20600=CARTESIAN_POINT ( 'NONE',  ( -5.045022908720540045, -16.91549468467126616, -232.0765493255083243 ) ) ;
#20602=CARTESIAN_POINT ( 'NONE',  ( -5.249799428260828904, -14.16826377401270065, -226.9124264195330056 ) ) ;
#20604=CARTESIAN_POINT ( 'NONE',  ( -11.87391433320165746, 8.920676825367966245, -232.2044275666449096 ) ) ;
#20605=CARTESIAN_POINT ( 'NONE',  ( 15.60497028854143764, -26.39208911975253002, -225.8550158017044112 ) ) ;
#20606=CARTESIAN_POINT ( 'NONE',  ( -3.326157069579807946, 13.92020081821418565, -220.5733722327383930 ) ) ;
#20607=CARTESIAN_POINT ( 'NONE',  ( 12.64197975508134597, -4.295353707277522304, -228.6481500018833799 ) ) ;
#20608=CARTESIAN_POINT ( 'NONE',  ( -25.61235545225478560, -15.41032726095661509, -226.9890212492312855 ) ) ;
#20609=CARTESIAN_POINT ( 'NONE',  ( -27.52457542293397097, 5.447957517019466067, -230.2717933641555135 ) ) ;
#20611=CARTESIAN_POINT ( 'NONE',  ( -3.389634396460917465, 16.42708991135657115, -221.9057377485790994 ) ) ;
#20612=CARTESIAN_POINT ( 'NONE',  ( -20.45797657813638182, 1.164962349958370336, -217.1306074022350572 ) ) ;
#20613=CARTESIAN_POINT ( 'NONE',  ( 8.689059922489732912, 15.18271246186214363, -218.7354841152034908 ) ) ;
#20614=CARTESIAN_POINT ( 'NONE',  ( 18.13412043358480474, 12.55378873098427128, -233.2186159706515696 ) ) ;
#20615=CARTESIAN_POINT ( 'NONE',  ( 5.917072789534883803, -21.18442853552521754, -235.1867574136372525 ) ) ;
#20617=CARTESIAN_POINT ( 'NONE',  ( 19.07698357483942786, 25.86742807064150895, -222.6991278896559834 ) ) ;
#20621=CARTESIAN_POINT ( 'NONE',  ( 9.923594862512629788, -27.47695806889172943, -228.4416101659923015 ) ) ;
#20622=CARTESIAN_POINT ( 'NONE',  ( -14.94618804342693075, 22.09718979644185666, -219.6454806548149463 ) ) ;
#20623=CARTESIAN_POINT ( 'NONE',  ( 3.291078285693179950, 23.55624334554876498, -217.3208248278388623 ) ) ;
#20624=CARTESIAN_POINT ( 'NONE',  ( -13.88883449434014672, -11.15328429608096172, -217.8357414694029046 ) ) ;
#20625=CARTESIAN_POINT ( 'NONE',  ( -15.32935061426341861, 5.146212415319166844, -225.5669090095357774 ) ) ;
#20626=CARTESIAN_POINT ( 'NONE',  ( 12.99334571784053338, 27.47142594410712846, -219.5003755906066658 ) ) ;
#20627=CARTESIAN_POINT ( 'NONE',  ( 7.743212835174657194, 11.90778931056080481, -226.0491028376908105 ) ) ;
#20628=CARTESIAN_POINT ( 'NONE',  ( 23.44453178257692727, -8.594063734448958769, -231.6993511358095361 ) ) ;
#20630=CARTESIAN_POINT ( 'NONE',  ( 13.37423534347618670, -3.100899090186935325, -222.2483675785374260 ) ) ;
#20634=CARTESIAN_POINT ( 'NONE',  ( 8.329997790135040603, 12.51216704542961899, -228.7022893680961602 ) ) ;
#20635=CARTESIAN_POINT ( 'NONE',  ( -19.19980083083115474, -2.588899828715947038, -216.2953230342753557 ) ) ;
#20636=CARTESIAN_POINT ( 'NONE',  ( -1.177898122437396333, -26.14463525305933445, -216.8677949074964033 ) ) ;
#20637=CARTESIAN_POINT ( 'NONE',  ( 18.00123703865980218, -15.82960056198189491, -233.0014896689109776 ) ) ;
#20638=CARTESIAN_POINT ( 'NONE',  ( -0.6272116608575281083, 20.18031380156121202, -219.3960054794027030 ) ) ;
#20640=CARTESIAN_POINT ( 'NONE',  ( 14.40184562439531213, 6.414772937171507650, -227.4651811604036595 ) ) ;
#20641=CARTESIAN_POINT ( 'NONE',  ( -11.49049084071896409, 11.06834963248926940, -218.3354249205727058 ) ) ;
#20642=CARTESIAN_POINT ( 'NONE',  ( -5.600903697806950632, 21.62055466701630735, -218.6671277943675307 ) ) ;
#20643=CARTESIAN_POINT ( 'NONE',  ( 14.79879825009101069, -3.130997509566451953, -219.4569190381675696 ) ) ;
#20646=CARTESIAN_POINT ( 'NONE',  ( -0.3197916200495275474, 16.38897215927557482, -229.9606066735827028 ) ) ;
#20647=CARTESIAN_POINT ( 'NONE',  ( -16.03353370602922467, 4.897644413504528060, -222.5335369890782999 ) ) ;
#20648=CARTESIAN_POINT ( 'NONE',  ( 14.82579616070250417, 22.96152595385638762, -233.8920860146931489 ) ) ;
#20649=CARTESIAN_POINT ( 'NONE',  ( 14.68951511424354273, -18.85605729411972575, -217.5026406474102885 ) ) ;
#20652=CARTESIAN_POINT ( 'NONE',  ( 1.217121169770782663, 15.31158828575123110, -230.6845728599757308 ) ) ;
#20653=CARTESIAN_POINT ( 'NONE',  ( -10.04615645102154886, -9.695712423306433791, -230.4834384258168996 ) ) ;
#20655=CARTESIAN_POINT ( 'NONE',  ( 16.00819137755116373, 4.595691552992191120, -229.5669508871464757 ) ) ;
#20656=CARTESIAN_POINT ( 'NONE',  ( -16.63766460830045091, 5.158675778507696208, -232.1659425527909093 ) ) ;
#20657=CARTESIAN_POINT ( 'NONE',  ( 21.30961698559626427, -20.48616475849644303, -228.5322376518520002 ) ) ;
#20659=CARTESIAN_POINT ( 'NONE',  ( -22.47200958260654957, 4.697452857301940732, -216.5879371680706242 ) ) ;
#20660=CARTESIAN_POINT ( 'NONE',  ( -29.95012366401462955, 4.746560250930182967, -224.6954343660969471 ) ) ;
#20661=CARTESIAN_POINT ( 'NONE',  ( -6.776147227169700749, -16.68571135823561846, -231.0772860317820232 ) ) ;
#20664=CARTESIAN_POINT ( 'NONE',  ( -25.80904414196669450, 12.19501778665756220, -219.1732313092283846 ) ) ;
#20665=CARTESIAN_POINT ( 'NONE',  ( 10.87273020620571629, -12.78363999705779186, -228.8712466752294858 ) ) ;
#20666=CARTESIAN_POINT ( 'NONE',  ( 12.85121247375660047, -2.863977387274604602, -224.0868061481347127 ) ) ;
#20668=CARTESIAN_POINT ( 'NONE',  ( 5.909674498212842408, 15.76475534640655773, -228.4922217450045139 ) ) ;
#20669=CARTESIAN_POINT ( 'NONE',  ( -13.58389614404818069, 15.11490620317918676, -215.3922994348461941 ) ) ;
#20670=CARTESIAN_POINT ( 'NONE',  ( 12.94599882983645145, 15.82237817288049442, -219.3332542656393116 ) ) ;
#20671=CARTESIAN_POINT ( 'NONE',  ( -4.572289063834428013, -16.67516242687949557, -229.9678395161569142 ) ) ;
#20673=CARTESIAN_POINT ( 'NONE',  ( 30.13983206778957324, -7.413543662652124944, -226.8644184361555745 ) ) ;
#20676=CARTESIAN_POINT ( 'NONE',  ( -17.99720854823001659, 13.97888873227035056, -232.2992184661552244 ) ) ;
#20677=CARTESIAN_POINT ( 'NONE',  ( -26.04932551096112192, 5.001193774903864409, -228.9498367494266802 ) ) ;
#20678=CARTESIAN_POINT ( 'NONE',  ( -11.36937006530106586, 5.486019310970209339, -224.0742584078730033 ) ) ;
#20679=CARTESIAN_POINT ( 'NONE',  ( -3.968800477764047319, -14.91200208314756104, -226.8245746385127575 ) ) ;
#20681=ORIENTED_EDGE ( 'NONE', *, *, #8464, .F. ) ;
#20682=CARTESIAN_POINT ( 'NONE',  ( 19.66580438618080251, 15.18147523775131624, -233.5153994334876586 ) ) ;
#20683=CARTESIAN_POINT ( 'NONE',  ( 7.956221944547102964, -16.14435353399512252, -220.6073666753051441 ) ) ;
#20684=CARTESIAN_POINT ( 'NONE',  ( 7.639528166734322667, 11.92751229241157596, -224.6077814063189635 ) ) ;
#20685=CARTESIAN_POINT ( 'NONE',  ( -9.443239614166923701, 9.388015667058336788, -222.3195230688234290 ) ) ;
#20688=CARTESIAN_POINT ( 'NONE',  ( 19.49137065790598555, 9.165486118354671419, -234.8706749352814995 ) ) ;
#20691=CARTESIAN_POINT ( 'NONE',  ( 9.333020543840051531, 16.91085096921651143, -217.7308990335875762 ) ) ;
#20694=CARTESIAN_POINT ( 'NONE',  ( -1.308474130992312023, -24.58654860180777391, -216.2430112183533026 ) ) ;
#20695=CARTESIAN_POINT ( 'NONE',  ( 19.06212547406409641, -9.287000003594721775, -232.7453815625877667 ) ) ;
#20698=CARTESIAN_POINT ( 'NONE',  ( 25.69300549816939494, 5.947472783069708946, -230.6131061331718115 ) ) ;
#20699=CARTESIAN_POINT ( 'NONE',  ( -14.94274040728286046, -6.247332224397157852, -226.1562440284360491 ) ) ;
#20700=CARTESIAN_POINT ( 'NONE',  ( -22.10934047915427314, 0.9940043559354312386, -216.9999999999999716 ) ) ;
#20701=CARTESIAN_POINT ( 'NONE',  ( 2.471164685565028662, 14.01327037412690935, -223.4905256513065410 ) ) ;
#20702=CARTESIAN_POINT ( 'NONE',  ( 0.07890756785233743464, 25.14108539708653822, -218.4152285319504756 ) ) ;
#20704=CARTESIAN_POINT ( 'NONE',  ( 25.75143957690053753, -9.476334075918805055, -216.1442976756887617 ) ) ;
#20706=CARTESIAN_POINT ( 'NONE',  ( 18.29617186523616468, 23.20920553663278341, -223.4372550713720216 ) ) ;
#20707=CARTESIAN_POINT ( 'NONE',  ( -15.46752262371512820, 15.15798787883389487, -233.5981584775992701 ) ) ;
#20708=CARTESIAN_POINT ( 'NONE',  ( -26.88784739727922357, 10.07520213145270915, -227.1866063047054922 ) ) ;
#20709=CARTESIAN_POINT ( 'NONE',  ( -8.465333986790207987, -12.59497810381903982, -228.1424919783533198 ) ) ;
#20711=CARTESIAN_POINT ( 'NONE',  ( 24.81079154715000357, 3.171651085595392772, -216.4177249688571578 ) ) ;
#20712=CARTESIAN_POINT ( 'NONE',  ( -8.985448925281199095, 11.82743561134668475, -224.1067108988273162 ) ) ;
#20713=CARTESIAN_POINT ( 'NONE',  ( 15.89102655998366664, 24.10108298038447572, -232.7733025413564008 ) ) ;
#20714=CARTESIAN_POINT ( 'NONE',  ( 25.40954707198727647, 2.077273811637330159, -219.3610170479527426 ) ) ;
#20715=CARTESIAN_POINT ( 'NONE',  ( -32.05942529185317369, -1.254016050025921425, -226.3193970476597485 ) ) ;
#20716=CARTESIAN_POINT ( 'NONE',  ( -13.08346052978740914, -7.620079078745922274, -220.3923444982454498 ) ) ;
#20717=CARTESIAN_POINT ( 'NONE',  ( -9.491065840222427497, 13.31995980477872266, -232.8537120564120073 ) ) ;
#20718=CARTESIAN_POINT ( 'NONE',  ( 1.127544764349826867, -27.89617517048659323, -231.9509945439240823 ) ) ;
#20719=CARTESIAN_POINT ( 'NONE',  ( -3.673551555920188783, 29.81207051619892923, -228.8770490300152005 ) ) ;
#20720=CARTESIAN_POINT ( 'NONE',  ( 19.73224149047082321, -2.635265996080750295, -233.5133592171236501 ) ) ;
#20721=CARTESIAN_POINT ( 'NONE',  ( -29.27492217116574480, -1.185422171198730501, -224.8132346143397342 ) ) ;
#20722=CARTESIAN_POINT ( 'NONE',  ( -18.05576253097465766, 2.935622250037499104, -232.1557308718028594 ) ) ;
#20725=CARTESIAN_POINT ( 'NONE',  ( -0.2748333203896175525, 17.57683079704640505, -221.1444293135629948 ) ) ;
#20726=CARTESIAN_POINT ( 'NONE',  ( 15.14536540539411114, 2.907144070186200580, -217.8738854795238922 ) ) ;
#20727=CARTESIAN_POINT ( 'NONE',  ( 19.72515656911863147, 14.02277373989196541, -218.0718040828188009 ) ) ;
#20728=CARTESIAN_POINT ( 'NONE',  ( 26.72610819325501907, 14.97064052581051108, -224.6384473985499426 ) ) ;
#20729=CARTESIAN_POINT ( 'NONE',  ( -1.925327751674894339, -31.30071588347811584, -225.0681195224254623 ) ) ;
#20730=CARTESIAN_POINT ( 'NONE',  ( 3.711349367426693746, 16.84755988915346236, -233.7359972593521888 ) ) ;
#20732=CARTESIAN_POINT ( 'NONE',  ( -12.81114484120449504, -26.81657559919244349, -231.7433950434849805 ) ) ;
#20733=CARTESIAN_POINT ( 'NONE',  ( -10.70754874174748039, 23.84972878377777405, -230.7991598016655246 ) ) ;
#20734=CARTESIAN_POINT ( 'NONE',  ( 17.24952650401854370, 25.19767938110938843, -224.5319471861414797 ) ) ;
#20735=CARTESIAN_POINT ( 'NONE',  ( -18.34948365288241590, -1.907751280579004893, -231.5848060246952116 ) ) ;
#20736=CARTESIAN_POINT ( 'NONE',  ( -14.01525440049806193, 8.239250543314939890, -226.5804714421811070 ) ) ;
#20737=CARTESIAN_POINT ( 'NONE',  ( -22.70558257617108922, 14.65737936663030538, -230.9775454010380997 ) ) ;
#20738=CARTESIAN_POINT ( 'NONE',  ( 21.14328650935969023, 6.072767611243683916, -217.6422864096696514 ) ) ;
#20740=CARTESIAN_POINT ( 'NONE',  ( 17.60676319847677007, 21.31475060840986302, -219.8266339603936785 ) ) ;
#20741=CARTESIAN_POINT ( 'NONE',  ( 13.35408364068459619, -22.25650632745845314, -229.3239852056058226 ) ) ;
#20743=CARTESIAN_POINT ( 'NONE',  ( 24.05238142633148968, -17.07083877791421500, -221.4615098029387070 ) ) ;
#20744=CARTESIAN_POINT ( 'NONE',  ( 1.030230143518703345, 18.27887886751213387, -229.5791973322770616 ) ) ;
#20746=CARTESIAN_POINT ( 'NONE',  ( 14.68783945462866924, 9.535285537539673228, -219.4694094309942045 ) ) ;
#20747=CARTESIAN_POINT ( 'NONE',  ( -23.03165807712271373, -11.67016847039487892, -215.7330867557714384 ) ) ;
#20748=CARTESIAN_POINT ( 'NONE',  ( -5.420780812268581883, -12.08122409751860360, -226.5143039284326392 ) ) ;
#20749=CARTESIAN_POINT ( 'NONE',  ( 1.752757082432757185, -17.15725705531007250, -232.7539178101738742 ) ) ;
#20750=CARTESIAN_POINT ( 'NONE',  ( -2.693916085894628942, 18.86613858709357672, -230.4911878356387263 ) ) ;
#20752=CARTESIAN_POINT ( 'NONE',  ( 27.66944030902029539, 6.857614156517904291, -220.9860880211026313 ) ) ;
#20753=CARTESIAN_POINT ( 'NONE',  ( -20.54164754914381064, 7.122791156791981493, -233.5720402887671980 ) ) ;
#20754=CARTESIAN_POINT ( 'NONE',  ( -8.316066124693966444, 26.67103469786491843, -222.2304303634109885 ) ) ;
#20755=CARTESIAN_POINT ( 'NONE',  ( 3.367418898937407867, 27.20023797116225595, -219.3349021808245709 ) ) ;
#20756=CARTESIAN_POINT ( 'NONE',  ( 12.93042813863272755, 0.4488092930645843914, -225.5263188864764174 ) ) ;
#20757=CARTESIAN_POINT ( 'NONE',  ( 17.65694480011521250, 15.62497337860048674, -235.2008064134603273 ) ) ;
#20758=CARTESIAN_POINT ( 'NONE',  ( 9.338484253624125486, -13.53666216847648052, -219.8958652322373837 ) ) ;
#20761=CARTESIAN_POINT ( 'NONE',  ( -2.772442535524381579, 13.75675912271027457, -228.9770533867650215 ) ) ;
#20762=CARTESIAN_POINT ( 'NONE',  ( -22.35595593184171292, -2.191382721379458332, -235.3044553127160441 ) ) ;
#20763=CARTESIAN_POINT ( 'NONE',  ( 23.48720700658024896, -2.145453947144424500, -217.8824464111000054 ) ) ;
#20764=CARTESIAN_POINT ( 'NONE',  ( 13.43730899468209294, 8.427513769504761498, -221.4030804848920297 ) ) ;
#20765=CARTESIAN_POINT ( 'NONE',  ( -20.94800339253696109, 4.477632454355491731, -216.5423208360950298 ) ) ;
#20766=CARTESIAN_POINT ( 'NONE',  ( 8.532614294830283441, -28.73326933124977955, -229.1610356131385231 ) ) ;
#20768=CARTESIAN_POINT ( 'NONE',  ( -7.189383125363055349, 14.28512618638020548, -231.7475838278701303 ) ) ;
#20769=CARTESIAN_POINT ( 'NONE',  ( -21.89065952084848021, -0.9940043559354364566, -216.9999999999999716 ) ) ;
#20770=CARTESIAN_POINT ( 'NONE',  ( -5.805911442544755552, -26.83424102279996504, -229.6222293353685302 ) ) ;
#20773=CARTESIAN_POINT ( 'NONE',  ( -13.10651848559790444, 3.262242204071156948, -224.3513854875720597 ) ) ;
#20774=CARTESIAN_POINT ( 'NONE',  ( 23.15933523859005660, -14.47549635653155775, -222.2572217030593436 ) ) ;
#20775=CARTESIAN_POINT ( 'NONE',  ( -24.25245498015852874, 0.2109992039763788352, -218.1398602137601301 ) ) ;
#20777=CARTESIAN_POINT ( 'NONE',  ( 12.98277799799954124, 10.30128574332056779, -221.9415428419440559 ) ) ;
#20778=CARTESIAN_POINT ( 'NONE',  ( -7.686214453470440411, 10.71593237010305444, -228.8058998235944159 ) ) ;
#20780=CARTESIAN_POINT ( 'NONE',  ( 13.17424634425744046, 10.51488364724239588, -221.4616598107521099 ) ) ;
#20781=CARTESIAN_POINT ( 'NONE',  ( 0.7148793108008648645, -17.78534256477599840, -218.6573294195452775 ) ) ;
#20782=CARTESIAN_POINT ( 'NONE',  ( 27.83450977899788370, 1.364662819714677511, -230.5442677252456463 ) ) ;
#20784=CARTESIAN_POINT ( 'NONE',  ( -4.386767007475907754, 14.39570986262862107, -223.2690175027443615 ) ) ;
#20785=CARTESIAN_POINT ( 'NONE',  ( -14.59766675578715223, 7.926254675926275972, -222.3706877972550444 ) ) ;
#20786=CARTESIAN_POINT ( 'NONE',  ( -12.13127060986278316, 5.971392262169284315, -229.0615017441034524 ) ) ;
#20788=CARTESIAN_POINT ( 'NONE',  ( -11.98034293927688765, -10.98662817740026121, -223.7553339400932373 ) ) ;
#20791=CARTESIAN_POINT ( 'NONE',  ( 16.20788843645364352, 6.828976201867700269, -231.6689701909764665 ) ) ;
#20792=CARTESIAN_POINT ( 'NONE',  ( 12.14783608763084644, -10.95966212275308571, -222.8518398773795184 ) ) ;
#20793=CARTESIAN_POINT ( 'NONE',  ( 14.68783945462866924, 9.535285537539673228, -219.4694094309942045 ) ) ;
#20794=CARTESIAN_POINT ( 'NONE',  ( -14.73016414256368911, 22.23431809695627237, -217.1425123644553707 ) ) ;
#20797=CARTESIAN_POINT ( 'NONE',  ( 12.08790845148079640, 6.355304031620478078, -220.0087475230167229 ) ) ;
#20799=CARTESIAN_POINT ( 'NONE',  ( 1.773982976645536835, 19.12448993322812285, -233.2315972735944172 ) ) ;
#20801=CARTESIAN_POINT ( 'NONE',  ( 8.021672912688133650, -23.92397517040199872, -233.3380040120402441 ) ) ;
#20802=CARTESIAN_POINT ( 'NONE',  ( 11.39114332821395692, -8.257479203742953189, -226.5648397932267528 ) ) ;
#20805=CARTESIAN_POINT ( 'NONE',  ( -23.70973587455150522, 20.45398817402440983, -228.9005348699235469 ) ) ;
#20806=CARTESIAN_POINT ( 'NONE',  ( -26.46950597041758968, -8.633348373924491170, -225.4226425040951085 ) ) ;
#20808=CARTESIAN_POINT ( 'NONE',  ( -15.83178333309709629, 2.467763724635483324, -230.4064772870105458 ) ) ;
#20809=CARTESIAN_POINT ( 'NONE',  ( 8.175342817246784577, 19.41817470142738244, -216.6818271833384699 ) ) ;
#20810=CARTESIAN_POINT ( 'NONE',  ( -1.973648319964989462, 15.33498294326524203, -220.9958390492969329 ) ) ;
#20812=CARTESIAN_POINT ( 'NONE',  ( 12.82249318900957391, -5.922664226158099510, -218.4318038749311768 ) ) ;
#20813=CARTESIAN_POINT ( 'NONE',  ( 25.69300549816939494, 5.947472783069708946, -230.6131061331718115 ) ) ;
#20814=CARTESIAN_POINT ( 'NONE',  ( -11.59479561055411345, 9.544396733298208702, -229.1494558965577255 ) ) ;
#20815=CARTESIAN_POINT ( 'NONE',  ( -27.11599398522282911, 10.60460483532474996, -224.7310548435675912 ) ) ;
#20816=CARTESIAN_POINT ( 'NONE',  ( -8.978805095734141872, -14.89723076936793156, -219.0730636071341451 ) ) ;
#20817=CARTESIAN_POINT ( 'NONE',  ( -16.15126510923403202, -0.4755054218165427615, -219.3066569788202571 ) ) ;
#20821=CARTESIAN_POINT ( 'NONE',  ( -11.13829636790841704, 14.30978168460582189, -218.6922574227322400 ) ) ;
#20822=CARTESIAN_POINT ( 'NONE',  ( 10.93653298376230687, 10.42959444671468106, -232.5920418140667039 ) ) ;
#20823=CARTESIAN_POINT ( 'NONE',  ( -18.46722752239034193, 0.9784074152395518809, -232.1633353206286188 ) ) ;
#20824=CARTESIAN_POINT ( 'NONE',  ( -32.13037437807204810, -1.025156162654832670, -224.7589498746283141 ) ) ;
#20825=CARTESIAN_POINT ( 'NONE',  ( -23.85568197540453994, -15.41036827548725618, -219.8503866864575969 ) ) ;
#20826=CARTESIAN_POINT ( 'NONE',  ( -14.84124724799726991, 21.42277200659090042, -233.6300684249849553 ) ) ;
#20827=CARTESIAN_POINT ( 'NONE',  ( -8.376153411442972541, -27.59911039556260448, -219.0729038785590888 ) ) ;
#20828=CARTESIAN_POINT ( 'NONE',  ( 8.812073984913094904, 13.12649198322903210, -229.9172071780580495 ) ) ;
#20829=CARTESIAN_POINT ( 'NONE',  ( 4.579865149819754677, -13.09122092233156387, -219.1296897471712839 ) ) ;
#20831=CARTESIAN_POINT ( 'NONE',  ( -27.92885697401080591, 6.962042978589167319, -220.9552227796709190 ) ) ;
#20832=PRESENTATION_STYLE_ASSIGNMENT (( #21270 ) ) ;
#20833=CARTESIAN_POINT ( 'NONE',  ( -5.589224416770360193, 14.13652937339764115, -225.1481999119820330 ) ) ;
#20834=CARTESIAN_POINT ( 'NONE',  ( -20.00523085820573499, 3.356386534894876927, -232.9491364426554298 ) ) ;
#20835=CARTESIAN_POINT ( 'NONE',  ( 24.58316096239279602, 5.861425670879941485, -231.3104446318280623 ) ) ;
#20836=CARTESIAN_POINT ( 'NONE',  ( 15.14859676485869500, 2.119979922547468032, -231.9009926880791284 ) ) ;
#20837=CARTESIAN_POINT ( 'NONE',  ( 1.444415905432371749, -18.02453083990606331, -216.1804672466811894 ) ) ;
#20838=CARTESIAN_POINT ( 'NONE',  ( 5.784594921161807513, 11.98867617302893329, -219.3746160931291058 ) ) ;
#20839=CARTESIAN_POINT ( 'NONE',  ( 27.40550551777678123, 5.967061366481472895, -228.7463788799179554 ) ) ;
#20840=CARTESIAN_POINT ( 'NONE',  ( -5.131528111146875126, -19.01772154664624992, -215.2265844479019563 ) ) ;
#20841=CARTESIAN_POINT ( 'NONE',  ( -4.142636420702924482, 14.17169704882741321, -225.1666440184957310 ) ) ;
#20842=CARTESIAN_POINT ( 'NONE',  ( 7.213476267053916757, 16.78447451494783138, -217.5857052077849687 ) ) ;
#20843=CARTESIAN_POINT ( 'NONE',  ( -18.11268275035277853, -3.459088653808292335, -218.4233329573673359 ) ) ;
#20844=CARTESIAN_POINT ( 'NONE',  ( -18.33565906012873725, 9.491905303418088025, -219.1855745749628568 ) ) ;
#20846=CARTESIAN_POINT ( 'NONE',  ( -5.028549462823471039, 18.55099042571767143, -234.6264744246184648 ) ) ;
#20847=CARTESIAN_POINT ( 'NONE',  ( 16.77055746703809191, 7.081497542956901370, -232.0295235404293521 ) ) ;
#20849=CARTESIAN_POINT ( 'NONE',  ( 7.033108278341462238, -17.71891568601925826, -230.1509483552532060 ) ) ;
#20850=ORIENTED_EDGE ( 'NONE', *, *, #6311, .F. ) ;
#20851=CARTESIAN_POINT ( 'NONE',  ( 8.211296573249146746, -12.45047565346596130, -222.1279395315445413 ) ) ;
#20852=CARTESIAN_POINT ( 'NONE',  ( -6.067446494494625142, 16.28408815813367028, -230.0786439517394513 ) ) ;
#20854=CARTESIAN_POINT ( 'NONE',  ( 12.99034161053428349, 11.71468708507361889, -230.9043293568357740 ) ) ;
#20855=CARTESIAN_POINT ( 'NONE',  ( 22.36788034568564854, -2.140002702436959225, -217.7104380410378610 ) ) ;
#20856=CARTESIAN_POINT ( 'NONE',  ( -25.10035252441274167, -15.33546242866430198, -228.3913311683031964 ) ) ;
#20857=CARTESIAN_POINT ( 'NONE',  ( 3.342529885312644833, -17.78621320651278737, -216.7788622297345853 ) ) ;
#20858=CARTESIAN_POINT ( 'NONE',  ( -5.589224416770360193, 14.13652937339764115, -225.1481999119820330 ) ) ;
#20860=CARTESIAN_POINT ( 'NONE',  ( 24.93482953594869755, 13.13888391581411241, -222.4369546851285691 ) ) ;
#20862=CARTESIAN_POINT ( 'NONE',  ( -11.02345917017863464, 29.02019856777526741, -223.9475008740665771 ) ) ;
#20863=CARTESIAN_POINT ( 'NONE',  ( -8.137644474477026435, 12.10064032984799098, -226.6735072060122036 ) ) ;
#20864=CARTESIAN_POINT ( 'NONE',  ( 10.40160332990717151, 27.59713857063802323, -221.5374724512453213 ) ) ;
#20865=CARTESIAN_POINT ( 'NONE',  ( -16.88145396433676027, 5.002512658926777434, -221.2364783498041731 ) ) ;
#20866=CARTESIAN_POINT ( 'NONE',  ( 16.53896178738450828, 2.691624496798088462, -232.5974196329879078 ) ) ;
#20867=CARTESIAN_POINT ( 'NONE',  ( 18.24334571313621467, -21.83696521683136282, -220.5798317591433886 ) ) ;
#20870=CARTESIAN_POINT ( 'NONE',  ( -2.934221234790329369, 15.07857928364152222, -230.9558365497803720 ) ) ;
#20871=CARTESIAN_POINT ( 'NONE',  ( 22.26090851979669338, -3.689523054771738586, -218.9825289563843285 ) ) ;
#20873=CARTESIAN_POINT ( 'NONE',  ( 24.42567939027770407, 10.22651298688739097, -219.4562066833365748 ) ) ;
#20874=CARTESIAN_POINT ( 'NONE',  ( -24.48580119005125866, 9.312492396273500006, -232.5498413856076070 ) ) ;
#20875=CARTESIAN_POINT ( 'NONE',  ( 5.668262076144046979, -25.28042871382391965, -216.8182873783340483 ) ) ;
#20877=CARTESIAN_POINT ( 'NONE',  ( -24.02434186778878455, 18.57431834865475651, -228.2662945587547370 ) ) ;
#20878=CARTESIAN_POINT ( 'NONE',  ( -16.09559989144903369, 12.31939076846282966, -216.7948290530243298 ) ) ;
#20880=CARTESIAN_POINT ( 'NONE',  ( -28.99926036811508467, 3.909990568804979194, -228.9613767892386988 ) ) ;
#20881=CARTESIAN_POINT ( 'NONE',  ( -15.43902962033193837, -12.71219713885795422, -232.7078469548986845 ) ) ;
#20883=CARTESIAN_POINT ( 'NONE',  ( 15.52031161554735128, 1.026483668354684076, -227.8437971491433132 ) ) ;
#20884=CARTESIAN_POINT ( 'NONE',  ( -11.67631226053870996, 6.737291529340801333, -227.3110382950315227 ) ) ;
#20885=CARTESIAN_POINT ( 'NONE',  ( 7.357019007885960526, -24.37006613449481662, -217.4041786725384782 ) ) ;
#20888=CARTESIAN_POINT ( 'NONE',  ( 21.68053922431529301, 13.05890675940072931, -230.5667798303363440 ) ) ;
#20889=CARTESIAN_POINT ( 'NONE',  ( -18.07648963816576781, 14.36622924931724654, -235.1425738388569187 ) ) ;
#20891=CARTESIAN_POINT ( 'NONE',  ( 15.20072702475037296, 19.31591084219522614, -219.7402199933931399 ) ) ;
#20892=CARTESIAN_POINT ( 'NONE',  ( -3.614824051224299950, -15.07124992037100064, -223.1721701483932065 ) ) ;
#20893=CARTESIAN_POINT ( 'NONE',  ( 25.70000612522241568, -7.596455516557234944, -216.8500112287931074 ) ) ;
#20895=CARTESIAN_POINT ( 'NONE',  ( -4.879985665934096772, 15.33285679834440174, -220.9402849574511833 ) ) ;
#20896=CARTESIAN_POINT ( 'NONE',  ( -26.64664107080812627, 5.256684826493772000, -228.0533579629717735 ) ) ;
#20897=CARTESIAN_POINT ( 'NONE',  ( -26.47501633019681577, 13.84484755257420119, -230.0154374881822719 ) ) ;
#20900=CARTESIAN_POINT ( 'NONE',  ( -11.82770121052164924, -14.33821066513346487, -229.8071374592849452 ) ) ;
#20902=CARTESIAN_POINT ( 'NONE',  ( 25.40954707198727647, 2.077273811637330159, -219.3610170479527426 ) ) ;
#20903=CARTESIAN_POINT ( 'NONE',  ( 3.242550426224029447, -16.70085388461110654, -229.1030317736733650 ) ) ;
#20904=CARTESIAN_POINT ( 'NONE',  ( 22.46220731426537043, 18.23201731183003460, -227.5436199598787539 ) ) ;
#20905=CARTESIAN_POINT ( 'NONE',  ( -7.395406416482832590, 12.93623984139929739, -219.2606224730616873 ) ) ;
#20907=ADVANCED_BREP_SHAPE_REPRESENTATION ( '', ( #21952, #6677 ), #13476 ) ;
#20908=CARTESIAN_POINT ( 'NONE',  ( 20.82555317450757215, 14.06078233701296476, -215.4201375757437802 ) ) ;
#20910=CARTESIAN_POINT ( 'NONE',  ( 4.656903975822286768, 13.45000048768594780, -227.6722060245555497 ) ) ;
#20911=CARTESIAN_POINT ( 'NONE',  ( 14.44151618910354706, 2.059759062152056064, -222.8188548941175782 ) ) ;
#20912=CARTESIAN_POINT ( 'NONE',  ( -7.832594822155400927, -23.57318293858060088, -216.4298491688572028 ) ) ;
#20913=CARTESIAN_POINT ( 'NONE',  ( 21.39922646226391478, -21.53954253117021977, -224.1701659532164967 ) ) ;
#20916=CARTESIAN_POINT ( 'NONE',  ( -10.98447002683091256, 8.146786682930290624, -230.8316952156193338 ) ) ;
#20917=CARTESIAN_POINT ( 'NONE',  ( 25.14972984070899997, 1.185371537549434029, -234.2576837523010909 ) ) ;
#20918=CARTESIAN_POINT ( 'NONE',  ( 20.47387447818710271, 7.390772095927000684, -234.0991886097562258 ) ) ;
#20919=CARTESIAN_POINT ( 'NONE',  ( 2.579827969572558111, 15.91317371615649101, -219.7652087782269916 ) ) ;
#20920=CARTESIAN_POINT ( 'NONE',  ( -0.4548635697939061306, 27.30478022265488036, -219.8474162243132071 ) ) ;
#20922=CARTESIAN_POINT ( 'NONE',  ( 20.78003164828882632, -23.67023879211220461, -227.8573985392403074 ) ) ;
#20924=CARTESIAN_POINT ( 'NONE',  ( 16.84848658399567611, 11.39632653812981644, -217.9589513831453473 ) ) ;
#20927=CARTESIAN_POINT ( 'NONE',  ( -22.57859951143173660, 16.82392524473188899, -219.5628058978911383 ) ) ;
#20928=CARTESIAN_POINT ( 'NONE',  ( -12.99458409358603284, 11.56864380452031504, -232.0274663316965018 ) ) ;
#20929=CARTESIAN_POINT ( 'NONE',  ( -26.09107693309126574, -10.38942742183557399, -230.9365759677854442 ) ) ;
#20930=CARTESIAN_POINT ( 'NONE',  ( -18.39892766464214446, 25.11039525536027739, -225.3444503920457294 ) ) ;
#20932=CARTESIAN_POINT ( 'NONE',  ( 14.83290459615719215, -2.296615622475745688, -226.9301701175285757 ) ) ;
#20933=CARTESIAN_POINT ( 'NONE',  ( 14.32449519560807438, 0.8432996792098175209, -220.3117614177709527 ) ) ;
#20934=CARTESIAN_POINT ( 'NONE',  ( -13.14888680331901583, 26.03314517226533908, -227.7900104434697539 ) ) ;
#20935=CARTESIAN_POINT ( 'NONE',  ( 14.75291830987536557, 13.43762972591284033, -235.1407057970265839 ) ) ;
#20936=CARTESIAN_POINT ( 'NONE',  ( 21.83031488337932657, -1.542591969257240070, -231.3901500139511427 ) ) ;
#20938=CARTESIAN_POINT ( 'NONE',  ( -11.66037817688884992, -1.871521667041048609, -223.1840616512448037 ) ) ;
#20939=CARTESIAN_POINT ( 'NONE',  ( -12.18037021406049547, -6.685450889859271051, -226.7642181357440734 ) ) ;
#20940=CARTESIAN_POINT ( 'NONE',  ( -23.95129667199961077, 20.99391807043993552, -227.1541646794576081 ) ) ;
#20941=CARTESIAN_POINT ( 'NONE',  ( -2.576162127940193169, -15.57202066281789321, -231.6911579627040396 ) ) ;
#20942=CARTESIAN_POINT ( 'NONE',  ( 10.07175337281514871, 14.76776740066196325, -231.7834566702614723 ) ) ;
#20943=CARTESIAN_POINT ( 'NONE',  ( 14.31773767102621875, -28.01644431351170894, -220.7875045263454865 ) ) ;
#20944=CARTESIAN_POINT ( 'NONE',  ( 14.44752737957290734, -0.3096824834134420112, -227.9839733948226410 ) ) ;
#20945=CARTESIAN_POINT ( 'NONE',  ( -16.81936022032888545, 5.700806722825413786, -218.5726178058217215 ) ) ;
#20947=CARTESIAN_POINT ( 'NONE',  ( -7.058999618647554541, 24.62458660126260312, -219.6630466582859356 ) ) ;
#20948=CARTESIAN_POINT ( 'NONE',  ( -28.61025869263052712, 6.891613135096296361, -222.2489362813765013 ) ) ;
#20949=CARTESIAN_POINT ( 'NONE',  ( 23.49048926389013658, 9.645778135078892035, -218.7307869890797463 ) ) ;
#20950=CARTESIAN_POINT ( 'NONE',  ( 20.88350594575732799, 13.65521425050155813, -232.8060468608549911 ) ) ;
#20951=CARTESIAN_POINT ( 'NONE',  ( -9.979217823323752512, -26.65442139683551659, -219.8174849573283325 ) ) ;
#20952=CARTESIAN_POINT ( 'NONE',  ( 18.26039090677515375, 26.14311541888654844, -228.1864986152887127 ) ) ;
#20955=CARTESIAN_POINT ( 'NONE',  ( -12.24325066776002657, -20.13554689852184509, -214.7483342848939856 ) ) ;
#20956=CARTESIAN_POINT ( 'NONE',  ( -10.02095171162140019, 11.02119725306997111, -224.1251327387667516 ) ) ;
#20957=CARTESIAN_POINT ( 'NONE',  ( 8.592982993077152187, 10.20906991731218838, -226.0923132092261483 ) ) ;
#20958=CARTESIAN_POINT ( 'NONE',  ( -13.91323058514953637, 8.006348396443080162, -225.5064972756604220 ) ) ;
#20960=CARTESIAN_POINT ( 'NONE',  ( 1.920320557106582893, 25.99317453242502296, -234.5637964893073217 ) ) ;
#20961=CARTESIAN_POINT ( 'NONE',  ( 24.60354977307301283, 7.993510024274534942, -218.5358880819990759 ) ) ;
#20963=CARTESIAN_POINT ( 'NONE',  ( 17.63166870185818169, -20.21345786093278107, -221.6360081359454739 ) ) ;
#20965=CARTESIAN_POINT ( 'NONE',  ( 12.78854151797817451, -25.92021405714643123, -222.0152117995072842 ) ) ;
#20967=CARTESIAN_POINT ( 'NONE',  ( -8.467651734177735534, 23.23776955534497546, -231.2693664226804913 ) ) ;
#20970=CARTESIAN_POINT ( 'NONE',  ( 9.333020543840051531, 16.91085096921651143, -217.7308990335875762 ) ) ;
#20971=CARTESIAN_POINT ( 'NONE',  ( 24.21331552874348958, 0.07051084380047288602, -231.7986140076958463 ) ) ;
#20972=CARTESIAN_POINT ( 'NONE',  ( -21.08965452150356867, -10.66825825602615296, -217.1903588586143314 ) ) ;
#20974=CARTESIAN_POINT ( 'NONE',  ( 1.904360901363437275, -12.77109371939166138, -224.5066922355585177 ) ) ;
#20975=CARTESIAN_POINT ( 'NONE',  ( -0.3589900283600636066, 18.35437183075527656, -220.3960288481451357 ) ) ;
#20977=CARTESIAN_POINT ( 'NONE',  ( 13.80707869872719762, 6.429545566348308760, -225.7152177910682553 ) ) ;
#20978=CARTESIAN_POINT ( 'NONE',  ( -17.65835845419170624, 22.55329142274348442, -231.2673511165784532 ) ) ;
#20979=CARTESIAN_POINT ( 'NONE',  ( -3.010752168931037698, 15.84372070116375575, -223.4060793985500482 ) ) ;
#20981=CARTESIAN_POINT ( 'NONE',  ( 0.8374361358884788720, 23.73768315274483953, -232.4065959030912154 ) ) ;
#20982=CARTESIAN_POINT ( 'NONE',  ( -24.92290506463145405, 6.124412323591598373, -220.3779252408000104 ) ) ;
#20983=CARTESIAN_POINT ( 'NONE',  ( 26.75877786246624623, 11.80320999550499117, -231.5572967531201414 ) ) ;
#20984=CARTESIAN_POINT ( 'NONE',  ( 6.869068212838696397, -24.78254998730118430, -231.2855974421026986 ) ) ;
#20985=CARTESIAN_POINT ( 'NONE',  ( 20.13946171159960841, -0.1427001808266660232, -233.7987036390019853 ) ) ;
#20987=CARTESIAN_POINT ( 'NONE',  ( 9.586902571418640662, 24.43292817174309661, -231.9968623198229807 ) ) ;
#20988=CARTESIAN_POINT ( 'NONE',  ( -27.54101393026537181, -2.112662437277116556, -233.6092940012385384 ) ) ;
#20990=CARTESIAN_POINT ( 'NONE',  ( 15.01439307471096463, 1.118969480519667048, -226.7488225241675366 ) ) ;
#20991=CARTESIAN_POINT ( 'NONE',  ( 1.623338700557370951, -21.82196275546919040, -234.1129525514646730 ) ) ;
#20992=CARTESIAN_POINT ( 'NONE',  ( -18.70100282803782576, 16.58357028540773115, -216.4425743468854080 ) ) ;
#20994=CARTESIAN_POINT ( 'NONE',  ( -12.39195900010699702, 23.13258866008456138, -233.4668451572263166 ) ) ;
#20996=CARTESIAN_POINT ( 'NONE',  ( -17.79285498209129202, 9.187865686019035749, -216.3798185811636756 ) ) ;
#20997=CARTESIAN_POINT ( 'NONE',  ( -13.44605823798860200, -7.860403065310468840, -219.7865185367595586 ) ) ;
#21000=CARTESIAN_POINT ( 'NONE',  ( -15.15434969228324924, 4.423874646950748613, -230.6144467931089821 ) ) ;
#21001=CARTESIAN_POINT ( 'NONE',  ( 7.317916060359300978, -13.14109500694934951, -227.5371884182924305 ) ) ;
#21003=CARTESIAN_POINT ( 'NONE',  ( 25.01541028746040141, 13.78427203520734423, -225.9266837950359843 ) ) ;
#21004=CARTESIAN_POINT ( 'NONE',  ( -10.14083745617744547, 19.87482866967577877, -216.0596634563153486 ) ) ;
#21006=CARTESIAN_POINT ( 'NONE',  ( 10.32480721127626033, 15.84468581819879773, -230.0799086455579072 ) ) ;
#21007=CARTESIAN_POINT ( 'NONE',  ( -0.8455829679720252567, -23.09678443543459991, -232.4899849032512122 ) ) ;
#21009=CARTESIAN_POINT ( 'NONE',  ( -11.03778527004271659, 26.96286968643956428, -225.4057095641571209 ) ) ;
#21010=CARTESIAN_POINT ( 'NONE',  ( -8.892156391762910062, 11.89593067802204551, -225.4519868197583889 ) ) ;
#21011=CARTESIAN_POINT ( 'NONE',  ( -21.12280458060320498, 13.61074013710079988, -216.5529903464332335 ) ) ;
#21014=CARTESIAN_POINT ( 'NONE',  ( -16.29786170208491924, -8.453292648900102790, -230.0691174225123632 ) ) ;
#21018=CARTESIAN_POINT ( 'NONE',  ( -21.89065952084848021, -0.9940043559354364566, -216.9999999999999716 ) ) ;
#21019=CARTESIAN_POINT ( 'NONE',  ( 7.144583572002897398, -18.19063289417396945, -230.4059351064080658 ) ) ;
#21020=CARTESIAN_POINT ( 'NONE',  ( 20.23125423326388628, 7.836699765464857137, -217.8891354894872450 ) ) ;
#21021=CARTESIAN_POINT ( 'NONE',  ( -10.51143808951550085, 11.41308718311005066, -231.3573069600382439 ) ) ;
#21022=CARTESIAN_POINT ( 'NONE',  ( 27.79290571682592770, 12.05347838982552666, -230.1298045326732051 ) ) ;
#21023=CARTESIAN_POINT ( 'NONE',  ( 12.04687593227112430, 27.54339840196571743, -224.6466266724203820 ) ) ;
#21026=CARTESIAN_POINT ( 'NONE',  ( -14.13781561609191328, -15.90667165809925621, -233.6615929499251649 ) ) ;
#21028=CARTESIAN_POINT ( 'NONE',  ( 22.44368505003003378, -11.72633196808685163, -232.1179326287041533 ) ) ;
#21031=CARTESIAN_POINT ( 'NONE',  ( -10.54177647804913320, 7.401649028325941515, -220.3980514230326264 ) ) ;
#21032=CARTESIAN_POINT ( 'NONE',  ( -17.17062072939792117, -6.705141685950851027, -229.6398969478225354 ) ) ;
#21033=CARTESIAN_POINT ( 'NONE',  ( -24.18895665211001500, 11.26087434487096139, -231.0040666710689550 ) ) ;
#21034=CARTESIAN_POINT ( 'NONE',  ( 21.77183241683778547, 12.04504704525620085, -233.6005549158834640 ) ) ;
#21035=CARTESIAN_POINT ( 'NONE',  ( 5.446894657575932719, 15.00061806465251557, -226.4498309983864317 ) ) ;
#21037=CARTESIAN_POINT ( 'NONE',  ( 11.42868579270797369, -5.440147491673143598, -220.7688621915004603 ) ) ;
#21038=CARTESIAN_POINT ( 'NONE',  ( 15.89706143421296147, 10.57416387607782227, -218.3862415393350318 ) ) ;
#21039=CARTESIAN_POINT ( 'NONE',  ( -13.43384090552117271, 6.057765724406720231, -225.7182623230366119 ) ) ;
#21040=CARTESIAN_POINT ( 'NONE',  ( -8.413706464639300719, 10.92140547936800843, -220.6417935981040728 ) ) ;
#21041=CARTESIAN_POINT ( 'NONE',  ( -22.19673167533144564, -9.562764463827019057, -233.1557790568585062 ) ) ;
#21042=CARTESIAN_POINT ( 'NONE',  ( -9.443239614166923701, 9.388015667058336788, -222.3195230688234290 ) ) ;
#21044=CARTESIAN_POINT ( 'NONE',  ( 28.65393683769942967, 4.398063292302325067, -219.1542358361629965 ) ) ;
#21045=CARTESIAN_POINT ( 'NONE',  ( -11.69222874857179484, 25.57550432052970280, -219.9467848335519591 ) ) ;
#21046=CARTESIAN_POINT ( 'NONE',  ( 24.00840102751045890, 17.37402299239434100, -218.3110108534040137 ) ) ;
#21047=CARTESIAN_POINT ( 'NONE',  ( -26.58771759052039485, 5.114955214121561511, -218.2823714869195442 ) ) ;
#21048=CARTESIAN_POINT ( 'NONE',  ( -15.92941692657317354, -7.780888323563449838, -232.0381278758927976 ) ) ;
#21049=CARTESIAN_POINT ( 'NONE',  ( 3.100794261777709782, 20.70580715608724276, -231.8781843337728219 ) ) ;
#21050=CARTESIAN_POINT ( 'NONE',  ( -6.163092920833200594, -27.00835405423771007, -232.1022292408408987 ) ) ;
#21051=CARTESIAN_POINT ( 'NONE',  ( 17.97843143658897347, 22.12221935793617078, -220.9346589834416079 ) ) ;
#21052=CARTESIAN_POINT ( 'NONE',  ( 5.521532699605532279, -19.36944961733043513, -235.0341191922501594 ) ) ;
#21056=CARTESIAN_POINT ( 'NONE',  ( 17.23039831256031817, 3.331158952577910615, -216.4027685342793461 ) ) ;
#21058=CARTESIAN_POINT ( 'NONE',  ( 27.81506808824343580, -10.52944849582878106, -221.0913368219556503 ) ) ;
#21059=CARTESIAN_POINT ( 'NONE',  ( 10.64798096806036121, 19.48085866535796740, -231.3996658690317361 ) ) ;
#21060=CARTESIAN_POINT ( 'NONE',  ( 29.81944548462877975, 8.043843257819576209, -228.1755181449411793 ) ) ;
#21061=CARTESIAN_POINT ( 'NONE',  ( 17.07668571305246985, 2.037405138410691485, -219.7626854147787867 ) ) ;
#21062=CARTESIAN_POINT ( 'NONE',  ( -7.007669255080013926, -23.60960382150139836, -233.3096631214588115 ) ) ;
#21064=CARTESIAN_POINT ( 'NONE',  ( 11.31331191788792623, 29.23420701778062281, -220.7538464529627333 ) ) ;
#21066=CARTESIAN_POINT ( 'NONE',  ( -4.737391463177558215, -17.33199396152823368, -215.7912354007318925 ) ) ;
#21067=CARTESIAN_POINT ( 'NONE',  ( -9.954421844142357756, 11.21484508112568079, -226.0177122452137439 ) ) ;
#21068=CARTESIAN_POINT ( 'NONE',  ( 20.26651059498356844, 18.95255124124090074, -231.7206897233655525 ) ) ;
#21069=CARTESIAN_POINT ( 'NONE',  ( -16.56270003954679382, 4.935922114544952777, -221.6503923146493378 ) ) ;
#21070=CARTESIAN_POINT ( 'NONE',  ( 3.744112528862662881, 31.76296354843916703, -227.8872370379487506 ) ) ;
#21071=CARTESIAN_POINT ( 'NONE',  ( 18.79638869589749461, 0.4878066561304963966, -219.5712168927955759 ) ) ;
#21073=CARTESIAN_POINT ( 'NONE',  ( 13.80508996112396680, -23.93364289317450400, -226.6703843709330783 ) ) ;
#21074=CARTESIAN_POINT ( 'NONE',  ( 12.20621255000322947, -21.57429421806300240, -232.1397031738524674 ) ) ;
#21075=CARTESIAN_POINT ( 'NONE',  ( -0.2748333203896175525, 17.57683079704640505, -221.1444293135629948 ) ) ;
#21078=CARTESIAN_POINT ( 'NONE',  ( 17.34727976380017722, 4.822939981779328811, -230.8836217450937909 ) ) ;
#21079=CARTESIAN_POINT ( 'NONE',  ( 16.08921376350389920, -2.840750994787607731, -229.5571464835293796 ) ) ;
#21080=CARTESIAN_POINT ( 'NONE',  ( -13.88883449434014672, -11.15328429608096172, -217.8357414694029046 ) ) ;
#21081=CARTESIAN_POINT ( 'NONE',  ( -8.376153411442972541, -27.59911039556260448, -219.0729038785590888 ) ) ;
#21082=CARTESIAN_POINT ( 'NONE',  ( -7.770318051073092036, 21.02940971564074957, -231.8751410922876630 ) ) ;
#21084=CARTESIAN_POINT ( 'NONE',  ( 15.99247752609008444, 10.72268246046808216, -230.5614800526110173 ) ) ;
#21085=CARTESIAN_POINT ( 'NONE',  ( -6.855867220396999251, 12.17758473459128332, -220.6375607554995213 ) ) ;
#21086=CARTESIAN_POINT ( 'NONE',  ( -11.11479000491124047, 20.76372272540567110, -218.2001872134434564 ) ) ;
#21089=CARTESIAN_POINT ( 'NONE',  ( 2.471164685565028662, 14.01327037412690935, -223.4905256513065410 ) ) ;
#21090=CARTESIAN_POINT ( 'NONE',  ( 17.91327661571172314, 1.545939370248587075, -216.9938266089438912 ) ) ;
#21091=CARTESIAN_POINT ( 'NONE',  ( 17.98589043827631428, 2.945998030785370592, -233.4030907785035538 ) ) ;
#21093=CARTESIAN_POINT ( 'NONE',  ( 6.930886114109415352, -28.33506752827666020, -226.0544877841801110 ) ) ;
#21096=CARTESIAN_POINT ( 'NONE',  ( 2.837900457371055563, 25.11342719071438978, -232.9871906064174709 ) ) ;
#21097=CARTESIAN_POINT ( 'NONE',  ( 17.01404819207892061, -3.492736430306117690, -221.2516733069050190 ) ) ;
#21100=CARTESIAN_POINT ( 'NONE',  ( 6.589392574981438599, -17.08498810221841069, -232.9613445306918322 ) ) ;
#21101=CARTESIAN_POINT ( 'NONE',  ( -12.74846050492543625, 19.93509882904884734, -216.0172840992881049 ) ) ;
#21102=CARTESIAN_POINT ( 'NONE',  ( -13.24620988741752825, 28.78239319002125285, -225.3527830703614256 ) ) ;
#21104=CARTESIAN_POINT ( 'NONE',  ( -9.740348021262962064, 16.12529029871877384, -216.4361617420699702 ) ) ;
#21105=CARTESIAN_POINT ( 'NONE',  ( -12.18037021406049547, -6.685450889859271051, -226.7642181357440734 ) ) ;
#21108=CARTESIAN_POINT ( 'NONE',  ( -25.29098058636142810, 5.014641116111857144, -217.4658967307323110 ) ) ;
#21109=CARTESIAN_POINT ( 'NONE',  ( 10.12607331509846986, -17.07097861414113638, -217.9029769802564545 ) ) ;
#21110=CARTESIAN_POINT ( 'NONE',  ( 14.40511183577193677, -1.529481993174749865, -222.4191515927619776 ) ) ;
#21111=CARTESIAN_POINT ( 'NONE',  ( -18.09776816382430908, 23.50806826204562583, -229.9568677523880638 ) ) ;
#21112=CARTESIAN_POINT ( 'NONE',  ( 12.51085646230496273, 9.582567546749562126, -224.6200301875240939 ) ) ;
#21113=CARTESIAN_POINT ( 'NONE',  ( -23.16143087541734502, 21.36835206473086046, -221.8715256527013651 ) ) ;
#21114=CARTESIAN_POINT ( 'NONE',  ( 13.62455467724876712, 0.2254024858538909992, -227.9921160535819809 ) ) ;
#21115=CARTESIAN_POINT ( 'NONE',  ( 20.64430047260004031, 12.67811357335941480, -231.0449411089858813 ) ) ;
#21116=CARTESIAN_POINT ( 'NONE',  ( 5.229904874806564408, -24.29892824652383609, -233.0630010234598046 ) ) ;
#21117=ORIENTED_EDGE ( 'NONE', *, *, #11520, .T. ) ;
#21118=CARTESIAN_POINT ( 'NONE',  ( 3.367418898937407867, 27.20023797116225595, -219.3349021808245709 ) ) ;
#21119=CARTESIAN_POINT ( 'NONE',  ( -10.65640919150578192, 23.79238421564942740, -218.1088542024188826 ) ) ;
#21120=CARTESIAN_POINT ( 'NONE',  ( 21.43345597994050777, 2.294722475943265838, -232.7243927205661294 ) ) ;
#21121=CARTESIAN_POINT ( 'NONE',  ( -11.98587399847077783, -10.70615994290841044, -225.3229167341726225 ) ) ;
#21124=CARTESIAN_POINT ( 'NONE',  ( 24.32561047128371001, 1.769413244618101011, -218.8629106451077462 ) ) ;
#21125=CARTESIAN_POINT ( 'NONE',  ( 0.7938325546108213615, -23.90362011959725663, -218.0438616059182380 ) ) ;
#21126=CARTESIAN_POINT ( 'NONE',  ( 16.84848658399567611, 11.39632653812981644, -217.9589513831453473 ) ) ;
#21127=CARTESIAN_POINT ( 'NONE',  ( -2.698926868850080041, 12.89339462271858316, -226.7595176699009585 ) ) ;
#21129=CARTESIAN_POINT ( 'NONE',  ( -16.08005950484750102, -0.1764640578214327904, -223.5999988222837942 ) ) ;
#21130=CARTESIAN_POINT ( 'NONE',  ( 3.449504654906655254, 27.59247159270940841, -231.3461799890608859 ) ) ;
#21131=CARTESIAN_POINT ( 'NONE',  ( 14.95656649340767430, 1.888692170932965597, -222.6673885184368089 ) ) ;
#21132=CARTESIAN_POINT ( 'NONE',  ( -14.34280792637948743, -22.10828917559366147, -217.4172704053049756 ) ) ;
#21133=CARTESIAN_POINT ( 'NONE',  ( 13.04434844185555420, -10.19049307777131297, -230.8679447648462713 ) ) ;
#21136=CARTESIAN_POINT ( 'NONE',  ( -12.02603758797190459, 8.152912069735307909, -218.2257190893353709 ) ) ;
#21137=CARTESIAN_POINT ( 'NONE',  ( -24.19871179313096476, -3.348666575842360160, -230.4488973568908534 ) ) ;
#21138=CARTESIAN_POINT ( 'NONE',  ( -21.19360951076126653, 12.15251088906093457, -217.9482185194656552 ) ) ;
#21139=CARTESIAN_POINT ( 'NONE',  ( 17.29648694364601980, 10.20782262162153842, -233.8400727604031317 ) ) ;
#21140=CARTESIAN_POINT ( 'NONE',  ( -1.565160934061885500, 18.19073094521525391, -232.0278805765578909 ) ) ;
#21142=CARTESIAN_POINT ( 'NONE',  ( 26.81360599170068326, -17.93330511230891844, -224.0089312182945491 ) ) ;
#21143=CARTESIAN_POINT ( 'NONE',  ( 17.00168025137501004, 6.212099629982537508, -219.0548246536471595 ) ) ;
#21144=CARTESIAN_POINT ( 'NONE',  ( -0.8357710952364670876, 15.48480697989137234, -216.9118565312697910 ) ) ;
#21145=CARTESIAN_POINT ( 'NONE',  ( -4.678665819194652187, 12.50541869316310262, -220.1509054161798247 ) ) ;
#21146=CARTESIAN_POINT ( 'NONE',  ( -13.63272521699743756, -3.226083955879493814, -228.1383267723209656 ) ) ;
#21147=CARTESIAN_POINT ( 'NONE',  ( -9.540790481621398200, 9.981116473660406996, -228.6478862620407995 ) ) ;
#21150=CARTESIAN_POINT ( 'NONE',  ( 19.63495056682994289, -4.096126682090319271, -232.1271738766904207 ) ) ;
#21151=CARTESIAN_POINT ( 'NONE',  ( -21.10507617219916199, 14.90539259013048756, -229.7677326419877488 ) ) ;
#21152=CARTESIAN_POINT ( 'NONE',  ( -16.90857133559978465, -0.4126725064255206687, -221.6276144895144569 ) ) ;
#21153=CARTESIAN_POINT ( 'NONE',  ( -14.68037037322036475, 3.441677802729143920, -220.1396515630443389 ) ) ;
#21154=CARTESIAN_POINT ( 'NONE',  ( 4.907833106823921376, 13.98151846258800290, -229.0190609869640923 ) ) ;
#21155=CARTESIAN_POINT ( 'NONE',  ( -26.09107693309126574, -10.38942742183557399, -230.9365759677854442 ) ) ;
#21156=CARTESIAN_POINT ( 'NONE',  ( 4.482815116226093188, 26.97722808566452812, -229.2080185206130238 ) ) ;
#21157=CARTESIAN_POINT ( 'NONE',  ( -5.240862053303020573, -11.96147391800445270, -224.1453450823045443 ) ) ;
#21158=CARTESIAN_POINT ( 'NONE',  ( 5.141746912158045468, 22.01688500372448232, -216.6678693612369386 ) ) ;
#21159=CARTESIAN_POINT ( 'NONE',  ( 17.14704237169575052, -19.77033640698606121, -215.4809218419665342 ) ) ;
#21160=CARTESIAN_POINT ( 'NONE',  ( 13.91172867693016890, -0.1003083830847898567, -227.9999999999999147 ) ) ;
#21162=CARTESIAN_POINT ( 'NONE',  ( -10.30870167223346456, 11.95603877111467561, -228.4123369090513336 ) ) ;
#21164=CARTESIAN_POINT ( 'NONE',  ( 23.33467929415965614, -0.4823873731835089940, -233.9427286327415629 ) ) ;
#21165=CARTESIAN_POINT ( 'NONE',  ( 3.689800395305025127, 23.07294874520714956, -219.2515233573129478 ) ) ;
#21166=CARTESIAN_POINT ( 'NONE',  ( -20.47640197314466093, 18.50423766437512541, -220.4440130802851456 ) ) ;
#21167=CARTESIAN_POINT ( 'NONE',  ( -19.86079186537285324, -0.7838168488858909821, -215.1601656726509475 ) ) ;
#21168=CARTESIAN_POINT ( 'NONE',  ( -15.89829452305285606, -16.08449805557013335, -231.9408725418336701 ) ) ;
#21169=CARTESIAN_POINT ( 'NONE',  ( 19.49137065790598555, 9.165486118354671419, -234.8706749352814995 ) ) ;
#21171=CARTESIAN_POINT ( 'NONE',  ( -0.6133843921297743584, -15.86829592205942419, -231.9438830533787268 ) ) ;
#21172=CARTESIAN_POINT ( 'NONE',  ( 3.219568897812384645, 28.82511222849302257, -221.5626884747494216 ) ) ;
#21173=CARTESIAN_POINT ( 'NONE',  ( 10.49811526528768368, 13.26166588535847701, -217.9009921269571919 ) ) ;
#21174=CARTESIAN_POINT ( 'NONE',  ( -12.70465517376339193, 12.03139199664008530, -229.6235454691090752 ) ) ;
#21176=AXIS2_PLACEMENT_3D ( 'NONE', #3767, #12778, #10863 ) ;
#21177=CARTESIAN_POINT ( 'NONE',  ( -0.4465333940385243228, 12.27026616490476485, -221.3722328744566425 ) ) ;
#21178=CARTESIAN_POINT ( 'NONE',  ( 13.14260364752544596, 5.866423290307341887, -222.7705901084601408 ) ) ;
#21180=CARTESIAN_POINT ( 'NONE',  ( 10.07328213880649592, -15.27579949576245966, -229.4560222226588451 ) ) ;
#21181=CARTESIAN_POINT ( 'NONE',  ( 7.680972971696337304, -18.49313070787806623, -217.8811398819712508 ) ) ;
#21182=CARTESIAN_POINT ( 'NONE',  ( -3.504118661534079582, 16.69899759879061918, -221.4378787282527128 ) ) ;
#21184=CARTESIAN_POINT ( 'NONE',  ( 21.53262694368047647, 11.06794636811408594, -231.8394491640143826 ) ) ;
#21185=CARTESIAN_POINT ( 'NONE',  ( 16.06750045776299629, -1.909440863493336860, -220.4398626676318713 ) ) ;
#21186=CARTESIAN_POINT ( 'NONE',  ( -13.72709560065558421, -5.132649126379569715, -227.9317987811764965 ) ) ;
#21187=CARTESIAN_POINT ( 'NONE',  ( 2.098184199980985376, -13.29281380427311099, -222.1652846463370281 ) ) ;
#21189=CARTESIAN_POINT ( 'NONE',  ( 6.729623925010410623, 16.84721552001897038, -219.9221131804260381 ) ) ;
#21191=CARTESIAN_POINT ( 'NONE',  ( 19.10353041285295816, 2.510539514498965730, -232.1135168369976896 ) ) ;
#21192=CARTESIAN_POINT ( 'NONE',  ( -9.716674560061926869, 27.56227806819028103, -219.4917914922789919 ) ) ;
#21193=CARTESIAN_POINT ( 'NONE',  ( 5.688640247940316641, 20.34961083808282822, -230.9155060479073711 ) ) ;
#21195=CARTESIAN_POINT ( 'NONE',  ( 15.37089934297015503, 20.64239674606488961, -217.2018742121147170 ) ) ;
#21196=CARTESIAN_POINT ( 'NONE',  ( -16.45414350258782221, 17.57852913985137988, -231.3969631806205598 ) ) ;
#21197=CARTESIAN_POINT ( 'NONE',  ( 14.81258087342262364, 2.398747990731791013, -230.9000679928271040 ) ) ;
#21198=CARTESIAN_POINT ( 'NONE',  ( 2.641673488600395636, -17.65289918763021149, -219.1873688300129288 ) ) ;
#21202=CARTESIAN_POINT ( 'NONE',  ( 11.82943521288609823, 27.58963564415041247, -226.1180395413371400 ) ) ;
#21203=CARTESIAN_POINT ( 'NONE',  ( -29.11561446909439965, 0.2226424683783513325, -217.8829860219008765 ) ) ;
#21205=CARTESIAN_POINT ( 'NONE',  ( -0.6367083786117293531, -29.73461014436635708, -220.1383336929387724 ) ) ;
#21207=CARTESIAN_POINT ( 'NONE',  ( -17.75316132689678383, 25.03468689048078843, -222.1645193425721061 ) ) ;
#21208=CARTESIAN_POINT ( 'NONE',  ( -6.111257124579617894, 15.89946952501658295, -216.3497764690875727 ) ) ;
#21210=CARTESIAN_POINT ( 'NONE',  ( -11.49049084071896409, 11.06834963248926940, -218.3354249205727058 ) ) ;
#21211=CARTESIAN_POINT ( 'NONE',  ( -21.14773328851117995, -13.15959238732831693, -217.2646803791660943 ) ) ;
#21214=CARTESIAN_POINT ( 'NONE',  ( -10.45786516112131892, 23.61456281964591852, -233.2869923610001592 ) ) ;
#21215=CARTESIAN_POINT ( 'NONE',  ( 6.466495776945791363, -21.72297233841655029, -216.6235280138562302 ) ) ;
#21217=CARTESIAN_POINT ( 'NONE',  ( -27.90314475660494153, 12.48829126175061077, -223.3300566725355338 ) ) ;
#21218=CARTESIAN_POINT ( 'NONE',  ( 14.65309016725241698, 3.424799466898550637, -221.5217808432381048 ) ) ;
#21219=CARTESIAN_POINT ( 'NONE',  ( 2.208705534715813101, 15.26926593729510984, -227.3643075380122980 ) ) ;
#21221=CARTESIAN_POINT ( 'NONE',  ( 14.02802030611117878, 3.063901161068346646, -225.6350222114233475 ) ) ;
#21222=CARTESIAN_POINT ( 'NONE',  ( -17.99186107021003167, -20.03292934477192944, -228.1636640080403424 ) ) ;
#21224=CARTESIAN_POINT ( 'NONE',  ( 3.291078285693179950, 23.55624334554876498, -217.3208248278388623 ) ) ;
#21225=CARTESIAN_POINT ( 'NONE',  ( -18.67270963783218463, 15.11229250701181925, -218.9067109956068578 ) ) ;
#21226=CARTESIAN_POINT ( 'NONE',  ( -8.221702953833418093, 11.87876791566348800, -223.9138461338794741 ) ) ;
#21227=CARTESIAN_POINT ( 'NONE',  ( -9.669661339602258820, -12.96780954771633532, -224.3029626631937106 ) ) ;
#21230=CARTESIAN_POINT ( 'NONE',  ( -16.20072894238734307, 0.5024448614660336210, -230.4554067149722130 ) ) ;
#21231=CARTESIAN_POINT ( 'NONE',  ( 7.513872959756128012, -15.38293111518118295, -221.6143039513618760 ) ) ;
#21232=CARTESIAN_POINT ( 'NONE',  ( 13.03557269046774714, 7.519834803053426775, -226.9490612297269081 ) ) ;
#21233=CARTESIAN_POINT ( 'NONE',  ( -2.772442535524381579, 13.75675912271027457, -228.9770533867650215 ) ) ;
#21234=CARTESIAN_POINT ( 'NONE',  ( -25.94982248293519689, 10.67899231259548287, -221.1273147719203962 ) ) ;
#21235=CARTESIAN_POINT ( 'NONE',  ( 14.02309809840729393, 19.05079204846204277, -234.6885355850075143 ) ) ;
#21237=CARTESIAN_POINT ( 'NONE',  ( 13.49011766416699842, 7.659170998773840111, -228.1905628957712793 ) ) ;
#21239=CARTESIAN_POINT ( 'NONE',  ( -13.88883449434014672, -11.15328429608096172, -217.8357414694029046 ) ) ;
#21240=CARTESIAN_POINT ( 'NONE',  ( 1.904360901363437275, -12.77109371939166138, -224.5066922355585177 ) ) ;
#21243=CARTESIAN_POINT ( 'NONE',  ( -11.79271689233719478, 3.876813423829604144, -228.6816298097564299 ) ) ;
#21244=CARTESIAN_POINT ( 'NONE',  ( 24.04182214053767908, -5.779968796880146975, -234.9365023861272164 ) ) ;
#21245=CARTESIAN_POINT ( 'NONE',  ( 5.833753951408669813, 12.47745132051510453, -226.2508980627489450 ) ) ;
#21246=CARTESIAN_POINT ( 'NONE',  ( 6.685304925496912354, 17.61973327427626046, -230.4152170797364931 ) ) ;
#21248=CARTESIAN_POINT ( 'NONE',  ( 6.498966860804143764, -11.65341448970024274, -221.3944939044252749 ) ) ;
#21249=CARTESIAN_POINT ( 'NONE',  ( 25.80927844399814930, 11.21489550116160316, -221.3538377621514996 ) ) ;
#21251=CARTESIAN_POINT ( 'NONE',  ( -4.155456637169709921, 11.30291311430030987, -225.2606024264729001 ) ) ;
#21252=CARTESIAN_POINT ( 'NONE',  ( -4.845359737286285551, 16.85396349487340117, -233.9229833851842670 ) ) ;
#21253=CARTESIAN_POINT ( 'NONE',  ( -27.06419889410506485, -1.187659473326917237, -217.6367138431444630 ) ) ;
#21254=CARTESIAN_POINT ( 'NONE',  ( -16.39453490553961856, 20.24836633112041184, -233.1722131570092245 ) ) ;
#21256=CARTESIAN_POINT ( 'NONE',  ( 27.92729748684602598, -8.572309054117944527, -222.6487661343338686 ) ) ;
#21257=AXIS2_PLACEMENT_3D ( 'NONE', #9728, #20164, #8048 ) ;
#21258=CARTESIAN_POINT ( 'NONE',  ( -4.021035526861677312, 25.02763064454595110, -216.6167103172201678 ) ) ;
#21259=CARTESIAN_POINT ( 'NONE',  ( 25.70350299105564318, 4.008313962570879241, -233.1578316763087173 ) ) ;
#21260=CARTESIAN_POINT ( 'NONE',  ( -16.63766460830045091, 5.158675778507696208, -232.1659425527909093 ) ) ;
#21261=CARTESIAN_POINT ( 'NONE',  ( 10.66614775643814994, 26.29080367171353672, -230.0818785118670178 ) ) ;
#21263=CARTESIAN_POINT ( 'NONE',  ( -4.211886032913159106, 20.62037006687756602, -216.9488349035050305 ) ) ;
#21264=CARTESIAN_POINT ( 'NONE',  ( -13.05629324012484282, -10.24599397043673221, -218.7452066004821347 ) ) ;
#21265=CARTESIAN_POINT ( 'NONE',  ( 10.50530447320976535, 20.19629329636330084, -217.1354359361034767 ) ) ;
#21266=CARTESIAN_POINT ( 'NONE',  ( 7.391697205318404684, -9.868666992833734497, -221.1858763705714068 ) ) ;
#21269=CARTESIAN_POINT ( 'NONE',  ( -12.06153928353927540, 8.661506524875534296, -226.8425068572842349 ) ) ;
#21270=SURFACE_STYLE_USAGE ( .BOTH. , #19371 ) ;
#21271=CARTESIAN_POINT ( 'NONE',  ( 24.68983475587330645, -0.6584631617853404784, -233.6195837498767958 ) ) ;
#21272=CARTESIAN_POINT ( 'NONE',  ( 2.021807401899061496, 24.17554150923399092, -230.4042646614662146 ) ) ;
#21273=CARTESIAN_POINT ( 'NONE',  ( -13.97943781666340790, 5.798109546139844639, -228.2992319913466019 ) ) ;
#21274=CARTESIAN_POINT ( 'NONE',  ( -13.09048442463468120, -0.002406630494250819839, -229.7150300986316438 ) ) ;
#21275=CARTESIAN_POINT ( 'NONE',  ( -17.60926409178586738, -17.65542935640887023, -231.2676365506119680 ) ) ;
#21276=CARTESIAN_POINT ( 'NONE',  ( 13.34963947135311102, 7.416462695144936390, -217.9359469527792044 ) ) ;
#21278=CARTESIAN_POINT ( 'NONE',  ( -16.38285517717123341, -14.67507636997927989, -214.6561055496966901 ) ) ;
#21279=CARTESIAN_POINT ( 'NONE',  ( 0.8374361358884788720, 23.73768315274483953, -232.4065959030912154 ) ) ;
#21280=CARTESIAN_POINT ( 'NONE',  ( 13.93840998928060415, 0.7705246578886114639, -220.8158265847476116 ) ) ;
#21282=CARTESIAN_POINT ( 'NONE',  ( -14.22959263369750182, 18.28478771081826793, -217.8090497856120464 ) ) ;
#21283=CARTESIAN_POINT ( 'NONE',  ( -1.584125552723561592, 20.48724127025963782, -214.7515060525244621 ) ) ;
#21284=CARTESIAN_POINT ( 'NONE',  ( -17.96792326766206926, -0.6237852504629022299, -217.9759415197746932 ) ) ;
#21285=CARTESIAN_POINT ( 'NONE',  ( -4.832117640292445060, -22.41582585812286865, -216.8192401332019870 ) ) ;
#21286=CARTESIAN_POINT ( 'NONE',  ( 15.69671663880151868, -19.77919342852767315, -217.9503656454650411 ) ) ;
#21288=CARTESIAN_POINT ( 'NONE',  ( 24.42567939027770407, 10.22651298688739097, -219.4562066833365748 ) ) ;
#21289=CARTESIAN_POINT ( 'NONE',  ( -24.78158512205813224, 1.917202307505101455, -217.2232489266994833 ) ) ;
#21290=CARTESIAN_POINT ( 'NONE',  ( -9.294226473174397540, -12.00440878504259601, -219.6990993854437875 ) ) ;
#21291=CARTESIAN_POINT ( 'NONE',  ( -18.44715843167851688, -19.86029123650958184, -231.9563062773970046 ) ) ;
#21292=CARTESIAN_POINT ( 'NONE',  ( 5.688640247940316641, 20.34961083808282822, -230.9155060479073711 ) ) ;
#21294=CARTESIAN_POINT ( 'NONE',  ( -13.34869474643618581, 6.516017165032126357, -231.2228057326931321 ) ) ;
#21295=CARTESIAN_POINT ( 'NONE',  ( -15.58461825850822180, 18.91734573546571951, -233.7691177939990723 ) ) ;
#21296=CARTESIAN_POINT ( 'NONE',  ( 6.136979247480394584, 21.37054498543370684, -230.9985475420231467 ) ) ;
#21297=CARTESIAN_POINT ( 'NONE',  ( 29.03861746756086859, -6.579333063807603743, -229.8282242506458317 ) ) ;
#21300=CARTESIAN_POINT ( 'NONE',  ( 8.592982993077152187, 10.20906991731218838, -226.0923132092261483 ) ) ;
#21301=CARTESIAN_POINT ( 'NONE',  ( -18.09605518090995702, 22.22778748761825085, -222.5443354630425290 ) ) ;
#21302=CARTESIAN_POINT ( 'NONE',  ( 29.96674103997387206, 4.060923908484647349, -228.5323681967686298 ) ) ;
#21303=CARTESIAN_POINT ( 'NONE',  ( 0.9095753368782393267, -25.50589708844611891, -231.1945442011520697 ) ) ;
#21306=CARTESIAN_POINT ( 'NONE',  ( 9.107417252317809186, 16.30291009569977234, -218.0131178633739921 ) ) ;
#21307=CARTESIAN_POINT ( 'NONE',  ( 13.24102317311734112, -10.11186274821533715, -227.6843928184991057 ) ) ;
#21308=CARTESIAN_POINT ( 'NONE',  ( -28.31595744342370580, 5.786754998807587924, -229.0820962600229223 ) ) ;
#21309=CARTESIAN_POINT ( 'NONE',  ( -2.270280637033633475, -14.48864307936496765, -230.4581659391201072 ) ) ;
#21311=CARTESIAN_POINT ( 'NONE',  ( 4.340445191644851874, 29.86837761166362881, -227.4879512554873315 ) ) ;
#21313=CARTESIAN_POINT ( 'NONE',  ( 6.839751633953758514, 19.11639828585652623, -235.1218211620789873 ) ) ;
#21315=CARTESIAN_POINT ( 'NONE',  ( -24.24202834850560606, 19.05981756344202438, -226.6980666352953335 ) ) ;
#21316=CARTESIAN_POINT ( 'NONE',  ( 29.05460218321669785, -4.534277981440765437, -222.0637325791020373 ) ) ;
#21320=CARTESIAN_POINT ( 'NONE',  ( -8.966714183099560032, 19.05224306381768073, -234.0879867025980445 ) ) ;
#21322=CARTESIAN_POINT ( 'NONE',  ( 8.082980660592431477, -16.66562551544545201, -231.4954396659114764 ) ) ;
#21324=EDGE_CURVE ( 'NONE', #11616, #4018, #3420, .T. ) ;
#21325=CARTESIAN_POINT ( 'NONE',  ( -20.18153419852512442, 14.25141268122526483, -233.5059133483111964 ) ) ;
#21326=CARTESIAN_POINT ( 'NONE',  ( -15.00242079508237936, 7.335218745534954898, -232.9526071471669013 ) ) ;
#21327=CARTESIAN_POINT ( 'NONE',  ( 4.238595127209166868, 26.19205419861516404, -230.1142052665570077 ) ) ;
#21329=CARTESIAN_POINT ( 'NONE',  ( 28.46362550855882745, 7.392895870364313282, -223.4682258299149566 ) ) ;
#21330=CARTESIAN_POINT ( 'NONE',  ( -8.696851061449722309, -24.60219662023354914, -220.1357990587600852 ) ) ;
#21332=CARTESIAN_POINT ( 'NONE',  ( 16.64575860537911112, 25.12688477742292648, -227.5050599151411745 ) ) ;
#21333=CARTESIAN_POINT ( 'NONE',  ( -12.14452111807825041, 26.21581784948545035, -221.1455569020914140 ) ) ;
#21334=CARTESIAN_POINT ( 'NONE',  ( -11.83206531956964902, 10.60028422373495260, -231.1115289952381033 ) ) ;
#21335=CARTESIAN_POINT ( 'NONE',  ( -26.50758677328550306, -10.71756779952945671, -226.4207925882492987 ) ) ;
#21338=CARTESIAN_POINT ( 'NONE',  ( -24.48580119005125866, 9.312492396273500006, -232.5498413856076070 ) ) ;
#21339=CARTESIAN_POINT ( 'NONE',  ( -9.935407011182972425, -19.19496561732008999, -215.7587022423821850 ) ) ;
#21340=CARTESIAN_POINT ( 'NONE',  ( 15.04627082534134175, 1.516717341649120865, -227.5893993471154317 ) ) ;
#21342=CARTESIAN_POINT ( 'NONE',  ( -6.474151797443945533, 21.29193859232740138, -215.9573456447696458 ) ) ;
#21343=CARTESIAN_POINT ( 'NONE',  ( 14.75092884331204957, -2.920601562751602209, -225.7127978773227426 ) ) ;
#21344=UNCERTAINTY_MEASURE_WITH_UNIT (LENGTH_MEASURE( 1.000000000000000082E-05 ), #11346, 'distance_accuracy_value', 'NONE');
#21345=CARTESIAN_POINT ( 'NONE',  ( -15.94549496081242346, -0.04271059606100771622, -224.7066567765017169 ) ) ;
#21346=CARTESIAN_POINT ( 'NONE',  ( 18.39533937270110187, 14.26564464607222504, -233.9088367426310242 ) ) ;
#21347=CARTESIAN_POINT ( 'NONE',  ( 25.33562512631297281, 12.25422971834577268, -228.6777356031426791 ) ) ;
#21349=CARTESIAN_POINT ( 'NONE',  ( -22.35595593184171292, -2.191382721379458332, -235.3044553127160441 ) ) ;
#21350=CARTESIAN_POINT ( 'NONE',  ( -8.878187501988019648, -11.23476449186280846, -221.0271673637577123 ) ) ;
#21352=CARTESIAN_POINT ( 'NONE',  ( 1.292981098121811279, -26.53499626907933262, -232.9055005154886828 ) ) ;
#21357=CARTESIAN_POINT ( 'NONE',  ( -6.702936938788568888, 25.88675107068059944, -218.1129661040884287 ) ) ;
#21358=CARTESIAN_POINT ( 'NONE',  ( 11.13603681652449318, -5.602932040673746172, -228.8141337797931101 ) ) ;
#21359=CARTESIAN_POINT ( 'NONE',  ( 15.05686526350529775, -5.555778903407086133, -220.1433349335996468 ) ) ;
#21360=CARTESIAN_POINT ( 'NONE',  ( -15.30864812529618391, 1.596444765892653717, -220.3859421844601627 ) ) ;
#21361=CARTESIAN_POINT ( 'NONE',  ( 17.31940731551425827, 24.90170669671083914, -222.9868986272316533 ) ) ;
#21362=CARTESIAN_POINT ( 'NONE',  ( 9.132190541728901323, 17.73033835127231939, -219.5524510795130766 ) ) ;
#21364=CARTESIAN_POINT ( 'NONE',  ( 5.681636183907174065, -27.87860296351749767, -230.4665658140699804 ) ) ;
#21366=CARTESIAN_POINT ( 'NONE',  ( -12.80532875684362715, 24.61139456694233374, -232.5885756414849084 ) ) ;
#21367=CARTESIAN_POINT ( 'NONE',  ( -19.61183938075907918, 22.25855138946451106, -229.5731876748794207 ) ) ;
#21368=CARTESIAN_POINT ( 'NONE',  ( -23.08212926897555306, -14.71479305961103101, -218.7697472404056214 ) ) ;
#21370=CARTESIAN_POINT ( 'NONE',  ( -23.52999999174766543, 19.39566142560855866, -221.9446938626390704 ) ) ;
#21372=CARTESIAN_POINT ( 'NONE',  ( 17.01060404384151781, -6.151862203644831162, -218.3248062500343849 ) ) ;
#21374=CARTESIAN_POINT ( 'NONE',  ( -5.762781846020777365, 12.94769902409342777, -223.1319556069387886 ) ) ;
#21375=STYLED_ITEM ( 'NONE', ( #9765 ), #20907 ) ;
#21376=CARTESIAN_POINT ( 'NONE',  ( 12.71499452845021416, 2.172589307656224378, -223.9381607050773084 ) ) ;
#21377=CARTESIAN_POINT ( 'NONE',  ( -9.749377714296398878, 10.28442384816749922, -229.3722863967025205 ) ) ;
#21378=CARTESIAN_POINT ( 'NONE',  ( 20.23125423326388628, 7.836699765464857137, -217.8891354894872450 ) ) ;
#21381=CARTESIAN_POINT ( 'NONE',  ( 5.079647427451626562, 16.77877517420371234, -220.7769382327915366 ) ) ;
#21382=CARTESIAN_POINT ( 'NONE',  ( -15.58529874627549461, -6.917566422457355202, -219.0138643999995054 ) ) ;
#21383=CARTESIAN_POINT ( 'NONE',  ( 11.87982377808925527, 10.85265283465803421, -229.5027252913499183 ) ) ;
#21384=CARTESIAN_POINT ( 'NONE',  ( -9.206457440458645891, -21.52042488620018545, -217.0715276568171248 ) ) ;
#21386=CARTESIAN_POINT ( 'NONE',  ( -22.24722865165759345, 18.77558306771206986, -226.5077042908023941 ) ) ;
#21387=CARTESIAN_POINT ( 'NONE',  ( 10.44758276073090109, -14.65753298717242714, -218.5965683461722904 ) ) ;
#21388=CARTESIAN_POINT ( 'NONE',  ( 7.249842700832647147, 18.24319783868832801, -219.1110502051974720 ) ) ;
#21389=CARTESIAN_POINT ( 'NONE',  ( -18.74633356284308761, 11.17209001323738704, -217.5809474206552068 ) ) ;
#21390=CARTESIAN_POINT ( 'NONE',  ( -13.00859847561873117, 4.399982435993697649, -231.0885370824921097 ) ) ;
#21391=CARTESIAN_POINT ( 'NONE',  ( -8.609577223708431148, -18.69066821291321290, -217.1995118692595099 ) ) ;
#21393=CARTESIAN_POINT ( 'NONE',  ( 10.85325209735074559, 11.82487774067193342, -216.5214842375702062 ) ) ;
#21395=CARTESIAN_POINT ( 'NONE',  ( -19.75796449794633602, -18.82837501718038453, -216.0857152239166794 ) ) ;
#21396=CARTESIAN_POINT ( 'NONE',  ( 3.367418898937407867, 27.20023797116225595, -219.3349021808245709 ) ) ;
#21397=CARTESIAN_POINT ( 'NONE',  ( 26.28575214971901630, 3.591103948354015696, -217.0994821834097763 ) ) ;
#21398=CARTESIAN_POINT ( 'NONE',  ( -5.762781846020777365, 12.94769902409342777, -223.1319556069387886 ) ) ;
#21399=CARTESIAN_POINT ( 'NONE',  ( 15.23494377589453919, 15.24947835004434538, -215.7641128510430519 ) ) ;
#21401=CARTESIAN_POINT ( 'NONE',  ( 1.866975752136456279, -28.95217164724439840, -224.5474425503401221 ) ) ;
#21403=CARTESIAN_POINT ( 'NONE',  ( -7.182761810198031505, -27.78193072152378207, -222.3754761716870973 ) ) ;
#21405=CARTESIAN_POINT ( 'NONE',  ( 25.18785298611088308, 3.974282393449815931, -218.7636041058819956 ) ) ;
#21406=CARTESIAN_POINT ( 'NONE',  ( 13.91151814069282722, -15.58123622716646572, -216.5183035683795367 ) ) ;
#21407=CARTESIAN_POINT ( 'NONE',  ( -19.31342342724724759, -3.870051895940637365, -217.8584481481169348 ) ) ;
#21408=CARTESIAN_POINT ( 'NONE',  ( -15.74157322273402748, -13.22745315869835636, -216.7831660370879661 ) ) ;
#21409=CARTESIAN_POINT ( 'NONE',  ( 14.61121792518381390, 23.81825453963186590, -227.9329146581663110 ) ) ;
#21411=CARTESIAN_POINT ( 'NONE',  ( -21.07387565400155438, 1.107905485989369554, -215.0000000023499069 ) ) ;
#21412=CARTESIAN_POINT ( 'NONE',  ( 0.6364901924797052857, 13.89978473517355617, -221.8840706290426397 ) ) ;
#21413=CARTESIAN_POINT ( 'NONE',  ( -0.3589900283600636066, 18.35437183075527656, -220.3960288481451357 ) ) ;
#21414=CARTESIAN_POINT ( 'NONE',  ( 28.08871713846552254, -6.057249427443905709, -231.1189077393881348 ) ) ;
#21416=CARTESIAN_POINT ( 'NONE',  ( 13.82984244654956107, 22.51831320572884820, -232.1830460045772213 ) ) ;
#21417=CARTESIAN_POINT ( 'NONE',  ( -12.01777041390050726, 10.97692933293401474, -227.6853890888168053 ) ) ;
#21418=CARTESIAN_POINT ( 'NONE',  ( -16.75232826114664775, 4.232868982398014346, -229.4158550594996200 ) ) ;
#21419=CARTESIAN_POINT ( 'NONE',  ( 6.250374750423979719, -27.98416211894771521, -222.2453514702945085 ) ) ;
#21423=CARTESIAN_POINT ( 'NONE',  ( 2.539761864897490007, 23.64215977235053501, -233.4645566207487661 ) ) ;
#21424=CARTESIAN_POINT ( 'NONE',  ( 19.27468327664662695, -19.23223527390535637, -221.0469535581208618 ) ) ;
#21425=CARTESIAN_POINT ( 'NONE',  ( -27.52457542293397097, 5.447957517019466067, -230.2717933641555135 ) ) ;
#21426=CARTESIAN_POINT ( 'NONE',  ( -13.13432812001650341, -19.42279346457301514, -216.4126494286626610 ) ) ;
#21428=CARTESIAN_POINT ( 'NONE',  ( 4.603870848087811218, 30.13529352683433515, -225.9623629403671430 ) ) ;
#21429=CARTESIAN_POINT ( 'NONE',  ( -2.218529449563984901, 24.06491599887877442, -214.8915873797660652 ) ) ;
#21431=CARTESIAN_POINT ( 'NONE',  ( -23.52999999174766543, 19.39566142560855866, -221.9446938626390704 ) ) ;
#21432=CARTESIAN_POINT ( 'NONE',  ( -22.73457989858237127, -6.881456255901889030, -216.4806380023168799 ) ) ;
#21435=CARTESIAN_POINT ( 'NONE',  ( -18.39892766464214446, 25.11039525536027739, -225.3444503920457294 ) ) ;
#21436=CARTESIAN_POINT ( 'NONE',  ( -11.08668407991722304, -24.47826551258279082, -233.9784602105897875 ) ) ;
#21437=CARTESIAN_POINT ( 'NONE',  ( 13.38839277810360429, -5.174145297632733786, -223.8523798909600941 ) ) ;
#21438=CARTESIAN_POINT ( 'NONE',  ( -17.17400284685640344, 24.63223427531467280, -220.6313524368512162 ) ) ;
#21439=CARTESIAN_POINT ( 'NONE',  ( -27.12694304224540076, 7.756125161462346540, -217.3817363082233101 ) ) ;
#21440=CARTESIAN_POINT ( 'NONE',  ( -1.248802714212398968, 14.93471382136348602, -228.4293827518713158 ) ) ;
#21441=CARTESIAN_POINT ( 'NONE',  ( -14.10849459794400751, -0.2436790717799666162, -223.1085195285415921 ) ) ;
#21442=CARTESIAN_POINT ( 'NONE',  ( -13.63442241228529994, 1.608023091903783008, -219.2326980015357094 ) ) ;
#21443=CARTESIAN_POINT ( 'NONE',  ( -11.27700245477877772, -16.92453807419676792, -219.4498264308321609 ) ) ;
#21446=CARTESIAN_POINT ( 'NONE',  ( 7.163080459435270164, 24.05253566895842354, -232.4475987112033408 ) ) ;
#21447=CARTESIAN_POINT ( 'NONE',  ( -15.77374768176864173, 20.07639682234129097, -218.6858893794192795 ) ) ;
#21448=CARTESIAN_POINT ( 'NONE',  ( -10.76972226383489506, 9.682563335906554158, -229.2555443445334333 ) ) ;
#21449=CARTESIAN_POINT ( 'NONE',  ( -21.98560163549725033, -7.841739570055646702, -218.0982455035688474 ) ) ;
#21452=CARTESIAN_POINT ( 'NONE',  ( -13.10651848559790444, 3.262242204071156948, -224.3513854875720597 ) ) ;
#21453=CARTESIAN_POINT ( 'NONE',  ( -9.899145469884247817, -15.57979392722981693, -233.4163339629578786 ) ) ;
#21454=CARTESIAN_POINT ( 'NONE',  ( 13.55929460187270053, 0.3562519042583365270, -227.9787723277739246 ) ) ;
#21455=CARTESIAN_POINT ( 'NONE',  ( -3.843007962268670585, 27.94983497691806917, -231.4302614368887703 ) ) ;
#21456=CARTESIAN_POINT ( 'NONE',  ( 14.85732601811957032, -2.750407783650710591, -223.7864485853946519 ) ) ;
#21457=CARTESIAN_POINT ( 'NONE',  ( -18.94444594796027914, 3.458349568010113728, -218.9807021659310635 ) ) ;
#21458=CARTESIAN_POINT ( 'NONE',  ( 19.20222574149634909, 21.83532798770326266, -218.6913543321078919 ) ) ;
#21459=CARTESIAN_POINT ( 'NONE',  ( 21.53262694368047647, 11.06794636811408594, -231.8394491640143826 ) ) ;
#21461=CARTESIAN_POINT ( 'NONE',  ( -21.73784594492672895, -5.247588939251936146, -214.6321000900504714 ) ) ;
#21462=CARTESIAN_POINT ( 'NONE',  ( -28.30937415889876618, -7.921132361018833556, -222.9755670691803857 ) ) ;
#21465=CARTESIAN_POINT ( 'NONE',  ( -1.243734262319729389, 14.23902626181890518, -226.4313640849764795 ) ) ;
#21466=CARTESIAN_POINT ( 'NONE',  ( 31.97344890504648518, -0.7122400102224841767, -225.1892660388073466 ) ) ;
#21467=CARTESIAN_POINT ( 'NONE',  ( 16.85953475301105442, -7.801609028127129086, -231.9437213283852941 ) ) ;
#21468=CARTESIAN_POINT ( 'NONE',  ( -21.43408368508570305, 3.680162304907783621, -233.1134812316964542 ) ) ;
#21469=CARTESIAN_POINT ( 'NONE',  ( 11.43247012502872728, 12.44034019618676190, -231.9336559008378629 ) ) ;
#21470=CARTESIAN_POINT ( 'NONE',  ( 12.84032013659066251, 19.10303921738740485, -230.8110334357214128 ) ) ;
#21472=CARTESIAN_POINT ( 'NONE',  ( 5.319567441806261066, -29.83260615907786573, -224.9444841741296841 ) ) ;
#21474=CARTESIAN_POINT ( 'NONE',  ( 4.849508625227819003, 24.02665844953846275, -214.9607406399067315 ) ) ;
#21475=CARTESIAN_POINT ( 'NONE',  ( -5.582510911615395699, 27.25430150734737111, -233.3200100877314469 ) ) ;
#21476=CARTESIAN_POINT ( 'NONE',  ( 22.35566739451469331, -4.954007294914331894, -217.4158986454943374 ) ) ;
#21477=CARTESIAN_POINT ( 'NONE',  ( -3.368164009525018265, 19.03203264544105622, -233.5986411977714567 ) ) ;
#21480=CARTESIAN_POINT ( 'NONE',  ( -6.255852670334142829, 13.96671599789818252, -220.4426911866496823 ) ) ;
#21481=CARTESIAN_POINT ( 'NONE',  ( 16.77642802340811556, -0.6192566135115280535, -218.8326447441449432 ) ) ;
#21482=CARTESIAN_POINT ( 'NONE',  ( -9.171998067665157350, 9.395241133357435714, -226.3428046914542051 ) ) ;
#21483=CARTESIAN_POINT ( 'NONE',  ( 22.46220731426537043, 18.23201731183003460, -227.5436199598787539 ) ) ;
#21484=CARTESIAN_POINT ( 'NONE',  ( -23.30703516638871875, -0.6243632158918477337, -216.1214812734271220 ) ) ;
#21487=CARTESIAN_POINT ( 'NONE',  ( -1.470815287892122125, 29.54293232078718745, -224.5855911371830302 ) ) ;
#21488=CARTESIAN_POINT ( 'NONE',  ( -12.14186164972853810, -9.217338937739926408, -220.4665480714278374 ) ) ;
#21489=CARTESIAN_POINT ( 'NONE',  ( 22.46220731426537043, 18.23201731183003460, -227.5436199598787539 ) ) ;
#21490=CARTESIAN_POINT ( 'NONE',  ( 3.979505144402133876, -26.19079129315300491, -216.2323960841296469 ) ) ;
#21492=CARTESIAN_POINT ( 'NONE',  ( -10.91003322996498071, 12.84665145358222382, -229.9786893781767958 ) ) ;
#21494=CARTESIAN_POINT ( 'NONE',  ( 12.44471834243122466, -10.90083019301730083, -219.2211511521849161 ) ) ;
#21495=CARTESIAN_POINT ( 'NONE',  ( 4.044213993247089967, 16.45246633354041421, -227.9255899743332918 ) ) ;
#21496=CARTESIAN_POINT ( 'NONE',  ( -10.02095171162140019, 11.02119725306997111, -224.1251327387667516 ) ) ;
#21497=CARTESIAN_POINT ( 'NONE',  ( -17.22166590524039265, 4.587137274468266135, -215.4863060638890033 ) ) ;
#21499=CARTESIAN_POINT ( 'NONE',  ( -17.17062072939792117, -6.705141685950851027, -229.6398969478225354 ) ) ;
#21500=CARTESIAN_POINT ( 'NONE',  ( 12.66989206167516357, 2.082990619159506007, -225.6419847029432901 ) ) ;
#21502=CARTESIAN_POINT ( 'NONE',  ( -24.71505016400469756, -15.67489082254766508, -232.1683526798342143 ) ) ;
#21503=CARTESIAN_POINT ( 'NONE',  ( -4.866400999161825780, 25.69921167300892861, -231.0100031340613782 ) ) ;
#21504=CARTESIAN_POINT ( 'NONE',  ( 21.96352831578506937, -0.3315607655626218175, -233.9427286327412787 ) ) ;
#21506=CARTESIAN_POINT ( 'NONE',  ( -6.581016643627174645, 27.50493254600863935, -230.8763182197739070 ) ) ;
#21507=CARTESIAN_POINT ( 'NONE',  ( 4.719925043692215993, 22.16918918211828782, -214.6883144083888908 ) ) ;
#21508=CARTESIAN_POINT ( 'NONE',  ( 8.467778565514151978, -25.57602835425881338, -228.7153423394380525 ) ) ;
#21510=CARTESIAN_POINT ( 'NONE',  ( -1.544051355262263225, -15.46116467022245011, -222.0171457641791903 ) ) ;
#21511=CARTESIAN_POINT ( 'NONE',  ( 26.48990917286906921, 12.16675355942207659, -225.0153622588060216 ) ) ;
#21512=CARTESIAN_POINT ( 'NONE',  ( 9.918856707546316542, -11.48950767347732871, -219.9734948840342668 ) ) ;
#21513=CARTESIAN_POINT ( 'NONE',  ( -26.07210576407111446, -8.413030596423759278, -230.6002792590230115 ) ) ;
#21514=CARTESIAN_POINT ( 'NONE',  ( -9.625604265899946554, -19.21123364792547505, -233.9327940972253259 ) ) ;
#21515=CARTESIAN_POINT ( 'NONE',  ( 6.136979247480394584, 21.37054498543370684, -230.9985475420231467 ) ) ;
#21517=CARTESIAN_POINT ( 'NONE',  ( -19.59898341672158040, 3.279988180491820504, -234.9371679595475086 ) ) ;
#21518=CARTESIAN_POINT ( 'NONE',  ( 9.586902571418640662, 24.43292817174309661, -231.9968623198229807 ) ) ;
#21519=CARTESIAN_POINT ( 'NONE',  ( 9.214796078729456497, 26.59493510027307650, -225.5796848805584318 ) ) ;
#21520=CARTESIAN_POINT ( 'NONE',  ( 16.95735638057670869, -14.83641200555466355, -235.2222363121530293 ) ) ;
#21521=CARTESIAN_POINT ( 'NONE',  ( 7.018811797190238622, 13.93862807232938472, -230.2855929063610176 ) ) ;
#21522=CARTESIAN_POINT ( 'NONE',  ( -19.33106196848021341, 9.919700385716687663, -219.0532654734256255 ) ) ;
#21523=CARTESIAN_POINT ( 'NONE',  ( -16.48591407464216729, 7.092323989942422635, -218.8909951703408012 ) ) ;
#21524=CARTESIAN_POINT ( 'NONE',  ( 1.304950495335150507, -16.28913491483048759, -229.3926418476436027 ) ) ;
#21525=B_SPLINE_CURVE_WITH_KNOTS ( 'NONE', 3,
 ( #19442, #12492, #5270, #7096, #9002, #19339, #12597, #9230, #3585, #5378, #2015, #20911, #16090, #661, #21131, #1902, #15760, #5614 ),
 .UNSPECIFIED., .F., .F.,
 ( 4, 2, 2, 2, 2, 2, 2, 2, 4 ),
 ( 0.003300329909327527622, 0.003720080272119055328, 0.004139830634910583035, 0.004559580997702110741, 0.004979331360493638448, 0.005399081723285166154, 0.005818832086076694728, 0.006238582448868222434, 0.006658332811659750140 ),
 .UNSPECIFIED. ) ;
#21528=CARTESIAN_POINT ( 'NONE',  ( 14.95414693437772868, 8.262206471704862665, -230.1862972580043163 ) ) ;
#21529=CARTESIAN_POINT ( 'NONE',  ( 21.42236089941604860, -11.78161700756472641, -230.3636358161748490 ) ) ;
#21531=CARTESIAN_POINT ( 'NONE',  ( -5.240862053303020573, -11.96147391800445270, -224.1453450823045443 ) ) ;
#21533=CARTESIAN_POINT ( 'NONE',  ( 0.9908753270255351575, 13.79205759140780430, -228.0165926715089881 ) ) ;
#21534=CARTESIAN_POINT ( 'NONE',  ( -4.365576370787875859, 13.02741211227440665, -230.2897948137907917 ) ) ;
#21536=CARTESIAN_POINT ( 'NONE',  ( -18.39892766464214446, 25.11039525536027739, -225.3444503920457294 ) ) ;
#21537=CARTESIAN_POINT ( 'NONE',  ( -27.10757994293576800, -10.52107906247675473, -229.7403242048749519 ) ) ;
#21541=CARTESIAN_POINT ( 'NONE',  ( -17.65835845419170624, 22.55329142274348442, -231.2673511165784532 ) ) ;
#21542=CARTESIAN_POINT ( 'NONE',  ( -1.366762408920091598, -18.58806247050231875, -233.7525452272278699 ) ) ;
#21543=CARTESIAN_POINT ( 'NONE',  ( 17.01060404384151781, -6.151862203644831162, -218.3248062500343849 ) ) ;
#21544=CARTESIAN_POINT ( 'NONE',  ( -11.24282496690421596, 12.44430180464951086, -232.4405891940542404 ) ) ;
#21545=CARTESIAN_POINT ( 'NONE',  ( 14.02802030611117878, 3.063901161068346646, -225.6350222114233475 ) ) ;
#21547=CARTESIAN_POINT ( 'NONE',  ( -2.665457046508036942, 16.94988614842223029, -218.7621057649994896 ) ) ;
#21549=CARTESIAN_POINT ( 'NONE',  ( 23.74723497152361062, 5.524508269105988134, -217.6012181427065002 ) ) ;
#21550=CARTESIAN_POINT ( 'NONE',  ( -18.48279503042009964, -19.02624011246567548, -221.2510238762918107 ) ) ;
#21552=CARTESIAN_POINT ( 'NONE',  ( -13.93825237094548619, 9.044872709574327985, -220.1275804576921757 ) ) ;
#21553=CARTESIAN_POINT ( 'NONE',  ( 8.821742718405863215, 10.82866050966069160, -221.4785132813277642 ) ) ;
#21554=CARTESIAN_POINT ( 'NONE',  ( 2.770531592831002143, 22.28948935999365943, -215.1307751200139649 ) ) ;
#21556=CARTESIAN_POINT ( 'NONE',  ( -15.65746202990257174, -5.535581341804817868, -220.4933418326074559 ) ) ;
#21559=CARTESIAN_POINT ( 'NONE',  ( -22.99617382825321599, 17.18101613848176967, -230.9512687019100099 ) ) ;
#21560=CARTESIAN_POINT ( 'NONE',  ( -3.294080042861979862, -13.96442541267666826, -227.2909938985368683 ) ) ;
#21562=CARTESIAN_POINT ( 'NONE',  ( -3.326157069579807946, 13.92020081821418565, -220.5733722327383930 ) ) ;
#21565=CARTESIAN_POINT ( 'NONE',  ( -21.89065952084834166, -0.9940043559354216907, -218.9999999999999716 ) ) ;
#21566=CARTESIAN_POINT ( 'NONE',  ( 11.41911493375616260, 8.796695304819765582, -229.7440655656592412 ) ) ;
#21570=CARTESIAN_POINT ( 'NONE',  ( 26.24002132888527328, 11.62331517472360964, -222.5300873157218859 ) ) ;
#21572=CARTESIAN_POINT ( 'NONE',  ( 15.00179858758994911, -7.185045179863253750, -227.1671253934038077 ) ) ;
#21573=CARTESIAN_POINT ( 'NONE',  ( -16.05483997570105714, -7.226811045751038165, -218.5819178105544438 ) ) ;
#21576=CARTESIAN_POINT ( 'NONE',  ( -1.386728072030569692, 16.52832439466973824, -230.7516952943509807 ) ) ;
#21577=CARTESIAN_POINT ( 'NONE',  ( 10.56552815906878529, -5.142824638143381755, -223.3550139360156663 ) ) ;
#21578=CARTESIAN_POINT ( 'NONE',  ( 13.38839277810360429, -5.174145297632733786, -223.8523798909600941 ) ) ;
#21579=CARTESIAN_POINT ( 'NONE',  ( -21.19360951076126653, 12.15251088906093457, -217.9482185194656552 ) ) ;
#21580=CARTESIAN_POINT ( 'NONE',  ( 13.10956039622986324, 4.581323766968698585, -221.0328522389722252 ) ) ;
#21581=CARTESIAN_POINT ( 'NONE',  ( 11.05872493453861161, 12.09300746323778775, -226.7727269015348952 ) ) ;
#21583=CARTESIAN_POINT ( 'NONE',  ( 11.73142668431994018, -22.53166313379442443, -233.8575593048731491 ) ) ;
#21585=CARTESIAN_POINT ( 'NONE',  ( -12.14471622011552832, 3.716031503296523653, -220.6237729066402835 ) ) ;
#21586=CARTESIAN_POINT ( 'NONE',  ( -4.877547524699579640, 12.94924496403020697, -219.3991240521417581 ) ) ;
#21587=CARTESIAN_POINT ( 'NONE',  ( 4.569118550756183339, 31.72363458735121000, -222.3920438419263519 ) ) ;
#21588=CARTESIAN_POINT ( 'NONE',  ( 15.22026983281163481, -5.531916908390004828, -229.4891270354009123 ) ) ;
#21589=CARTESIAN_POINT ( 'NONE',  ( -10.45786516112131892, 23.61456281964591852, -233.2869923610001592 ) ) ;
#21591=CARTESIAN_POINT ( 'NONE',  ( 2.471991688031208945, 13.88348721647344419, -230.6707754746932437 ) ) ;
#21592=CARTESIAN_POINT ( 'NONE',  ( 22.49659352743751128, 7.060662713609715979, -215.7089950799439180 ) ) ;
#21593=CARTESIAN_POINT ( 'NONE',  ( -27.90314475660494153, 12.48829126175061077, -223.3300566725355338 ) ) ;
#21594=CARTESIAN_POINT ( 'NONE',  ( 13.03557269046774714, 7.519834803053426775, -226.9490612297269081 ) ) ;
#21595=CARTESIAN_POINT ( 'NONE',  ( 6.729623925010410623, 16.84721552001897038, -219.9221131804260381 ) ) ;
#21597=CARTESIAN_POINT ( 'NONE',  ( 5.791579991237209235, 15.48299465423324861, -228.0203551130359472 ) ) ;
#21598=CARTESIAN_POINT ( 'NONE',  ( -12.13177435108894642, -8.392035797555511323, -228.8392847287196332 ) ) ;
#21599=CARTESIAN_POINT ( 'NONE',  ( 12.58590500897257947, 11.38573988265384607, -230.4867078522624695 ) ) ;
#21600=CARTESIAN_POINT ( 'NONE',  ( -0.1762641309874839746, -13.43768854674724977, -229.3744256026976416 ) ) ;
#21603=CARTESIAN_POINT ( 'NONE',  ( -10.40174557315337900, 22.75579539577861965, -231.4492192189165962 ) ) ;
#21605=CARTESIAN_POINT ( 'NONE',  ( 17.56598174185312899, -13.96259959359126768, -216.8519506175684626 ) ) ;
#21606=CARTESIAN_POINT ( 'NONE',  ( 18.75523091462765990, 19.46592657336209697, -230.4909883316157391 ) ) ;
#21607=CARTESIAN_POINT ( 'NONE',  ( -25.19248792833826300, 13.40115236862232528, -221.2817950683888455 ) ) ;
#21608=CARTESIAN_POINT ( 'NONE',  ( -11.87391433320165746, 8.920676825367966245, -232.2044275666449096 ) ) ;
#21609=CARTESIAN_POINT ( 'NONE',  ( -19.84632485794307399, -12.65249528142034485, -231.0223831579344278 ) ) ;
#21610=CARTESIAN_POINT ( 'NONE',  ( 8.373295497769937867, 8.203271496719947820, -226.1884629658694053 ) ) ;
#21613=CARTESIAN_POINT ( 'NONE',  ( -9.442378551029269929, -6.949684989614740793, -225.4111852319283855 ) ) ;
#21614=CARTESIAN_POINT ( 'NONE',  ( 2.464084843620814702, 29.35663482419208492, -227.0015060686748143 ) ) ;
#21615=CARTESIAN_POINT ( 'NONE',  ( 12.25122766587143630, 4.035812653434439845, -225.7709573147497224 ) ) ;
#21617=CARTESIAN_POINT ( 'NONE',  ( -12.33583941212908108, 22.27382123621224608, -231.6290720151527296 ) ) ;
#21618=CARTESIAN_POINT ( 'NONE',  ( 9.100443535964535258, 24.01370002727352215, -234.5397711707082635 ) ) ;
#21620=CARTESIAN_POINT ( 'NONE',  ( 7.754512012237808172, -26.66010948812077430, -222.3649102068104924 ) ) ;
#21621=CARTESIAN_POINT ( 'NONE',  ( -7.086613078029399659, -28.17108726511417771, -223.6412629831645233 ) ) ;
#21623=CARTESIAN_POINT ( 'NONE',  ( -13.00859847561873117, 4.399982435993697649, -231.0885370824921097 ) ) ;
#21624=CARTESIAN_POINT ( 'NONE',  ( 25.83609367470520723, -15.13481494965009411, -225.4685613576401124 ) ) ;
#21625=CARTESIAN_POINT ( 'NONE',  ( -22.20848920810297855, -2.028924892417935055, -232.4401719831211039 ) ) ;
#21626=CARTESIAN_POINT ( 'NONE',  ( -20.76924187596804217, -21.50248317380421170, -228.3679492147379335 ) ) ;
#21627=CARTESIAN_POINT ( 'NONE',  ( 9.425340689562565544, 25.38932416188112384, -221.3391712389563963 ) ) ;
#21629=CARTESIAN_POINT ( 'NONE',  ( 21.43345597994050777, 2.294722475943265838, -232.7243927205661294 ) ) ;
#21630=CARTESIAN_POINT ( 'NONE',  ( 4.656903975822286768, 13.45000048768594780, -227.6722060245555497 ) ) ;
#21631=CARTESIAN_POINT ( 'NONE',  ( -2.806347010929339802, 19.90767250424812573, -230.9206976900916004 ) ) ;
#21632=CARTESIAN_POINT ( 'NONE',  ( 9.163585743560105357, -20.90777124155954425, -214.7369711139705259 ) ) ;
#21633=CARTESIAN_POINT ( 'NONE',  ( 21.77183241683778547, 12.04504704525620085, -233.6005549158834640 ) ) ;
#21634=CARTESIAN_POINT ( 'NONE',  ( -18.33565906012873725, 9.491905303418088025, -219.1855745749628568 ) ) ;
#21635=CARTESIAN_POINT ( 'NONE',  ( -16.90857133559978465, -0.4126725064255206687, -221.6276144895144569 ) ) ;
#21636=CARTESIAN_POINT ( 'NONE',  ( -6.454554286546707154, -27.99704349260872149, -227.4356265632874852 ) ) ;
#21640=CARTESIAN_POINT ( 'NONE',  ( 10.55627441269396094, 10.31758739525044888, -223.1990319438957613 ) ) ;
#21641=CARTESIAN_POINT ( 'NONE',  ( 23.95414175253014477, -14.38191447464009087, -225.3623377062671125 ) ) ;
#21642=CARTESIAN_POINT ( 'NONE',  ( -29.22672729369577738, 6.588740615114764054, -224.9915299386302934 ) ) ;
#21644=CARTESIAN_POINT ( 'NONE',  ( -12.42894476027428929, -17.97759322220185396, -216.3110355466728834 ) ) ;
#21647=CARTESIAN_POINT ( 'NONE',  ( -3.060450601941519189, 13.29454208326677289, -222.0135664617158682 ) ) ;
#21648=CARTESIAN_POINT ( 'NONE',  ( -4.678665819194652187, 12.50541869316310262, -220.1509054161798247 ) ) ;
#21650=CARTESIAN_POINT ( 'NONE',  ( -4.620781219515533778, 16.99182040716223696, -217.1278208835672672 ) ) ;
#21651=CARTESIAN_POINT ( 'NONE',  ( -30.78084016402396372, -2.501288241119758116, -224.5721874330603214 ) ) ;
#21654=CARTESIAN_POINT ( 'NONE',  ( -4.620781219515533778, 16.99182040716223696, -217.1278208835672672 ) ) ;
#21656=CARTESIAN_POINT ( 'NONE',  ( -4.737391463177558215, -17.33199396152823368, -215.7912354007318925 ) ) ;
#21658=CARTESIAN_POINT ( 'NONE',  ( 25.46470895113276711, -14.41152162994631070, -228.1811935238409035 ) ) ;
#21659=CARTESIAN_POINT ( 'NONE',  ( -6.474151797443945533, 21.29193859232740138, -215.9573456447696458 ) ) ;
#21661=CARTESIAN_POINT ( 'NONE',  ( -26.47501633019681577, 13.84484755257420119, -230.0154374881822719 ) ) ;
#21662=CARTESIAN_POINT ( 'NONE',  ( 0.7903203334012884884, 21.30772501796948859, -217.9064416298261619 ) ) ;
#21663=CARTESIAN_POINT ( 'NONE',  ( -14.29986196492902550, 0.06805469746732484282, -227.4167624117703213 ) ) ;
#21664=CARTESIAN_POINT ( 'NONE',  ( 13.71585692689473213, 6.523039003617190801, -224.4540437369149402 ) ) ;
#21665=CARTESIAN_POINT ( 'NONE',  ( -9.669661339602258820, -12.96780954771633532, -224.3029626631937106 ) ) ;
#21667=CARTESIAN_POINT ( 'NONE',  ( -9.954421844142357756, 11.21484508112568079, -226.0177122452137439 ) ) ;
#21668=CARTESIAN_POINT ( 'NONE',  ( 16.69977105456987232, 16.51652889326612694, -233.6667933521891030 ) ) ;
#21669=CARTESIAN_POINT ( 'NONE',  ( -0.1452471002967452851, 24.29564289358754081, -234.0861481044164805 ) ) ;
#21670=CARTESIAN_POINT ( 'NONE',  ( -29.43130594997593974, -3.977420319584657360, -224.3854249914923571 ) ) ;
#21673=CARTESIAN_POINT ( 'NONE',  ( -10.30050448363967419, 10.07750059423401190, -220.1837019037183723 ) ) ;
#21674=CARTESIAN_POINT ( 'NONE',  ( -13.06588638656279322, -26.69120070130052014, -220.2265807429280642 ) ) ;
#21675=CARTESIAN_POINT ( 'NONE',  ( 10.85888002857596923, 15.81835858589122878, -232.3913150909872627 ) ) ;
#21679=CARTESIAN_POINT ( 'NONE',  ( -23.43012680803641956, 15.46310457140252304, -230.0052977649806962 ) ) ;
#21680=CARTESIAN_POINT ( 'NONE',  ( 8.343316395906509086, 11.57404413652245800, -231.1403332574589911 ) ) ;
#21683=CARTESIAN_POINT ( 'NONE',  ( 21.25094435758043332, 17.68230636442804027, -229.7964888993842010 ) ) ;
#21685=CARTESIAN_POINT ( 'NONE',  ( -22.13988250630526267, 1.271659148212506141, -215.1660654604927458 ) ) ;
#21686=CARTESIAN_POINT ( 'NONE',  ( -25.10035252441274167, -15.33546242866430198, -228.3913311683031964 ) ) ;
#21689=CARTESIAN_POINT ( 'NONE',  ( -4.824452364631481416, 22.01523768541901305, -216.8350837474290245 ) ) ;
#21690=CARTESIAN_POINT ( 'NONE',  ( 12.55122320111375700, -1.519965464208375749, -221.0350040576933281 ) ) ;
#21692=CARTESIAN_POINT ( 'NONE',  ( 23.44296991241933981, -12.51566675729016964, -231.4065378011870564 ) ) ;
#21693=CARTESIAN_POINT ( 'NONE',  ( -14.07336028695978314, 1.752429266630609828, -222.9750305084206161 ) ) ;
#21694=CARTESIAN_POINT ( 'NONE',  ( 26.28575214971901630, 3.591103948354015696, -217.0994821834097763 ) ) ;
#21695=CARTESIAN_POINT ( 'NONE',  ( 10.01015180241662605, 20.19019600914695900, -219.1042218506083543 ) ) ;
#21697=CARTESIAN_POINT ( 'NONE',  ( -0.5904090961472509003, -15.19049578300894510, -228.4387523405810612 ) ) ;
#21699=CARTESIAN_POINT ( 'NONE',  ( -31.04415783139704388, 5.868882651865275690, -221.1472518903637194 ) ) ;
#21700=CARTESIAN_POINT ( 'NONE',  ( 7.174260007897984792, 9.971262771497068300, -226.2872513832048469 ) ) ;
#21701=CARTESIAN_POINT ( 'NONE',  ( 4.849508625227819003, 24.02665844953846275, -214.9607406399067315 ) ) ;
#21702=CARTESIAN_POINT ( 'NONE',  ( 17.78250599636351481, -9.160802950715318360, -218.6762383290621869 ) ) ;
#21703=CARTESIAN_POINT ( 'NONE',  ( 0.9046320824004248085, 13.39785254849979701, -226.4815711199935890 ) ) ;
#21704=CARTESIAN_POINT ( 'NONE',  ( -13.69675006931110417, 3.702342960760605539, -228.0723273272095355 ) ) ;
#21705=CARTESIAN_POINT ( 'NONE',  ( 11.31331191788792623, 29.23420701778062281, -220.7538464529627333 ) ) ;
#21706=CARTESIAN_POINT ( 'NONE',  ( -25.11055959288653128, 8.701823109978603199, -230.2231080656787583 ) ) ;
#21707=CARTESIAN_POINT ( 'NONE',  ( -19.00318367631585659, 13.14621133775862916, -233.8403879275295765 ) ) ;
#21709=CARTESIAN_POINT ( 'NONE',  ( 28.02123297569005089, 5.903198806000402143, -227.5759114383273811 ) ) ;
#21710=CARTESIAN_POINT ( 'NONE',  ( 3.635089269978064141, 27.05650967970794341, -222.4639105745756638 ) ) ;
#21713=CARTESIAN_POINT ( 'NONE',  ( 11.21155440434494643, 24.57152134148167733, -221.7155903571010356 ) ) ;
#21714=CARTESIAN_POINT ( 'NONE',  ( -11.07688804854283049, -12.81333559660784971, -232.1241261852632363 ) ) ;
#21715=CARTESIAN_POINT ( 'NONE',  ( 16.38151749656409351, 8.902090001712490874, -231.2955017965201989 ) ) ;
#21716=CARTESIAN_POINT ( 'NONE',  ( -9.132447960227011663, -28.48575439045284696, -228.2342138548108892 ) ) ;
#21718=CARTESIAN_POINT ( 'NONE',  ( -4.742143146070755932, 15.01230778631049567, -221.4832709320255049 ) ) ;
#21719=CARTESIAN_POINT ( 'NONE',  ( 10.62272209279942992, -9.818939940036045755, -222.1403336352628344 ) ) ;
#21720=CARTESIAN_POINT ( 'NONE',  ( 25.40172858355122898, 15.07073195964820833, -229.0276483847865450 ) ) ;
#21721=CARTESIAN_POINT ( 'NONE',  ( -7.250603130619442283, 20.89725557392719324, -217.7893896917081520 ) ) ;
#21722=CARTESIAN_POINT ( 'NONE',  ( -21.85741505224184777, 1.741064654082184582, -235.1654459941842390 ) ) ;
#21723=CARTESIAN_POINT ( 'NONE',  ( -18.47336874364275516, -4.831184938305232990, -219.8627234292127639 ) ) ;
#21724=CARTESIAN_POINT ( 'NONE',  ( 14.17826651990317188, -1.167225063855702683, -222.4240311848849387 ) ) ;
#21726=( GEOMETRIC_REPRESENTATION_CONTEXT ( 3 ) GLOBAL_UNCERTAINTY_ASSIGNED_CONTEXT ( ( #875 ) ) GLOBAL_UNIT_ASSIGNED_CONTEXT ( ( #1097, #13032, #4802 ) ) REPRESENTATION_CONTEXT ( 'NONE', 'WORKASPACE' ) );
#21728=CARTESIAN_POINT ( 'NONE',  ( -30.46088052942827318, -8.161173215405806758, -225.9185547777119893 ) ) ;
#21729=CARTESIAN_POINT ( 'NONE',  ( 21.26803326031697949, 19.54255073453192892, -230.5813148908474659 ) ) ;
#21730=CARTESIAN_POINT ( 'NONE',  ( 24.81079154715000357, 3.171651085595392772, -216.4177249688571578 ) ) ;
#21731=CARTESIAN_POINT ( 'NONE',  ( 3.001892273201697048, 27.20292285420111966, -216.7800154582108689 ) ) ;
#21732=CARTESIAN_POINT ( 'NONE',  ( 7.587775680576782200, 20.81864918083767435, -235.2547171215352364 ) ) ;
#21734=CARTESIAN_POINT ( 'NONE',  ( 4.834917880317126659, -18.50358955815650219, -219.1181532354089256 ) ) ;
#21736=CARTESIAN_POINT ( 'NONE',  ( -7.180402128846711918, -26.42159752827261698, -220.2116303544826224 ) ) ;
#21737=CARTESIAN_POINT ( 'NONE',  ( -12.61443312487471324, 8.399394471292156439, -217.5740162615319093 ) ) ;
#21738=CARTESIAN_POINT ( 'NONE',  ( 9.104026917753444081, -10.66572815660443041, -221.9193219976906448 ) ) ;
#21739=CARTESIAN_POINT ( 'NONE',  ( -16.20471097821853235, -2.781505378741172319, -220.1484675126197317 ) ) ;
#21741=CARTESIAN_POINT ( 'NONE',  ( -11.28700884291539630, -21.85791790461604478, -233.5354093188319951 ) ) ;
#21743=CARTESIAN_POINT ( 'NONE',  ( 11.83256327006771969, 5.988634687709346593, -225.8999299265561831 ) ) ;
#21745=CARTESIAN_POINT ( 'NONE',  ( -11.07173923371951574, 9.938770595667456575, -229.9381419817434562 ) ) ;
#21746=CARTESIAN_POINT ( 'NONE',  ( 19.61276001257277102, 19.97122404150989894, -229.5162757829903342 ) ) ;
#21747=CARTESIAN_POINT ( 'NONE',  ( 11.13678936984666912, 26.95732789089726111, -228.8350761760834757 ) ) ;
#21748=CARTESIAN_POINT ( 'NONE',  ( 16.97369223523349646, 15.19068754808448851, -217.0779026324121332 ) ) ;
#21749=CARTESIAN_POINT ( 'NONE',  ( 7.391697205318404684, -9.868666992833734497, -221.1858763705714068 ) ) ;
#21750=CARTESIAN_POINT ( 'NONE',  ( 25.38325563848796662, 11.05100313887457553, -217.8685524735130628 ) ) ;
#21751=CARTESIAN_POINT ( 'NONE',  ( -9.679547659771646551, 14.60131434979866505, -230.4338124916943968 ) ) ;
#21752=CARTESIAN_POINT ( 'NONE',  ( -13.01444359484612079, -23.32256785062423887, -219.1545357706015693 ) ) ;
#21753=CARTESIAN_POINT ( 'NONE',  ( -20.94800339253696109, 4.477632454355491731, -216.5423208360950298 ) ) ;
#21755=CARTESIAN_POINT ( 'NONE',  ( 24.57222455393806015, 12.08236629421828212, -229.7319216558644541 ) ) ;
#21756=CARTESIAN_POINT ( 'NONE',  ( 23.31955656579280145, -13.39010844438576520, -228.3495985225334266 ) ) ;
#21760=CARTESIAN_POINT ( 'NONE',  ( -2.576162127940193169, -15.57202066281789321, -231.6911579627040396 ) ) ;
#21761=CARTESIAN_POINT ( 'NONE',  ( -3.673551555920188783, 29.81207051619892923, -228.8770490300152005 ) ) ;
#21762=CARTESIAN_POINT ( 'NONE',  ( -4.877547524699579640, 12.94924496403020697, -219.3991240521417581 ) ) ;
#21764=CARTESIAN_POINT ( 'NONE',  ( 0.9908753270255351575, 13.79205759140780430, -228.0165926715089881 ) ) ;
#21765=CARTESIAN_POINT ( 'NONE',  ( -16.30907414568449454, -3.310091733494833655, -231.8954501777161283 ) ) ;
#21768=CARTESIAN_POINT ( 'NONE',  ( 5.248230734842167955, 23.54336384919183445, -216.8914391693808739 ) ) ;
#21769=CARTESIAN_POINT ( 'NONE',  ( -13.66010072360327676, -23.28416639572314750, -215.9262288161416166 ) ) ;
#21770=CARTESIAN_POINT ( 'NONE',  ( 15.65513449100897780, -26.00057195821942457, -227.4103383097017570 ) ) ;
#21771=CARTESIAN_POINT ( 'NONE',  ( 15.54083024098960486, -10.44392130763852222, -217.6620978190037476 ) ) ;
#21772=CARTESIAN_POINT ( 'NONE',  ( -12.33997807949817904, 15.01940705987184188, -217.6798968600957380 ) ) ;
#21774=CARTESIAN_POINT ( 'NONE',  ( 8.312165662451315384, 13.84431584962456974, -225.8109542921768025 ) ) ;
#21775=CARTESIAN_POINT ( 'NONE',  ( -26.02440924314744919, 2.824604386891162111, -232.0644005296583430 ) ) ;
#21776=CARTESIAN_POINT ( 'NONE',  ( -21.12280458060320498, 13.61074013710079988, -216.5529903464332335 ) ) ;
#21777=CARTESIAN_POINT ( 'NONE',  ( -25.45695634607983848, -10.72451519803311015, -228.5848280742264933 ) ) ;
#21780=CARTESIAN_POINT ( 'NONE',  ( -17.99720854823001659, 13.97888873227035056, -232.2992184661552244 ) ) ;
#21781=CARTESIAN_POINT ( 'NONE',  ( 3.846342036506673612, 16.55327908958690131, -231.1358846258000597 ) ) ;
#21782=CARTESIAN_POINT ( 'NONE',  ( -5.590964611773372894, 13.92546790642523113, -228.7941110425196882 ) ) ;
#21783=CARTESIAN_POINT ( 'NONE',  ( -26.75342641616541783, -10.60804028525731546, -225.2137697103424898 ) ) ;
#21786=CARTESIAN_POINT ( 'NONE',  ( -15.58461825850822180, 18.91734573546571951, -233.7691177939990723 ) ) ;
#21787=CARTESIAN_POINT ( 'NONE',  ( -2.916193397327769166, -13.79856165086501107, -222.9033574188488842 ) ) ;
#21788=CARTESIAN_POINT ( 'NONE',  ( 14.73698509926073186, 4.443590625350892331, -227.4062002049096236 ) ) ;
#21789=CARTESIAN_POINT ( 'NONE',  ( 17.68508104102419409, 23.41266195669770767, -227.5327139115408954 ) ) ;
#21793=CARTESIAN_POINT ( 'NONE',  ( -14.30096418567650041, 6.974026439069829664, -228.7941652905285537 ) ) ;
#21794=CARTESIAN_POINT ( 'NONE',  ( 17.89221702206198117, 0.2742047965568425449, -220.2420650470893122 ) ) ;
#21799=CARTESIAN_POINT ( 'NONE',  ( 17.22969587606878505, -8.834803756807117381, -230.2348533348707917 ) ) ;
#21800=CARTESIAN_POINT ( 'NONE',  ( -25.98129645912436914, -15.13773040547512139, -224.1390156429105787 ) ) ;
#21803=CARTESIAN_POINT ( 'NONE',  ( 5.248013545904832711, 18.51731616863089158, -219.3673127389703552 ) ) ;
#21804=CARTESIAN_POINT ( 'NONE',  ( 18.59830189133340639, -20.05840858737748533, -233.4490516770458157 ) ) ;
#21805=CARTESIAN_POINT ( 'NONE',  ( 28.52058947142581502, -1.755848367977142610, -221.9695116608532715 ) ) ;
#21806=CARTESIAN_POINT ( 'NONE',  ( -17.39737143130126285, 7.531548707695031375, -232.0788227848755696 ) ) ;
#21807=CARTESIAN_POINT ( 'NONE',  ( -15.83894155097017631, 1.950284868793920712, -224.5615909987450038 ) ) ;
#21808=CARTESIAN_POINT ( 'NONE',  ( 13.38540196930496862, 9.639609424068478205, -227.8779021328794840 ) ) ;
#21810=CARTESIAN_POINT ( 'NONE',  ( 10.42186625103445152, -25.39807580958450473, -217.7675295214572202 ) ) ;
#21812=CARTESIAN_POINT ( 'NONE',  ( -30.66857674073067130, 4.440060741118782239, -229.9901150862898476 ) ) ;
#21813=CARTESIAN_POINT ( 'NONE',  ( 3.764125772070460396, 11.78312483992801596, -228.3484643988637970 ) ) ;
#21814=CARTESIAN_POINT ( 'NONE',  ( 4.754245974719506940, 31.05377813473586102, -220.6166503949300193 ) ) ;
#21815=CARTESIAN_POINT ( 'NONE',  ( 13.86395146404758982, -8.823451364178625411, -228.3963352256065491 ) ) ;
#21816=CARTESIAN_POINT ( 'NONE',  ( -3.755296588130283553, 23.77975947300719284, -233.7323173085780752 ) ) ;
#21817=CARTESIAN_POINT ( 'NONE',  ( -27.90314475660494153, 12.48829126175061077, -223.3300566725355338 ) ) ;
#21818=CARTESIAN_POINT ( 'NONE',  ( 13.32754126089433377, 12.31312334927721963, -234.6033665822900218 ) ) ;
#21819=CARTESIAN_POINT ( 'NONE',  ( -15.54392142943450317, 6.670312097614393920, -219.6934017696036676 ) ) ;
#21820=CARTESIAN_POINT ( 'NONE',  ( -2.698926868850080041, 12.89339462271858316, -226.7595176699009585 ) ) ;
#21821=CARTESIAN_POINT ( 'NONE',  ( 22.02796522526679723, 16.41909032291435366, -220.1590600991317217 ) ) ;
#21822=CARTESIAN_POINT ( 'NONE',  ( 14.61121792518381390, 23.81825453963186590, -227.9329146581663110 ) ) ;
#21823=CARTESIAN_POINT ( 'NONE',  ( 23.36729170583618398, -5.500043712341283531, -232.1593072787115375 ) ) ;
#21826=CARTESIAN_POINT ( 'NONE',  ( -14.93108815068229589, -1.792787290847115633, -227.6165763581034582 ) ) ;
#21827=CARTESIAN_POINT ( 'NONE',  ( 10.78187269046063435, 10.73871010366167944, -221.9206544238666368 ) ) ;
#21828=CARTESIAN_POINT ( 'NONE',  ( -9.447593206125553422, -28.82180577676834332, -226.7547558591687675 ) ) ;
#21830=CARTESIAN_POINT ( 'NONE',  ( -11.03778527004271659, 26.96286968643956428, -225.4057095641571209 ) ) ;
#21831=CARTESIAN_POINT ( 'NONE',  ( 13.66436340482409761, -13.84785698770488871, -232.6553000701566134 ) ) ;
#21832=CARTESIAN_POINT ( 'NONE',  ( 16.43556216695724004, 8.397919695511960825, -216.7971521583719152 ) ) ;
#21833=CARTESIAN_POINT ( 'NONE',  ( -8.317278876689359279, 23.15034512777772235, -218.2935523245793092 ) ) ;
#21834=CARTESIAN_POINT ( 'NONE',  ( -5.861205904341304951, 14.21969934012253312, -219.3213214613830644 ) ) ;
#21836=CARTESIAN_POINT ( 'NONE',  ( -19.26019478805205054, -16.72235099301716943, -219.5158537523224993 ) ) ;
#21837=CARTESIAN_POINT ( 'NONE',  ( 30.65249971456167799, 3.724008896938769464, -225.4815109119605552 ) ) ;
#21838=CARTESIAN_POINT ( 'NONE',  ( -13.36635042947306573, -0.3940246778032021058, -227.3384152261055249 ) ) ;
#21839=CARTESIAN_POINT ( 'NONE',  ( 18.81274554574540403, 10.85963742466947224, -234.0446454529665345 ) ) ;
#21840=CARTESIAN_POINT ( 'NONE',  ( -21.26441444091935296, 10.69428164102106926, -219.3434466924981336 ) ) ;
#21841=CARTESIAN_POINT ( 'NONE',  ( 1.220475224794998370, 29.83033731899746144, -230.4224274340063801 ) ) ;
#21842=CARTESIAN_POINT ( 'NONE',  ( 8.343316395906509086, 11.57404413652245800, -231.1403332574589911 ) ) ;
#21844=CARTESIAN_POINT ( 'NONE',  ( -16.91104737563547644, -22.20641354538343748, -232.3619262256263482 ) ) ;
#21847=CARTESIAN_POINT ( 'NONE',  ( 4.002939343642331949, -22.37368820207002429, -217.8631878264377804 ) ) ;
#21849=CARTESIAN_POINT ( 'NONE',  ( -11.10150084103673684, 3.549415896002023896, -226.0408865487038952 ) ) ;
#21850=CARTESIAN_POINT ( 'NONE',  ( 23.44296991241933981, -12.51566675729016964, -231.4065378011870564 ) ) ;
#21851=CARTESIAN_POINT ( 'NONE',  ( -14.73155177304599306, -1.817590056890399763, -226.9769936995019748 ) ) ;
#21852=CARTESIAN_POINT ( 'NONE',  ( -13.67406442719345883, -9.319000780081536206, -231.1492214949047934 ) ) ;
#21853=CARTESIAN_POINT ( 'NONE',  ( 15.74259730902452858, 17.40808440793174583, -232.1327802909178786 ) ) ;
#21855=CARTESIAN_POINT ( 'NONE',  ( -8.548213857283494477, 12.07277636836182211, -222.5354997492170241 ) ) ;
#21856=CARTESIAN_POINT ( 'NONE',  ( 10.25308675723727347, 13.16459519580956972, -229.3963488176951273 ) ) ;
#21857=CARTESIAN_POINT ( 'NONE',  ( -3.843007962268670585, 27.94983497691806917, -231.4302614368887703 ) ) ;
#21858=CARTESIAN_POINT ( 'NONE',  ( 10.14297843322460402, 14.69845403004500639, -219.2805000163441207 ) ) ;
#21859=CARTESIAN_POINT ( 'NONE',  ( 27.54866699188204748, -16.08959018098719085, -223.7550031907416326 ) ) ;
#21860=CARTESIAN_POINT ( 'NONE',  ( -10.46043650402819125, 8.998596506756641134, -222.4402691847174083 ) ) ;
#21861=CARTESIAN_POINT ( 'NONE',  ( -5.786930954831501772, 15.78543306641166311, -231.0475152612371517 ) ) ;
#21862=CARTESIAN_POINT ( 'NONE',  ( -17.81508947870519322, -18.77243306401324219, -218.1930932538018340 ) ) ;
#21865=CARTESIAN_POINT ( 'NONE',  ( 15.42212722119060864, 5.401662248084913465, -220.8333402320903645 ) ) ;
#21866=CARTESIAN_POINT ( 'NONE',  ( 14.47405021949252557, -20.16114635186222159, -231.2055612633458566 ) ) ;
#21867=CARTESIAN_POINT ( 'NONE',  ( -16.74094048923576494, 16.03040267675914521, -217.9177456399057178 ) ) ;
#21869=CARTESIAN_POINT ( 'NONE',  ( 2.808299412262623473, 18.06245856371233316, -217.9832661743849656 ) ) ;
#21870=CARTESIAN_POINT ( 'NONE',  ( -11.36971918743327237, -8.287084598727400220, -223.1364763414170227 ) ) ;
#21872=CARTESIAN_POINT ( 'NONE',  ( -24.48812334466693486, 4.469247780253509106, -230.3044243311433945 ) ) ;
#21873=CARTESIAN_POINT ( 'NONE',  ( 14.02309809840729393, 19.05079204846204277, -234.6885355850075143 ) ) ;
#21875=CARTESIAN_POINT ( 'NONE',  ( 4.603870848087811218, 30.13529352683433515, -225.9623629403671430 ) ) ;
#21876=CARTESIAN_POINT ( 'NONE',  ( 22.50501984129641286, -15.15275112778533284, -228.8333022290248664 ) ) ;
#21879=CARTESIAN_POINT ( 'NONE',  ( 4.340445191644851874, 29.86837761166362881, -227.4879512554873315 ) ) ;
#21880=CARTESIAN_POINT ( 'NONE',  ( -8.215923615656011592, -19.99105411527736820, -235.1422105638354481 ) ) ;
#21881=CARTESIAN_POINT ( 'NONE',  ( 1.752757082432757185, -17.15725705531007250, -232.7539178101738742 ) ) ;
#21883=CARTESIAN_POINT ( 'NONE',  ( -9.982417347796181062, 8.907629238417765549, -225.5124013436514474 ) ) ;
#21884=CARTESIAN_POINT ( 'NONE',  ( 8.961491954973460849, 17.27041174997091844, -219.7661252763212474 ) ) ;
#21885=CARTESIAN_POINT ( 'NONE',  ( -29.95012366401462955, 4.746560250930182967, -224.6954343660969471 ) ) ;
#21886=CARTESIAN_POINT ( 'NONE',  ( -21.29946384424354733, 21.01772963953914442, -222.5871995662667757 ) ) ;
#21887=CARTESIAN_POINT ( 'NONE',  ( -20.80379704402785990, -7.385557752804055909, -217.9407440132496845 ) ) ;
#21889=CARTESIAN_POINT ( 'NONE',  ( -10.70754874174748039, 23.84972878377777405, -230.7991598016655246 ) ) ;
#21890=CARTESIAN_POINT ( 'NONE',  ( 12.88374853655145458, 4.106359831454843068, -228.1016120772327440 ) ) ;
#21891=CARTESIAN_POINT ( 'NONE',  ( 2.804048525646705148, 30.59371477727813726, -220.6614663749232363 ) ) ;
#21892=CARTESIAN_POINT ( 'NONE',  ( 17.56598174185312899, -13.96259959359126768, -216.8519506175684626 ) ) ;
#21895=CARTESIAN_POINT ( 'NONE',  ( -25.80904414196669450, 12.19501778665756220, -219.1732313092283846 ) ) ;
#21896=CARTESIAN_POINT ( 'NONE',  ( -12.51550321509044927, -6.200974036110347143, -231.2371560537167170 ) ) ;
#21898=CARTESIAN_POINT ( 'NONE',  ( 8.496844655769807630, 14.66037471857024599, -219.1631158796573118 ) ) ;
#21900=CARTESIAN_POINT ( 'NONE',  ( 14.90979066288448429, -1.927202206923867234, -222.7790985701595616 ) ) ;
#21902=CARTESIAN_POINT ( 'NONE',  ( -13.98136146596813845, 3.850743984385103680, -228.7620665878280590 ) ) ;
#21903=CARTESIAN_POINT ( 'NONE',  ( -11.39536650977235510, 9.246300577217761330, -228.4898727004871546 ) ) ;
#21904=CARTESIAN_POINT ( 'NONE',  ( 17.47660375112063491, 0.1533180678384444551, -220.6249646429494931 ) ) ;
#21905=( NAMED_UNIT ( * ) SI_UNIT ( $, .STERADIAN. ) SOLID_ANGLE_UNIT ( ) );
#21906=CARTESIAN_POINT ( 'NONE',  ( 15.41510009650066770, 0.5889348971793676446, -222.0565507956523277 ) ) ;
#21907=CARTESIAN_POINT ( 'NONE',  ( 18.46552355142154411, 5.019711608606525211, -231.5099115070375433 ) ) ;
#21908=CARTESIAN_POINT ( 'NONE',  ( -21.89482327431018760, 1.733733432562314158, -233.1353281693111796 ) ) ;
#21909=CARTESIAN_POINT ( 'NONE',  ( 15.34439776706934921, -6.609831973102724412, -222.6284221295667862 ) ) ;
#21910=CARTESIAN_POINT ( 'NONE',  ( -28.18501077041064562, -8.523171531337160545, -227.0531053546762337 ) ) ;
#21913=CARTESIAN_POINT ( 'NONE',  ( 0.07890756785233743464, 25.14108539708653822, -218.4152285319504756 ) ) ;
#21914=CARTESIAN_POINT ( 'NONE',  ( 13.82710435306955432, -11.68840971183345800, -215.7775723145259974 ) ) ;
#21915=CARTESIAN_POINT ( 'NONE',  ( 6.260999666360449467, -13.19315344885661645, -220.2890618333529744 ) ) ;
#21916=CARTESIAN_POINT ( 'NONE',  ( -13.51406939156936104, 10.04301168678160749, -230.1761202643687056 ) ) ;
#21917=CARTESIAN_POINT ( 'NONE',  ( 17.91327661571172314, 1.545939370248587075, -216.9938266089438912 ) ) ;
#21918=CARTESIAN_POINT ( 'NONE',  ( 16.26115440404298340, 3.800605480264513059, -219.2833057824682612 ) ) ;
#21920=CARTESIAN_POINT ( 'NONE',  ( -1.178362239076253370, -26.64461120719161613, -230.8441371545519019 ) ) ;
#21922=CARTESIAN_POINT ( 'NONE',  ( -23.68377094563794572, 13.02263794644603578, -215.9752901280847652 ) ) ;
#21923=CARTESIAN_POINT ( 'NONE',  ( 7.803634760976553508, 10.78293796201124266, -229.6314106675118865 ) ) ;
#21924=CARTESIAN_POINT ( 'NONE',  ( -0.04850409037381671340, 14.20520396026658716, -231.8092226852533031 ) ) ;
#21925=CARTESIAN_POINT ( 'NONE',  ( 23.00003818093501806, -2.342406833639917085, -233.2756072794339843 ) ) ;
#21926=CARTESIAN_POINT ( 'NONE',  ( 5.069241901512100412, 14.34986542013820632, -229.6420000777802954 ) ) ;
#21927=CARTESIAN_POINT ( 'NONE',  ( -18.46722752239034193, 0.9784074152395518809, -232.1633353206286188 ) ) ;
#21929=CARTESIAN_POINT ( 'NONE',  ( 9.169328349715531346, 20.85917603618721472, -214.7000934853629133 ) ) ;
#21930=CARTESIAN_POINT ( 'NONE',  ( -17.91550223652134122, 4.809113705933536487, -230.6324822114035555 ) ) ;
#21931=CARTESIAN_POINT ( 'NONE',  ( -10.45786516112131892, 23.61456281964591852, -233.2869923610001592 ) ) ;
#21932=CARTESIAN_POINT ( 'NONE',  ( 15.01439307471096463, 1.118969480519667048, -226.7488225241675366 ) ) ;
#21933=CARTESIAN_POINT ( 'NONE',  ( 15.28499842775873319, 22.98894588155567931, -221.0942409093412095 ) ) ;
#21936=CARTESIAN_POINT ( 'NONE',  ( -17.92628912275201003, -0.6090139417824500523, -215.7724435048976943 ) ) ;
#21937=CARTESIAN_POINT ( 'NONE',  ( -14.27403737459813193, -10.90264666745762057, -220.2309642783388597 ) ) ;
#21939=CARTESIAN_POINT ( 'NONE',  ( -9.233762381136051189, 19.18161952504991419, -232.0796851897838451 ) ) ;
#21941=CARTESIAN_POINT ( 'NONE',  ( 6.869068212838696397, -24.78254998730118430, -231.2855974421026986 ) ) ;
#21942=CARTESIAN_POINT ( 'NONE',  ( 23.08329078023534109, 11.96623404944238978, -217.1428499060670845 ) ) ;
#21943=CARTESIAN_POINT ( 'NONE',  ( -12.67219131930435694, 19.52425521811199971, -218.0046184995277372 ) ) ;
#21944=CARTESIAN_POINT ( 'NONE',  ( -8.201407585998298444, 17.38801480109368924, -216.6295241303755006 ) ) ;
#21946=CARTESIAN_POINT ( 'NONE',  ( -23.94935377092574669, -14.34094158514532680, -226.5194954081123342 ) ) ;
#21947=CARTESIAN_POINT ( 'NONE',  ( 8.329997790135040603, 12.51216704542961899, -228.7022893680961602 ) ) ;
#21948=CARTESIAN_POINT ( 'NONE',  ( -18.88344489807484905, 1.071113352238720617, -230.0966926586188208 ) ) ;
#21950=CARTESIAN_POINT ( 'NONE',  ( -23.51371042417668633, 2.081716773471995463, -216.9231029201042418 ) ) ;
#21951=CARTESIAN_POINT ( 'NONE',  ( 17.97920459523930958, 17.43922474653955490, -233.2737719749805763 ) ) ;
#21952=MANIFOLD_SOLID_BREP ( 'Cavity1', #9021 ) ;
#21953=CARTESIAN_POINT ( 'NONE',  ( -15.82760502346409304, 5.624826830110399634, -227.5369622385896946 ) ) ;
#21954=CARTESIAN_POINT ( 'NONE',  ( 0.1866476013601106043, 25.93503619265524307, -233.5574764272258790 ) ) ;
#21955=CARTESIAN_POINT ( 'NONE',  ( 27.58248235015124550, 10.80791576765187934, -226.6933256641281389 ) ) ;
#21957=CARTESIAN_POINT ( 'NONE',  ( -17.08385316318651448, -18.56764924811779949, -215.7277288032969977 ) ) ;
#21959=CARTESIAN_POINT ( 'NONE',  ( -11.18311023676720062, -15.30649302686804347, -231.8766562234714002 ) ) ;
#21960=CARTESIAN_POINT ( 'NONE',  ( -20.02994071726468661, 1.326980477106467271, -234.9527056834518532 ) ) ;
#21961=CARTESIAN_POINT ( 'NONE',  ( 6.131461862964278531, -15.14974102410872625, -231.6805438559109973 ) ) ;
#21962=CARTESIAN_POINT ( 'NONE',  ( 14.15946391865398013, -0.7413617426029489588, -228.5799580636366670 ) ) ;
#21963=CARTESIAN_POINT ( 'NONE',  ( -16.20471097821853235, -2.781505378741172319, -220.1484675126197317 ) ) ;
#21964=CARTESIAN_POINT ( 'NONE',  ( 26.39436175479395885, 14.32821500273865034, -221.6819523832376149 ) ) ;
#21966=CARTESIAN_POINT ( 'NONE',  ( -15.63515374589483109, 24.59141623553136569, -226.9057426066772507 ) ) ;
#21967=CARTESIAN_POINT ( 'NONE',  ( 13.60311248493089131, 7.003372205918751092, -219.1738832909067867 ) ) ;
#21968=CARTESIAN_POINT ( 'NONE',  ( 21.25094435758043332, 17.68230636442804027, -229.7964888993842010 ) ) ;
#21969=CARTESIAN_POINT ( 'NONE',  ( 10.49810582199713416, 9.357428619962972149, -224.5466107281195605 ) ) ;
#21970=CARTESIAN_POINT ( 'NONE',  ( 26.45187990207246997, -15.96729416691344383, -220.4105496189887674 ) ) ;
#21971=CARTESIAN_POINT ( 'NONE',  ( -8.892156391762910062, 11.89593067802204551, -225.4519868197583889 ) ) ;
#21973=CARTESIAN_POINT ( 'NONE',  ( -15.23434562258889891, -0.4010941804143903222, -220.4743703065900036 ) ) ;
#21976=CARTESIAN_POINT ( 'NONE',  ( 16.84848658399567611, 11.39632653812981644, -217.9589513831453473 ) ) ;
#21977=CARTESIAN_POINT ( 'NONE',  ( 4.470318609411144450, -14.75491745724135306, -219.7618428768379886 ) ) ;
#21978=CARTESIAN_POINT ( 'NONE',  ( -24.18895665211001500, 11.26087434487096139, -231.0040666710689550 ) ) ;
#21979=CARTESIAN_POINT ( 'NONE',  ( 3.080453011304693511, 29.32691491905673331, -222.8956499783474499 ) ) ;
#21980=CARTESIAN_POINT ( 'NONE',  ( -18.44715843167851688, -19.86029123650958184, -231.9563062773970046 ) ) ;
#21982=CARTESIAN_POINT ( 'NONE',  ( -18.46822229429615447, 3.027586163204024405, -230.1002726880134333 ) ) ;
#21983=CIRCLE ( 'NONE', #21257, 1.000000000000000888 ) ;
#21984=CARTESIAN_POINT ( 'NONE',  ( 12.92410717862594893, 29.37236178718849189, -224.5435071569520744 ) ) ;
#21986=CARTESIAN_POINT ( 'NONE',  ( -2.934221234790329369, 15.07857928364152222, -230.9558365497803720 ) ) ;
#21987=CARTESIAN_POINT ( 'NONE',  ( 17.03334375980016446, -6.184066897328505341, -231.2622903164569834 ) ) ;
#21988=CARTESIAN_POINT ( 'NONE',  ( 24.64273247744971229, -10.07127014888436278, -217.7281412196979602 ) ) ;
#21990=CARTESIAN_POINT ( 'NONE',  ( -0.3969026096611234511, 20.89748314411456676, -216.3289738411752978 ) ) ;
#21991=CARTESIAN_POINT ( 'NONE',  ( -26.37829495954481374, -14.45191861565034053, -218.9345690753252711 ) ) ;
#21992=CARTESIAN_POINT ( 'NONE',  ( 14.65870393774896030, -26.09170264574407838, -221.2973805112574723 ) ) ;
#21993=CARTESIAN_POINT ( 'NONE',  ( 12.31511859722645852, -8.491226738247512174, -220.9006323875693738 ) ) ;
#21994=CARTESIAN_POINT ( 'NONE',  ( -15.72555926117677139, 17.60926865496976745, -217.2114552733360142 ) ) ;
#21995=CARTESIAN_POINT ( 'NONE',  ( 9.653903571287008489, 19.16609876806546353, -219.1149796918802792 ) ) ;
#21996=CARTESIAN_POINT ( 'NONE',  ( -12.44873260470819787, 7.411970124596155785, -229.4214091473984070 ) ) ;
#21997=CARTESIAN_POINT ( 'NONE',  ( -12.10258892854866275, 5.599955477755926836, -221.6590149575334010 ) ) ;
#21998=CARTESIAN_POINT ( 'NONE',  ( -12.22799442060091657, -11.48557521842085372, -222.2662941369099201 ) ) ;
#22001=CARTESIAN_POINT ( 'NONE',  ( -8.407534899841293097, 16.91942258446019665, -231.3029992963236339 ) ) ;
#22002=CARTESIAN_POINT ( 'NONE',  ( 11.96568375430165254, 8.504117401580989721, -219.8633768076029753 ) ) ;
#22003=CARTESIAN_POINT ( 'NONE',  ( 0.1866476013601106043, 25.93503619265524307, -233.5574764272258790 ) ) ;
#22004=CARTESIAN_POINT ( 'NONE',  ( 15.56514059923893178, -9.210181625211102840, -232.5361143517874325 ) ) ;
#22006=CARTESIAN_POINT ( 'NONE',  ( -17.17400284685640344, 24.63223427531467280, -220.6313524368512162 ) ) ;
#22007=CARTESIAN_POINT ( 'NONE',  ( -15.10499565381530118, -6.968761303117489980, -233.6783966751926869 ) ) ;
#22009=CARTESIAN_POINT ( 'NONE',  ( 15.33737796850231305, 13.57479350230705428, -232.3313557812109025 ) ) ;
#22012=CARTESIAN_POINT ( 'NONE',  ( 12.84024077373997841, -14.50125846907313054, -216.8496453050001946 ) ) ;
#22014=CARTESIAN_POINT ( 'NONE',  ( -20.43618815875133521, 1.403378831510147196, -232.9646741665398224 ) ) ;
#22015=CARTESIAN_POINT ( 'NONE',  ( -8.413706464639300719, 10.92140547936800843, -220.6417935981040728 ) ) ;
#22018=CARTESIAN_POINT ( 'NONE',  ( 20.88210880980788531, 0.9259446317980322139, -218.6312544800709929 ) ) ;
#22020=CARTESIAN_POINT ( 'NONE',  ( -6.266309075335420253, -15.78290365675015572, -230.2363798222519051 ) ) ;
#22023=CARTESIAN_POINT ( 'NONE',  ( 17.07668571305246985, 2.037405138410691485, -219.7626854147787867 ) ) ;
#22025=CARTESIAN_POINT ( 'NONE',  ( 20.43533161254376296, -19.75510188685668567, -224.2614117135439074 ) ) ;
#22026=CARTESIAN_POINT ( 'NONE',  ( -26.22594988380878789, -0.1068133454905619700, -219.1167922977186322 ) ) ;
#22029=CARTESIAN_POINT ( 'NONE',  ( 10.89019654021101857, 23.08162452736882031, -220.1893104909416934 ) ) ;
#22030=CARTESIAN_POINT ( 'NONE',  ( 9.167096742983094515, -14.53852251116023986, -217.0563232478103828 ) ) ;
#22031=CARTESIAN_POINT ( 'NONE',  ( 11.78320976064766690, -8.193118641535518165, -222.2581747538435479 ) ) ;
#22033=CARTESIAN_POINT ( 'NONE',  ( -22.24722865165759345, 18.77558306771206986, -226.5077042908023941 ) ) ;
#22034=CARTESIAN_POINT ( 'NONE',  ( 17.23498165643884761, 6.576565757823654934, -216.5785374982484655 ) ) ;
#22035=CARTESIAN_POINT ( 'NONE',  ( 19.31922195716811430, 9.600631919686000160, -218.1359845693048101 ) ) ;
#22037=CARTESIAN_POINT ( 'NONE',  ( -10.06242375715308945, -19.11710762076843295, -231.0938065448402199 ) ) ;
#22041=CARTESIAN_POINT ( 'NONE',  ( -21.85741505224184777, 1.741064654082184582, -235.1654459941842390 ) ) ;
#22043=CARTESIAN_POINT ( 'NONE',  ( 17.88619020626327938, 19.43517936004721847, -216.7078103882350604 ) ) ;
#22044=CARTESIAN_POINT ( 'NONE',  ( 9.413533971304945069, -13.52850967935795623, -226.9656141048783695 ) ) ;
#22045=CARTESIAN_POINT ( 'NONE',  ( 5.623554730548537606, 15.65270319720736225, -231.3185741195121068 ) ) ;
#22046=CARTESIAN_POINT ( 'NONE',  ( -22.11084984981285118, 10.96048252433489623, -216.6117774006995376 ) ) ;
#22047=CARTESIAN_POINT ( 'NONE',  ( 5.434119414999338815, 11.18343085245738777, -221.0450680983404936 ) ) ;
#22049=CARTESIAN_POINT ( 'NONE',  ( -18.63458318964815774, 8.046101765467303935, -217.8151248213926863 ) ) ;
#22050=CARTESIAN_POINT ( 'NONE',  ( -7.913358619554302642, 16.16796202616373890, -233.0981776325470491 ) ) ;
#22051=CARTESIAN_POINT ( 'NONE',  ( 18.60971343765040942, 2.368090295052050820, -218.6871071987073094 ) ) ;
#22053=CARTESIAN_POINT ( 'NONE',  ( 2.659252340503933443, 26.58135124637517777, -228.4751214701929314 ) ) ;
#22055=CYLINDRICAL_SURFACE ( 'NONE', #17094, 3.000000000000002665 ) ;
#22056=CARTESIAN_POINT ( 'NONE',  ( -19.88402822078561627, -6.951120502836210413, -232.7962440186676361 ) ) ;
#22057=CARTESIAN_POINT ( 'NONE',  ( -22.61701582078733708, 5.416317966792455252, -214.6955127214549748 ) ) ;
#22058=CARTESIAN_POINT ( 'NONE',  ( -20.64589292112740537, -18.79971917946562598, -222.0410088502282520 ) ) ;
#22060=CARTESIAN_POINT ( 'NONE',  ( -8.317278876689359279, 23.15034512777772235, -218.2935523245793092 ) ) ;
#22061=CARTESIAN_POINT ( 'NONE',  ( 1.874647746501092893, -15.20125101474619633, -222.7462710229423521 ) ) ;
#22063=CARTESIAN_POINT ( 'NONE',  ( 10.14297843322460402, 14.69845403004500639, -219.2805000163441207 ) ) ;
#22064=CARTESIAN_POINT ( 'NONE',  ( -8.030397104878142400, 15.90963402996711373, -230.6518438502475590 ) ) ;
#22065=CARTESIAN_POINT ( 'NONE',  ( -14.12265793148702464, 24.49085167151569919, -218.3312790639385241 ) ) ;
#22067=CARTESIAN_POINT ( 'NONE',  ( -15.75487091793989158, -3.404709188850186585, -225.0852311470768825 ) ) ;
#22068=CARTESIAN_POINT ( 'NONE',  ( 18.23324537670537993, 23.47692953258263771, -224.8333321331434433 ) ) ;
#22069=CARTESIAN_POINT ( 'NONE',  ( -25.06333669508177309, 2.553070212212491530, -230.2963116797556893 ) ) ;
#22070=CARTESIAN_POINT ( 'NONE',  ( -27.01279207917464475, 4.316569700791554887, -221.4451031230926219 ) ) ;
#22073=CARTESIAN_POINT ( 'NONE',  ( -26.70887854271809658, -5.532318215328999145, -217.2738835169348306 ) ) ;
#22074=CARTESIAN_POINT ( 'NONE',  ( 17.29648694364601980, 10.20782262162153842, -233.8400727604031317 ) ) ;
#22076=CARTESIAN_POINT ( 'NONE',  ( -15.32935061426341861, 5.146212415319166844, -225.5669090095357774 ) ) ;
#22077=CARTESIAN_POINT ( 'NONE',  ( 11.13671218404335761, 30.21738803452449673, -224.2405745632392211 ) ) ;
#22078=CARTESIAN_POINT ( 'NONE',  ( 14.65697969206133067, 11.40587726087447606, -233.3943609825344652 ) ) ;
#22079=CARTESIAN_POINT ( 'NONE',  ( -13.20345004609422723, -27.40577205094947644, -221.7016714442654290 ) ) ;
#22081=CARTESIAN_POINT ( 'NONE',  ( -4.879290506874147226, -14.18937706998098136, -223.0759034783553147 ) ) ;
#22082=CARTESIAN_POINT ( 'NONE',  ( -14.74212732455322161, 0.2624230007780231633, -231.8143822214177874 ) ) ;
#22083=CARTESIAN_POINT ( 'NONE',  ( 2.178520447619924472, -13.56847537563065487, -221.4085897031499428 ) ) ;
#22084=CARTESIAN_POINT ( 'NONE',  ( -10.84997096467605182, 25.01800101807719301, -232.4518260228253155 ) ) ;
#22085=CARTESIAN_POINT ( 'NONE',  ( 17.72923050078999907, -1.936365952008033853, -232.4832991314195567 ) ) ;
#22086=CARTESIAN_POINT ( 'NONE',  ( -15.89118508636071958, -1.798691612803976492, -229.3605869667087234 ) ) ;
#22087=CARTESIAN_POINT ( 'NONE',  ( 12.14863411169100971, 10.95505907656739097, -219.3725293661985063 ) ) ;
#22089=CARTESIAN_POINT ( 'NONE',  ( -10.94147694953847250, 13.90730769817462864, -218.7797619932150042 ) ) ;
#22090=CARTESIAN_POINT ( 'NONE',  ( 13.88312867625433711, 12.44451767566605760, -217.7066242262208391 ) ) ;
#22092=CARTESIAN_POINT ( 'NONE',  ( 10.83706092800007781, 10.12544885278926543, -227.1716144446442343 ) ) ;
#22093=CARTESIAN_POINT ( 'NONE',  ( 12.63974878616558328, 15.03448928898568759, -231.7036488814491406 ) ) ;
#22094=CARTESIAN_POINT ( 'NONE',  ( 7.292867580403318506, -17.79718201325288263, -215.1213547356373397 ) ) ;
#22096=CARTESIAN_POINT ( 'NONE',  ( -12.66290653391502907, 23.44312233264792411, -230.9359094203250606 ) ) ;
#22100=CARTESIAN_POINT ( 'NONE',  ( 9.471595414968767557, -23.22249338881061931, -232.1368331642201497 ) ) ;
#22101=CARTESIAN_POINT ( 'NONE',  ( -22.04240660558204823, 19.10355008918698871, -223.9524535985323723 ) ) ;
#22102=B_SPLINE_CURVE_WITH_KNOTS ( 'NONE', 3,
 ( #968, #11538, #4556, #16498, #16279, #8175, #13340, #2649, #9859, #14708, #16724, #18078, #17973, #854, #4665, #7949, #14602, #2537, #4226, #1301, #15041, #9636, #21543, #11105, #9530, #7731, #6133, #21437, #6027, #13007, #12901, #19748, #19969, #4440, #9745, #11323, #18192, #2755, #14813, #11432, #21658, #6249, #13123, #18301, #16607, #2860, #1189, #8067, #14932, #21771, #6360, #13232, #20078, #21993, #17061, #20412, #5108, #1410, #16946, #17168, #173, #7042, #10414, #4777, #20637, #3198, #20297, #10081, #17275, #3534, #12103, #11990, #20182, #3090, #18741, #13457, #18850, #11877, #8515, #8727, #5222, #9973, #10305, #15268, #1849, #3425, #10192, #15593, #11653, #18524, #1746, #16833, #3308, #6587, #13576, #8282, #4892, #15151, #18636, #11772, #1522, #18958, #8400, #22118, #6705, #5001, #1638, #15378, #22225, #6816, #13682, #20518, #8620, #15481, #54, #6927, #13797, #17506, #14135, #19065, #12546, #1965, #2401, #19178, #16143, #17613, #14355, #2073, #15709, #3640, #715, #7265, #2179, #20857, #5561, #10850, #9060, #19500, #21187, #20974, #13914, #5773, #16039, #20749, #394, #611, #12212, #12654, #14021, #2291, #19290, #10639, #4089, #5441, #10521, #12323, #10965, #17836, #3754, #9283, #17390, #8843, #5330, #7155, #15926, #7486, #8953, #286, #17724, #15817, #12439, #3867, #10747, #19393, #504, #7380, #14248, #21081, #5668, #3976, #9176, #11405, #11077, #12764, #17944, #2508, #4300, #4410, #16360, #937, #2835, #16691, #20050, #14458, #8035, #14680, #21514, #21741, #19825, #18164, #6332, #14785, #6106, #2728, #18380, #14901, #2618, #19613, #13093, #5998, #7702, #19720, #9830, #14572, #1048, #11292, #18274, #12871, #7589, #2943, #7921, #823, #9386, #11182, #21291, #4637, #21626, #6218, #19940, #1159, #9499, #4198, #5887, #16248, #21408, #9717, #18049, #7815, #12977, #16578, #16471, #9609, #4527, #13205, #11511, #22200, #21852, #18825, #8489, #18933, #1493, #18610, #6899, #12077, #20608, #20269, #8596, #1610, #13548, #6441, #5194, #18717, #13769, #15457, #16919, #10387, #8371, #30, #3397, #1272, #10056, #10279, #13310, #3508, #1381, #11964, #6676, #4865, #8147, #15124, #20152, #15352, #15012, #11742, #20383, #4977, #17145, #4745, #11624, #16806, #3281, #1721, #21963, #18496, #20493, #3172, #3057, #9946, #15241, #6788, #22086, #8257, #11852, #6556, #10166, #13428, #17035, #5083, #13657, #143, #20721, #5302, #13994, #14107, #5411, #16009, #1936, #8697 ),
 .UNSPECIFIED., .F., .F.,
 ( 4, 2, 2, 2, 2, 2, 2, 2, 2, 2, 2, 2, 2, 2, 2, 2, 2, 2, 2, 2, 2, 2, 2, 2, 2, 2, 2, 2, 2, 2, 2, 2, 2, 2, 2, 2, 2, 2, 2, 2, 2, 2, 2, 2, 2, 2, 2, 2, 2, 2, 2, 2, 2, 2, 2, 2, 2, 2, 2, 2, 2, 2, 2, 2, 2, 2, 2, 2, 2, 2, 2, 2, 2, 2, 2, 2, 2, 2, 2, 2, 2, 2, 2, 2, 2, 2, 2, 2, 2, 2, 2, 2, 2, 2, 2, 2, 2, 2, 2, 2, 2, 2, 2, 2, 2, 2, 2, 2, 2, 2, 2, 2, 2, 2, 2, 2, 2, 2, 2, 2, 2, 2, 2, 2, 2, 2, 2, 2, 2, 2, 2, 2, 2, 2, 2, 2, 2, 2, 2, 2, 2, 2, 2, 2, 2, 2, 2, 2, 2, 2, 2, 2, 2, 2, 2, 2, 2, 2, 4 ),
 ( 0.5316166001436728461, 0.5336398250262029963, 0.5353489984423374093, 0.5370581718584717112, 0.5404765186907403152, 0.5438948655230090301, 0.5473132123552777450, 0.5507315591875463490, 0.5541499060198149529, 0.5575682528520836678, 0.5609865996843523828, 0.5644049465166209867, 0.5661141199327552886, 0.5678232933488895906, 0.5712416401811581945, 0.5729508135972924965, 0.5746599870134267984, 0.5780783338456955134, 0.5814966806779642283, 0.5849150275102328322, 0.5883333743425015472, 0.5917517211747702621, 0.5951700680070388660, 0.5985884148393075810, 0.6020067616715762959, 0.6037159350877105979, 0.6054251085038448998, 0.6088434553361135038, 0.6122618021683822187, 0.6139709755845166317, 0.6156801490006509336, 0.6190984958329195376, 0.6225168426651882525, 0.6259351894974569674, 0.6293535363297255714, 0.6327718831619942863, 0.6361902299942630012, 0.6396085768265316052, 0.6430269236588003201, 0.6447360970749347331, 0.6464452704910690350, 0.6498636173233376390, 0.6532819641556063539, 0.6549911375717407669, 0.6567003109878750688, 0.6601186578201436728, 0.6635370046524122767, 0.6669553514846809916, 0.6703736983169497066, 0.6737920451492183105, 0.6772103919814870254, 0.6806287388137557404, 0.6840470856460243443, 0.6857562590621586462, 0.6866108457702257972, 0.6874654324782930592, 0.6908837793105617742, 0.6943021261428303781, 0.6960112995589646800, 0.6977204729750989820, 0.7011388198073676969, 0.7045571666396364119, 0.7079755134719050158, 0.7113938603041736197, 0.7148122071364423347, 0.7182305539687110496, 0.7216489008009796535, 0.7250672476332483685, 0.7267764210493827814, 0.7284855944655170834, 0.7319039412977856873, 0.7353222881300544023, 0.7387406349623231172, 0.7421589817945917211, 0.7455773286268603250, 0.7489956754591290400, 0.7524140222913977549, 0.7558323691236663588, 0.7592507159559350738, 0.7626690627882037887, 0.7660874096204723926, 0.7695057564527411076, 0.7729241032850098225, 0.7763424501172784264, 0.7797607969495471414, 0.7831791437818158563, 0.7865974906140844602, 0.7900158374463531752, 0.7934341842786218901, 0.7968525311108904940, 0.8002708779431590980, 0.8036892247754278129, 0.8053983981915622259, 0.8071075716076965278, 0.8105259184399651318, 0.8122350918560994337, 0.8139442652722337357, 0.8173626121045024506, 0.8207809589367711656, 0.8241993057690397695, 0.8276176526013083734, 0.8310359994335770883, 0.8344543462658458033, 0.8378726930981144072, 0.8412910399303832332, 0.8430002133465175351, 0.8447093867626518371, 0.8481277335949204410, 0.8515460804271891559, 0.8549644272594578709, 0.8583827740917264748, 0.8618011209239951897, 0.8652194677562639047, 0.8686378145885325086, 0.8720561614208012235, 0.8754745082530699385, 0.8788928550853385424, 0.8823112019176071463, 0.8857295487498758613, 0.8874387221660102743, 0.8891478955821445762, 0.8925662424144131801, 0.8942754158305474821, 0.8959845892466818951, 0.8994029360789506100, 0.9028212829112192139, 0.9062396297434879289, 0.9096579765757566438, 0.9130763234080252477, 0.9164946702402939627, 0.9199130170725626776, 0.9233313639048312815, 0.9250405373209655835, 0.9267497107370999965, 0.9301680575693687114, 0.9335864044016373153, 0.9352955778177716173, 0.9370047512339059192, 0.9404230980661746342, 0.9438414448984433491, 0.9472597917307119531, 0.9506781385629806680, 0.9540964853952493829, 0.9575148322275179869, 0.9609331790597867018, 0.9643515258920554167, 0.9660606993081897187, 0.9677698727243240207, 0.9711882195565927356, 0.9728973929727271486, 0.9746065663888614505, 0.9780249132211300545, 0.9814432600533987694, 0.9848616068856674843, 0.9882799537179360883, 0.9912099652884520662, 0.9941399768589680441, 0.9970699884294840221, 1.000000000000000000 ),
 .UNSPECIFIED. ) ;
#22103=CARTESIAN_POINT ( 'NONE',  ( 2.630208337444488453, 16.40323635460054774, -219.2570070657488088 ) ) ;
#22104=CARTESIAN_POINT ( 'NONE',  ( -26.98579662683621194, -8.531126968542736222, -229.5232528995939845 ) ) ;
#22106=CARTESIAN_POINT ( 'NONE',  ( -17.64438593497130370, 2.824953307685432069, -229.4443205246391813 ) ) ;
#22108=CARTESIAN_POINT ( 'NONE',  ( 22.90621760533471019, 17.25363305745006670, -230.8615280072714597 ) ) ;
#22110=CARTESIAN_POINT ( 'NONE',  ( -11.02345917017863464, 29.02019856777526741, -223.9475008740665771 ) ) ;
#22111=CARTESIAN_POINT ( 'NONE',  ( 27.02504508796729255, -10.76203424748690907, -225.6681254905965943 ) ) ;
#22113=CARTESIAN_POINT ( 'NONE',  ( 13.93061470302797389, -11.80544459979379646, -217.9389246709861538 ) ) ;
#22115=CARTESIAN_POINT ( 'NONE',  ( 0.9908753270255351575, 13.79205759140780430, -228.0165926715089881 ) ) ;
#22116=CARTESIAN_POINT ( 'NONE',  ( -15.39182838237880446, -1.300641671086574469, -219.0680177603771597 ) ) ;
#22117=CARTESIAN_POINT ( 'NONE',  ( -12.42894476027428929, -17.97759322220185396, -216.3110355466728834 ) ) ;
#22118=CARTESIAN_POINT ( 'NONE',  ( 8.709470447750865318, -17.43408031369701661, -216.5121658579468829 ) ) ;
#22119=CARTESIAN_POINT ( 'NONE',  ( -25.98311979368102342, 15.13734258059737670, -220.6162231662327429 ) ) ;
#22120=CARTESIAN_POINT ( 'NONE',  ( 16.49020573214642837, 22.44566021525517741, -224.7841662740084701 ) ) ;
#22121=CARTESIAN_POINT ( 'NONE',  ( -22.99617382825321599, 17.18101613848176967, -230.9512687019100099 ) ) ;
#22122=CARTESIAN_POINT ( 'NONE',  ( -12.13127060986278316, 5.971392262169284315, -229.0615017441034524 ) ) ;
#22123=CARTESIAN_POINT ( 'NONE',  ( -24.05661684749028240, -8.720095227435134433, -219.0096885115910084 ) ) ;
#22124=ORIENTED_EDGE ( 'NONE', *, *, #16914, .T. ) ;
#22125=CARTESIAN_POINT ( 'NONE',  ( -4.170472558179216804, 16.67407401355319152, -230.2690496885289804 ) ) ;
#22126=CARTESIAN_POINT ( 'NONE',  ( 25.50289296650958448, 5.998088869914441901, -233.1161630295026157 ) ) ;
#22127=CARTESIAN_POINT ( 'NONE',  ( 5.784594921161807513, 11.98867617302893329, -219.3746160931291058 ) ) ;
#22128=CARTESIAN_POINT ( 'NONE',  ( 10.05733608402134216, -9.620616164199983444, -224.9449885650552119 ) ) ;
#22131=CARTESIAN_POINT ( 'NONE',  ( -3.003186468682855104, 15.63968344752823469, -231.5301608670590667 ) ) ;
#22132=CARTESIAN_POINT ( 'NONE',  ( -24.34656557913400476, -15.24755813437383267, -217.2726941375463809 ) ) ;
#22134=CARTESIAN_POINT ( 'NONE',  ( 22.46220731426537043, 18.23201731183003460, -227.5436199598787539 ) ) ;
#22136=CARTESIAN_POINT ( 'NONE',  ( 25.46470895113276711, -14.41152162994631070, -228.1811935238409035 ) ) ;
#22138=CARTESIAN_POINT ( 'NONE',  ( -23.49379658590067876, 11.46840048879614393, -217.2519070826072323 ) ) ;
#22139=CARTESIAN_POINT ( 'NONE',  ( 17.28149325064817887, -1.074788064772476792, -229.5315781944399305 ) ) ;
#22140=CARTESIAN_POINT ( 'NONE',  ( -13.66944713747931139, -25.56883467164384527, -222.3908458502962731 ) ) ;
#22141=CARTESIAN_POINT ( 'NONE',  ( 18.06016678184731461, 2.257982981100609354, -218.9983079406065940 ) ) ;
#22143=CARTESIAN_POINT ( 'NONE',  ( 15.64298904066490259, -12.83894575744357880, -230.8789486217465594 ) ) ;
#22148=CARTESIAN_POINT ( 'NONE',  ( 11.73428189025226942, 12.46434742632455084, -228.1539301014595083 ) ) ;
#22149=CARTESIAN_POINT ( 'NONE',  ( 5.079647427451626562, 16.77877517420371234, -220.7769382327915366 ) ) ;
#22150=CARTESIAN_POINT ( 'NONE',  ( 7.820185266007354308, -13.10000580370673440, -218.6580452893993254 ) ) ;
#22151=CARTESIAN_POINT ( 'NONE',  ( 11.14834367153813233, -21.42845646353120870, -216.4520112529555718 ) ) ;
#22153=CARTESIAN_POINT ( 'NONE',  ( -11.48592899399814726, 13.65854631785387774, -230.8311022452805616 ) ) ;
#22154=CARTESIAN_POINT ( 'NONE',  ( -18.90911063232017142, 5.352531560950812839, -219.6301177803536575 ) ) ;
#22155=CARTESIAN_POINT ( 'NONE',  ( 14.65309016725241698, 3.424799466898550637, -221.5217808432381048 ) ) ;
#22157=CARTESIAN_POINT ( 'NONE',  ( -6.911745780724915633, -15.37483479843349699, -221.7918796665217656 ) ) ;
#22160=CARTESIAN_POINT ( 'NONE',  ( 8.343316395906509086, 11.57404413652245800, -231.1403332574589911 ) ) ;
#22161=CARTESIAN_POINT ( 'NONE',  ( 18.44909377000590922, -20.66544815256419199, -223.5047567001167863 ) ) ;
#22162=CARTESIAN_POINT ( 'NONE',  ( 10.07175337281514871, 14.76776740066196325, -231.7834566702614723 ) ) ;
#22163=CARTESIAN_POINT ( 'NONE',  ( -16.74550766701807447, 3.787526820511904813, -217.9802846976114381 ) ) ;
#22165=CARTESIAN_POINT ( 'NONE',  ( 24.00840102751045890, 17.37402299239434100, -218.3110108534040137 ) ) ;
#22166=CARTESIAN_POINT ( 'NONE',  ( -24.19163806436329978, 8.131440952769249719, -230.9341214615949127 ) ) ;
#22167=CARTESIAN_POINT ( 'NONE',  ( -0.1571923090946999446, 19.34188126963334398, -216.6893131123363787 ) ) ;
#22169=CARTESIAN_POINT ( 'NONE',  ( 5.668262076144046979, -25.28042871382391965, -216.8182873783340483 ) ) ;
#22170=CARTESIAN_POINT ( 'NONE',  ( 20.89700225552940793, -4.547446057044195911, -232.3806459760843666 ) ) ;
#22173=CARTESIAN_POINT ( 'NONE',  ( 24.58316096239279602, 5.861425670879941485, -231.3104446318280623 ) ) ;
#22174=CARTESIAN_POINT ( 'NONE',  ( -24.24026017931571175, -14.11860166261188354, -224.3835235244768569 ) ) ;
#22176=CARTESIAN_POINT ( 'NONE',  ( 5.377793152941013233, -17.45375835550001753, -231.2474386379397231 ) ) ;
#22177=CARTESIAN_POINT ( 'NONE',  ( 29.81944548462877975, 8.043843257819576209, -228.1755181449411793 ) ) ;
#22178=CARTESIAN_POINT ( 'NONE',  ( -10.30870167223346456, 11.95603877111467561, -228.4123369090513336 ) ) ;
#22179=CARTESIAN_POINT ( 'NONE',  ( -9.964021556040458805, 12.25789996591640119, -217.8262340283327774 ) ) ;
#22181=CARTESIAN_POINT ( 'NONE',  ( 16.57791564354289093, -3.035441731457511949, -233.7002882787241163 ) ) ;
#22183=CARTESIAN_POINT ( 'NONE',  ( 11.67669251569587985, 24.04736029062789981, -218.5856804285192254 ) ) ;
#22185=CARTESIAN_POINT ( 'NONE',  ( -15.51814470728089645, 2.949994979016113739, -222.8331727603033130 ) ) ;
#22186=CARTESIAN_POINT ( 'NONE',  ( 18.50073117969547098, -1.889592114545683987, -232.6396648696776026 ) ) ;
#22188=CARTESIAN_POINT ( 'NONE',  ( 8.903385417657583289, 10.41040586594612272, -227.6527940987422198 ) ) ;
#22189=CARTESIAN_POINT ( 'NONE',  ( -22.19349712985372491, 11.03542788991621748, -219.7744882786627443 ) ) ;
#22190=CARTESIAN_POINT ( 'NONE',  ( 1.773237071419721422, 13.09828209437875302, -220.6531024550077404 ) ) ;
#22192=CARTESIAN_POINT ( 'NONE',  ( 13.59483335902903178, 5.678732573479117640, -228.5032236586631313 ) ) ;
#22193=CARTESIAN_POINT ( 'NONE',  ( -9.208465596459861402, -9.574166310164313742, -220.4340298767933177 ) ) ;
#22195=CARTESIAN_POINT ( 'NONE',  ( -11.96638064467250473, -24.81952708901905069, -229.8544473269683692 ) ) ;
#22196=CARTESIAN_POINT ( 'NONE',  ( -8.653738780971721667, 11.12943719949617893, -219.7525355316396087 ) ) ;
#22197=CARTESIAN_POINT ( 'NONE',  ( 7.021536848793814123, -14.49751826649810482, -218.4909385705359455 ) ) ;
#22198=CARTESIAN_POINT ( 'NONE',  ( -2.698926868850080041, 12.89339462271858316, -226.7595176699009585 ) ) ;
#22199=CARTESIAN_POINT ( 'NONE',  ( 19.25263663724807728, -8.631913731826720948, -234.6583132812941983 ) ) ;
#22200=CARTESIAN_POINT ( 'NONE',  ( -13.21314811618155716, -9.038438575223175064, -230.6430079410957603 ) ) ;
#22201=CARTESIAN_POINT ( 'NONE',  ( 8.778334628954494789, 12.71782457734010841, -222.1923057070808909 ) ) ;
#22203=CARTESIAN_POINT ( 'NONE',  ( -9.115411286166651195, 13.66191091052436235, -230.3338332872444312 ) ) ;
#22204=CARTESIAN_POINT ( 'NONE',  ( 13.64836464229338198, 15.83060743948028737, -232.0893758582176929 ) ) ;
#22205=CARTESIAN_POINT ( 'NONE',  ( 14.32085100525799248, 9.220655089380342062, -219.9006227404039464 ) ) ;
#22206=CARTESIAN_POINT ( 'NONE',  ( 20.54489901492447501, 10.52141067440427591, -216.2005526543161693 ) ) ;
#22207=CARTESIAN_POINT ( 'NONE',  ( 6.835279263914467052, -26.27742004305391177, -233.7345821414606348 ) ) ;
#22208=CARTESIAN_POINT ( 'NONE',  ( -3.712761995161701911, 23.50704853188985766, -216.1220552374512067 ) ) ;
#22210=CARTESIAN_POINT ( 'NONE',  ( 13.96153919378708075, -19.04487818418218481, -231.5728976975466367 ) ) ;
#22211=CARTESIAN_POINT ( 'NONE',  ( -15.36327147092456791, 5.453733681707060299, -220.0043800961136355 ) ) ;
#22212=CARTESIAN_POINT ( 'NONE',  ( -1.772400894765090662, 19.49811434610897010, -217.8797837662441168 ) ) ;
#22213=CARTESIAN_POINT ( 'NONE',  ( -11.39823187951283501, -7.998194509987097689, -226.8062974464413912 ) ) ;
#22214=CARTESIAN_POINT ( 'NONE',  ( -24.92290506463145405, 6.124412323591598373, -220.3779252408000104 ) ) ;
#22216=CARTESIAN_POINT ( 'NONE',  ( 12.03015173539790617, 23.46358517874481109, -216.0611092640310744 ) ) ;
#22218=CARTESIAN_POINT ( 'NONE',  ( 13.43170911749896490, 19.07691563292472026, -232.7497845103644636 ) ) ;
#22219=CARTESIAN_POINT ( 'NONE',  ( 13.38912848839664704, -8.011079660592983487, -223.8512906815321628 ) ) ;
#22220=CARTESIAN_POINT ( 'NONE',  ( 15.91397826126795323, -3.183288324723350549, -218.2846031002558504 ) ) ;
#22222=CARTESIAN_POINT ( 'NONE',  ( -1.249406995060579062, 25.48934319316224162, -216.9406480707515072 ) ) ;
#22223=CARTESIAN_POINT ( 'NONE',  ( -17.20514689733751368, -7.568958929800959190, -215.6459182133127115 ) ) ;
#22224=CARTESIAN_POINT ( 'NONE',  ( -3.734153817218577309, -19.72686645808614614, -233.9207428641194610 ) ) ;
#22225=CARTESIAN_POINT ( 'NONE',  ( 6.260999666360449467, -13.19315344885661645, -220.2890618333529744 ) ) ;
#22226=CARTESIAN_POINT ( 'NONE',  ( -10.94147694953847250, 13.90730769817462864, -218.7797619932150042 ) ) ;
#22227=CARTESIAN_POINT ( 'NONE',  ( 14.72046356508972309, 21.23077830076469041, -229.4562045376679578 ) ) ;
#22228=CARTESIAN_POINT ( 'NONE',  ( -25.61997837663875188, 10.01664178086244483, -231.6711741719404074 ) ) ;
#22229=CARTESIAN_POINT ( 'NONE',  ( -11.30246491834384770, 5.534029070539333794, -225.8243940897388597 ) ) ;
#22230=CARTESIAN_POINT ( 'NONE',  ( -23.21124258271143503, -15.80671483884278317, -224.0808897361354468 ) ) ;
#22232=CARTESIAN_POINT ( 'NONE',  ( -11.16203726658389606, 26.27101666727781648, -227.8592829514190612 ) ) ;
#22233=CARTESIAN_POINT ( 'NONE',  ( 20.10109416526603709, 2.018147939476731434, -216.1034161917718848 ) ) ;
#22234=CARTESIAN_POINT ( 'NONE',  ( 17.60070748514786132, 25.68479983175475567, -229.9331108608050158 ) ) ;
#22236=CARTESIAN_POINT ( 'NONE',  ( 11.29822263435752205, -11.23247557268489771, -230.2410575525588570 ) ) ;
#22239=CARTESIAN_POINT ( 'NONE',  ( 0.4042326456706432647, 15.50845657815858303, -219.2680337625893401 ) ) ;
#22240=CARTESIAN_POINT ( 'NONE',  ( -21.94322237485859972, -13.31528874885349900, -215.4027562252440759 ) ) ;
#22242=CARTESIAN_POINT ( 'NONE',  ( 16.84848658399567611, 11.39632653812981644, -217.9589513831453473 ) ) ;
#22243=CARTESIAN_POINT ( 'NONE',  ( -28.59157645096996347, 5.137867505054540374, -220.4667042235044505 ) ) ;
#22244=CARTESIAN_POINT ( 'NONE',  ( 9.584731462935641488, -12.36622837314704348, -230.4796538097028531 ) ) ;
#22245=CARTESIAN_POINT ( 'NONE',  ( -28.99926036811508467, 3.909990568804979194, -228.9613767892386988 ) ) ;
#22246=CARTESIAN_POINT ( 'NONE',  ( 12.91815243135930480, 5.607966342865584153, -224.2227256053222959 ) ) ;
#22247=CARTESIAN_POINT ( 'NONE',  ( -1.981531036097845533, -15.05108582582333909, -227.0172948689592829 ) ) ;
#22248=CARTESIAN_POINT ( 'NONE',  ( 14.19800769603076240, 4.587407146151301518, -224.2928935459285071 ) ) ;
#22250=CARTESIAN_POINT ( 'NONE',  ( 14.67088464789753388, -9.947482835004686663, -220.6944058341955497 ) ) ;
#22251=CARTESIAN_POINT ( 'NONE',  ( 14.76992028084322683, -2.175943223131179494, -227.0668203386748019 ) ) ;
#22253=CARTESIAN_POINT ( 'NONE',  ( 12.60818910183731489, 13.02403301690871729, -229.3305689548085695 ) ) ;
#22254=CARTESIAN_POINT ( 'NONE',  ( 3.522445101072706475, 23.08420003150784439, -231.7850044194335055 ) ) ;
#22255=CARTESIAN_POINT ( 'NONE',  ( 15.68748001070188458, -20.89997441943167900, -216.2583427777263125 ) ) ;
#22256=CARTESIAN_POINT ( 'NONE',  ( 6.053458391837899910, -12.85229775019162268, -220.9645494416007523 ) ) ;
#22257=CARTESIAN_POINT ( 'NONE',  ( -14.94618804342693075, 22.09718979644185666, -219.6454806548149463 ) ) ;
#22258=CARTESIAN_POINT ( 'NONE',  ( -16.03353370602922467, 4.897644413504528060, -222.5335369890782999 ) ) ;
#22259=CARTESIAN_POINT ( 'NONE',  ( 14.72648027392381387, 10.15511732729369676, -229.5776536674053716 ) ) ;
#22260=CARTESIAN_POINT ( 'NONE',  ( -6.877419757825867563, -14.31154863906730412, -224.3431884172090918 ) ) ;
#22263=CARTESIAN_POINT ( 'NONE',  ( 15.28706223449149348, 2.473424253736659306, -227.9634568993954531 ) ) ;
#22264=CARTESIAN_POINT ( 'NONE',  ( 11.60500945006145024, -11.05507752957471190, -226.0500390094313730 ) ) ;
ENDSEC;
END-ISO-10303-21;
